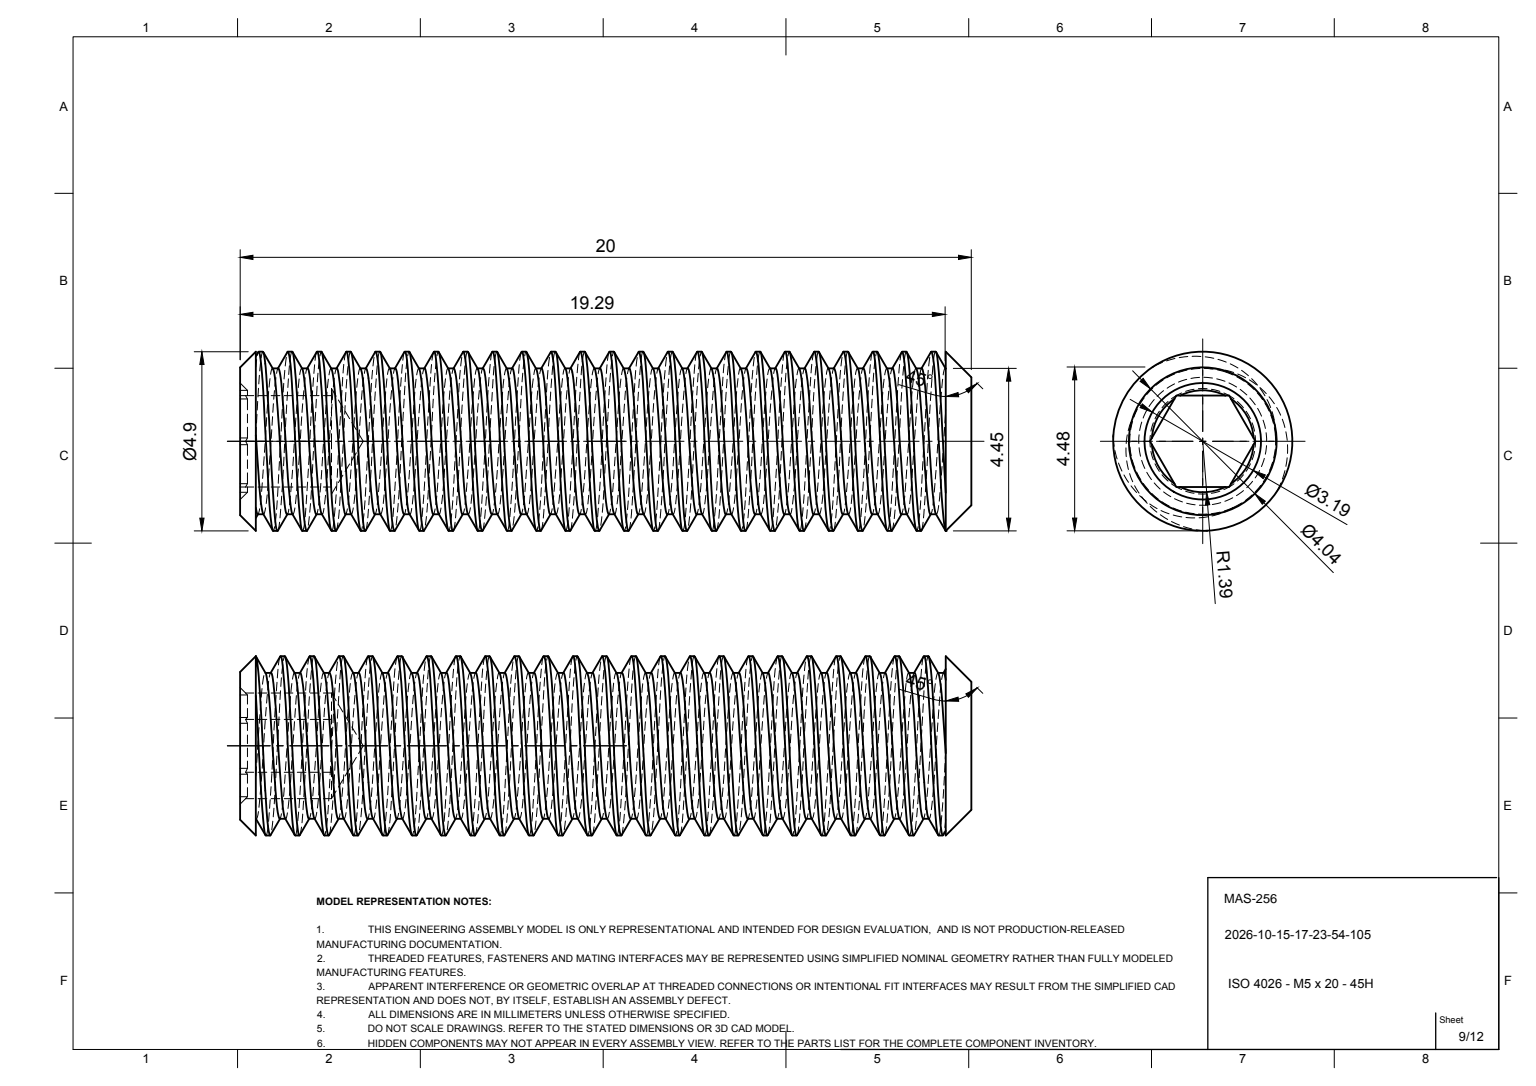
ISO-10303-21;
HEADER;
/* Generated by software containing ST-Developer
 * from STEP Tools, Inc. (www.steptools.com) 
 */

FILE_DESCRIPTION(
/* description */ (''),
/* implementation_level */ '2;1');

FILE_NAME(
/* name */ 'ISO 4026 - M5 x 20 - 45H.step',
/* time_stamp */ '2026-10-14T18:40:07-07:00',
/* author */ (''),
/* organization */ (''),
/* preprocessor_version */ 'ST-DEVELOPER v20.2',
/* originating_system */ 'Autodesk Translation Framework v15.15.0.0',
/* authorisation */ '');

FILE_SCHEMA (('AUTOMOTIVE_DESIGN { 1 0 10303 214 3 1 1 }'));
ENDSEC;

DATA;
#10=MECHANICAL_DESIGN_GEOMETRIC_PRESENTATION_REPRESENTATION('',(#838),#81040);
#344=(
BOUNDED_CURVE()
B_SPLINE_CURVE(2,(#63186,#63187,#63188),.UNSPECIFIED.,.F.,.F.)
B_SPLINE_CURVE_WITH_KNOTS((3,3),(0.,0.0126130588257634),.UNSPECIFIED.)
CURVE()
GEOMETRIC_REPRESENTATION_ITEM()
RATIONAL_B_SPLINE_CURVE((1.,1.00234596681246,1.00329298027559))
REPRESENTATION_ITEM('')
);
#345=(
BOUNDED_CURVE()
B_SPLINE_CURVE(2,(#63192,#63193,#63194),.UNSPECIFIED.,.F.,.F.)
B_SPLINE_CURVE_WITH_KNOTS((3,3),(0.0296897347922137,0.0423027936179765),
 .UNSPECIFIED.)
CURVE()
GEOMETRIC_REPRESENTATION_ITEM()
RATIONAL_B_SPLINE_CURVE((1.00329298027598,1.00234596681273,1.))
REPRESENTATION_ITEM('')
);
#346=(
BOUNDED_CURVE()
B_SPLINE_CURVE(2,(#63196,#63197,#63198),.UNSPECIFIED.,.F.,.F.)
B_SPLINE_CURVE_WITH_KNOTS((3,3),(0.,0.0126130588257622),.UNSPECIFIED.)
CURVE()
GEOMETRIC_REPRESENTATION_ITEM()
RATIONAL_B_SPLINE_CURVE((1.,1.00234596681263,1.00329298027583))
REPRESENTATION_ITEM('')
);
#347=(
BOUNDED_CURVE()
B_SPLINE_CURVE(2,(#63202,#63203,#63204),.UNSPECIFIED.,.F.,.F.)
B_SPLINE_CURVE_WITH_KNOTS((3,3),(0.0296897347922138,0.0423027936179762),
 .UNSPECIFIED.)
CURVE()
GEOMETRIC_REPRESENTATION_ITEM()
RATIONAL_B_SPLINE_CURVE((1.00329298027583,1.00234596681263,1.))
REPRESENTATION_ITEM('')
);
#348=(
BOUNDED_CURVE()
B_SPLINE_CURVE(2,(#63206,#63207,#63208),.UNSPECIFIED.,.F.,.F.)
B_SPLINE_CURVE_WITH_KNOTS((3,3),(0.,0.0126130588257628),.UNSPECIFIED.)
CURVE()
GEOMETRIC_REPRESENTATION_ITEM()
RATIONAL_B_SPLINE_CURVE((1.,1.00234596681273,1.00329298027598))
REPRESENTATION_ITEM('')
);
#349=(
BOUNDED_CURVE()
B_SPLINE_CURVE(2,(#63212,#63213,#63214),.UNSPECIFIED.,.F.,.F.)
B_SPLINE_CURVE_WITH_KNOTS((3,3),(0.0296897347922133,0.0423027936179766),
 .UNSPECIFIED.)
CURVE()
GEOMETRIC_REPRESENTATION_ITEM()
RATIONAL_B_SPLINE_CURVE((1.00329298027559,1.00234596681246,1.))
REPRESENTATION_ITEM('')
);
#350=(
BOUNDED_CURVE()
B_SPLINE_CURVE(2,(#63216,#63217,#63218),.UNSPECIFIED.,.F.,.F.)
B_SPLINE_CURVE_WITH_KNOTS((3,3),(0.,0.0126130588257654),.UNSPECIFIED.)
CURVE()
GEOMETRIC_REPRESENTATION_ITEM()
RATIONAL_B_SPLINE_CURVE((1.,1.00234596681226,1.00329298027532))
REPRESENTATION_ITEM('')
);
#351=(
BOUNDED_CURVE()
B_SPLINE_CURVE(2,(#63222,#63223,#63224),.UNSPECIFIED.,.F.,.F.)
B_SPLINE_CURVE_WITH_KNOTS((3,3),(0.029689734792212,0.0423027936179753),
 .UNSPECIFIED.)
CURVE()
GEOMETRIC_REPRESENTATION_ITEM()
RATIONAL_B_SPLINE_CURVE((1.00329298027571,1.00234596681254,1.))
REPRESENTATION_ITEM('')
);
#352=(
BOUNDED_CURVE()
B_SPLINE_CURVE(2,(#63226,#63227,#63228),.UNSPECIFIED.,.F.,.F.)
B_SPLINE_CURVE_WITH_KNOTS((3,3),(0.,0.0126130588257619),.UNSPECIFIED.)
CURVE()
GEOMETRIC_REPRESENTATION_ITEM()
RATIONAL_B_SPLINE_CURVE((1.,1.00234596681263,1.00329298027583))
REPRESENTATION_ITEM('')
);
#353=(
BOUNDED_CURVE()
B_SPLINE_CURVE(2,(#63232,#63233,#63234),.UNSPECIFIED.,.F.,.F.)
B_SPLINE_CURVE_WITH_KNOTS((3,3),(0.0296897347922146,0.0423027936179762),
 .UNSPECIFIED.)
CURVE()
GEOMETRIC_REPRESENTATION_ITEM()
RATIONAL_B_SPLINE_CURVE((1.00329298027583,1.00234596681263,1.))
REPRESENTATION_ITEM('')
);
#354=(
BOUNDED_CURVE()
B_SPLINE_CURVE(2,(#63236,#63237,#63238),.UNSPECIFIED.,.F.,.F.)
B_SPLINE_CURVE_WITH_KNOTS((3,3),(0.,0.0126130588257574),.UNSPECIFIED.)
CURVE()
GEOMETRIC_REPRESENTATION_ITEM()
RATIONAL_B_SPLINE_CURVE((1.,1.002345966813,1.00329298027635))
REPRESENTATION_ITEM('')
);
#355=(
BOUNDED_CURVE()
B_SPLINE_CURVE(2,(#63241,#63242,#63243),.UNSPECIFIED.,.F.,.F.)
B_SPLINE_CURVE_WITH_KNOTS((3,3),(0.029689734792213,0.0423027936179761),
 .UNSPECIFIED.)
CURVE()
GEOMETRIC_REPRESENTATION_ITEM()
RATIONAL_B_SPLINE_CURVE((1.00329298027557,1.00234596681244,1.))
REPRESENTATION_ITEM('')
);
#366=B_SPLINE_SURFACE_WITH_KNOTS('',3,3,((#61760,#61761,#61762,#61763,#61764,
#61765,#61766,#61767,#61768,#61769,#61770,#61771,#61772,#61773,#61774,#61775,
#61776,#61777,#61778,#61779,#61780,#61781,#61782,#61783,#61784,#61785,#61786,
#61787,#61788,#61789,#61790,#61791,#61792,#61793,#61794,#61795,#61796,#61797,
#61798,#61799,#61800,#61801,#61802,#61803,#61804,#61805,#61806,#61807,#61808,
#61809,#61810,#61811,#61812,#61813,#61814,#61815,#61816,#61817,#61818,#61819,
#61820,#61821,#61822,#61823,#61824,#61825,#61826,#61827,#61828,#61829,#61830,
#61831,#61832,#61833,#61834,#61835,#61836,#61837,#61838,#61839,#61840,#61841,
#61842,#61843,#61844,#61845,#61846,#61847,#61848,#61849,#61850,#61851,#61852,
#61853,#61854,#61855,#61856,#61857,#61858,#61859,#61860,#61861,#61862,#61863,
#61864,#61865,#61866,#61867,#61868,#61869,#61870,#61871,#61872,#61873,#61874,
#61875,#61876,#61877,#61878,#61879,#61880,#61881,#61882,#61883,#61884,#61885,
#61886,#61887,#61888,#61889,#61890,#61891,#61892,#61893,#61894,#61895,#61896,
#61897,#61898,#61899,#61900,#61901,#61902,#61903,#61904,#61905,#61906,#61907,
#61908,#61909,#61910,#61911,#61912,#61913),(#61914,#61915,#61916,#61917,
#61918,#61919,#61920,#61921,#61922,#61923,#61924,#61925,#61926,#61927,#61928,
#61929,#61930,#61931,#61932,#61933,#61934,#61935,#61936,#61937,#61938,#61939,
#61940,#61941,#61942,#61943,#61944,#61945,#61946,#61947,#61948,#61949,#61950,
#61951,#61952,#61953,#61954,#61955,#61956,#61957,#61958,#61959,#61960,#61961,
#61962,#61963,#61964,#61965,#61966,#61967,#61968,#61969,#61970,#61971,#61972,
#61973,#61974,#61975,#61976,#61977,#61978,#61979,#61980,#61981,#61982,#61983,
#61984,#61985,#61986,#61987,#61988,#61989,#61990,#61991,#61992,#61993,#61994,
#61995,#61996,#61997,#61998,#61999,#62000,#62001,#62002,#62003,#62004,#62005,
#62006,#62007,#62008,#62009,#62010,#62011,#62012,#62013,#62014,#62015,#62016,
#62017,#62018,#62019,#62020,#62021,#62022,#62023,#62024,#62025,#62026,#62027,
#62028,#62029,#62030,#62031,#62032,#62033,#62034,#62035,#62036,#62037,#62038,
#62039,#62040,#62041,#62042,#62043,#62044,#62045,#62046,#62047,#62048,#62049,
#62050,#62051,#62052,#62053,#62054,#62055,#62056,#62057,#62058,#62059,#62060,
#62061,#62062,#62063,#62064,#62065,#62066,#62067),(#62068,#62069,#62070,
#62071,#62072,#62073,#62074,#62075,#62076,#62077,#62078,#62079,#62080,#62081,
#62082,#62083,#62084,#62085,#62086,#62087,#62088,#62089,#62090,#62091,#62092,
#62093,#62094,#62095,#62096,#62097,#62098,#62099,#62100,#62101,#62102,#62103,
#62104,#62105,#62106,#62107,#62108,#62109,#62110,#62111,#62112,#62113,#62114,
#62115,#62116,#62117,#62118,#62119,#62120,#62121,#62122,#62123,#62124,#62125,
#62126,#62127,#62128,#62129,#62130,#62131,#62132,#62133,#62134,#62135,#62136,
#62137,#62138,#62139,#62140,#62141,#62142,#62143,#62144,#62145,#62146,#62147,
#62148,#62149,#62150,#62151,#62152,#62153,#62154,#62155,#62156,#62157,#62158,
#62159,#62160,#62161,#62162,#62163,#62164,#62165,#62166,#62167,#62168,#62169,
#62170,#62171,#62172,#62173,#62174,#62175,#62176,#62177,#62178,#62179,#62180,
#62181,#62182,#62183,#62184,#62185,#62186,#62187,#62188,#62189,#62190,#62191,
#62192,#62193,#62194,#62195,#62196,#62197,#62198,#62199,#62200,#62201,#62202,
#62203,#62204,#62205,#62206,#62207,#62208,#62209,#62210,#62211,#62212,#62213,
#62214,#62215,#62216,#62217,#62218,#62219,#62220,#62221),(#62222,#62223,
#62224,#62225,#62226,#62227,#62228,#62229,#62230,#62231,#62232,#62233,#62234,
#62235,#62236,#62237,#62238,#62239,#62240,#62241,#62242,#62243,#62244,#62245,
#62246,#62247,#62248,#62249,#62250,#62251,#62252,#62253,#62254,#62255,#62256,
#62257,#62258,#62259,#62260,#62261,#62262,#62263,#62264,#62265,#62266,#62267,
#62268,#62269,#62270,#62271,#62272,#62273,#62274,#62275,#62276,#62277,#62278,
#62279,#62280,#62281,#62282,#62283,#62284,#62285,#62286,#62287,#62288,#62289,
#62290,#62291,#62292,#62293,#62294,#62295,#62296,#62297,#62298,#62299,#62300,
#62301,#62302,#62303,#62304,#62305,#62306,#62307,#62308,#62309,#62310,#62311,
#62312,#62313,#62314,#62315,#62316,#62317,#62318,#62319,#62320,#62321,#62322,
#62323,#62324,#62325,#62326,#62327,#62328,#62329,#62330,#62331,#62332,#62333,
#62334,#62335,#62336,#62337,#62338,#62339,#62340,#62341,#62342,#62343,#62344,
#62345,#62346,#62347,#62348,#62349,#62350,#62351,#62352,#62353,#62354,#62355,
#62356,#62357,#62358,#62359,#62360,#62361,#62362,#62363,#62364,#62365,#62366,
#62367,#62368,#62369,#62370,#62371,#62372,#62373,#62374,#62375)),
 .UNSPECIFIED.,.F.,.F.,.F.,(4,4),(4,1,1,1,1,1,1,1,1,1,1,1,1,1,1,1,1,1,1,
1,1,1,1,1,1,1,1,1,1,1,1,1,1,1,1,1,1,1,1,1,1,1,1,1,1,1,1,1,1,1,1,1,1,1,1,
1,1,1,1,1,1,1,1,1,1,1,1,1,1,1,1,1,1,1,1,1,1,1,1,1,1,1,1,1,1,1,1,1,1,1,1,
1,1,1,1,1,1,1,1,1,1,1,1,1,1,1,1,1,1,1,1,1,1,1,1,1,1,1,1,1,1,1,1,1,1,1,1,
1,1,1,1,1,1,1,1,1,1,1,1,1,1,1,1,1,1,1,1,1,1,1,1,4),(-0.000410693813861421,
0.0529897430905959),(8.30815772716268,9.30327942982552,10.2984011324884,
11.2935228351512,12.288644537814,13.2837662404769,14.2788879431397,15.2740096458026,
16.2691313484654,17.2642530511282,18.2593747537911,19.2544964564539,20.2496181591168,
21.2447398617796,22.2398615644424,23.2349832671053,24.2301049697681,25.225226672431,
26.2203483750938,27.2154700777567,28.2105917804195,29.2057134830823,30.2008351857452,
31.195956888408,32.1910785910709,33.1862002937337,34.1813219963965,35.1764436990594,
36.1715654017222,37.1666871043851,38.1618088070479,39.1569305097107,40.1520522123736,
41.1471739150364,42.1422956176993,43.1374173203621,44.132539023025,45.1276607256878,
46.1227824283506,47.1179041310135,48.1130258336763,49.1081475363392,50.103269239002,
51.0983909416648,52.0935126443277,53.0886343469905,54.0837560496534,55.0788777523162,
56.073999454979,57.0691211576419,58.0642428603047,59.0593645629676,60.0544862656304,
61.0496079682933,62.0447296709561,63.0398513736189,64.0349730762818,65.0300947789446,
66.0252164816075,67.0203381842703,68.0154598869331,69.010581589596,70.0057032922588,
71.0008249949217,71.9959466975845,72.9910684002473,73.9861901029102,74.981311805573,
75.9764335082359,76.9715552108987,77.9666769135615,78.9617986162244,79.9569203188872,
80.9520420215501,81.9471637242129,82.9422854268758,83.9374071295386,84.9325288322014,
85.9276505348643,86.9227722375271,87.91789394019,88.9130156428528,89.9081373455156,
90.9032590481785,91.8983807508413,92.8935024535042,93.888624156167,94.8837458588298,
95.8788675614927,96.8739892641555,97.8691109668184,98.8642326694812,99.859354372144,
100.854476074807,101.84959777747,102.844719480133,103.839841182795,104.834962885458,
105.830084588121,106.825206290784,107.820327993447,108.81544969611,109.810571398772,
110.805693101435,111.800814804098,112.795936506761,113.791058209424,114.786179912087,
115.781301614749,116.776423317412,117.771545020075,118.766666722738,119.761788425401,
120.756910128064,121.752031830727,122.747153533389,123.742275236052,124.737396938715,
125.732518641378,126.727640344041,127.722762046704,128.717883749366,129.713005452029,
130.708127154692,131.703248857355,132.698370560018,133.693492262681,134.688613965343,
135.683735668006,136.678857370669,137.673979073332,138.669100775995,139.664222478658,
140.659344181321,141.654465883983,142.649587586646,143.644709289309,144.639830991972,
145.634952694635,146.630074397298,147.62519609996,148.620317802623,149.615439505286,
150.610561207949,151.605682910612,152.600804613275,153.595926315937,154.5910480186,
155.586169721263,156.581291423926,157.576413126589,158.571945523066),
 .UNSPECIFIED.);
#367=B_SPLINE_SURFACE_WITH_KNOTS('',3,3,((#62563,#62564,#62565,#62566,#62567,
#62568,#62569,#62570,#62571,#62572,#62573,#62574,#62575,#62576,#62577,#62578,
#62579,#62580,#62581,#62582,#62583,#62584,#62585,#62586,#62587,#62588,#62589,
#62590,#62591,#62592,#62593,#62594,#62595,#62596,#62597,#62598,#62599,#62600,
#62601,#62602,#62603,#62604,#62605,#62606,#62607,#62608,#62609,#62610,#62611,
#62612,#62613,#62614,#62615,#62616,#62617,#62618,#62619,#62620,#62621,#62622,
#62623,#62624,#62625,#62626,#62627,#62628,#62629,#62630,#62631,#62632,#62633,
#62634,#62635,#62636,#62637,#62638,#62639,#62640,#62641,#62642,#62643,#62644,
#62645,#62646,#62647,#62648,#62649,#62650,#62651,#62652,#62653,#62654,#62655,
#62656,#62657,#62658,#62659,#62660,#62661,#62662,#62663,#62664,#62665,#62666,
#62667,#62668,#62669,#62670,#62671,#62672,#62673,#62674,#62675,#62676,#62677,
#62678,#62679,#62680,#62681,#62682,#62683,#62684,#62685,#62686,#62687,#62688,
#62689,#62690,#62691,#62692,#62693,#62694,#62695,#62696,#62697,#62698,#62699,
#62700,#62701,#62702,#62703,#62704,#62705,#62706,#62707,#62708,#62709,#62710,
#62711,#62712,#62713,#62714,#62715,#62716),(#62717,#62718,#62719,#62720,
#62721,#62722,#62723,#62724,#62725,#62726,#62727,#62728,#62729,#62730,#62731,
#62732,#62733,#62734,#62735,#62736,#62737,#62738,#62739,#62740,#62741,#62742,
#62743,#62744,#62745,#62746,#62747,#62748,#62749,#62750,#62751,#62752,#62753,
#62754,#62755,#62756,#62757,#62758,#62759,#62760,#62761,#62762,#62763,#62764,
#62765,#62766,#62767,#62768,#62769,#62770,#62771,#62772,#62773,#62774,#62775,
#62776,#62777,#62778,#62779,#62780,#62781,#62782,#62783,#62784,#62785,#62786,
#62787,#62788,#62789,#62790,#62791,#62792,#62793,#62794,#62795,#62796,#62797,
#62798,#62799,#62800,#62801,#62802,#62803,#62804,#62805,#62806,#62807,#62808,
#62809,#62810,#62811,#62812,#62813,#62814,#62815,#62816,#62817,#62818,#62819,
#62820,#62821,#62822,#62823,#62824,#62825,#62826,#62827,#62828,#62829,#62830,
#62831,#62832,#62833,#62834,#62835,#62836,#62837,#62838,#62839,#62840,#62841,
#62842,#62843,#62844,#62845,#62846,#62847,#62848,#62849,#62850,#62851,#62852,
#62853,#62854,#62855,#62856,#62857,#62858,#62859,#62860,#62861,#62862,#62863,
#62864,#62865,#62866,#62867,#62868,#62869,#62870),(#62871,#62872,#62873,
#62874,#62875,#62876,#62877,#62878,#62879,#62880,#62881,#62882,#62883,#62884,
#62885,#62886,#62887,#62888,#62889,#62890,#62891,#62892,#62893,#62894,#62895,
#62896,#62897,#62898,#62899,#62900,#62901,#62902,#62903,#62904,#62905,#62906,
#62907,#62908,#62909,#62910,#62911,#62912,#62913,#62914,#62915,#62916,#62917,
#62918,#62919,#62920,#62921,#62922,#62923,#62924,#62925,#62926,#62927,#62928,
#62929,#62930,#62931,#62932,#62933,#62934,#62935,#62936,#62937,#62938,#62939,
#62940,#62941,#62942,#62943,#62944,#62945,#62946,#62947,#62948,#62949,#62950,
#62951,#62952,#62953,#62954,#62955,#62956,#62957,#62958,#62959,#62960,#62961,
#62962,#62963,#62964,#62965,#62966,#62967,#62968,#62969,#62970,#62971,#62972,
#62973,#62974,#62975,#62976,#62977,#62978,#62979,#62980,#62981,#62982,#62983,
#62984,#62985,#62986,#62987,#62988,#62989,#62990,#62991,#62992,#62993,#62994,
#62995,#62996,#62997,#62998,#62999,#63000,#63001,#63002,#63003,#63004,#63005,
#63006,#63007,#63008,#63009,#63010,#63011,#63012,#63013,#63014,#63015,#63016,
#63017,#63018,#63019,#63020,#63021,#63022,#63023,#63024),(#63025,#63026,
#63027,#63028,#63029,#63030,#63031,#63032,#63033,#63034,#63035,#63036,#63037,
#63038,#63039,#63040,#63041,#63042,#63043,#63044,#63045,#63046,#63047,#63048,
#63049,#63050,#63051,#63052,#63053,#63054,#63055,#63056,#63057,#63058,#63059,
#63060,#63061,#63062,#63063,#63064,#63065,#63066,#63067,#63068,#63069,#63070,
#63071,#63072,#63073,#63074,#63075,#63076,#63077,#63078,#63079,#63080,#63081,
#63082,#63083,#63084,#63085,#63086,#63087,#63088,#63089,#63090,#63091,#63092,
#63093,#63094,#63095,#63096,#63097,#63098,#63099,#63100,#63101,#63102,#63103,
#63104,#63105,#63106,#63107,#63108,#63109,#63110,#63111,#63112,#63113,#63114,
#63115,#63116,#63117,#63118,#63119,#63120,#63121,#63122,#63123,#63124,#63125,
#63126,#63127,#63128,#63129,#63130,#63131,#63132,#63133,#63134,#63135,#63136,
#63137,#63138,#63139,#63140,#63141,#63142,#63143,#63144,#63145,#63146,#63147,
#63148,#63149,#63150,#63151,#63152,#63153,#63154,#63155,#63156,#63157,#63158,
#63159,#63160,#63161,#63162,#63163,#63164,#63165,#63166,#63167,#63168,#63169,
#63170,#63171,#63172,#63173,#63174,#63175,#63176,#63177,#63178)),
 .UNSPECIFIED.,.F.,.F.,.F.,(4,4),(4,1,1,1,1,1,1,1,1,1,1,1,1,1,1,1,1,1,1,
1,1,1,1,1,1,1,1,1,1,1,1,1,1,1,1,1,1,1,1,1,1,1,1,1,1,1,1,1,1,1,1,1,1,1,1,
1,1,1,1,1,1,1,1,1,1,1,1,1,1,1,1,1,1,1,1,1,1,1,1,1,1,1,1,1,1,1,1,1,1,1,1,
1,1,1,1,1,1,1,1,1,1,1,1,1,1,1,1,1,1,1,1,1,1,1,1,1,1,1,1,1,1,1,1,1,1,1,1,
1,1,1,1,1,1,1,1,1,1,1,1,1,1,1,1,1,1,1,1,1,1,1,1,4),(-0.000364258179702487,
0.0530361410367657),(11.6159825333414,12.6115149000043,13.6066366026672,
14.60175830533,15.5968800079929,16.5920017106557,17.5871234133185,18.5822451159814,
19.5773668186442,20.5724885213071,21.5676102239699,22.5627319266327,23.5578536292956,
24.5529753319584,25.5480970346213,26.5432187372841,27.5383404399469,28.5334621426098,
29.5285838452726,30.5237055479355,31.5188272505983,32.5139489532611,33.509070655924,
34.5041923585868,35.4993140612497,36.4944357639125,37.4895574665754,38.4846791692382,
39.479800871901,40.4749225745639,41.4700442772267,42.4651659798896,43.4602876825524,
44.4554093852152,45.4505310878781,46.4456527905409,47.4407744932038,48.4358961958666,
49.4310178985294,50.4261396011923,51.4212613038551,52.416383006518,53.4115047091808,
54.4066264118436,55.4017481145065,56.3968698171693,57.3919915198322,58.387113222495,
59.3822349251579,60.3773566278207,61.3724783304835,62.3676000331464,63.3627217358092,
64.3578434384721,65.3529651411349,66.3480868437977,67.3432085464606,68.3383302491234,
69.3334519517863,70.3285736544491,71.3236953571119,72.3188170597748,73.3139387624376,
74.3090604651005,75.3041821677633,76.2993038704262,77.294425573089,78.2895472757518,
79.2846689784147,80.2797906810775,81.2749123837404,82.2700340864032,83.265155789066,
84.2602774917289,85.2553991943917,86.2505208970546,87.2456425997174,88.2407643023802,
89.2358860050431,90.2310077077059,91.2261294103688,92.2212511130316,93.2163728156945,
94.2114945183573,95.2066162210201,96.201737923683,97.1968596263458,98.1919813290087,
99.1871030316715,100.182224734334,101.177346436997,102.17246813966,103.167589842323,
104.162711544986,105.157833247649,106.152954950311,107.148076652974,108.143198355637,
109.1383200583,110.133441760963,111.128563463626,112.123685166288,113.118806868951,
114.113928571614,115.109050274277,116.10417197694,117.099293679603,118.094415382265,
119.089537084928,120.084658787591,121.079780490254,122.074902192917,123.07002389558,
124.065145598243,125.060267300905,126.055389003568,127.050510706231,128.045632408894,
129.040754111557,130.03587581422,131.030997516882,132.026119219545,133.021240922208,
134.016362624871,135.011484327534,136.006606030197,137.001727732859,137.996849435522,
138.991971138185,139.987092840848,140.982214543511,141.977336246174,142.972457948837,
143.967579651499,144.962701354162,145.957823056825,146.952944759488,147.948066462151,
148.943188164814,149.938309867476,150.933431570139,151.928553272802,152.923674975465,
153.918796678128,154.913918380791,155.909040083453,156.904161786116,157.899283488779,
158.894405191442,159.889526894105,160.884648596768,161.87977029943),
 .UNSPECIFIED.);
#543=B_SPLINE_CURVE_WITH_KNOTS('',3,(#43212,#43213,#43214,#43215,#43216,
#43217,#43218,#43219,#43220,#43221,#43222,#43223,#43224,#43225,#43226,#43227,
#43228,#43229,#43230,#43231,#43232,#43233,#43234,#43235,#43236,#43237,#43238,
#43239,#43240,#43241,#43242,#43243,#43244,#43245,#43246,#43247,#43248,#43249,
#43250,#43251,#43252,#43253,#43254,#43255,#43256,#43257,#43258,#43259,#43260,
#43261,#43262,#43263,#43264,#43265,#43266,#43267,#43268,#43269,#43270,#43271,
#43272,#43273,#43274,#43275,#43276,#43277,#43278,#43279,#43280,#43281,#43282,
#43283,#43284,#43285,#43286,#43287,#43288,#43289,#43290,#43291,#43292,#43293,
#43294,#43295,#43296,#43297,#43298,#43299,#43300,#43301,#43302,#43303,#43304,
#43305,#43306,#43307,#43308,#43309,#43310,#43311,#43312,#43313,#43314,#43315,
#43316,#43317,#43318,#43319,#43320,#43321,#43322,#43323,#43324,#43325,#43326,
#43327,#43328,#43329,#43330,#43331,#43332,#43333,#43334,#43335,#43336,#43337,
#43338,#43339,#43340,#43341,#43342,#43343,#43344,#43345,#43346,#43347,#43348,
#43349,#43350,#43351,#43352,#43353,#43354,#43355,#43356,#43357,#43358,#43359,
#43360,#43361,#43362,#43363,#43364,#43365,#43366,#43367,#43368,#43369,#43370,
#43371,#43372,#43373,#43374,#43375,#43376,#43377,#43378,#43379,#43380,#43381,
#43382,#43383,#43384,#43385),.UNSPECIFIED.,.F.,.F.,(4,2,2,2,2,2,2,2,2,2,
2,2,2,2,2,2,2,2,2,2,2,2,2,2,2,2,2,2,2,2,2,2,2,2,2,2,2,2,2,2,2,2,2,2,2,2,
2,2,2,2,2,2,2,2,2,2,2,2,2,2,2,2,2,2,2,2,2,2,2,2,2,2,2,2,2,2,2,2,2,2,2,2,
2,2,2,2,4),(-1.02623154465591,-1.02612355094225,-1.0171949105878,-1.00173095718431,
-0.985469014925391,-0.982771946333453,-0.981106865955899,-0.979811649677182,
-0.978304805833221,-0.975593204166809,-0.962004888593598,-0.929009570235146,
-0.890102622931837,-0.885357205821845,-0.882392485048737,-0.88007255803002,
-0.87749442072948,-0.873218763358691,-0.856815386493199,-0.795998925748137,
-0.785774339547155,-0.783194740653446,-0.781700335240677,-0.780528775129861,
-0.778903222255259,-0.775642448166408,-0.771379179015789,-0.761149449011797,
-0.715168121526073,-0.690933730558083,-0.686443744461884,-0.683553504484392,
-0.681237215680206,-0.678604823233647,-0.674096245039031,-0.654637962169762,
-0.609759140741896,-0.587984786080504,-0.584837995230912,-0.583218043592144,
-0.581928744021515,-0.580398002638214,-0.577543750440399,-0.560583467376236,
-0.531668237094072,-0.491978203796283,-0.487259509009561,-0.48431303144165,
-0.482008603588994,-0.479449131679121,-0.475208298310883,-0.459005836096745,
-0.427573337459186,-0.416862164322599,-0.411468759639921,-0.388730249711721,
-0.385591832645818,-0.383978822110257,-0.382688106401478,-0.381143962853957,
-0.378268391996503,-0.361258822960958,-0.332370712217255,-0.292727546811052,
-0.287970926659497,-0.28499512806325,-0.282663948925388,-0.28007054667004,
-0.275762761562799,-0.259131125602471,-0.194877347651408,-0.187936721290845,
-0.185704718486579,-0.184300457443206,-0.182978277960871,-0.181156364600397,
-0.176843676191297,-0.156826183459693,-0.104384960191217,-0.0934748581158038,
-0.0896010514422441,-0.0873381573714681,-0.0849755616014679,-0.0818995433479831,
-0.0753249891341137,-0.0493613703757626,-0.00320473719929889),
 .UNSPECIFIED.);
#544=B_SPLINE_CURVE_WITH_KNOTS('',3,(#43388,#43389,#43390,#43391,#43392,
#43393,#43394,#43395,#43396,#43397,#43398,#43399,#43400,#43401,#43402,#43403,
#43404,#43405,#43406,#43407,#43408,#43409,#43410,#43411,#43412,#43413,#43414,
#43415,#43416,#43417,#43418,#43419,#43420,#43421,#43422,#43423,#43424,#43425,
#43426,#43427,#43428,#43429,#43430,#43431,#43432,#43433,#43434,#43435,#43436,
#43437,#43438,#43439,#43440,#43441,#43442,#43443,#43444,#43445,#43446,#43447,
#43448,#43449,#43450,#43451,#43452,#43453,#43454,#43455,#43456,#43457,#43458,
#43459,#43460,#43461,#43462,#43463,#43464,#43465,#43466,#43467,#43468,#43469,
#43470,#43471,#43472,#43473,#43474,#43475,#43476,#43477,#43478,#43479,#43480,
#43481,#43482,#43483,#43484,#43485,#43486,#43487,#43488,#43489,#43490,#43491,
#43492,#43493,#43494,#43495,#43496,#43497,#43498,#43499,#43500,#43501,#43502,
#43503,#43504,#43505),.UNSPECIFIED.,.F.,.F.,(4,3,3,3,3,3,3,3,3,3,3,3,3,
3,3,3,3,3,3,3,3,3,3,3,3,3,3,3,3,3,3,3,3,3,3,3,3,3,3,4),(11.6163931973415,
11.7237672656018,11.8347357199021,11.9420294578483,12.0493244336209,12.1566495119213,
12.264033585161,12.3715827272617,12.4792279734473,12.5870706422788,12.6115149000043,
12.7155317843677,12.8193765837255,12.9230806912589,13.0267085981463,13.1302971854635,
13.2338832777977,13.3375740056834,13.4413213587812,13.5452523118071,13.6066366026672,
13.7117447872625,13.8166959584208,13.9215236686367,14.0262853677174,14.1310163775997,
14.2357519758657,14.3405953724673,14.4454990552932,14.5505798283899,14.60175830533,
14.7069309232771,14.8119246326924,14.9168178106501,15.0216457587039,15.1264436979783,
15.2312999910099,15.3361865597888,15.4412122486148,15.503392487373),
 .UNSPECIFIED.);
#545=B_SPLINE_CURVE_WITH_KNOTS('',3,(#43510,#43511,#43512,#43513,#43514,
#43515,#43516,#43517,#43518,#43519,#43520,#43521,#43522,#43523,#43524,#43525,
#43526,#43527,#43528,#43529,#43530,#43531,#43532,#43533,#43534,#43535,#43536,
#43537,#43538,#43539,#43540,#43541,#43542,#43543,#43544,#43545,#43546,#43547,
#43548,#43549,#43550,#43551,#43552,#43553,#43554,#43555,#43556,#43557,#43558,
#43559,#43560,#43561,#43562,#43563,#43564,#43565,#43566,#43567,#43568,#43569,
#43570,#43571,#43572,#43573,#43574,#43575,#43576,#43577,#43578,#43579,#43580,
#43581,#43582,#43583,#43584,#43585,#43586,#43587,#43588,#43589,#43590,#43591,
#43592,#43593,#43594,#43595,#43596,#43597,#43598,#43599,#43600,#43601,#43602,
#43603,#43604,#43605,#43606,#43607,#43608,#43609,#43610,#43611,#43612,#43613,
#43614,#43615,#43616,#43617,#43618,#43619,#43620,#43621,#43622,#43623,#43624,
#43625,#43626,#43627,#43628,#43629,#43630,#43631,#43632,#43633,#43634,#43635,
#43636,#43637,#43638,#43639,#43640,#43641,#43642,#43643,#43644,#43645,#43646,
#43647,#43648,#43649,#43650,#43651,#43652,#43653,#43654,#43655,#43656,#43657,
#43658,#43659,#43660,#43661,#43662,#43663,#43664,#43665,#43666,#43667,#43668,
#43669,#43670,#43671,#43672,#43673,#43674,#43675,#43676,#43677,#43678,#43679,
#43680,#43681,#43682,#43683,#43684,#43685,#43686,#43687,#43688,#43689,#43690,
#43691,#43692,#43693,#43694,#43695,#43696,#43697,#43698,#43699,#43700,#43701,
#43702,#43703,#43704,#43705,#43706,#43707,#43708,#43709,#43710,#43711,#43712,
#43713,#43714,#43715,#43716,#43717,#43718,#43719,#43720,#43721,#43722,#43723,
#43724,#43725,#43726,#43727),.UNSPECIFIED.,.F.,.F.,(4,2,2,2,2,2,2,2,2,2,
2,2,2,2,2,2,2,2,2,2,2,2,2,2,2,2,2,2,2,2,2,2,2,2,2,2,2,2,2,2,2,2,2,2,2,2,
2,2,2,2,2,2,2,2,2,2,2,2,2,2,2,2,2,2,2,2,2,2,2,2,2,2,2,2,2,2,2,2,2,2,2,2,
2,2,2,2,2,2,2,2,2,2,2,2,2,2,2,2,2,2,2,2,2,2,2,2,2,2,4),(-2.28248600441818,
-2.2811956203742,-2.27687867721623,-2.27429210537512,-2.27220672013212,
-2.26937453435887,-2.26390906147731,-2.22240610456411,-2.1817125094513,
-2.17715654769303,-2.17543396354253,-2.17420503146357,-2.17287531524768,
-2.17098113067247,-2.16619035367949,-2.15916593209376,-2.13720086913996,
-2.08636498668884,-2.07952178065835,-2.07645687560523,-2.07411645664894,
-2.07161205809893,-2.06766952812952,-2.05478977904954,-2.03300524837185,
-2.00749534956624,-1.98067095547916,-1.97747634366124,-1.97584649129612,
-1.97455315241394,-1.97301858782097,-1.97017919487622,-1.9539413515156,
-1.89828031814689,-1.88325787526814,-1.87893503696039,-1.87634720382067,
-1.87426208439326,-1.87143195211724,-1.86597629628848,-1.82340189586034,
-1.78382863243893,-1.7792291896914,-1.77750098335071,-1.77627059073702,
-1.77494229662179,-1.77305485838914,-1.76830562448201,-1.74354356694527,
-1.70296881418663,-1.68482176820919,-1.6802749108557,-1.67761170307872,
-1.67530475013581,-1.67247298103653,-1.66700863526789,-1.62565360567816,
-1.58480006736649,-1.58025253527128,-1.57853116236556,-1.57730263481814,
-1.5759727918622,-1.57407758744025,-1.56927988593347,-1.56224194230279,
-1.54020668903168,-1.48947398675752,-1.48261819767435,-1.47955102359204,
-1.47721021482659,-1.47470670166459,-1.470768313846,-1.45792728125288,-1.43623945027337,
-1.41793753057054,-1.38622919963296,-1.38140332677764,-1.37944788184294,
-1.37823958839674,-1.37688861791258,-1.37488987940457,-1.36940037275679,
-1.36097330322796,-1.33073525762771,-1.29150189459091,-1.28418747392266,
-1.28124341165959,-1.27907187837465,-1.27671086179762,-1.27347240216341,
-1.26582988204842,-1.25520228059614,-1.2242321460654,-1.18720437551511,
-1.18246923433969,-1.18052893863192,-1.17920364751265,-1.1778234421524,
-1.17568254853977,-1.16908911148502,-1.15824282282221,-1.10372071610207,
-1.08761413813402,-1.08318926839738,-1.08058044249789,-1.07850064437566,
-1.0757066274937,-1.07041846733174,-1.02623154465591),.UNSPECIFIED.);
#546=B_SPLINE_CURVE_WITH_KNOTS('',3,(#43729,#43730,#43731,#43732,#43733,
#43734,#43735),.UNSPECIFIED.,.F.,.F.,(4,3,4),(15.503392487373,15.5968800079929,
15.707963267949),.UNSPECIFIED.);
#547=B_SPLINE_CURVE_WITH_KNOTS('',3,(#43736,#43737,#43738,#43739,#43740,
#43741,#43742,#43743,#43744,#43745,#43746,#43747,#43748,#43749,#43750,#43751,
#43752,#43753,#43754,#43755,#43756,#43757,#43758,#43759,#43760,#43761,#43762,
#43763,#43764,#43765,#43766,#43767,#43768,#43769,#43770,#43771,#43772,#43773,
#43774,#43775,#43776,#43777,#43778,#43779,#43780,#43781,#43782,#43783,#43784,
#43785,#43786,#43787,#43788,#43789,#43790,#43791,#43792,#43793,#43794,#43795,
#43796,#43797,#43798,#43799,#43800,#43801,#43802,#43803,#43804,#43805,#43806,
#43807,#43808,#43809,#43810,#43811,#43812,#43813,#43814,#43815,#43816,#43817,
#43818,#43819,#43820,#43821,#43822,#43823,#43824,#43825,#43826,#43827,#43828,
#43829,#43830,#43831,#43832,#43833,#43834,#43835,#43836,#43837,#43838,#43839,
#43840,#43841,#43842,#43843,#43844,#43845,#43846,#43847,#43848,#43849,#43850,
#43851,#43852,#43853,#43854,#43855,#43856,#43857,#43858,#43859,#43860,#43861,
#43862,#43863,#43864,#43865,#43866,#43867,#43868,#43869,#43870,#43871,#43872,
#43873,#43874,#43875,#43876,#43877,#43878,#43879,#43880,#43881,#43882,#43883,
#43884,#43885,#43886,#43887,#43888,#43889,#43890,#43891,#43892,#43893,#43894,
#43895,#43896,#43897,#43898,#43899,#43900,#43901,#43902,#43903,#43904,#43905,
#43906,#43907,#43908,#43909,#43910,#43911,#43912,#43913,#43914,#43915,#43916,
#43917,#43918,#43919,#43920,#43921,#43922,#43923,#43924,#43925,#43926,#43927,
#43928,#43929,#43930,#43931,#43932,#43933,#43934,#43935,#43936,#43937,#43938,
#43939,#43940,#43941,#43942,#43943,#43944,#43945,#43946,#43947,#43948,#43949),
 .UNSPECIFIED.,.F.,.F.,(4,2,2,2,2,2,2,2,2,2,2,2,2,2,2,2,2,2,2,2,2,2,2,2,
2,2,2,2,2,2,2,2,2,2,2,2,2,2,2,2,2,2,2,2,2,2,2,2,2,2,2,2,2,2,2,2,2,2,2,2,
2,2,2,2,2,2,2,2,2,2,2,2,2,2,2,2,2,2,2,2,2,2,2,2,2,2,2,2,2,2,2,2,2,2,2,2,
2,2,2,2,2,2,2,2,2,2,4),(-2.51348919495808,-2.45995851601186,-2.44925790244611,
-2.44158591510701,-2.43835650598829,-2.43601015635019,-2.4338578317885,
-2.43094871564621,-2.42376843780528,-2.37888300757562,-2.35263301679549,
-2.34484531596076,-2.34133001370335,-2.33859305270455,-2.33707981008272,
-2.33707269722718,-2.33706552307515,-2.33705828660438,-2.33577007911729,
-2.33415682383674,-2.33103861367995,-2.31009322063273,-2.27757904817603,
-2.25647341571697,-2.2438584508448,-2.23994050890193,-2.23743859686416,
-2.23509122518325,-2.2320036340304,-2.22505040650899,-2.17556520315596,
-2.15294426444102,-2.14579343223834,-2.14093587092273,-2.13902757770181,
-2.13769230437777,-2.13646400042466,-2.13474609670009,-2.13023488163978,
-2.08914229634523,-2.04807187876847,-2.04262861400778,-2.03980093767237,
-2.0377159797013,-2.0351262401371,-2.03079518447029,-2.01569288510483,-1.96004720133005,
-1.94913195234409,-1.94250852294172,-1.94036332624446,-1.93898170892837,
-1.93765828295266,-1.93572277165681,-1.93100843533646,-1.8937024317923,
-1.86296822323266,-1.85239159405453,-1.84477896167686,-1.84154836800767,
-1.83919138771524,-1.83702240249185,-1.83408005137926,-1.82676119050772,
-1.78762460911556,-1.7572348490669,-1.74878710216705,-1.7432898879598,-1.74129215945478,
-1.73994297505554,-1.73873568407142,-1.73678361862874,-1.73197564748851,
-1.69766276544465,-1.66518545527833,-1.65397499034014,-1.64601344078746,
-1.64272271925054,-1.64035279401862,-1.63819303988256,-1.63474720272636,
-1.6264172664817,-1.56276533470499,-1.54600974083554,-1.54314824158543,
-1.54160863683973,-1.540315373341,-1.53869096107488,-1.53552191650157,-1.51130281904821,
-1.47920823824311,-1.45300836406659,-1.44645045873991,-1.44340459316045,
-1.44107511265488,-1.4388518615698,-1.43506654701195,-1.42456374894158,
-1.36362634903188,-1.34701421169184,-1.34415923886547,-1.34262140174274,
-1.34132835458456,-1.33970275810793,-1.33652791435823,-1.31186486080438,
-1.29822679571031),.UNSPECIFIED.);
#548=B_SPLINE_CURVE_WITH_KNOTS('',3,(#43954,#43955,#43956,#43957,#43958,
#43959,#43960,#43961,#43962,#43963,#43964,#43965,#43966,#43967,#43968,#43969,
#43970,#43971,#43972,#43973,#43974,#43975,#43976,#43977,#43978,#43979,#43980,
#43981,#43982,#43983,#43984,#43985,#43986,#43987,#43988,#43989,#43990,#43991,
#43992,#43993,#43994,#43995,#43996,#43997,#43998,#43999,#44000,#44001,#44002,
#44003,#44004,#44005,#44006,#44007,#44008,#44009,#44010,#44011,#44012,#44013,
#44014,#44015,#44016,#44017,#44018,#44019,#44020,#44021,#44022,#44023,#44024,
#44025,#44026,#44027,#44028,#44029,#44030,#44031,#44032,#44033,#44034,#44035,
#44036,#44037,#44038,#44039,#44040,#44041,#44042,#44043,#44044,#44045,#44046,
#44047,#44048,#44049,#44050,#44051,#44052,#44053,#44054,#44055,#44056,#44057,
#44058,#44059,#44060,#44061,#44062,#44063,#44064,#44065,#44066,#44067,#44068,
#44069,#44070,#44071,#44072,#44073,#44074,#44075,#44076,#44077,#44078,#44079,
#44080,#44081,#44082,#44083,#44084,#44085,#44086,#44087,#44088,#44089,#44090,
#44091,#44092,#44093,#44094,#44095,#44096,#44097,#44098,#44099,#44100,#44101,
#44102,#44103,#44104,#44105,#44106,#44107,#44108,#44109,#44110,#44111,#44112,
#44113,#44114,#44115,#44116,#44117,#44118,#44119,#44120,#44121,#44122,#44123,
#44124,#44125,#44126,#44127,#44128,#44129,#44130,#44131,#44132,#44133,#44134,
#44135,#44136,#44137,#44138,#44139,#44140,#44141,#44142,#44143,#44144,#44145,
#44146,#44147,#44148,#44149,#44150,#44151,#44152,#44153,#44154,#44155,#44156,
#44157,#44158,#44159,#44160,#44161),.UNSPECIFIED.,.F.,.F.,(4,2,2,2,2,2,
2,2,2,2,2,2,2,2,2,2,2,2,2,2,2,2,2,2,2,2,2,2,2,2,2,2,2,2,2,2,2,2,2,2,2,2,
2,2,2,2,2,2,2,2,2,2,2,2,2,2,2,2,2,2,2,2,2,2,2,2,2,2,2,2,2,2,2,2,2,2,2,2,
2,2,2,2,2,2,2,2,2,2,2,2,2,2,2,2,2,2,2,2,2,2,2,2,2,4),(-3.53887107067202,
-3.50922941979923,-3.48733849991634,-3.47441513608124,-3.470467913123,-3.46796246119239,
-3.46562239711216,-3.46255988650963,-3.4557302926679,-3.40474048486825,
-3.38284495091239,-3.37583391707794,-3.37105038581197,-3.36915729607683,
-3.36782775521713,-3.3665985055681,-3.36487483895307,-3.36031064471525,
-3.31982533440377,-3.27816235897577,-3.27269644904552,-3.26986406919186,
-3.26755671103684,-3.26489313546167,-3.2603458836294,-3.24220191796138,
-3.20157591866347,-3.17681570460497,-3.17206648536367,-3.17017882791212,
-3.16885032819734,-3.16761981723845,-3.1658913646053,-3.16129051200363,
-3.12177121208322,-3.07920057734017,-3.07373035941,-3.0708971336758,-3.06881155608696,
-3.06622548522212,-3.0619111241625,-3.04697946666633,-2.99708607414523,
-2.98220671927603,-2.9767183889018,-2.97275102426313,-2.97099491119951,
-2.96968835147231,-2.96823377014834,-2.9657612443333,-2.95697562944232,
-2.89459661138065,-2.88367988327608,-2.87587851006771,-2.87261431699605,
-2.87024941465539,-2.86808457032404,-2.86516515011988,-2.85799153066069,
-2.81315219504935,-2.78712172843256,-2.77936190439719,-2.77419973397115,
-2.77224900268981,-2.77090836458305,-2.76969179651282,-2.76801607549204,
-2.76376836909518,-2.719655069334,-2.68136267313181,-2.67579019806618,-2.67293625034027,
-2.67064898845357,-2.66800983413166,-2.6635681375633,-2.64681610415624,
-2.59300891475173,-2.58220210556648,-2.57562530060871,-2.57348515905856,
-2.57210425470312,-2.57077848069766,-2.56883592423162,-2.56408679120747,
-2.52775288602899,-2.49631919577921,-2.48560181711695,-2.4779096554613,
-2.47466341619169,-2.47230152682221,-2.4701325213564,-2.46719697413253,
-2.45990329011298,-2.41824165612287,-2.38095092334477,-2.37622882016353,
-2.37429070004303,-2.37296574929545,-2.37158352194142,-2.36943753105829,
-2.36281254517813,-2.351896197006,-2.29615580431147,-2.28248600441818),
 .UNSPECIFIED.);
#549=B_SPLINE_CURVE_WITH_KNOTS('',3,(#44162,#44163,#44164,#44165,#44166,
#44167,#44168,#44169,#44170,#44171,#44172,#44173,#44174,#44175,#44176,#44177,
#44178,#44179,#44180,#44181,#44182,#44183,#44184,#44185,#44186,#44187,#44188,
#44189,#44190,#44191,#44192,#44193,#44194,#44195,#44196,#44197,#44198,#44199,
#44200,#44201,#44202,#44203,#44204,#44205,#44206,#44207,#44208,#44209,#44210,
#44211,#44212,#44213,#44214,#44215,#44216,#44217,#44218,#44219,#44220,#44221,
#44222,#44223,#44224,#44225,#44226,#44227,#44228,#44229,#44230,#44231,#44232,
#44233,#44234,#44235,#44236,#44237,#44238,#44239,#44240,#44241,#44242,#44243,
#44244,#44245,#44246,#44247,#44248,#44249,#44250,#44251,#44252,#44253,#44254,
#44255,#44256,#44257,#44258,#44259,#44260,#44261,#44262,#44263,#44264,#44265,
#44266,#44267,#44268,#44269,#44270,#44271,#44272,#44273,#44274,#44275,#44276,
#44277,#44278,#44279,#44280,#44281,#44282,#44283,#44284,#44285,#44286,#44287,
#44288,#44289,#44290,#44291,#44292,#44293,#44294,#44295,#44296,#44297,#44298,
#44299,#44300,#44301,#44302,#44303,#44304,#44305,#44306,#44307,#44308,#44309,
#44310,#44311,#44312,#44313,#44314,#44315,#44316,#44317,#44318,#44319,#44320,
#44321,#44322,#44323,#44324,#44325,#44326,#44327,#44328,#44329,#44330,#44331,
#44332,#44333,#44334,#44335,#44336,#44337,#44338,#44339,#44340,#44341,#44342,
#44343,#44344,#44345,#44346,#44347,#44348,#44349,#44350,#44351,#44352,#44353,
#44354,#44355,#44356,#44357,#44358,#44359,#44360,#44361,#44362,#44363,#44364,
#44365,#44366,#44367,#44368,#44369,#44370,#44371,#44372,#44373,#44374,#44375,
#44376,#44377,#44378,#44379,#44380,#44381),.UNSPECIFIED.,.F.,.F.,(4,2,2,
2,2,2,2,2,2,2,2,2,2,2,2,2,2,2,2,2,2,2,2,2,2,2,2,2,2,2,2,2,2,2,2,2,2,2,2,
2,2,2,2,2,2,2,2,2,2,2,2,2,2,2,2,2,2,2,2,2,2,2,2,2,2,2,2,2,2,2,2,2,2,2,2,
2,2,2,2,2,2,2,2,2,2,2,2,2,2,2,2,2,2,2,2,2,2,2,2,2,2,2,2,2,2,2,2,2,2,4),
(-1.29822679571031,-1.27895328969278,-1.25748672292451,-1.24864679765181,
-1.24511425309564,-1.24293884239871,-1.24058220098635,-1.23736524512498,
-1.22984615447287,-1.2194403163622,-1.16517567209637,-1.15788701334334,
-1.14761048742258,-1.14502837285733,-1.14353448051516,-1.1423664724244,
-1.14074924654084,-1.13751266436597,-1.13328644493537,-1.12317473779889,
-1.0786034610789,-1.05258498715359,-1.04802980704026,-1.04512275966436,
-1.04280920358247,-1.04019728265348,-1.03576682629165,-1.0173495029958,
-0.995874651050368,-0.95342497157346,-0.947648200200771,-0.94554254440962,
-0.944305538288356,-0.942981332078365,-0.941118073008606,-0.936522665539095,
-0.913386836116961,-0.888507509418362,-0.853989835326333,-0.849240647417688,
-0.846275000556268,-0.843955225127735,-0.841378163669728,-0.837106446233343,
-0.820747916845267,-0.760566052442591,-0.749677041194939,-0.747043947049844,
-0.74553806763779,-0.74425367182106,-0.742590563867531,-0.739123204089172,
-0.70954213204649,-0.657042481989379,-0.650393441978837,-0.64736294342257,
-0.645027347281515,-0.642507002341059,-0.638494072369844,-0.624950277399896,
-0.577450201276283,-0.551551734857781,-0.548362023650472,-0.546732844587719,
-0.545439098388867,-0.543902956566073,-0.541057689924605,-0.524698486331764,
-0.467528651101692,-0.45382606962641,-0.449641770181674,-0.447083822184037,
-0.444759448228052,-0.441757309449051,-0.435435615512219,-0.41104635857681,
-0.370013757478364,-0.36653701133575,-0.351960870592596,-0.349342541283221,
-0.347700151387892,-0.346405670633289,-0.344880089868795,-0.342083786621802,
-0.326831189945612,-0.280945091773491,-0.256309066476146,-0.251806534446449,
-0.248915399231092,-0.246603147222507,-0.243980528682811,-0.239708530630539,
-0.223567978482093,-0.191787527481715,-0.155877454641331,-0.151109484257704,
-0.149163463807437,-0.147836747515223,-0.146456246517117,-0.144319167732365,
-0.138696197858469,-0.11440300777536,-0.0894439206500073,-0.0577409661094255,
-0.0530218085822374,-0.0500650464892128,-0.0477461167947669,-0.0451637001010432,
-0.0424932371688889,-0.0416143629966081),.UNSPECIFIED.);
#550=B_SPLINE_CURVE_WITH_KNOTS('',3,(#44386,#44387,#44388,#44389,#44390,
#44391,#44392,#44393,#44394,#44395,#44396,#44397,#44398,#44399,#44400,#44401,
#44402,#44403,#44404,#44405,#44406,#44407,#44408,#44409,#44410,#44411,#44412,
#44413,#44414,#44415,#44416,#44417,#44418,#44419,#44420,#44421,#44422,#44423,
#44424,#44425,#44426,#44427,#44428,#44429,#44430,#44431,#44432,#44433,#44434,
#44435,#44436,#44437,#44438,#44439,#44440,#44441,#44442,#44443,#44444,#44445,
#44446,#44447,#44448,#44449,#44450,#44451,#44452,#44453,#44454,#44455,#44456,
#44457,#44458,#44459,#44460,#44461,#44462,#44463,#44464,#44465,#44466,#44467,
#44468,#44469,#44470,#44471,#44472,#44473,#44474,#44475,#44476,#44477,#44478,
#44479,#44480,#44481,#44482,#44483,#44484,#44485,#44486,#44487,#44488,#44489,
#44490,#44491,#44492,#44493,#44494,#44495,#44496,#44497,#44498,#44499,#44500,
#44501,#44502,#44503,#44504,#44505,#44506,#44507,#44508,#44509,#44510,#44511,
#44512,#44513,#44514,#44515,#44516,#44517,#44518,#44519,#44520,#44521,#44522,
#44523,#44524,#44525,#44526,#44527,#44528,#44529,#44530,#44531,#44532,#44533,
#44534,#44535,#44536,#44537,#44538,#44539,#44540,#44541,#44542,#44543,#44544,
#44545,#44546,#44547,#44548,#44549,#44550,#44551,#44552,#44553,#44554,#44555,
#44556,#44557,#44558,#44559,#44560,#44561,#44562,#44563,#44564,#44565,#44566,
#44567,#44568,#44569,#44570,#44571,#44572,#44573,#44574,#44575,#44576,#44577,
#44578,#44579,#44580,#44581,#44582,#44583,#44584,#44585,#44586,#44587,#44588,
#44589,#44590,#44591,#44592,#44593,#44594,#44595,#44596,#44597,#44598,#44599,
#44600,#44601,#44602,#44603,#44604,#44605,#44606,#44607,#44608,#44609,#44610,
#44611,#44612,#44613),.UNSPECIFIED.,.F.,.F.,(4,2,2,2,2,2,2,2,2,2,2,2,2,
2,2,2,2,2,2,2,2,2,2,2,2,2,2,2,2,2,2,2,2,2,2,2,2,2,2,2,2,2,2,2,2,2,2,2,2,
2,2,2,2,2,2,2,2,2,2,2,2,2,2,2,2,2,2,2,2,2,2,2,2,2,2,2,2,2,2,2,2,2,2,2,2,
2,2,2,2,2,2,2,2,2,2,2,2,2,2,2,2,2,2,2,2,2,2,2,2,2,2,2,2,4),(-4.79482997017295,
-4.77764623982758,-4.76922698254938,-4.76374262386725,-4.76174563263966,
-4.76039581283252,-4.7591881320624,-4.75723372644256,-4.75241090604438,
-4.72110610674379,-4.69427235077831,-4.67790801877642,-4.67084377371781,
-4.66534344969845,-4.66251519899233,-4.66029444284504,-4.65770135159296,
-4.65335261600249,-4.63807321811889,-4.59409640502174,-4.56937372866805,
-4.56462882140078,-4.56274222830511,-4.56141425632179,-4.56018405801937,
-4.5584558033292,-4.5538535997449,-4.51440833386472,-4.47142065959173,-4.46617668390806,
-4.46339089781846,-4.46131078331815,-4.45869309379428,-4.45423220543829,
-4.43786809123279,-4.38366584296189,-4.37283694175938,-4.36625098757193,
-4.36411006014671,-4.36272920012707,-4.36140395163977,-4.35946289693512,
-4.35472108591198,-4.318207846487,-4.28691406775286,-4.27622501850695,-4.26854888940172,
-4.26530580909572,-4.262944914523,-4.26077591839745,-4.25783900633327,-4.25056161927958,
-4.20863871521683,-4.19581447241706,-4.1714906864455,-4.16678286524389,
-4.16490205653054,-4.16357507980018,-4.16234333255227,-4.16060952994487,
-4.15596723145889,-4.11714354836527,-4.07376345262449,-4.06841021923842,
-4.06560155388367,-4.06351906919686,-4.06091752448886,-4.05653085092519,
-4.04084227114978,-3.98588408005581,-3.97501007467649,-3.9684043906448,
-3.96626096522958,-3.96487947694789,-3.9635544656636,-3.96161505461155,
-3.95688373404647,-3.9198347620443,-3.88892102005205,-3.87830615709546,
-3.87067079777651,-3.86743438585452,-3.86507451263597,-3.86290378945798,
-3.85996046878927,-3.8526461892945,-3.81327521715505,-3.78308608347465,
-3.77466625112952,-3.76918128045648,-3.76718391610852,-3.76583379955797,
-3.76462581931788,-3.76267086652365,-3.75784638340767,-3.72605209796989,
-3.69169657447381,-3.67417021710501,-3.66980669939626,-3.66721000705005,
-3.66489490984255,-3.66196566879379,-3.65733558871987,-3.6289447070153,
-3.57735130450709,-3.57280642681377,-3.56938034182256,-3.56772567830787,
-3.56643068883029,-3.56491515314762,-3.56223822761924,-3.55074954275652,
-3.5395432496804,-3.53887107067202),.UNSPECIFIED.);
#551=B_SPLINE_CURVE_WITH_KNOTS('',3,(#44615,#44616,#44617,#44618,#44619,
#44620),.UNSPECIFIED.,.F.,.F.,(4,2,4),(-0.0416143629966081,-0.0385168137734201,
-0.000582969486234699),.UNSPECIFIED.);
#552=B_SPLINE_CURVE_WITH_KNOTS('',3,(#44621,#44622,#44623,#44624,#44625,
#44626,#44627,#44628,#44629,#44630,#44631,#44632,#44633,#44634,#44635,#44636,
#44637,#44638,#44639,#44640,#44641,#44642,#44643,#44644,#44645,#44646,#44647,
#44648,#44649,#44650,#44651,#44652,#44653,#44654,#44655,#44656,#44657,#44658,
#44659,#44660,#44661,#44662,#44663,#44664,#44665,#44666,#44667,#44668,#44669,
#44670,#44671,#44672,#44673,#44674,#44675,#44676,#44677,#44678,#44679,#44680,
#44681,#44682,#44683,#44684,#44685,#44686,#44687,#44688,#44689,#44690,#44691,
#44692,#44693,#44694,#44695,#44696,#44697,#44698,#44699,#44700,#44701,#44702,
#44703,#44704,#44705,#44706,#44707,#44708,#44709,#44710,#44711,#44712,#44713,
#44714,#44715,#44716,#44717,#44718,#44719,#44720,#44721,#44722,#44723,#44724,
#44725,#44726,#44727,#44728,#44729,#44730,#44731,#44732,#44733,#44734,#44735,
#44736,#44737,#44738,#44739,#44740,#44741,#44742,#44743,#44744,#44745,#44746,
#44747,#44748,#44749,#44750,#44751,#44752,#44753,#44754,#44755,#44756,#44757,
#44758,#44759,#44760,#44761,#44762,#44763,#44764,#44765,#44766,#44767,#44768,
#44769,#44770,#44771,#44772,#44773,#44774,#44775,#44776,#44777,#44778,#44779,
#44780,#44781,#44782,#44783,#44784,#44785,#44786,#44787,#44788,#44789,#44790,
#44791,#44792,#44793,#44794,#44795,#44796,#44797,#44798,#44799,#44800,#44801),
 .UNSPECIFIED.,.F.,.F.,(4,3,3,3,3,3,3,3,3,3,3,3,3,3,3,3,3,3,3,3,3,3,3,3,
3,3,3,3,3,3,3,3,3,3,3,3,3,3,3,3,3,3,3,3,3,3,3,3,3,3,3,3,3,3,3,3,3,3,3,3,
4),(28.274333882559,28.4078755781023,28.5334621426098,28.6384554085175,
28.7432919913857,28.8480062043826,28.9526551590355,29.0572743614538,29.1618992742995,
29.2666344758122,29.3714312307972,29.4764081877237,29.5285838452726,29.6335770945177,
29.7384136605605,29.8431278565749,29.9477767941578,30.0523959794451,30.1570208751251,
30.2617560595375,30.3665527974347,30.4715297374735,30.5237055479355,30.6286987928139,
30.7335353543564,30.838249545694,30.9428984784934,31.0475176588977,31.1521425496021,
31.256877728932,31.3616744616784,31.4666513965143,31.5188272505983,31.6238205022426,
31.7286570706674,31.8333712690265,31.9380202089294,32.0426393965084,32.147264294448,
32.2519994810554,32.3567962211141,32.461773163239,32.5139489532611,32.6189422022832,
32.7237787680559,32.8284929637316,32.9331419009333,33.0377610857974,33.1423859810126,
33.2471211649,33.3519179022371,33.4568948416669,33.509070655924,33.6145354527492,
33.7193523119969,33.8240640404197,33.9287062339165,34.0347269330688,34.1393751681461,
34.2460820993359,34.3527890305257),.UNSPECIFIED.);
#553=B_SPLINE_CURVE_WITH_KNOTS('',3,(#44807,#44808,#44809,#44810,#44811,
#44812,#44813,#44814,#44815,#44816,#44817,#44818,#44819,#44820,#44821,#44822,
#44823,#44824,#44825,#44826,#44827,#44828,#44829,#44830,#44831,#44832,#44833,
#44834,#44835,#44836,#44837,#44838,#44839,#44840,#44841,#44842,#44843,#44844,
#44845,#44846,#44847,#44848,#44849,#44850,#44851,#44852,#44853,#44854,#44855,
#44856,#44857,#44858,#44859,#44860,#44861,#44862,#44863,#44864,#44865,#44866,
#44867,#44868,#44869,#44870,#44871,#44872,#44873,#44874,#44875,#44876,#44877,
#44878,#44879,#44880,#44881,#44882,#44883,#44884,#44885,#44886,#44887,#44888,
#44889,#44890,#44891,#44892,#44893,#44894,#44895,#44896,#44897,#44898,#44899,
#44900,#44901,#44902,#44903,#44904,#44905,#44906,#44907,#44908,#44909,#44910,
#44911,#44912,#44913,#44914,#44915,#44916,#44917,#44918,#44919,#44920,#44921,
#44922,#44923,#44924,#44925,#44926,#44927,#44928,#44929,#44930,#44931,#44932,
#44933,#44934,#44935,#44936,#44937,#44938,#44939,#44940,#44941,#44942,#44943,
#44944,#44945,#44946,#44947,#44948,#44949,#44950,#44951,#44952,#44953,#44954,
#44955,#44956,#44957,#44958,#44959,#44960,#44961,#44962,#44963,#44964,#44965,
#44966,#44967,#44968,#44969,#44970,#44971,#44972,#44973,#44974,#44975,#44976,
#44977,#44978,#44979,#44980,#44981,#44982,#44983,#44984,#44985,#44986,#44987,
#44988,#44989,#44990,#44991,#44992,#44993,#44994,#44995,#44996,#44997,#44998,
#44999,#45000,#45001,#45002,#45003,#45004,#45005,#45006,#45007,#45008,#45009,
#45010,#45011,#45012,#45013,#45014,#45015,#45016,#45017,#45018,#45019,#45020,
#45021,#45022,#45023,#45024,#45025,#45026,#45027,#45028,#45029,#45030,#45031,
#45032,#45033,#45034,#45035,#45036,#45037,#45038,#45039,#45040,#45041,#45042,
#45043,#45044,#45045,#45046,#45047,#45048,#45049,#45050,#45051,#45052,#45053,
#45054,#45055,#45056,#45057,#45058,#45059,#45060,#45061,#45062),
 .UNSPECIFIED.,.F.,.F.,(4,2,2,2,2,2,2,2,2,2,2,2,2,2,2,2,2,2,2,2,2,2,2,2,
2,2,2,2,2,2,2,2,2,2,2,2,2,2,2,2,2,2,2,2,2,2,2,2,2,2,2,2,2,2,2,2,2,2,2,2,
2,2,2,2,2,2,2,2,2,2,2,2,2,2,2,2,2,2,2,2,2,2,2,2,2,2,2,2,2,2,2,2,2,2,2,2,
2,2,2,2,2,2,2,2,2,2,2,2,2,2,2,2,2,2,2,2,2,2,2,2,2,2,2,2,2,2,2,4),(-1.21647185737743,
-1.21574655815076,-1.21140130549938,-1.19412114657841,-1.16062994279692,
-1.12762346677669,-1.12280095659216,-1.12084607037418,-1.11963790956277,
-1.11828737085617,-1.11628900652554,-1.11079885561553,-1.10236991516711,
-1.07212174717415,-1.0328502328975,-1.02553392661769,-1.02258987310533,
-1.02041863281981,-1.01805821985302,-1.01482112132328,-1.00718443816655,
-0.996566735416115,-0.965644232856276,-0.928543458792508,-0.923811121510414,
-0.92187123342243,-0.920545882514452,-0.919164018685551,-0.91701998760303,
-0.910412110785537,-0.8995355742952,-0.844509223842372,-0.828891860005707,
-0.824511168412601,-0.821910458068376,-0.819827131788921,-0.817015353896145,
-0.81164951182727,-0.767426867210257,-0.761872755202397,-0.747367535836241,
-0.739496965535903,-0.726512349777988,-0.723978604624732,-0.722362145974492,
-0.721069457705053,-0.719523812841109,-0.716632311116422,-0.699084973079515,
-0.670756543271938,-0.631506502268718,-0.626768082625019,-0.623805964803542,
-0.621486979092822,-0.618908767952702,-0.614630387967659,-0.598184357742755,
-0.536935064731781,-0.527071046981134,-0.524524638498465,-0.523038839300196,
-0.521869498478946,-0.520240452832437,-0.516945085351468,-0.512620914457062,
-0.502167929542529,-0.453496104684904,-0.433510236196657,-0.427593378772528,
-0.424669907447243,-0.422354800141479,-0.419753289145133,-0.415370062620266,
-0.397595933830812,-0.360476731321582,-0.345496125494898,-0.328842668633675,
-0.326127853350555,-0.324456598900775,-0.323159978644721,-0.321655589971298,
-0.318956768971214,-0.305610888592713,-0.273764237793886,-0.233455786535155,
-0.228729439617405,-0.225770751020104,-0.223451904777254,-0.223416428661751,
-0.223365488623818,-0.223318920660677,-0.22327634690799,-0.223237421829452,
-0.223201829683931,-0.223169282092572,-0.223139515701249,-0.223112290223071,
-0.223087386375076,-0.223064604014682,-0.223043760455055,-0.223024689007459,
-0.223007237569998,-0.222980072421483,-0.222953431311812,-0.222927301882303,
-0.222901672115073,-0.220168080228804,-0.215097309546578,-0.208729735302207,
-0.194653055997958,-0.135256349340276,-0.128422165925436,-0.126172185808727,
-0.124766764027862,-0.123440046395093,-0.121563596451935,-0.116887027265773,
-0.0929104680205791,-0.0540443370026769,-0.0386634350423491,-0.0307681848463778,
-0.0277285071760984,-0.0255325108033753,-0.0233171458246013,-0.0210389377766114,
-0.0180653078849011,-0.0113560425394448,-0.000720790627167),
 .UNSPECIFIED.);
#554=B_SPLINE_CURVE_WITH_KNOTS('',3,(#45063,#45064,#45065,#45066),
 .UNSPECIFIED.,.F.,.F.,(4,4),(-4.83557347754785,-4.79482997017295),
 .UNSPECIFIED.);
#555=B_SPLINE_CURVE_WITH_KNOTS('',3,(#45068,#45069,#45070,#45071,#45072,
#45073,#45074,#45075,#45076,#45077),.UNSPECIFIED.,.F.,.F.,(4,3,3,4),(34.3527890305257,
34.45776855454,34.5041923585868,34.5575191894877),.UNSPECIFIED.);
#556=B_SPLINE_CURVE_WITH_KNOTS('',3,(#45078,#45079,#45080,#45081,#45082,
#45083,#45084,#45085,#45086,#45087,#45088,#45089,#45090,#45091,#45092,#45093,
#45094,#45095,#45096,#45097,#45098,#45099,#45100,#45101,#45102,#45103,#45104,
#45105,#45106,#45107,#45108,#45109,#45110,#45111,#45112,#45113,#45114,#45115,
#45116,#45117,#45118,#45119,#45120,#45121,#45122,#45123,#45124,#45125,#45126,
#45127,#45128,#45129,#45130,#45131,#45132,#45133,#45134,#45135,#45136,#45137,
#45138,#45139,#45140,#45141,#45142,#45143,#45144,#45145,#45146,#45147,#45148,
#45149,#45150,#45151,#45152,#45153,#45154,#45155,#45156,#45157,#45158,#45159,
#45160,#45161,#45162,#45163,#45164,#45165,#45166,#45167,#45168,#45169,#45170,
#45171,#45172,#45173,#45174,#45175,#45176,#45177,#45178,#45179,#45180,#45181,
#45182,#45183,#45184,#45185,#45186,#45187,#45188,#45189,#45190,#45191,#45192,
#45193,#45194,#45195,#45196,#45197,#45198,#45199,#45200,#45201,#45202,#45203,
#45204,#45205,#45206,#45207,#45208,#45209,#45210,#45211,#45212,#45213,#45214,
#45215,#45216,#45217,#45218,#45219,#45220,#45221,#45222,#45223,#45224,#45225,
#45226,#45227,#45228,#45229,#45230,#45231,#45232,#45233,#45234,#45235,#45236,
#45237,#45238,#45239,#45240,#45241,#45242,#45243,#45244,#45245,#45246,#45247,
#45248,#45249,#45250,#45251,#45252,#45253,#45254,#45255,#45256,#45257,#45258,
#45259,#45260,#45261,#45262,#45263,#45264,#45265,#45266,#45267,#45268,#45269,
#45270,#45271,#45272,#45273,#45274,#45275,#45276,#45277,#45278,#45279,#45280,
#45281,#45282,#45283,#45284,#45285,#45286,#45287,#45288,#45289,#45290,#45291,
#45292,#45293,#45294,#45295,#45296,#45297,#45298,#45299,#45300,#45301,#45302,
#45303),.UNSPECIFIED.,.F.,.F.,(4,2,2,2,2,2,2,2,2,2,2,2,2,2,2,2,2,2,2,2,
2,2,2,2,2,2,2,2,2,2,2,2,2,2,2,2,2,2,2,2,2,2,2,2,2,2,2,2,2,2,2,2,2,2,2,2,
2,2,2,2,2,2,2,2,2,2,2,2,2,2,2,2,2,2,2,2,2,2,2,2,2,2,2,2,2,2,2,2,2,2,2,2,
2,2,2,2,2,2,2,2,2,2,2,2,2,2,2,2,2,2,2,2,4),(-2.51415926376174,-2.45595526132352,
-2.44112870201634,-2.43452733147181,-2.42926422031906,-2.42647356109047,
-2.42418954217027,-2.42149939363548,-2.41683691594838,-2.39707458547378,
-2.35094125696788,-2.33730636174485,-2.33212687745788,-2.32948552374808,
-2.32782396871898,-2.326294915424,-2.32628755800407,-2.32628014471568,-2.32627267422959,
-2.32626514551919,-2.32625755771562,-2.32624990970272,-2.32624220000473,
-2.32623442757019,-2.32622659123447,-2.32621868979411,-2.32496383987108,
-2.32334421218533,-2.32019835187765,-2.28767943860881,-2.26308488322178,
-2.23749095992347,-2.23101021476857,-2.22797818918882,-2.22565002438273,
-2.22310713799184,-2.21899074630113,-2.20589127340483,-2.14801148543067,
-2.13159679594088,-2.12874919284554,-2.12721258566695,-2.12591890451106,
-2.12429039737408,-2.12110376386547,-2.09598235628415,-2.05862531199044,
-2.04337535354933,-2.03335250231701,-2.02975417991429,-2.02732287246096,
-2.02496766086127,-2.02215054080926,-2.01513674188087,-1.9658654929862,
-1.95999471481222,-1.93541361300809,-1.9306801491706,-1.92879455543864,
-1.9274660726498,-1.92623442727144,-1.92450281351788,-1.91988148136306,
-1.88068929779506,-1.83778802082334,-1.83231421054579,-1.82947960385203,
-1.82717135622286,-1.82450778460227,-1.81996305645371,-1.80186986694142,
-1.76119638828816,-1.73639913349757,-1.73164560845845,-1.72975686854339,
-1.7284278215718,-1.72719697685618,-1.7254682890548,-1.72086863832788,-1.68127207798351,
-1.63862324798777,-1.63322505035667,-1.63040604947331,-1.62832139991219,
-1.62572423664867,-1.62136204267509,-1.60595289813047,-1.55651091477708,
-1.53664836875506,-1.53238776034315,-1.53057996895369,-1.52926513719045,
-1.52783349288848,-1.5254657537729,-1.51765735873293,-1.45415996457956,
-1.44318799478322,-1.43535578666817,-1.43208580874529,-1.42971924490477,
-1.42755461856165,-1.42463811815043,-1.41748492338795,-1.37215876014298,
-1.34645902812729,-1.33875441889072,-1.33361926215697,-1.33167212977002,
-1.33033187909921,-1.32911403718709,-1.32743443630268,-1.32316557584655,
-1.29810802178685),.UNSPECIFIED.);
#557=B_SPLINE_CURVE_WITH_KNOTS('',3,(#45308,#45309,#45310,#45311,#45312,
#45313,#45314,#45315,#45316,#45317,#45318,#45319,#45320,#45321,#45322,#45323,
#45324,#45325,#45326,#45327,#45328,#45329,#45330,#45331,#45332,#45333,#45334,
#45335,#45336,#45337,#45338,#45339,#45340,#45341,#45342,#45343,#45344,#45345,
#45346,#45347,#45348,#45349,#45350,#45351,#45352,#45353,#45354,#45355,#45356,
#45357,#45358,#45359,#45360,#45361,#45362,#45363,#45364,#45365,#45366,#45367,
#45368,#45369,#45370,#45371,#45372,#45373,#45374,#45375,#45376,#45377,#45378,
#45379,#45380,#45381,#45382,#45383,#45384,#45385,#45386,#45387,#45388,#45389,
#45390,#45391,#45392,#45393,#45394,#45395,#45396,#45397,#45398,#45399,#45400,
#45401,#45402,#45403,#45404,#45405,#45406,#45407,#45408,#45409,#45410,#45411,
#45412,#45413,#45414,#45415,#45416,#45417,#45418,#45419,#45420,#45421,#45422,
#45423,#45424,#45425,#45426,#45427,#45428,#45429,#45430,#45431,#45432,#45433,
#45434,#45435,#45436,#45437,#45438,#45439,#45440,#45441,#45442,#45443,#45444,
#45445,#45446,#45447,#45448,#45449,#45450,#45451,#45452,#45453,#45454,#45455,
#45456,#45457,#45458,#45459,#45460,#45461,#45462,#45463,#45464,#45465,#45466,
#45467,#45468,#45469,#45470,#45471,#45472,#45473,#45474,#45475,#45476,#45477,
#45478,#45479,#45480,#45481,#45482,#45483,#45484,#45485,#45486,#45487,#45488,
#45489,#45490,#45491,#45492,#45493,#45494,#45495,#45496,#45497,#45498,#45499,
#45500,#45501,#45502,#45503,#45504,#45505,#45506,#45507,#45508,#45509,#45510,
#45511,#45512,#45513,#45514,#45515,#45516,#45517,#45518,#45519),
 .UNSPECIFIED.,.F.,.F.,(4,2,2,2,2,2,2,2,2,2,2,2,2,2,2,2,2,2,2,2,2,2,2,2,
2,2,2,2,2,2,2,2,2,2,2,2,2,2,2,2,2,2,2,2,2,2,2,2,2,2,2,2,2,2,2,2,2,2,2,2,
2,2,2,2,2,2,2,2,2,2,2,2,2,2,2,2,2,2,2,2,2,2,2,2,2,2,2,2,2,2,2,2,2,2,2,2,
2,2,2,2,2,2,2,2,2,4),(-2.47295895309433,-2.44885936015139,-2.42419073849797,
-2.41783273887889,-2.41482448410038,-2.41250015570533,-2.40994705421754,
-2.40578159271537,-2.39223916332579,-2.33091091400115,-2.32240612463165,
-2.31688006810118,-2.31535570403553,-2.31412526478104,-2.31285727071393,
-2.31129528108774,-2.30833276977913,-2.29138578503038,-2.25408028794101,
-2.23337007549272,-2.22092288113042,-2.21702746204059,-2.21453321692116,
-2.21218836561025,-2.20909736242905,-2.20210785950399,-2.1526253717665,
-2.12977042082761,-2.12257655604796,-2.11769920213401,-2.11579142600398,
-2.11445905282926,-2.11323313253996,-2.11152211860302,-2.1070531863777,
-2.06511431395827,-2.02468895833362,-2.01927338729105,-2.0164512905228,
-2.01436682142138,-2.01177305459244,-2.00742417792338,-1.99215762227006,
-1.93671938522095,-1.92049283900378,-1.91765352130429,-1.91611884903683,
-1.91482528343907,-1.91319500426234,-1.9099992639834,-1.8818553179476,-1.86947680546592,
-1.8258164753382,-1.82031104387951,-1.81747029700834,-1.81516209315476,
-1.81250417492365,-1.80798271493916,-1.79014346356711,-1.74932881024771,
-1.72440976591321,-1.71964544664394,-1.71775522863683,-1.71642609751042,
-1.71519594002091,-1.71346925608493,-1.70888312775535,-1.66896429166959,
-1.62681496629872,-1.62131035018889,-1.61846980829889,-1.61616166478901,
-1.61350369818846,-1.60898186989493,-1.59113674761483,-1.54330699008263,
-1.52934334943206,-1.52408093000085,-1.52024034953513,-1.51850703450817,
-1.51720342664469,-1.51573663905622,-1.51320952468757,-1.50387412678734,
-1.44208537499504,-1.42559853136642,-1.42131675556956,-1.41873774531891,
-1.41641883129294,-1.41345789590429,-1.40872353746256,-1.36923943640455,
-1.34043543714986,-1.32350222914285,-1.32063419059999,-1.31909349594471,
-1.31780047657174,-1.3161779760227,-1.31301816763087,-1.28949542319404,
-1.25744063422231,-1.22824698623945,-1.22359274400703,-1.22065587844616,
-1.21833957189857,-1.21647185737743),.UNSPECIFIED.);
#558=B_SPLINE_CURVE_WITH_KNOTS('',3,(#45520,#45521,#45522,#45523,#45524,
#45525,#45526,#45527,#45528,#45529,#45530,#45531,#45532,#45533,#45534,#45535,
#45536,#45537,#45538,#45539,#45540,#45541,#45542,#45543,#45544,#45545,#45546,
#45547,#45548,#45549,#45550,#45551,#45552,#45553,#45554,#45555,#45556,#45557,
#45558,#45559,#45560,#45561,#45562,#45563,#45564,#45565,#45566,#45567,#45568,
#45569,#45570,#45571,#45572,#45573,#45574,#45575,#45576,#45577,#45578,#45579,
#45580,#45581,#45582,#45583,#45584,#45585,#45586,#45587,#45588,#45589,#45590,
#45591,#45592,#45593,#45594,#45595,#45596,#45597,#45598,#45599,#45600,#45601,
#45602,#45603,#45604,#45605,#45606,#45607,#45608,#45609,#45610,#45611,#45612,
#45613,#45614,#45615,#45616,#45617,#45618,#45619,#45620,#45621,#45622,#45623,
#45624,#45625,#45626,#45627,#45628,#45629,#45630,#45631,#45632,#45633,#45634,
#45635,#45636,#45637,#45638,#45639,#45640,#45641,#45642,#45643,#45644,#45645,
#45646,#45647,#45648,#45649,#45650,#45651,#45652,#45653,#45654,#45655,#45656,
#45657,#45658,#45659,#45660,#45661,#45662,#45663,#45664,#45665,#45666,#45667,
#45668,#45669,#45670,#45671,#45672,#45673,#45674,#45675,#45676,#45677,#45678,
#45679,#45680,#45681,#45682,#45683,#45684,#45685,#45686,#45687,#45688,#45689,
#45690,#45691,#45692,#45693,#45694,#45695,#45696,#45697,#45698,#45699,#45700,
#45701,#45702,#45703,#45704,#45705,#45706,#45707,#45708,#45709,#45710,#45711,
#45712,#45713,#45714,#45715,#45716,#45717,#45718,#45719,#45720,#45721,#45722,
#45723,#45724,#45725,#45726,#45727,#45728,#45729,#45730,#45731,#45732,#45733),
 .UNSPECIFIED.,.F.,.F.,(4,2,2,2,2,2,2,2,2,2,2,2,2,2,2,2,2,2,2,2,2,2,2,2,
2,2,2,2,2,2,2,2,2,2,2,2,2,2,2,2,2,2,2,2,2,2,2,2,2,2,2,2,2,2,2,2,2,2,2,2,
2,2,2,2,2,2,2,2,2,2,2,2,2,2,2,2,2,2,2,2,2,2,2,2,2,2,2,2,2,2,2,2,2,2,2,2,
2,2,2,2,2,2,2,2,2,2,4),(-1.29810802178685,-1.27921968545388,-1.25740555526706,
-1.23913038927513,-1.23457302838182,-1.23190672518364,-1.22959893476656,
-1.22676847374173,-1.2213140342513,-1.17962531716193,-1.13908164133103,
-1.13451676629869,-1.13279266191125,-1.13156307978308,-1.13023314682969,
-1.12833945162829,-1.12355409597805,-1.11654090740784,-1.09463840588977,
-1.0436781063232,-1.03684524936847,-1.03378163402275,-1.03144086216804,
-1.02893478620726,-1.02498686655944,-1.01206414164423,-0.990174758022966,
-0.960432153605713,-0.954391929902206,-0.937617396760882,-0.934897699586889,
-0.933224903647788,-0.931928030582676,-0.930424431422591,-0.92772965350664,
-0.914459243445751,-0.882965176492135,-0.845615597736493,-0.838306231331341,
-0.835368303227181,-0.833198359625308,-0.830836242992282,-0.827591150025706,
-0.819908708757381,-0.809208565701869,-0.777869762669467,-0.741335846481875,
-0.736590370490525,-0.734648110946369,-0.733322144659396,-0.731940632363951,
-0.729798874527761,-0.723211649543973,-0.712383419186299,-0.658201778397501,
-0.641810645576294,-0.637345838904488,-0.634726400837247,-0.632645200840464,
-0.629858340402704,-0.624613627725498,-0.581988792211057,-0.542068460938666,
-0.537480744494982,-0.53575373735109,-0.534523436709312,-0.533194238350855,
-0.531304075073505,-0.526540631472104,-0.501635579523521,-0.46088752252969,
-0.443006830540535,-0.438482072609989,-0.435823246267246,-0.433514881573657,
-0.430674738472802,-0.425173053104665,-0.382423295479736,-0.343084514515821,
-0.338470607530021,-0.336740056333561,-0.335508758284075,-0.334180185378971,
-0.332293707319613,-0.327554064687245,-0.302907111397752,-0.259189159116442,
-0.243603092652693,-0.239224539240506,-0.236623827500584,-0.234539791031282,
-0.231782183630919,-0.226613675264722,-0.220084264009965,-0.205490397402259,
-0.171518442852611,-0.141918102513248,-0.138721093394758,-0.137090410452765,
-0.135796653401168,-0.134261898089649,-0.131422819245342,-0.115206972302946,
-0.0787110639488752,-0.0628294140565956,-0.0449915074260607,-0.0415745928430485),
 .UNSPECIFIED.);
#559=B_SPLINE_CURVE_WITH_KNOTS('',3,(#45739,#45740,#45741,#45742,#45743,
#45744,#45745,#45746,#45747,#45748,#45749,#45750,#45751,#45752,#45753,#45754,
#45755,#45756,#45757,#45758,#45759,#45760,#45761,#45762,#45763,#45764,#45765,
#45766,#45767,#45768,#45769,#45770,#45771,#45772,#45773,#45774,#45775,#45776,
#45777,#45778,#45779,#45780,#45781,#45782,#45783,#45784,#45785,#45786,#45787,
#45788,#45789,#45790,#45791,#45792,#45793,#45794,#45795,#45796,#45797,#45798,
#45799,#45800,#45801,#45802,#45803,#45804,#45805,#45806,#45807,#45808,#45809,
#45810,#45811,#45812,#45813,#45814,#45815,#45816,#45817,#45818,#45819,#45820,
#45821,#45822,#45823,#45824,#45825,#45826,#45827,#45828,#45829,#45830,#45831,
#45832,#45833,#45834,#45835,#45836,#45837,#45838,#45839,#45840,#45841,#45842,
#45843,#45844,#45845,#45846,#45847,#45848,#45849,#45850,#45851,#45852,#45853,
#45854,#45855,#45856,#45857,#45858,#45859,#45860,#45861,#45862,#45863,#45864,
#45865,#45866,#45867,#45868,#45869,#45870,#45871,#45872,#45873,#45874,#45875,
#45876,#45877,#45878,#45879,#45880,#45881,#45882,#45883,#45884,#45885,#45886,
#45887,#45888,#45889,#45890,#45891,#45892,#45893,#45894,#45895,#45896,#45897,
#45898,#45899,#45900,#45901,#45902,#45903,#45904,#45905,#45906,#45907,#45908,
#45909,#45910,#45911,#45912,#45913,#45914,#45915,#45916,#45917,#45918,#45919,
#45920,#45921,#45922,#45923,#45924,#45925,#45926,#45927,#45928,#45929,#45930,
#45931,#45932,#45933,#45934,#45935,#45936,#45937,#45938,#45939,#45940,#45941,
#45942,#45943,#45944,#45945,#45946,#45947,#45948,#45949,#45950),
 .UNSPECIFIED.,.F.,.F.,(4,2,2,2,2,2,2,2,2,2,2,2,2,2,2,2,2,2,2,2,2,2,2,2,
2,2,2,2,2,2,2,2,2,2,2,2,2,2,2,2,2,2,2,2,2,2,2,2,2,2,2,2,2,2,2,2,2,2,2,2,
2,2,2,2,2,2,2,2,2,2,2,2,2,2,2,2,2,2,2,2,2,2,2,2,2,2,2,2,2,2,2,2,2,2,2,2,
2,2,2,2,2,2,2,2,2,4),(-1.21635119563388,-1.21207693671559,-1.19844759531399,
-1.19587794698547,-1.19425035099548,-1.19295682588383,-1.19141972505711,
-1.18856944154117,-1.17208333925388,-1.11309186406727,-1.10098107335217,
-1.09698257431772,-1.0944656612982,-1.09212938763119,-1.0890399361622,-1.08224769086417,
-1.05418399880212,-1.01644351206329,-0.999686296433748,-0.996967468468187,
-0.995295017567689,-0.993998289871211,-0.992494718966433,-0.989799651530586,
-0.976520655133499,-0.944984061690785,-0.907692231951055,-0.90038466347107,
-0.897447591220026,-0.895278003603272,-0.892916007321181,-0.889670593564283,
-0.881985074577244,-0.871279020686648,-0.839907549747837,-0.803427769017373,
-0.7986811834416,-0.796738853724702,-0.795412967688485,-0.794031665585379,
-0.791890453571497,-0.785306640849499,-0.774485835176934,-0.720415292109332,
-0.703926583731855,-0.699453709753687,-0.696832666042673,-0.694751896931358,
-0.691967797231712,-0.686735487484548,-0.64551684598223,-0.604077088579714,
-0.599565585103356,-0.597848675202553,-0.596621137953344,-0.595289942912662,
-0.593388713075026,-0.588553985358996,-0.581444358726452,-0.559036431683413,
-0.508893290218511,-0.502661604160232,-0.499274297743984,-0.49690976655445,
-0.494491691723901,-0.49095549117952,-0.481377810867618,-0.46703959914776,
-0.409751164883505,-0.40156629560217,-0.399156747565236,-0.397715926037381,
-0.396404654981518,-0.394618485250298,-0.390482406086816,-0.371756048263399,
-0.324110396351523,-0.306076910972717,-0.301537001155339,-0.298874719136166,
-0.296566659625016,-0.29373110166172,-0.288251708739175,-0.244198789376967,
-0.206226513255702,-0.201550418454958,-0.199651325819143,-0.198332751277305,
-0.19712369071345,-0.195239451184165,-0.190233719447223,-0.182788182716142,
-0.158564860469068,-0.111171174588618,-0.10399933478888,-0.101157208042907,
-0.0987957852667561,-0.0963731207737606,-0.0928157729289583,-0.0830895012703083,
-0.0684493069859314,-0.0395665089118686,-0.00519260416459741,-0.00195456514998335,
-0.000894772399990085,-0.000582812181395608),.UNSPECIFIED.);
#560=B_SPLINE_CURVE_WITH_KNOTS('',3,(#45951,#45952,#45953,#45954,#45955,
#45956,#45957,#45958,#45959,#45960,#45961,#45962,#45963,#45964,#45965,#45966),
 .UNSPECIFIED.,.F.,.F.,(4,2,2,2,2,2,2,4),(-2.51378930048981,-2.51347511735793,
-2.51242511769801,-2.51119511618193,-2.509198543763,-2.50386821565292,-2.49916942911693,
-2.47295895309433),.UNSPECIFIED.);
#561=B_SPLINE_CURVE_WITH_KNOTS('',3,(#45968,#45969,#45970,#45971,#45972,
#45973,#45974,#45975,#45976,#45977,#45978,#45979,#45980,#45981,#45982,#45983),
 .UNSPECIFIED.,.F.,.F.,(4,2,2,2,2,2,2,4),(-0.0415745928430485,-0.0404697249184593,
-0.0378114675414129,-0.0355028788490026,-0.033286401809328,-0.0305091547635283,
-0.0262748328075838,-0.000581010966936684),.UNSPECIFIED.);
#562=B_SPLINE_CURVE_WITH_KNOTS('',3,(#45984,#45985,#45986,#45987,#45988,
#45989,#45990,#45991,#45992,#45993,#45994,#45995,#45996,#45997,#45998,#45999,
#46000,#46001,#46002,#46003,#46004,#46005,#46006,#46007,#46008,#46009,#46010,
#46011,#46012,#46013,#46014,#46015,#46016,#46017,#46018,#46019,#46020,#46021,
#46022,#46023,#46024,#46025,#46026,#46027,#46028,#46029,#46030,#46031,#46032,
#46033,#46034,#46035,#46036,#46037,#46038,#46039,#46040,#46041,#46042,#46043,
#46044,#46045,#46046,#46047,#46048,#46049,#46050,#46051,#46052,#46053,#46054,
#46055,#46056,#46057,#46058,#46059,#46060,#46061,#46062,#46063,#46064,#46065,
#46066,#46067,#46068,#46069,#46070,#46071,#46072,#46073,#46074,#46075,#46076,
#46077,#46078,#46079,#46080,#46081,#46082,#46083,#46084,#46085,#46086,#46087,
#46088,#46089,#46090,#46091,#46092,#46093,#46094,#46095,#46096,#46097,#46098,
#46099,#46100,#46101,#46102,#46103,#46104,#46105,#46106,#46107,#46108,#46109,
#46110,#46111,#46112,#46113,#46114,#46115,#46116,#46117,#46118,#46119,#46120,
#46121,#46122,#46123,#46124,#46125,#46126,#46127,#46128,#46129,#46130,#46131,
#46132,#46133,#46134,#46135,#46136,#46137,#46138,#46139,#46140,#46141,#46142,
#46143,#46144,#46145,#46146,#46147,#46148,#46149,#46150,#46151,#46152,#46153,
#46154,#46155,#46156,#46157,#46158,#46159,#46160,#46161,#46162,#46163,#46164,
#46165,#46166,#46167,#46168,#46169,#46170,#46171,#46172,#46173,#46174,#46175,
#46176,#46177,#46178,#46179,#46180,#46181,#46182,#46183,#46184,#46185,#46186,
#46187),.UNSPECIFIED.,.F.,.F.,(4,2,2,2,2,2,2,2,2,2,2,2,2,2,2,2,2,2,2,2,
2,2,2,2,2,2,2,2,2,2,2,2,2,2,2,2,2,2,2,2,2,2,2,2,2,2,2,2,2,2,2,2,2,2,2,2,
2,2,2,2,2,2,2,2,2,2,2,2,2,2,2,2,2,2,2,2,2,2,2,2,2,2,2,2,2,2,2,2,2,2,2,2,
2,2,2,2,2,2,2,2,2,4),(-2.51486360124677,-2.48403448716676,-2.45940953353798,
-2.45467126794229,-2.45278458334456,-2.4514556130955,-2.45022374120684,
-2.4484921160338,-2.44387308597346,-2.40461054723988,-2.38051108660902,
-2.36710296080089,-2.35803643117646,-2.35469104542183,-2.35252903686565,
-2.35018327990953,-2.34709395636076,-2.3401208102182,-2.28982035667201,
-2.26751988023639,-2.26042907836603,-2.2556037056259,-2.25370326378715,
-2.25237165648517,-2.25114296638613,-2.24942341637417,-2.24489669596251,
-2.2036451249633,-2.16257882785529,-2.15714412037568,-2.15431696599936,
-2.15223078681754,-2.14963748721678,-2.14529560393497,-2.13011299363908,
-2.07453448222296,-2.05828890689929,-2.0554473756231,-2.05391162340847,
-2.05261721713411,-2.05098596671736,-2.04778858253313,-2.01879006596697,
-1.98665963626305,-1.97056016401614,-1.96357182846481,-1.95806431332904,
-1.95522196527578,-1.95291220141417,-1.95025219941751,-1.94572649715321,
-1.92785973427864,-1.88702599408337,-1.86209738422806,-1.85733049396155,
-1.85543908995706,-1.85410906846883,-1.85287804180157,-1.85115007668674,
-1.84656006016643,-1.80663506731546,-1.76432930337709,-1.75888592787529,
-1.75605678149165,-1.75374785620934,-1.75107777205386,-1.74650788670798,
-1.72808338397844,-1.68070786973389,-1.66684723767386,-1.66160951953553,
-1.65778232774098,-1.6560507619294,-1.65474664477987,-1.65327726100032,
-1.65074119392919,-1.64132371175794,-1.57957476062324,-1.56308307315322,
-1.55879889922861,-1.5562182430151,-1.55389772104179,-1.55093455602256,
-1.5461962745907,-1.50671247433801,-1.47794789754119,-1.46092342575762,
-1.45805028099995,-1.45650786442857,-1.45521400168965,-1.45359120108154,
-1.45043300679088,-1.42726983135739,-1.38359092894409,-1.36437053185251,
-1.35988241854872,-1.35725698896054,-1.35494388063394,-1.3520538140911,
-1.34755704445447,-1.32311316954842,-1.29859447736914),.UNSPECIFIED.);
#563=B_SPLINE_CURVE_WITH_KNOTS('',3,(#46192,#46193,#46194,#46195,#46196,
#46197,#46198,#46199,#46200,#46201,#46202,#46203,#46204,#46205,#46206,#46207,
#46208,#46209,#46210,#46211,#46212,#46213,#46214,#46215,#46216,#46217,#46218,
#46219,#46220,#46221,#46222,#46223,#46224,#46225,#46226,#46227,#46228,#46229,
#46230,#46231,#46232,#46233,#46234,#46235,#46236,#46237,#46238,#46239,#46240,
#46241,#46242,#46243,#46244,#46245,#46246,#46247,#46248,#46249,#46250,#46251,
#46252,#46253,#46254,#46255,#46256,#46257,#46258,#46259,#46260,#46261,#46262,
#46263,#46264,#46265,#46266,#46267,#46268,#46269,#46270,#46271,#46272,#46273,
#46274,#46275,#46276,#46277,#46278,#46279,#46280,#46281,#46282,#46283,#46284,
#46285,#46286,#46287,#46288,#46289,#46290,#46291,#46292,#46293,#46294,#46295,
#46296,#46297,#46298,#46299,#46300,#46301,#46302,#46303,#46304,#46305,#46306,
#46307,#46308,#46309,#46310,#46311,#46312,#46313,#46314,#46315,#46316,#46317,
#46318,#46319,#46320,#46321,#46322,#46323,#46324,#46325,#46326,#46327,#46328,
#46329,#46330,#46331,#46332,#46333,#46334,#46335,#46336,#46337,#46338,#46339,
#46340,#46341,#46342,#46343,#46344,#46345,#46346,#46347,#46348,#46349,#46350,
#46351,#46352,#46353,#46354,#46355,#46356,#46357,#46358,#46359,#46360,#46361,
#46362,#46363,#46364,#46365,#46366,#46367,#46368,#46369,#46370,#46371,#46372,
#46373,#46374,#46375,#46376,#46377,#46378,#46379,#46380,#46381,#46382,#46383,
#46384,#46385,#46386,#46387,#46388,#46389,#46390,#46391,#46392,#46393,#46394,
#46395,#46396,#46397,#46398,#46399,#46400,#46401),.UNSPECIFIED.,.F.,.F.,
(4,2,2,2,2,2,2,2,2,2,2,2,2,2,2,2,2,2,2,2,2,2,2,2,2,2,2,2,2,2,2,2,2,2,2,
2,2,2,2,2,2,2,2,2,2,2,2,2,2,2,2,2,2,2,2,2,2,2,2,2,2,2,2,2,2,2,2,2,2,2,2,
2,2,2,2,2,2,2,2,2,2,2,2,2,2,2,2,2,2,2,2,2,2,2,2,2,2,2,2,2,2,2,2,2,4),(-2.47309949534992,
-2.47127547339437,-2.45596006103672,-2.40491628643083,-2.39650863763585,
-2.39102905683977,-2.38903204129656,-2.387681681759,-2.38647312092219,-2.38451655599,
-2.37968473310878,-2.34873412281988,-2.32256922059027,-2.30553640783741,
-2.29827512753788,-2.29264198515644,-2.28979067358952,-2.28752610877192,
-2.28493184131325,-2.28058202631575,-2.26531082848368,-2.20986465472809,
-2.19363535655162,-2.19079553552778,-2.18926058893448,-2.18796679075073,
-2.18633621672529,-2.18313989340236,-2.15500002971538,-2.14261097198826,
-2.09858912234754,-2.09329500086617,-2.09049757612045,-2.08841510342249,
-2.08580273203755,-2.0813713009813,-2.06523230300893,-2.01636580159925,
-1.99675119591292,-1.99251736917353,-1.99071416212996,-1.98940007293583,
-1.98796647751316,-1.98558996315499,-1.97770421885991,-1.91429458288821,
-1.9033265672142,-1.89549651655011,-1.89222689205334,-1.88986038948655,
-1.88769568549551,-1.88477887864323,-1.87762391498049,-1.83233270826694,
-1.79710198034846,-1.79323600267408,-1.7914979399305,-1.79019359028901,
-1.78872909218208,-1.78621279111138,-1.77699129438329,-1.71507102457687,
-1.69857269557366,-1.69428966290926,-1.69171020055042,-1.68939107364854,
-1.68643013346672,-1.68169630883242,-1.64216279367231,-1.61325631853494,
-1.59645466063384,-1.59359163290892,-1.59205190488581,-1.59075867741116,
-1.58913462970404,-1.58596806924658,-1.56197965001694,-1.52371842417782,
-1.50831703627055,-1.50153991034737,-1.49616569710578,-1.49335192528585,
-1.49126810996243,-1.48866807496836,-1.48429162041681,-1.46872416729493,
-1.41360197174489,-1.3973997909313,-1.39456123801109,-1.39302661330261,
-1.39173286921736,-1.39010208809483,-1.38690454782772,-1.35708558526728,
-1.31884710612772,-1.30080077525413,-1.29639700584974,-1.29379077646065,
-1.29147608003524,-1.28855932084928,-1.28397261106968,-1.25702096238711,
-1.2318851758174,-1.21887035561419,-1.21635119563388),.UNSPECIFIED.);
#564=B_SPLINE_CURVE_WITH_KNOTS('',3,(#46402,#46403,#46404,#46405,#46406,
#46407,#46408,#46409,#46410,#46411,#46412,#46413,#46414,#46415,#46416,#46417,
#46418,#46419,#46420,#46421,#46422,#46423,#46424,#46425,#46426,#46427,#46428,
#46429,#46430,#46431,#46432,#46433,#46434,#46435,#46436,#46437,#46438,#46439,
#46440,#46441,#46442,#46443,#46444,#46445,#46446,#46447,#46448,#46449,#46450,
#46451,#46452,#46453,#46454,#46455,#46456,#46457,#46458,#46459,#46460,#46461,
#46462,#46463,#46464,#46465,#46466,#46467,#46468,#46469,#46470,#46471,#46472,
#46473,#46474,#46475,#46476,#46477,#46478,#46479,#46480,#46481,#46482,#46483,
#46484,#46485,#46486,#46487,#46488,#46489,#46490,#46491,#46492,#46493,#46494,
#46495,#46496,#46497,#46498,#46499,#46500,#46501,#46502,#46503,#46504,#46505,
#46506,#46507,#46508,#46509,#46510,#46511,#46512,#46513,#46514,#46515,#46516,
#46517,#46518,#46519,#46520,#46521,#46522,#46523,#46524,#46525,#46526,#46527,
#46528,#46529,#46530,#46531,#46532,#46533,#46534,#46535,#46536,#46537,#46538,
#46539,#46540,#46541,#46542,#46543,#46544,#46545,#46546,#46547,#46548,#46549,
#46550,#46551,#46552,#46553,#46554,#46555,#46556,#46557,#46558,#46559,#46560,
#46561,#46562,#46563,#46564,#46565,#46566,#46567,#46568,#46569,#46570,#46571,
#46572,#46573,#46574,#46575,#46576,#46577,#46578,#46579,#46580,#46581,#46582,
#46583,#46584,#46585,#46586,#46587,#46588,#46589,#46590,#46591,#46592,#46593,
#46594,#46595,#46596,#46597,#46598,#46599,#46600,#46601,#46602,#46603,#46604,
#46605,#46606,#46607,#46608,#46609,#46610,#46611,#46612,#46613,#46614,#46615,
#46616,#46617,#46618,#46619,#46620,#46621,#46622,#46623,#46624,#46625,#46626,
#46627,#46628,#46629,#46630,#46631),.UNSPECIFIED.,.F.,.F.,(4,2,2,2,2,2,
2,2,2,2,2,2,2,2,2,2,2,2,2,2,2,2,2,2,2,2,2,2,2,2,2,2,2,2,2,2,2,2,2,2,2,2,
2,2,2,2,2,2,2,2,2,2,2,2,2,2,2,2,2,2,2,2,2,2,2,2,2,2,2,2,2,2,2,2,2,2,2,2,
2,2,2,2,2,2,2,2,2,2,2,2,2,2,2,2,2,2,2,2,2,2,2,2,2,2,2,2,2,2,2,2,2,2,2,2,
4),(-1.29859447736914,-1.28129283734518,-1.26820788588034,-1.2631684333074,
-1.25945426865517,-1.25774374785694,-1.25644235569197,-1.25496132484305,
-1.25237185122733,-1.24082785893824,-1.21516384004797,-1.16979233478358,
-1.162639221935,-1.15972194754688,-1.15755644932196,-1.15518864174769,-1.15191642406315,
-1.1440763531082,-1.13309031562372,-1.06942196452236,-1.06170599567376,
-1.0593480342408,-1.05791807363478,-1.05660155986945,-1.05478690255315,
-1.05048942982765,-1.03029546681689,-0.978697638071059,-0.965382691780355,
-0.961240019357399,-0.958690243456607,-0.95636193703801,-0.953338548582027,
-0.946910346128419,-0.921731856699086,-0.888847539858425,-0.864065687375207,
-0.860886464234897,-0.859259032453427,-0.857964765139316,-0.856425750023858,
-0.853569203110952,-0.836963675480725,-0.776223441941107,-0.765537558119888,
-0.761724595605466,-0.759494709965725,-0.757165137336825,-0.754130468325904,
-0.747640946311518,-0.721989899614708,-0.68730331149973,-0.681821045869953,
-0.677837000456514,-0.664290686584514,-0.661724609722285,-0.660097688471191,
-0.658803613579935,-0.657264574536392,-0.654407318071632,-0.637777125920965,
-0.576594586152884,-0.566277214713519,-0.562516695795688,-0.5602971750145,
-0.557963746862912,-0.554899642784734,-0.548250413348906,-0.52134826547736,
-0.490388923078804,-0.465763674943844,-0.462587198713617,-0.460960615809743,
-0.459666727180571,-0.458127811600798,-0.455270526206553,-0.438632178116423,
-0.377279559925415,-0.3671078915294,-0.36336875654538,-0.361153567188859,
-0.358818646675264,-0.355742441571501,-0.349026011748525,-0.321584123080141,
-0.295621854099429,-0.266687527647133,-0.263490946993484,-0.261860210784585,
-0.260566267907173,-0.259031122765637,-0.256190880536305,-0.239955303435136,
-0.184399156138189,-0.169244673385418,-0.16490679653023,-0.162314912300009,
-0.160229323722529,-0.160187496920376,-0.160147215561924,-0.160108385173283,
-0.160070918697468,-0.157225475235737,-0.15169789706795,-0.144559425541735,
-0.127947301775496,-0.106655130377444,-0.0699756605761903,-0.0652331800173265,
-0.0632912907347226,-0.0619652915547201,-0.0605834626182379,-0.0584407227816428,
-0.051846602696853,-0.0412924016477382),.UNSPECIFIED.);
#565=B_SPLINE_CURVE_WITH_KNOTS('',3,(#46637,#46638,#46639,#46640,#46641,
#46642,#46643,#46644,#46645,#46646,#46647,#46648,#46649,#46650,#46651,#46652,
#46653,#46654,#46655,#46656,#46657,#46658,#46659,#46660,#46661,#46662,#46663,
#46664,#46665,#46666,#46667,#46668,#46669,#46670,#46671,#46672,#46673,#46674,
#46675,#46676,#46677,#46678,#46679,#46680,#46681,#46682,#46683,#46684,#46685,
#46686,#46687,#46688,#46689,#46690,#46691,#46692,#46693,#46694,#46695,#46696,
#46697,#46698,#46699,#46700,#46701,#46702,#46703,#46704,#46705,#46706,#46707,
#46708,#46709,#46710,#46711,#46712,#46713,#46714,#46715,#46716,#46717,#46718,
#46719,#46720,#46721,#46722,#46723,#46724,#46725,#46726,#46727,#46728,#46729,
#46730,#46731,#46732,#46733,#46734,#46735,#46736,#46737,#46738,#46739,#46740,
#46741,#46742,#46743,#46744,#46745,#46746,#46747,#46748,#46749,#46750,#46751,
#46752,#46753,#46754,#46755,#46756,#46757,#46758,#46759,#46760,#46761,#46762,
#46763,#46764,#46765,#46766,#46767,#46768,#46769,#46770,#46771,#46772,#46773,
#46774,#46775,#46776,#46777,#46778,#46779,#46780,#46781,#46782,#46783,#46784,
#46785,#46786,#46787,#46788,#46789,#46790,#46791,#46792,#46793,#46794,#46795,
#46796,#46797,#46798,#46799,#46800,#46801,#46802,#46803,#46804,#46805,#46806,
#46807,#46808,#46809,#46810,#46811,#46812,#46813,#46814,#46815,#46816,#46817,
#46818,#46819,#46820,#46821,#46822,#46823,#46824,#46825,#46826,#46827,#46828,
#46829,#46830,#46831,#46832,#46833,#46834,#46835,#46836,#46837,#46838,#46839,
#46840,#46841,#46842,#46843,#46844,#46845,#46846,#46847,#46848,#46849,#46850),
 .UNSPECIFIED.,.F.,.F.,(4,2,2,2,2,2,2,2,2,2,2,2,2,2,2,2,2,2,2,2,2,2,2,2,
2,2,2,2,2,2,2,2,2,2,2,2,2,2,2,2,2,2,2,2,2,2,2,2,2,2,2,2,2,2,2,2,2,2,2,2,
2,2,2,2,2,2,2,2,2,2,2,2,2,2,2,2,2,2,2,2,2,2,2,2,2,2,2,2,2,2,2,2,2,2,2,2,
2,2,2,2,2,2,2,2,2,2,4),(-1.21647209020946,-1.20589754521165,-1.17728609578228,
-1.17264689952674,-1.1697137667687,-1.16739678821615,-1.16479923697488,
-1.16043729128841,-1.14296139717832,-1.10880317286871,-1.09664657958352,
-1.09359574351831,-1.08782688556157,-1.07362109533104,-1.07102075317838,
-1.06938357257115,-1.06808910253175,-1.06655872237724,-1.06374126600813,
-1.04803646139591,-0.998223915396606,-0.977575769909869,-0.972853143571639,
-0.970148711929969,-0.967864416501892,-0.965087923199884,-0.959895474988632,
-0.921988001161925,-0.881110384082842,-0.873542277167189,-0.871202010586539,
-0.869776299564524,-0.868458714016256,-0.866635502902323,-0.862285213711711,
-0.841584302635778,-0.781913120280027,-0.774961987239186,-0.771876960211157,
-0.769532311194114,-0.767034120193988,-0.763123862939929,-0.750552668497476,
-0.729540240789816,-0.692915539454742,-0.689092808822501,-0.675376451790558,
-0.672801756170647,-0.671172440856944,-0.669878557342289,-0.668342221213909,
-0.665496475777756,-0.649130957240392,-0.591892213373294,-0.578244083325774,
-0.574065535528693,-0.571508697372987,-0.569183762550786,-0.566178680668933,
-0.559842405967283,-0.53534628654806,-0.493815537298598,-0.489903610915842,
-0.476285836237096,-0.473716544678314,-0.472088936057674,-0.47079523786801,
-0.469257738613073,-0.466406210156904,-0.449897471486241,-0.390592061796495,
-0.378739380276266,-0.374772798373961,-0.372262637225479,-0.369923422814105,
-0.366816339259474,-0.359928228156171,-0.331080622654647,-0.296216517854237,
-0.292222645233031,-0.277342208287288,-0.274709165460133,-0.273062352041594,
-0.271767585211212,-0.270245401868124,-0.267464838261181,-0.252545203241682,
-0.209212567071252,-0.181880435471606,-0.177266988788374,-0.174342167002432,
-0.172026731425725,-0.169527458724321,-0.165387238678503,-0.160407971473687,
-0.150490071467178,-0.122941966355962,-0.0808072168409335,-0.076350980466186,
-0.074641486042469,-0.0734157974432842,-0.0720826928009046,-0.0701722454890665,
-0.0652792612178099,-0.0580560680089516,-0.0350476812884346,-0.000583285542807006),
 .UNSPECIFIED.);
#566=B_SPLINE_CURVE_WITH_KNOTS('',3,(#46851,#46852,#46853,#46854,#46855,
#46856,#46857,#46858,#46859,#46860,#46861,#46862,#46863,#46864,#46865,#46866,
#46867,#46868),.UNSPECIFIED.,.F.,.F.,(4,2,2,2,2,2,2,2,4),(-2.51402391418862,
-2.50161511808339,-2.49426729550675,-2.49130566087207,-2.48903181552238,
-2.48681378261952,-2.48461343489582,-2.48094913905227,-2.47309949534992),
 .UNSPECIFIED.);
#567=B_SPLINE_CURVE_WITH_KNOTS('',3,(#46870,#46871,#46872,#46873),
 .UNSPECIFIED.,.F.,.F.,(4,4),(-0.0412924016477382,-0.00058319047411503),
 .UNSPECIFIED.);
#568=B_SPLINE_CURVE_WITH_KNOTS('',3,(#46874,#46875,#46876,#46877,#46878,
#46879,#46880,#46881,#46882,#46883,#46884,#46885,#46886,#46887,#46888,#46889,
#46890,#46891,#46892,#46893,#46894,#46895,#46896,#46897,#46898,#46899,#46900,
#46901,#46902,#46903,#46904,#46905,#46906,#46907,#46908,#46909,#46910,#46911,
#46912,#46913,#46914,#46915,#46916,#46917,#46918,#46919,#46920,#46921,#46922,
#46923,#46924,#46925,#46926,#46927,#46928,#46929,#46930,#46931,#46932,#46933,
#46934,#46935,#46936,#46937,#46938,#46939,#46940,#46941,#46942,#46943,#46944,
#46945,#46946,#46947,#46948,#46949,#46950,#46951,#46952,#46953,#46954,#46955,
#46956,#46957,#46958,#46959,#46960,#46961,#46962,#46963,#46964,#46965,#46966,
#46967,#46968,#46969,#46970,#46971,#46972,#46973,#46974,#46975,#46976,#46977,
#46978,#46979,#46980,#46981,#46982,#46983,#46984,#46985,#46986,#46987,#46988,
#46989,#46990,#46991,#46992,#46993,#46994,#46995,#46996,#46997,#46998,#46999,
#47000,#47001,#47002,#47003,#47004,#47005,#47006,#47007,#47008,#47009,#47010,
#47011,#47012,#47013,#47014,#47015,#47016,#47017,#47018,#47019,#47020,#47021,
#47022,#47023,#47024,#47025,#47026,#47027,#47028,#47029,#47030,#47031,#47032,
#47033,#47034,#47035,#47036,#47037,#47038,#47039,#47040,#47041,#47042,#47043,
#47044,#47045,#47046,#47047,#47048,#47049,#47050,#47051,#47052,#47053,#47054,
#47055,#47056,#47057,#47058,#47059,#47060,#47061,#47062,#47063,#47064,#47065,
#47066,#47067,#47068,#47069,#47070,#47071,#47072,#47073,#47074,#47075,#47076,
#47077,#47078,#47079,#47080,#47081,#47082,#47083,#47084,#47085,#47086,#47087,
#47088,#47089,#47090,#47091,#47092,#47093,#47094,#47095,#47096,#47097,#47098,
#47099,#47100,#47101,#47102,#47103,#47104,#47105,#47106,#47107,#47108,#47109,
#47110,#47111,#47112,#47113),.UNSPECIFIED.,.F.,.F.,(4,2,2,2,2,2,2,2,2,2,
2,2,2,2,2,2,2,2,2,2,2,2,2,2,2,2,2,2,2,2,2,2,2,2,2,2,2,2,2,2,2,2,2,2,2,2,
2,2,2,2,2,2,2,2,2,2,2,2,2,2,2,2,2,2,2,2,2,2,2,2,2,2,2,2,2,2,2,2,2,2,2,2,
2,2,2,2,2,2,2,2,2,2,2,2,2,2,2,2,2,2,2,2,2,2,2,2,2,2,2,2,2,2,2,2,2,2,2,2,
2,4),(-2.51466580210535,-2.48688043602376,-2.48277505446942,-2.48005091685726,
-2.47784835815228,-2.47556362045631,-2.47286451274943,-2.46816601787414,
-2.44788520736209,-2.43123540376619,-2.39822109209008,-2.38199005697294,
-2.37914957060266,-2.3776142267035,-2.37632007114578,-2.37468901830606,
-2.37149167276508,-2.34203292298677,-2.30698665792291,-2.29296590346264,
-2.28661466642606,-2.28156095138116,-2.27882637395884,-2.27880121072071,
-2.27877556151567,-2.27874941389501,-2.27872275507702,-2.27869557186183,
-2.27867790142337,-2.27865859030209,-2.27863748217226,-2.27861440508373,
-2.27858916990709,-2.27856156847561,-2.27853137153467,-2.27849832659295,
-2.2784621552807,-2.27842255072964,-2.27837917458935,-2.27833165364839,
-2.2782795759228,-2.2782362568903,-2.27816849121875,-2.27806256515577,-2.27572531069299,
-2.2726878408054,-2.26600358860942,-2.21372177780222,-2.18363399095287,
-2.18034140120792,-2.1787124315905,-2.17754261698338,-2.17605547546703,
-2.17350518619371,-2.1636065206156,-2.10238719054798,-2.08593977255182,
-2.08165972058762,-2.07908023978216,-2.07675994361423,-2.07379591987535,
-2.06905393715311,-2.02967739097466,-2.00112346715458,-1.98382227877162,
-1.98093875177067,-1.97939428168329,-1.97810076280821,-1.97648099236103,
-1.97333620040045,-1.95168560699098,-1.89917127732409,-1.88620410615282,
-1.88225086801538,-1.87974324891727,-1.87740230765782,-1.87434030136554,
-1.86751886251849,-1.81639903645351,-1.78569005745561,-1.78219212378759,
-1.78052287570537,-1.77923766987557,-1.7777354265077,-1.77511904348417,
-1.76444159799782,-1.70405503714433,-1.68767854334814,-1.68340466630013,
-1.68082672169296,-1.67850641648367,-1.67554045928842,-1.67079147746974,
-1.6366133362829,-1.59931894013552,-1.58532429091377,-1.58258963623933,
-1.58107717856096,-1.57978108284506,-1.57812019096764,-1.57544095440127,
-1.5596530589867,-1.52414295979256,-1.49330714115335,-1.48618344248167,
-1.48303394117644,-1.48068764341093,-1.47819318793872,-1.47430020272724,
-1.46302056253795,-1.41965460667862,-1.38992742748971,-1.38474642238979,
-1.38279217985026,-1.38145025889512,-1.38023340354888,-1.37855843139856,
-1.37431868058543,-1.33008093193916,-1.29825834795597),.UNSPECIFIED.);
#569=B_SPLINE_CURVE_WITH_KNOTS('',3,(#47118,#47119,#47120,#47121,#47122,
#47123,#47124,#47125,#47126,#47127,#47128,#47129,#47130,#47131,#47132,#47133,
#47134,#47135,#47136,#47137,#47138,#47139,#47140,#47141,#47142,#47143,#47144,
#47145,#47146,#47147,#47148,#47149,#47150,#47151,#47152,#47153,#47154,#47155,
#47156,#47157,#47158,#47159,#47160,#47161,#47162,#47163,#47164,#47165,#47166,
#47167,#47168,#47169,#47170,#47171,#47172,#47173,#47174,#47175,#47176,#47177,
#47178,#47179,#47180,#47181,#47182,#47183,#47184,#47185,#47186,#47187,#47188,
#47189,#47190,#47191,#47192,#47193,#47194,#47195,#47196,#47197,#47198,#47199,
#47200,#47201,#47202,#47203,#47204,#47205,#47206,#47207,#47208,#47209,#47210,
#47211,#47212,#47213,#47214,#47215,#47216,#47217,#47218,#47219,#47220,#47221,
#47222,#47223,#47224,#47225,#47226,#47227,#47228,#47229,#47230,#47231,#47232,
#47233,#47234,#47235,#47236,#47237,#47238,#47239,#47240,#47241,#47242,#47243,
#47244,#47245,#47246,#47247,#47248,#47249,#47250,#47251,#47252,#47253,#47254,
#47255,#47256,#47257,#47258,#47259,#47260,#47261,#47262,#47263,#47264,#47265,
#47266,#47267,#47268,#47269,#47270,#47271,#47272,#47273,#47274,#47275,#47276,
#47277,#47278,#47279,#47280,#47281,#47282,#47283,#47284,#47285,#47286,#47287,
#47288,#47289,#47290,#47291,#47292,#47293,#47294,#47295,#47296,#47297,#47298,
#47299,#47300,#47301,#47302,#47303,#47304,#47305,#47306,#47307,#47308,#47309,
#47310,#47311,#47312,#47313,#47314,#47315,#47316,#47317,#47318,#47319,#47320,
#47321,#47322,#47323,#47324,#47325,#47326,#47327,#47328,#47329,#47330,#47331,
#47332,#47333,#47334,#47335,#47336,#47337,#47338,#47339,#47340,#47341),
 .UNSPECIFIED.,.F.,.F.,(4,2,2,2,2,2,2,2,2,2,2,2,2,2,2,2,2,2,2,2,2,2,2,2,
2,2,2,2,2,2,2,2,2,2,2,2,2,2,2,2,2,2,2,2,2,2,2,2,2,2,2,2,2,2,2,2,2,2,2,2,
2,2,2,2,2,2,2,2,2,2,2,2,2,2,2,2,2,2,2,2,2,2,2,2,2,2,2,2,2,2,2,2,2,2,2,2,
2,2,2,2,2,2,2,2,2,2,2,2,2,2,2,4),(-2.4734065574123,-2.47297094298435,-2.46819529786363,
-2.46570077595541,-2.46356993923343,-2.46219069903809,-2.46086279749131,
-2.45891133447964,-2.45411149328566,-2.41957982033227,-2.39731631674372,
-2.37192125438772,-2.36680120692414,-2.36450853056401,-2.36216850816659,
-2.35965931269944,-2.35569815671919,-2.34389108645553,-2.30261089368116,
-2.27161104047677,-2.2663939033618,-2.26439611016055,-2.26304535843778,
-2.26183654803884,-2.2598797668444,-2.2550483480496,-2.2224529611183,-2.1886717061223,
-2.17720764647332,-2.16910831427439,-2.16579433853441,-2.16341932628676,
-2.16126284188574,-2.15783926750935,-2.15147425401397,-2.10279534521424,
-2.07054523797849,-2.06670121460668,-2.06496693257838,-2.06366284590181,
-2.062195794547,-2.05966883269793,-2.05034059131633,-1.98852054316546,-1.97202744021389,
-1.96774419256317,-1.96516432295667,-1.96284465350098,-1.95988277733525,
-1.95514696292316,-1.91564611785823,-1.88704685311041,-1.86991096625504,
-1.86703424787001,-1.86549140296358,-1.86419805741198,-1.86257700882889,
-1.86002925029812,-1.84679845275327,-1.83938011510562,-1.82656853589027,
-1.80145622565971,-1.77658074803303,-1.77019356539879,-1.76717876093513,
-1.76485248085871,-1.76230034545287,-1.75814350271749,-1.74469187152918,
-1.68719789561958,-1.6708084491133,-1.6679614382322,-1.66642475992443,-1.66513078620306,
-1.66350161623062,-1.66031282125465,-1.63454604213219,-1.60799301556141,
-1.58618626350811,-1.57329380082639,-1.56934835693358,-1.56684230940579,
-1.56450048853119,-1.56143394646554,-1.55458797190715,-1.50367731083793,
-1.48170022316211,-1.47467177393256,-1.46987857180819,-1.46798328022903,
-1.46665274259573,-1.46542301038193,-1.4636992611816,-1.45913961508351,
-1.41890134726393,-1.41680857109891,-1.37718360549119,-1.37156448972294,
-1.3686998114636,-1.3663889940198,-1.36374653607847,-1.35929561310345,-1.3423972858068,
-1.29381662297137,-1.27470587676728,-1.27052657001854,-1.2687324676093,
-1.26741955150624,-1.26616162001951,-1.26395179797613,-1.25742858636991,
-1.21647209020946),.UNSPECIFIED.);
#570=B_SPLINE_CURVE_WITH_KNOTS('',3,(#47342,#47343,#47344,#47345,#47346,
#47347,#47348,#47349,#47350,#47351,#47352,#47353,#47354,#47355,#47356,#47357,
#47358,#47359,#47360,#47361,#47362,#47363,#47364,#47365,#47366,#47367,#47368,
#47369,#47370,#47371,#47372,#47373,#47374,#47375,#47376,#47377,#47378,#47379,
#47380,#47381,#47382,#47383,#47384,#47385,#47386,#47387,#47388,#47389,#47390,
#47391,#47392,#47393,#47394,#47395,#47396,#47397,#47398,#47399,#47400,#47401,
#47402,#47403,#47404,#47405,#47406,#47407,#47408,#47409,#47410,#47411,#47412,
#47413,#47414,#47415,#47416,#47417,#47418,#47419,#47420,#47421,#47422,#47423,
#47424,#47425,#47426,#47427,#47428,#47429,#47430,#47431,#47432,#47433,#47434,
#47435,#47436,#47437,#47438,#47439,#47440,#47441,#47442,#47443,#47444,#47445,
#47446,#47447,#47448,#47449,#47450,#47451,#47452,#47453,#47454,#47455,#47456,
#47457,#47458,#47459,#47460,#47461,#47462,#47463,#47464,#47465,#47466,#47467,
#47468,#47469,#47470,#47471,#47472,#47473,#47474,#47475,#47476,#47477,#47478,
#47479,#47480,#47481,#47482,#47483,#47484,#47485,#47486,#47487,#47488,#47489,
#47490,#47491,#47492,#47493,#47494,#47495,#47496,#47497,#47498,#47499,#47500,
#47501,#47502,#47503,#47504,#47505,#47506,#47507,#47508,#47509,#47510,#47511,
#47512,#47513,#47514,#47515,#47516,#47517,#47518,#47519,#47520,#47521,#47522,
#47523,#47524,#47525,#47526,#47527,#47528,#47529,#47530,#47531,#47532,#47533,
#47534,#47535,#47536,#47537,#47538,#47539,#47540,#47541,#47542,#47543,#47544,
#47545,#47546,#47547,#47548,#47549,#47550,#47551,#47552,#47553,#47554,#47555,
#47556,#47557,#47558,#47559,#47560,#47561,#47562,#47563,#47564,#47565,#47566,
#47567,#47568,#47569,#47570,#47571,#47572,#47573,#47574,#47575,#47576,#47577,
#47578,#47579),.UNSPECIFIED.,.F.,.F.,(4,2,2,2,2,2,2,2,2,2,2,2,2,2,2,2,2,
2,2,2,2,2,2,2,2,2,2,2,2,2,2,2,2,2,2,2,2,2,2,2,2,2,2,2,2,2,2,2,2,2,2,2,2,
2,2,2,2,2,2,2,2,2,2,2,2,2,2,2,2,2,2,2,2,2,2,2,2,2,2,2,2,2,2,2,2,2,2,2,2,
2,2,2,2,2,2,2,2,2,2,2,2,2,2,2,2,2,2,2,2,2,2,2,2,2,2,2,2,2,4),(-1.29825834795597,
-1.29123229092342,-1.28602653061877,-1.28324731967477,-1.28116624603691,
-1.27853959641259,-1.27404412637148,-1.25730238843777,-1.22458933826295,
-1.19048854204325,-1.18567886039837,-1.18372563591847,-1.18251742264463,
-1.18116576825898,-1.17916390624951,-1.17365253509172,-1.16518073419774,
-1.1046732911913,-1.09040568752403,-1.08615969824611,-1.08358801057558,
-1.08126657320199,-1.0782897747918,-1.07210141763832,-1.04869905839798,
-1.02244590874265,-0.991437463326771,-0.986604499062264,-0.98464753312995,
-0.98343874508643,-0.982088148423329,-0.980090820162957,-0.974610538158568,
-0.966202942906196,-0.936106345915818,-0.896617770542071,-0.889303357891865,
-0.886359127148623,-0.884187423377715,-0.881826185490253,-0.878587373419486,
-0.870943890916088,-0.860314813266051,-0.829341363081878,-0.792290315776044,
-0.787553784610154,-0.785612862203943,-0.784287032959841,-0.782904896261069,
-0.780760835209874,-0.774155979058116,-0.763287687444722,-0.708443228461425,
-0.692639211776866,-0.68823984302026,-0.685634550525839,-0.683551169459506,
-0.680744019251714,-0.675402913302647,-0.632480468576317,-0.593034951823787,
-0.588426491595111,-0.586696601157218,-0.585465433331811,-0.584136622106021,
-0.582249183658804,-0.577503904549001,-0.552798002155749,-0.512281684402921,
-0.493995753103682,-0.489437230267483,-0.486770463735911,-0.484462403020355,
-0.481631776240677,-0.476177541548953,-0.469272896926145,-0.453448973639084,
-0.416407945837161,-0.391843153536159,-0.388662103396604,-0.387034752223112,
-0.385741088598687,-0.384203429399182,-0.381351076316759,-0.364821427219705,
-0.305192063682197,-0.293613971076619,-0.289682514395162,-0.287180055190972,
-0.284837889688967,-0.281711620366249,-0.274716410776126,-0.244971085234562,
-0.213389191432959,-0.192666474932515,-0.189556669796834,-0.187944726748438,
-0.18669092098631,-0.186683178564903,-0.186675500392306,-0.186667885331728,
-0.186660332243027,-0.186652840091513,-0.186645407650691,-0.186638033859088,
-0.186630717608753,-0.185102328142878,-0.183441804139831,-0.180803067062052,
-0.175631169124425,-0.162027308915024,-0.11606608232098,-0.0961395206307786,
-0.0914679593369492,-0.088775632090244,-0.0864915565936915,-0.0837030370058112,
-0.0784507275611289,-0.041493788302871),.UNSPECIFIED.);
#571=B_SPLINE_CURVE_WITH_KNOTS('',3,(#47585,#47586,#47587,#47588,#47589,
#47590,#47591,#47592,#47593,#47594,#47595,#47596,#47597,#47598,#47599,#47600,
#47601,#47602,#47603,#47604,#47605,#47606,#47607,#47608,#47609,#47610,#47611,
#47612,#47613,#47614,#47615,#47616,#47617,#47618,#47619,#47620,#47621,#47622,
#47623,#47624,#47625,#47626,#47627,#47628,#47629,#47630,#47631,#47632,#47633,
#47634,#47635,#47636,#47637,#47638,#47639,#47640,#47641,#47642,#47643,#47644,
#47645,#47646,#47647,#47648,#47649,#47650,#47651,#47652,#47653,#47654,#47655,
#47656,#47657,#47658,#47659,#47660,#47661,#47662,#47663,#47664,#47665,#47666,
#47667,#47668,#47669,#47670,#47671,#47672,#47673,#47674,#47675,#47676,#47677,
#47678,#47679,#47680,#47681,#47682,#47683,#47684,#47685,#47686,#47687,#47688,
#47689,#47690,#47691,#47692,#47693,#47694,#47695,#47696,#47697,#47698,#47699,
#47700,#47701,#47702,#47703,#47704,#47705,#47706,#47707,#47708,#47709,#47710,
#47711,#47712,#47713,#47714,#47715,#47716,#47717,#47718,#47719,#47720,#47721,
#47722,#47723,#47724,#47725,#47726,#47727,#47728,#47729,#47730,#47731,#47732,
#47733,#47734,#47735,#47736,#47737,#47738,#47739,#47740,#47741,#47742,#47743,
#47744,#47745,#47746,#47747,#47748,#47749,#47750,#47751,#47752,#47753,#47754,
#47755,#47756,#47757,#47758,#47759,#47760,#47761,#47762,#47763,#47764,#47765,
#47766,#47767,#47768),.UNSPECIFIED.,.F.,.F.,(4,3,3,3,3,3,3,3,3,3,3,3,3,
3,3,3,3,3,3,3,3,3,3,3,3,3,3,3,3,3,3,3,3,3,3,3,3,3,3,3,3,3,3,3,3,3,3,3,3,
3,3,3,3,3,3,3,3,3,3,3,3,4),(72.2566310325653,72.3602553809559,72.4638199284958,
72.5673616020167,72.6732883015743,72.7769587590038,72.8840135796256,72.9910684002473,
73.0960616494774,73.200898215455,73.3056124113295,73.4102613487264,73.5148805337815,
73.6195054291833,73.7242406132493,73.8290373507608,73.9340142903564,73.9861901029102,
74.0911833521404,74.1960199181177,74.3007341139922,74.4053830513891,74.5100022364442,
74.6146271318463,74.7193623159124,74.8241590534239,74.9291359930195,74.981311805573,
75.0863050548031,75.1911416207804,75.2958558166549,75.4005047540517,75.5051239391068,
75.6097488345088,75.7144840185748,75.8192807560863,75.9242576956819,75.9764335082359,
76.0814267574661,76.1862633234431,76.2909775193177,76.3956264567146,76.5002456417698,
76.6048705371713,76.7096057212374,76.8144024587489,76.9193793983445,76.9715552108987,
77.0765484601287,77.1813850261059,77.2860992219805,77.3907481593772,77.4953673444324,
77.5999922398345,77.7047274239005,77.8095241614122,77.9145011010078,77.9666769135615,
78.0739238974765,78.1810066065371,78.2879201148065,78.336051653945),
 .UNSPECIFIED.);
#572=B_SPLINE_CURVE_WITH_KNOTS('',3,(#47769,#47770,#47771,#47772),
 .UNSPECIFIED.,.F.,.F.,(4,4),(-2.51409019964695,-2.4734065574123),
 .UNSPECIFIED.);
#573=B_SPLINE_CURVE_WITH_KNOTS('',3,(#47774,#47775,#47776,#47777,#47778,
#47779),.UNSPECIFIED.,.F.,.F.,(4,2,4),(-0.041493788302871,-0.0346416690046193,
-0.000583262449505623),.UNSPECIFIED.);
#574=B_SPLINE_CURVE_WITH_KNOTS('',3,(#47780,#47781,#47782,#47783,#47784,
#47785,#47786,#47787,#47788,#47789,#47790,#47791,#47792,#47793,#47794,#47795,
#47796,#47797,#47798,#47799,#47800,#47801,#47802,#47803,#47804,#47805,#47806,
#47807,#47808,#47809,#47810,#47811,#47812,#47813,#47814,#47815,#47816,#47817,
#47818,#47819,#47820,#47821,#47822,#47823,#47824,#47825,#47826,#47827,#47828,
#47829,#47830,#47831,#47832,#47833,#47834,#47835,#47836,#47837,#47838,#47839,
#47840,#47841,#47842,#47843,#47844,#47845,#47846,#47847,#47848,#47849,#47850,
#47851,#47852,#47853,#47854,#47855,#47856,#47857,#47858,#47859,#47860,#47861,
#47862,#47863,#47864,#47865,#47866,#47867,#47868,#47869,#47870,#47871,#47872,
#47873,#47874,#47875,#47876,#47877,#47878,#47879,#47880,#47881,#47882,#47883,
#47884,#47885,#47886,#47887,#47888,#47889,#47890,#47891,#47892,#47893,#47894,
#47895,#47896,#47897,#47898,#47899,#47900,#47901,#47902,#47903,#47904,#47905,
#47906,#47907,#47908,#47909,#47910,#47911,#47912,#47913,#47914,#47915,#47916,
#47917,#47918,#47919,#47920,#47921,#47922,#47923,#47924,#47925,#47926,#47927,
#47928,#47929,#47930,#47931,#47932,#47933,#47934,#47935,#47936,#47937,#47938,
#47939,#47940,#47941,#47942,#47943,#47944,#47945,#47946,#47947,#47948,#47949,
#47950,#47951,#47952,#47953,#47954,#47955,#47956,#47957,#47958,#47959,#47960,
#47961,#47962,#47963,#47964,#47965,#47966,#47967,#47968,#47969,#47970,#47971,
#47972,#47973,#47974,#47975,#47976,#47977,#47978,#47979,#47980,#47981,#47982,
#47983,#47984,#47985,#47986,#47987,#47988,#47989,#47990,#47991,#47992,#47993,
#47994,#47995,#47996,#47997,#47998,#47999,#48000,#48001,#48002,#48003),
 .UNSPECIFIED.,.F.,.F.,(4,2,2,2,2,2,2,2,2,2,2,2,2,2,2,2,2,2,2,2,2,2,2,2,
2,2,2,2,2,2,2,2,2,2,2,2,2,2,2,2,2,2,2,2,2,2,2,2,2,2,2,2,2,2,2,2,2,2,2,2,
2,2,2,2,2,2,2,2,2,2,2,2,2,2,2,2,2,2,2,2,2,2,2,2,2,2,2,2,2,2,2,2,2,2,2,2,
2,2,2,2,2,2,2,2,2,2,2,2,2,2,2,4),(-2.51380311614403,-2.5057188902465,-2.50390337305145,
-2.50257646804571,-2.50135832362811,-2.50014405372957,-2.49847678018933,
-2.49513428537836,-2.48528681981277,-2.44176071704383,-2.41372553721965,
-2.40693781727606,-2.4038499815795,-2.40151474568926,-2.39930555125731,
-2.39559180528697,-2.38558201918726,-2.32022389081281,-2.31145165745222,
-2.30762322644957,-2.30548677708257,-2.30362737465592,-2.30231906796012,
-2.30109681102103,-2.2993992272215,-2.29502015054223,-2.25255271667082,
-2.2122212141153,-2.20699962375403,-2.20421810288363,-2.20213792126715,
-2.19951586008346,-2.19503687021547,-2.17846988738744,-2.12446576606885,
-2.10836160348672,-2.10552785894564,-2.10399453337647,-2.1027011064052,
-2.10106973833147,-2.09786813605386,-2.06988250608802,-2.03673414804337,
-2.02068900706426,-2.01371865924593,-2.00822332833925,-2.00538488588434,
-2.00307712132473,-2.00041811730562,-1.99589094348477,-1.9779692450429,
-1.93720972933782,-1.91233601420066,-1.90757622789669,-1.90568688219965,
-1.90435804943943,-1.90312791592093,-1.90140092337691,-1.89681126371826,
-1.85701485778536,-1.81449304220479,-1.80915018370927,-1.80634320712155,
-1.80426040555171,-1.80165643180366,-1.79726072499105,-1.78148587064127,
-1.72660185231637,-1.71573004400992,-1.70912479807251,-1.70698105967961,
-1.70559925545828,-1.70427384355068,-1.70233369566118,-1.69759982566183,
-1.66056625049074,-1.62962657454605,-1.61900536744556,-1.61136602308453,
-1.60812841143886,-1.60576784127861,-1.60359660075783,-1.60065276770379,
-1.59333819324359,-1.5538687041214,-1.52373991786759,-1.51532798084632,
-1.50984642709876,-1.50784921361958,-1.50649887481976,-1.50529044989673,
-1.50333432227674,-1.49850466511426,-1.46609143223948,-1.43219103696873,
-1.42070617305763,-1.41259625959539,-1.40928120813914,-1.40690654525286,
-1.4047511351797,-1.4013308910304,-1.39497634440314,-1.34617882612164,-1.3228721828953,
-1.31559392671055,-1.31067345759629,-1.30875891696104,-1.30742515108399,
-1.30620059109701,-1.30449499662752,-1.3000647200745,-1.29834900329513),
 .UNSPECIFIED.);
#575=B_SPLINE_CURVE_WITH_KNOTS('',3,(#48009,#48010,#48011,#48012,#48013,
#48014,#48015,#48016,#48017,#48018,#48019,#48020,#48021,#48022,#48023,#48024,
#48025,#48026,#48027,#48028,#48029,#48030,#48031,#48032,#48033,#48034,#48035,
#48036,#48037,#48038,#48039,#48040,#48041,#48042,#48043,#48044,#48045,#48046,
#48047,#48048,#48049,#48050,#48051,#48052,#48053,#48054,#48055,#48056,#48057,
#48058,#48059,#48060,#48061,#48062,#48063,#48064,#48065,#48066,#48067,#48068,
#48069,#48070,#48071,#48072,#48073,#48074,#48075,#48076,#48077,#48078,#48079,
#48080,#48081,#48082,#48083,#48084,#48085,#48086,#48087,#48088,#48089,#48090,
#48091,#48092,#48093,#48094,#48095,#48096,#48097,#48098,#48099,#48100,#48101,
#48102,#48103,#48104,#48105,#48106,#48107,#48108,#48109,#48110,#48111,#48112,
#48113,#48114,#48115,#48116,#48117,#48118,#48119,#48120,#48121,#48122,#48123,
#48124,#48125,#48126,#48127,#48128,#48129,#48130,#48131,#48132,#48133,#48134,
#48135,#48136,#48137,#48138,#48139,#48140,#48141,#48142,#48143,#48144,#48145,
#48146,#48147,#48148,#48149,#48150,#48151,#48152,#48153,#48154,#48155,#48156,
#48157,#48158,#48159,#48160,#48161,#48162,#48163,#48164,#48165,#48166,#48167,
#48168,#48169,#48170,#48171,#48172,#48173,#48174,#48175,#48176,#48177,#48178,
#48179,#48180,#48181,#48182,#48183,#48184,#48185,#48186,#48187,#48188,#48189,
#48190,#48191,#48192,#48193,#48194,#48195,#48196,#48197,#48198,#48199,#48200,
#48201,#48202,#48203,#48204,#48205,#48206,#48207,#48208,#48209,#48210,#48211,
#48212,#48213,#48214,#48215,#48216,#48217,#48218,#48219,#48220,#48221,#48222,
#48223,#48224,#48225,#48226,#48227,#48228,#48229,#48230,#48231,#48232,#48233,
#48234,#48235,#48236,#48237,#48238,#48239,#48240,#48241,#48242,#48243,#48244,
#48245,#48246),.UNSPECIFIED.,.F.,.F.,(4,2,2,2,2,2,2,2,2,2,2,2,2,2,2,2,2,
2,2,2,2,2,2,2,2,2,2,2,2,2,2,2,2,2,2,2,2,2,2,2,2,2,2,2,2,2,2,2,2,2,2,2,2,
2,2,2,2,2,2,2,2,2,2,2,2,2,2,2,2,2,2,2,2,2,2,2,2,2,2,2,2,2,2,2,2,2,2,2,2,
2,2,2,2,2,2,2,2,2,2,2,2,2,2,2,2,2,2,2,2,2,2,2,2,2,2,2,2,2,4),(-1.21658137004514,
-1.1891249839804,-1.1843917540007,-1.18143090687014,-1.17911169725611,-1.17653198226384,
-1.17224815723712,-1.15574253158255,-1.09376935906015,-1.08456372110044,
-1.08204876568971,-1.08058446891245,-1.07927988123128,-1.07754095822139,
-1.07367086323986,-1.06835697899584,-1.0541898966876,-1.00572967857163,
-0.988715278580078,-0.984255077292539,-0.981610878746839,-0.979300866989459,
-0.976440201664556,-0.970838824113962,-0.931739979786828,-0.888544954491291,
-0.884191888413404,-0.882497926606543,-0.881276221370208,-0.879939249599092,
-0.878009546020247,-0.872991747009221,-0.865522653847871,-0.841170505219558,
-0.793952846619021,-0.786766266065938,-0.783921548247851,-0.781559209727695,
-0.77913686767823,-0.775582341858262,-0.765878726818815,-0.751285666006921,
-0.721090668731977,-0.690178943060794,-0.685342668611477,-0.683385110578194,
-0.682176185169055,-0.680825658063772,-0.678828821404486,-0.673352317519568,
-0.66495265862472,-0.634910248621997,-0.59535003929974,-0.588036431321171,
-0.585092277732971,-0.582920543405897,-0.580559187884376,-0.577320061322963,
-0.569675110979303,-0.559043485783338,-0.52805790291404,-0.491021286121869,
-0.486284099893265,-0.484343028524726,-0.483017137351736,-0.481634975426314,
-0.479490943649205,-0.472886718508895,-0.462020032633777,-0.407207753238175,
-0.391371892227016,-0.386969374816044,-0.384363333825422,-0.382279973594379,
-0.379473655660843,-0.374136846508977,-0.330609740525097,-0.291816863380292,
-0.287164954229007,-0.285429083749242,-0.28419628866504,-0.282868640438062,
-0.280987634957947,-0.276283151283912,-0.252013880783432,-0.222217868926318,
-0.193681998635353,-0.189039120965494,-0.186105130120254,-0.183845936529115,
-0.183750679937684,-0.183675581972278,-0.183615743063987,-0.183567664959165,
-0.183528781625933,-0.183497169253304,-0.183444700826453,-0.183394391883649,
-0.183346079567604,-0.183299616694927,-0.183254869807652,-0.183211717708318,
-0.183170049975852,-0.183129765793954,-0.183090772939764,-0.183052986826154,
-0.180212188641947,-0.177123262222999,-0.172136563485539,-0.162198427827386,
-0.115791646890992,-0.090547535821272,-0.0873640374779424,-0.0857360691090431,
-0.0844422519689053,-0.0829048087542316,-0.0800539024920105,-0.0635645684128408,
-0.000583171670547464),.UNSPECIFIED.);
#576=B_SPLINE_CURVE_WITH_KNOTS('',3,(#48247,#48248,#48249,#48250,#48251,
#48252,#48253),.UNSPECIFIED.,.F.,.F.,(4,3,4),(78.336051653945,78.4428050925864,
78.5398163397449),.UNSPECIFIED.);
#577=B_SPLINE_CURVE_WITH_KNOTS('',3,(#48254,#48255,#48256,#48257,#48258,
#48259,#48260,#48261,#48262,#48263,#48264,#48265,#48266,#48267,#48268,#48269,
#48270,#48271,#48272,#48273,#48274,#48275,#48276,#48277,#48278,#48279,#48280,
#48281,#48282,#48283,#48284,#48285,#48286,#48287,#48288,#48289,#48290,#48291,
#48292,#48293,#48294,#48295,#48296,#48297,#48298,#48299,#48300,#48301,#48302,
#48303,#48304,#48305,#48306,#48307,#48308,#48309,#48310,#48311,#48312,#48313,
#48314,#48315,#48316,#48317,#48318,#48319,#48320,#48321,#48322,#48323,#48324,
#48325,#48326,#48327,#48328,#48329,#48330,#48331,#48332,#48333,#48334,#48335,
#48336,#48337,#48338,#48339,#48340,#48341,#48342,#48343,#48344,#48345,#48346,
#48347,#48348,#48349,#48350,#48351,#48352,#48353,#48354,#48355,#48356,#48357,
#48358,#48359,#48360,#48361,#48362,#48363,#48364,#48365,#48366,#48367,#48368,
#48369,#48370,#48371,#48372,#48373,#48374,#48375,#48376,#48377,#48378,#48379,
#48380,#48381,#48382,#48383,#48384,#48385,#48386,#48387,#48388,#48389,#48390,
#48391,#48392,#48393,#48394,#48395,#48396,#48397,#48398,#48399,#48400,#48401,
#48402,#48403,#48404,#48405,#48406,#48407,#48408,#48409,#48410,#48411,#48412,
#48413,#48414,#48415,#48416,#48417,#48418,#48419,#48420,#48421,#48422,#48423,
#48424,#48425,#48426,#48427,#48428,#48429,#48430,#48431,#48432,#48433,#48434,
#48435,#48436,#48437,#48438,#48439,#48440,#48441,#48442,#48443,#48444,#48445,
#48446,#48447,#48448,#48449,#48450,#48451,#48452,#48453,#48454,#48455,#48456,
#48457,#48458,#48459,#48460,#48461,#48462,#48463,#48464,#48465,#48466,#48467),
 .UNSPECIFIED.,.F.,.F.,(4,2,2,2,2,2,2,2,2,2,2,2,2,2,2,2,2,2,2,2,2,2,2,2,
2,2,2,2,2,2,2,2,2,2,2,2,2,2,2,2,2,2,2,2,2,2,2,2,2,2,2,2,2,2,2,2,2,2,2,2,
2,2,2,2,2,2,2,2,2,2,2,2,2,2,2,2,2,2,2,2,2,2,2,2,2,2,2,2,2,2,2,2,2,2,2,2,
2,2,2,2,2,2,2,2,2,2,4),(-1.29834900329513,-1.25769021628927,-1.21735607324619,
-1.21263190090603,-1.20967386889312,-1.20735510138914,-1.20477406029058,
-1.20048375289467,-1.18389667504742,-1.12081858482312,-1.11261720688062,
-1.11020573147173,-1.10876440566488,-1.10745315500985,-1.10566768037584,
-1.1015361016775,-1.08285159066525,-1.03535184568982,-1.01714043042331,
-1.01258739326859,-1.00992196706622,-1.0078447531676,-1.00511361576107,
-1.00013392309523,-0.970900720720121,-0.935194953403005,-0.927291043545992,
-0.914321163787172,-0.911787692663085,-0.910171056051705,-0.908877980806288,
-0.90733158191397,-0.904437888767709,-0.886850461634557,-0.858538343808799,
-0.819287970420795,-0.814548009231563,-0.811584950934823,-0.809265243273779,
-0.806686244241806,-0.802406591509152,-0.78595612430463,-0.7246961065986,
-0.71482123216225,-0.712273339026079,-0.710786918663496,-0.709617240942895,
-0.70798792288454,-0.704692698584166,-0.700369134651098,-0.689919742061426,
-0.641322050429228,-0.632048711086285,-0.618247549860236,-0.614051893361414,
-0.611491123602568,-0.609166864531534,-0.606168650993029,-0.599869433120256,
-0.575652327407577,-0.535264902496132,-0.531253714115416,-0.516369866010922,
-0.513736250728469,-0.512089083090206,-0.510794040321335,-0.509271535630656,
-0.506490392836548,-0.49156785183812,-0.448228001386511,-0.42086121195442,
-0.416260735079831,-0.413339515701385,-0.411024012225265,-0.408419758047953,
-0.404026337512082,-0.386128308483794,-0.348514712031086,-0.3401378681956,
-0.335459963329045,-0.331895901021324,-0.317310579935759,-0.314691496716336,
-0.313048744779638,-0.311754048660356,-0.310228294326044,-0.307431898677704,
-0.292184788732463,-0.246355848138599,-0.221671323967535,-0.217152841288632,
-0.214256590269068,-0.21216828598887,-0.209677527262702,-0.20707537119769,
-0.203265316565563,-0.196486150564352,-0.181078706396089,-0.142737591051673,
-0.118770649616248,-0.115603323007869,-0.113978849986806,-0.112685266448303,
-0.111145086787342,-0.108281161234025,-0.0914698421241412,-0.0414797095138316),
 .UNSPECIFIED.);
#578=B_SPLINE_CURVE_WITH_KNOTS('',3,(#48472,#48473,#48474,#48475,#48476,
#48477,#48478,#48479,#48480,#48481,#48482,#48483,#48484,#48485,#48486,#48487,
#48488,#48489,#48490,#48491,#48492,#48493,#48494,#48495,#48496,#48497,#48498,
#48499,#48500,#48501,#48502,#48503,#48504,#48505,#48506,#48507,#48508,#48509,
#48510,#48511,#48512,#48513,#48514,#48515,#48516,#48517,#48518,#48519,#48520,
#48521,#48522,#48523,#48524,#48525,#48526,#48527,#48528,#48529,#48530,#48531,
#48532,#48533,#48534,#48535,#48536,#48537,#48538,#48539,#48540,#48541,#48542,
#48543,#48544,#48545,#48546,#48547,#48548,#48549,#48550,#48551,#48552,#48553,
#48554,#48555,#48556,#48557,#48558,#48559,#48560,#48561,#48562,#48563,#48564,
#48565,#48566,#48567,#48568,#48569,#48570,#48571,#48572,#48573,#48574,#48575,
#48576,#48577,#48578,#48579,#48580,#48581,#48582,#48583,#48584,#48585,#48586,
#48587,#48588,#48589,#48590,#48591,#48592,#48593,#48594,#48595,#48596,#48597,
#48598,#48599,#48600,#48601,#48602,#48603,#48604,#48605,#48606,#48607,#48608,
#48609,#48610,#48611,#48612,#48613,#48614,#48615,#48616,#48617,#48618,#48619,
#48620,#48621,#48622,#48623,#48624,#48625,#48626,#48627,#48628,#48629,#48630,
#48631,#48632,#48633,#48634,#48635,#48636,#48637,#48638,#48639,#48640,#48641,
#48642,#48643,#48644,#48645,#48646,#48647,#48648,#48649,#48650,#48651,#48652,
#48653,#48654,#48655,#48656,#48657,#48658,#48659,#48660,#48661,#48662,#48663,
#48664,#48665,#48666,#48667,#48668,#48669,#48670,#48671,#48672,#48673,#48674,
#48675,#48676,#48677,#48678,#48679,#48680,#48681,#48682,#48683),
 .UNSPECIFIED.,.F.,.F.,(4,2,2,2,2,2,2,2,2,2,2,2,2,2,2,2,2,2,2,2,2,2,2,2,
2,2,2,2,2,2,2,2,2,2,2,2,2,2,2,2,2,2,2,2,2,2,2,2,2,2,2,2,2,2,2,2,2,2,2,2,
2,2,2,2,2,2,2,2,2,2,2,2,2,2,2,2,2,2,2,2,2,2,2,2,2,2,2,2,2,2,2,2,2,2,2,2,
2,2,2,2,2,2,2,2,2,4),(-2.47330352940323,-2.47280614242241,-2.4711756610841,
-2.46797964661157,-2.43960318315561,-2.42172026383921,-2.40591459269085,
-2.38677460043587,-2.37943395651363,-2.37618822907268,-2.37382579792882,
-2.37165566101622,-2.36871761703384,-2.36140609639352,-2.32049284656353,
-2.29148639305627,-2.27915696341582,-2.27658115067425,-2.27532535894301,
-2.2741550328263,-2.27267372870349,-2.27014746237708,-2.26050939864939,
-2.19903388004811,-2.18256954668905,-2.17828905454494,-2.17571000992547,
-2.17339055189566,-2.17042821398372,-2.16569017671535,-2.126337966641,-2.09782835895185,
-2.08048501145368,-2.07760059542768,-2.07605623995757,-2.07476316327683,
-2.07314438168212,-2.07000276304802,-2.04844520065214,-1.99588895420398,
-1.98290086511098,-1.97894623463244,-1.9764388474031,-1.97409889657658,
-1.97103929983643,-1.96422796104393,-1.91305571414945,-1.88238468702453,
-1.87890681664904,-1.87724177884773,-1.87595733776832,-1.87445308451574,
-1.87182665421821,-1.8610179778599,-1.80653839398111,-1.78511786598161,
-1.78049289825892,-1.77783848381455,-1.77552993218143,-1.77268441683706,
-1.76833045158494,-1.74687689351158,-1.69787064445871,-1.68225286051899,
-1.67943989844966,-1.67791078637913,-1.67661667464073,-1.67497904740741,
-1.67237633995476,-1.65811016173779,-1.65252892927466,-1.6128500606956,
-1.58884361882339,-1.58257311247748,-1.57958078748119,-1.57725770531214,
-1.57469480614609,-1.57048780261165,-1.55657746088346,-1.50562015581286,
-1.49060640987102,-1.48508494857162,-1.48109885171595,-1.47933909390867,
-1.47803171681945,-1.47657829054539,-1.47411213578008,-1.46539313685228,
-1.40292039766669,-1.38637984987438,-1.38209329515882,-1.37951302275186,
-1.37719399952684,-1.3742343382562,-1.36950488169606,-1.32953036843299,
-1.29738107416082,-1.28397005257281,-1.28126745941335,-1.27976221539201,
-1.27846564292004,-1.27679548575481,-1.27408449122815,-1.25752712896311,
-1.22864179188508,-1.21658137004514),.UNSPECIFIED.);
#579=B_SPLINE_CURVE_WITH_KNOTS('',3,(#48685,#48686,#48687,#48688,#48689,
#48690,#48691,#48692,#48693,#48694,#48695,#48696,#48697,#48698,#48699,#48700,
#48701,#48702),.UNSPECIFIED.,.F.,.F.,(4,2,2,2,2,2,2,2,4),(-0.0414797095138316,
-0.0326304630026233,-0.0206541176175663,-0.0166774261868832,-0.0141649808844975,
-0.0119423353386409,-0.00967246363527554,-0.00562235294686388,-0.000582410650389689),
 .UNSPECIFIED.);
#580=B_SPLINE_CURVE_WITH_KNOTS('',3,(#48703,#48704,#48705,#48706,#48707,
#48708,#48709,#48710,#48711,#48712,#48713,#48714,#48715,#48716,#48717,#48718,
#48719,#48720,#48721,#48722,#48723,#48724,#48725,#48726,#48727,#48728,#48729,
#48730,#48731,#48732,#48733,#48734,#48735,#48736,#48737,#48738,#48739,#48740,
#48741,#48742,#48743,#48744,#48745,#48746,#48747,#48748,#48749,#48750,#48751,
#48752,#48753,#48754,#48755,#48756,#48757,#48758,#48759,#48760,#48761,#48762,
#48763,#48764,#48765,#48766,#48767,#48768,#48769,#48770,#48771,#48772,#48773,
#48774,#48775,#48776,#48777,#48778,#48779,#48780,#48781,#48782,#48783,#48784,
#48785,#48786,#48787,#48788,#48789,#48790,#48791,#48792,#48793,#48794,#48795,
#48796,#48797,#48798,#48799,#48800,#48801,#48802,#48803,#48804,#48805,#48806,
#48807,#48808,#48809,#48810,#48811,#48812,#48813,#48814,#48815,#48816,#48817,
#48818,#48819,#48820,#48821,#48822,#48823,#48824,#48825,#48826,#48827,#48828,
#48829,#48830,#48831,#48832,#48833,#48834,#48835,#48836,#48837,#48838,#48839,
#48840,#48841,#48842,#48843,#48844,#48845,#48846,#48847,#48848,#48849,#48850,
#48851,#48852,#48853,#48854,#48855,#48856,#48857,#48858,#48859,#48860,#48861,
#48862,#48863,#48864,#48865,#48866,#48867,#48868,#48869,#48870,#48871,#48872,
#48873,#48874,#48875,#48876,#48877,#48878,#48879,#48880,#48881,#48882,#48883,
#48884,#48885,#48886,#48887,#48888,#48889,#48890,#48891,#48892,#48893,#48894,
#48895,#48896,#48897,#48898,#48899,#48900,#48901,#48902,#48903,#48904,#48905,
#48906),.UNSPECIFIED.,.F.,.F.,(4,2,2,2,2,2,2,2,2,2,2,2,2,2,2,2,2,2,2,2,
2,2,2,2,2,2,2,2,2,2,2,2,2,2,2,2,2,2,2,2,2,2,2,2,2,2,2,2,2,2,2,2,2,2,2,2,
2,2,2,2,2,2,2,2,2,2,2,2,2,2,2,2,2,2,2,2,2,2,2,2,2,2,2,2,2,2,2,2,2,2,2,2,
2,2,2,2,2,2,2,2,2,4),(-2.51371035365293,-2.4579504817706,-2.43416740516342,
-2.43004801671431,-2.42826483372786,-2.42695409888032,-2.42569340243194,
-2.42346779248273,-2.41682035801184,-2.35198938452692,-2.34096226702292,
-2.33559623235447,-2.33235203769843,-2.32953209064636,-2.32727584407651,
-2.32477982545212,-2.32087622259088,-2.3095078309908,-2.24961716772916,
-2.23306859439498,-2.2302157801933,-2.22867820112247,-2.22738479512049,
-2.22575801653735,-2.22257881244245,-2.19266679039188,-2.16151537431149,
-2.14539267592957,-2.13839880197559,-2.13288853662587,-2.13004669736339,
-2.12773829558897,-2.12508091436886,-2.12056222319378,-2.10276249916337,
-2.06192160984306,-2.03698100262777,-2.03221454124705,-2.03032391678356,
-2.02899465054679,-2.0277644886657,-2.02603796230798,-2.02145355324458,
-1.98147467137878,-1.93910692738182,-1.93376530375697,-1.93095824545593,
-1.92865178809561,-1.92596695496633,-1.92132805618564,-1.90187319043129,
-1.85083571142052,-1.83500549762557,-1.83218303215559,-1.83065185447081,
-1.82935786235572,-1.82772276086709,-1.82512848123981,-1.81102895595153,
-1.80513103306592,-1.78987777237792,-1.76117246414887,-1.74649221279437,
-1.73674525407137,-1.7331849049545,-1.73076151742669,-1.72840040203304,
-1.72555985795933,-1.71839878120607,-1.67081827678341,-1.64668913940135,
-1.6392602371041,-1.63426322589407,-1.6323367728804,-1.63100052242948,-1.62977826650148,
-1.62774906672787,-1.62247715032362,-1.55594593902264,-1.54485413063994,
-1.53695669802163,-1.53367609684562,-1.53130770775992,-1.5291454278617,
-1.52623813228733,-1.51913780518289,-1.47286199762123,-1.43759508102176,
-1.43434305891225,-1.43272266618112,-1.43155422303622,-1.43006225098546,
-1.42748922832941,-1.41732204744941,-1.35642138730097,-1.34000533668762,
-1.33572919419386,-1.3331513145379,-1.33083197846093,-1.32786851809341,
-1.32312609003501,-1.29776408237656),.UNSPECIFIED.);
#581=B_SPLINE_CURVE_WITH_KNOTS('',3,(#48912,#48913,#48914,#48915,#48916,
#48917,#48918,#48919,#48920,#48921,#48922,#48923,#48924,#48925,#48926,#48927,
#48928,#48929,#48930,#48931,#48932,#48933,#48934,#48935,#48936,#48937,#48938,
#48939,#48940,#48941,#48942,#48943,#48944,#48945,#48946,#48947,#48948,#48949,
#48950,#48951,#48952,#48953,#48954,#48955,#48956,#48957,#48958,#48959,#48960,
#48961,#48962,#48963,#48964,#48965,#48966,#48967,#48968,#48969,#48970,#48971,
#48972,#48973,#48974,#48975,#48976,#48977,#48978,#48979,#48980,#48981,#48982,
#48983,#48984,#48985,#48986,#48987,#48988,#48989,#48990,#48991,#48992,#48993,
#48994,#48995,#48996,#48997,#48998,#48999,#49000,#49001,#49002,#49003,#49004,
#49005,#49006,#49007,#49008,#49009,#49010,#49011,#49012,#49013,#49014,#49015,
#49016,#49017,#49018,#49019,#49020,#49021,#49022,#49023,#49024,#49025,#49026,
#49027,#49028,#49029,#49030,#49031,#49032,#49033,#49034,#49035,#49036,#49037,
#49038,#49039,#49040,#49041,#49042,#49043,#49044,#49045,#49046,#49047,#49048,
#49049,#49050,#49051,#49052,#49053,#49054,#49055,#49056,#49057,#49058,#49059,
#49060,#49061,#49062,#49063,#49064,#49065,#49066,#49067,#49068,#49069,#49070,
#49071,#49072,#49073,#49074,#49075,#49076,#49077,#49078,#49079,#49080,#49081,
#49082,#49083,#49084,#49085,#49086,#49087,#49088,#49089,#49090,#49091,#49092,
#49093,#49094,#49095,#49096,#49097,#49098,#49099,#49100,#49101,#49102,#49103,
#49104,#49105,#49106,#49107,#49108,#49109,#49110,#49111,#49112,#49113),
 .UNSPECIFIED.,.F.,.F.,(4,2,2,2,2,2,2,2,2,2,2,2,2,2,2,2,2,2,2,2,2,2,2,2,
2,2,2,2,2,2,2,2,2,2,2,2,2,2,2,2,2,2,2,2,2,2,2,2,2,2,2,2,2,2,2,2,2,2,2,2,
2,2,2,2,2,2,2,2,2,2,2,2,2,2,2,2,2,2,2,2,2,2,2,2,2,2,2,2,2,2,2,2,2,2,2,2,
2,2,2,2,4),(-1.21683047486584,-1.20679256159222,-1.16543709119454,-1.15844305223591,
-1.15617277744239,-1.15476283884563,-1.15343845239932,-1.15157488200906,
-1.14697850405559,-1.12383611992667,-1.09895533047361,-1.06443264535201,
-1.05968271506895,-1.0567166080109,-1.05439647483337,-1.05181901809905,
-1.04754664991083,-1.03118564928897,-0.970992344237733,-0.960105421157891,
-0.957472203332062,-0.955966145548304,-0.954681525503829,-0.953018031781168,
-0.949549535957342,-0.919942748590857,-0.867462827865426,-0.860809245694334,
-0.857777619158547,-0.855441539367763,-0.85292105326658,-0.84890872049112,
-0.835375022146676,-0.787857423192222,-0.761950954079996,-0.758760696070722,
-0.757131243673212,-0.75583729204823,-0.754300923174751,-0.751455243089941,
-0.735093884907736,-0.677919693028221,-0.664211245605211,-0.660025908777287,
-0.65746749366856,-0.655142804267596,-0.652140412272213,-0.645818768518974,
-0.621433276428417,-0.580427602991764,-0.576908853820052,-0.562329284511881,
-0.559710511922897,-0.558067866435139,-0.556773194997694,-0.555247400364807,
-0.552450753535979,-0.537197571217976,-0.491318514544147,-0.466663890333215,
-0.462160077727896,-0.459268318599959,-0.456955695209536,-0.454332792450086,
-0.44985392187971,-0.430755985057016,-0.387693860348781,-0.363777477763212,
-0.360610822319399,-0.358986486659055,-0.357692902078161,-0.356152590255361,
-0.3532880729308,-0.336462345462607,-0.273037661111589,-0.264549335977496,
-0.26107690882888,-0.25891193296584,-0.256545443178191,-0.253276419378178,
-0.245714404202163,-0.235092338387338,-0.204152554346614,-0.177308349506666,
-0.164066311524436,-0.161518036181473,-0.159896923336077,-0.158603699368851,
-0.157061198063145,-0.154514459216343,-0.141476710761522,-0.110310002664115,
-0.0724072341375291,-0.0650899867698462,-0.0621454468154719,-0.0599738095846168,
-0.0576129282440144,-0.0543751205765847,-0.0507846473231634,-0.0394419541871347,
-0.000582966585860259),.UNSPECIFIED.);
#582=B_SPLINE_CURVE_WITH_KNOTS('',3,(#49114,#49115,#49116,#49117,#49118,
#49119,#49120,#49121,#49122,#49123,#49124,#49125),.UNSPECIFIED.,.F.,.F.,
(4,2,2,2,2,4),(-2.5139747976882,-2.47986063878101,-2.47727398228966,-2.47563484175021,
-2.47409990132521,-2.47330352940323),.UNSPECIFIED.);
#583=B_SPLINE_CURVE_WITH_KNOTS('',3,(#49126,#49127,#49128,#49129,#49130,
#49131,#49132,#49133,#49134,#49135,#49136,#49137,#49138,#49139,#49140,#49141,
#49142,#49143,#49144,#49145,#49146,#49147,#49148,#49149,#49150,#49151,#49152,
#49153,#49154,#49155,#49156,#49157,#49158,#49159,#49160,#49161,#49162,#49163,
#49164,#49165,#49166,#49167,#49168,#49169,#49170,#49171,#49172,#49173,#49174,
#49175,#49176,#49177,#49178,#49179,#49180,#49181,#49182,#49183,#49184,#49185,
#49186,#49187,#49188,#49189,#49190,#49191,#49192,#49193,#49194,#49195,#49196,
#49197,#49198,#49199,#49200,#49201,#49202,#49203,#49204,#49205,#49206,#49207,
#49208,#49209,#49210,#49211,#49212,#49213,#49214,#49215,#49216,#49217,#49218,
#49219,#49220,#49221,#49222,#49223,#49224,#49225,#49226,#49227,#49228,#49229,
#49230,#49231,#49232,#49233,#49234,#49235,#49236,#49237,#49238,#49239,#49240,
#49241,#49242,#49243,#49244,#49245,#49246,#49247,#49248,#49249,#49250,#49251,
#49252,#49253,#49254,#49255,#49256,#49257,#49258,#49259,#49260,#49261,#49262,
#49263,#49264,#49265,#49266,#49267,#49268,#49269,#49270,#49271,#49272,#49273,
#49274,#49275,#49276,#49277,#49278,#49279,#49280,#49281,#49282,#49283,#49284,
#49285,#49286,#49287,#49288,#49289,#49290,#49291,#49292,#49293,#49294,#49295,
#49296,#49297,#49298,#49299,#49300,#49301,#49302,#49303,#49304,#49305,#49306,
#49307,#49308,#49309,#49310,#49311,#49312,#49313,#49314,#49315,#49316,#49317,
#49318,#49319,#49320,#49321,#49322,#49323,#49324,#49325,#49326,#49327,#49328,
#49329,#49330,#49331,#49332,#49333,#49334,#49335,#49336,#49337,#49338,#49339,
#49340,#49341,#49342,#49343,#49344,#49345),.UNSPECIFIED.,.F.,.F.,(4,2,2,
2,2,2,2,2,2,2,2,2,2,2,2,2,2,2,2,2,2,2,2,2,2,2,2,2,2,2,2,2,2,2,2,2,2,2,2,
2,2,2,2,2,2,2,2,2,2,2,2,2,2,2,2,2,2,2,2,2,2,2,2,2,2,2,2,2,2,2,2,2,2,2,2,
2,2,2,2,2,2,2,2,2,2,2,2,2,2,2,2,2,2,2,2,2,2,2,2,2,2,2,2,2,2,2,2,2,2,4),
(-1.29776408237656,-1.28432009226333,-1.25680382844245,-1.2528784758829,
-1.23800659097861,-1.23537428957193,-1.23372784705557,-1.23243331005041,
-1.23091132484804,-1.22813094060947,-1.21320760685108,-1.1698366198042,
-1.14253210028953,-1.13793505328303,-1.13501546220267,-1.13270090182622,
-1.13009734162604,-1.12570420162332,-1.10779405108135,-1.07011660389385,
-1.06348480410166,-1.03951434998688,-1.03634797718423,-1.03472404202459,
-1.03343091275736,-1.03189130473323,-1.02902852341146,-1.01222648624909,
-0.983346385135795,-0.943834982664761,-0.93910228251295,-0.93614177289407,
-0.933822831428776,-0.931243418614563,-0.926960104619756,-0.9104565711911,
-0.848492997300875,-0.839286150291822,-0.836771264950108,-0.835307088991741,
-0.834002664845639,-0.832264035653893,-0.828394895937816,-0.823082526364711,
-0.808920694111929,-0.76047429163564,-0.743450207156665,-0.738989535784814,
-0.73634541689553,-0.734035695925081,-0.731175676896869,-0.725576499116564,
-0.68652992082639,-0.643280646736572,-0.638934287405839,-0.637241530728495,
-0.636020230429521,-0.634683168190679,-0.632752438849346,-0.627726975238482,
-0.620242377925727,-0.595801390165363,-0.548722755129127,-0.541621265703519,
-0.538742473485475,-0.536586957222302,-0.534211696795687,-0.530894923104883,
-0.522776324393855,-0.51127450535185,-0.477290137704637,-0.44492794974094,
-0.440100232826018,-0.438144219647476,-0.436935662348577,-0.435584973786195,
-0.43358689960873,-0.428100753148054,-0.419680792069218,-0.389499198547466,
-0.350124516892673,-0.342808609693789,-0.339864240633898,-0.337692598974088,
-0.33533158697108,-0.332093371917713,-0.324452658339215,-0.313828379069186,
-0.282877708697353,-0.245786866345511,-0.24106096326923,-0.239121886924017,
-0.237796481891147,-0.236413959221531,-0.234381199865635,-0.228326969423526,
-0.185284654858206,-0.17930286323177,-0.147675970453935,-0.1429582134248,
-0.140001846486526,-0.137682927946228,-0.13510021508179,-0.130803582133839,
-0.114308930124998,-0.0928284065903526,-0.0721380315305199,-0.0444747427209316,
-0.041277742169082,-0.0412313986595946),.UNSPECIFIED.);
#584=B_SPLINE_CURVE_WITH_KNOTS('',3,(#49350,#49351,#49352,#49353,#49354,
#49355,#49356,#49357,#49358,#49359,#49360,#49361,#49362,#49363,#49364,#49365,
#49366,#49367,#49368,#49369,#49370,#49371,#49372,#49373,#49374,#49375,#49376,
#49377,#49378,#49379,#49380,#49381,#49382,#49383,#49384,#49385,#49386,#49387,
#49388,#49389,#49390,#49391,#49392,#49393,#49394,#49395,#49396,#49397,#49398,
#49399,#49400,#49401,#49402,#49403,#49404,#49405,#49406,#49407,#49408,#49409,
#49410,#49411,#49412,#49413,#49414,#49415,#49416,#49417,#49418,#49419,#49420,
#49421,#49422,#49423,#49424,#49425,#49426,#49427,#49428,#49429,#49430,#49431,
#49432,#49433,#49434,#49435,#49436,#49437,#49438,#49439,#49440,#49441,#49442,
#49443,#49444,#49445,#49446,#49447,#49448,#49449,#49450,#49451,#49452,#49453,
#49454,#49455,#49456,#49457,#49458,#49459,#49460,#49461,#49462,#49463,#49464,
#49465,#49466,#49467,#49468,#49469,#49470,#49471,#49472,#49473,#49474,#49475,
#49476,#49477,#49478,#49479,#49480,#49481,#49482,#49483,#49484,#49485,#49486,
#49487,#49488,#49489,#49490,#49491,#49492,#49493,#49494,#49495,#49496,#49497,
#49498,#49499,#49500,#49501,#49502,#49503,#49504,#49505,#49506,#49507,#49508,
#49509,#49510,#49511,#49512,#49513,#49514,#49515,#49516,#49517,#49518,#49519,
#49520,#49521,#49522,#49523,#49524,#49525,#49526,#49527,#49528,#49529,#49530,
#49531,#49532,#49533,#49534,#49535,#49536,#49537,#49538,#49539,#49540,#49541,
#49542,#49543,#49544,#49545,#49546,#49547,#49548,#49549,#49550,#49551,#49552,
#49553,#49554,#49555,#49556,#49557,#49558,#49559,#49560,#49561,#49562,#49563,
#49564,#49565,#49566,#49567,#49568,#49569,#49570,#49571),.UNSPECIFIED.,
 .F.,.F.,(4,2,2,2,2,2,2,2,2,2,2,2,2,2,2,2,2,2,2,2,2,2,2,2,2,2,2,2,2,2,2,
2,2,2,2,2,2,2,2,2,2,2,2,2,2,2,2,2,2,2,2,2,2,2,2,2,2,2,2,2,2,2,2,2,2,2,2,
2,2,2,2,2,2,2,2,2,2,2,2,2,2,2,2,2,2,2,2,2,2,2,2,2,2,2,2,2,2,2,2,2,2,2,2,
2,2,2,2,2,2,2,4),(-2.47379053097235,-2.47277706034237,-2.45616941361428,
-2.45187626101787,-2.44929391236621,-2.44697422438702,-2.44401536844734,
-2.4392905461352,-2.4002035463753,-2.37895316559793,-2.36207130719172,-2.35611108284694,
-2.35194700764502,-2.35014091991578,-2.34881997424031,-2.34740211450615,
-2.34509699755382,-2.3378229275557,-2.28755552908443,-2.2681124474593,-2.26017314504604,
-2.25408168955763,-2.25112344436621,-2.24880395067457,-2.24622152430073,
-2.24192755427174,-2.22722079040336,-2.2202433820079,-2.21471035435831,
-2.17644297809176,-2.15703383368175,-2.15282214965174,-2.15102263979531,
-2.14970904056391,-2.14827362748805,-2.14588934700611,-2.13793590743231,
-2.07459555771243,-2.05799040386735,-2.05369808027617,-2.05111626267205,
-2.04879707225391,-2.04583887922292,-2.0411151726313,-2.00202601282964,
-1.96913687927961,-1.95556962679675,-1.9528580948639,-1.95135075592513,
-1.95005420588683,-1.94838644972539,-1.94568396764216,-1.92934438661946,
-1.9139883508809,-1.8891589058606,-1.86281369368209,-1.85623546600458,-1.85318489192438,
-1.85085378274345,-1.84863046111866,-1.84484870177201,-1.83437924532905,
-1.77954755202239,-1.75904552485829,-1.75471657034165,-1.75289705397616,
-1.75158018145489,-1.75015316904785,-1.74780669110749,-1.74018419259941,
-1.67646746340632,-1.66548488211813,-1.65764669069571,-1.65437552253935,
-1.65200856163981,-1.64984389111909,-1.64692781252371,-1.63977807666126,
-1.59436499454103,-1.56872167767359,-1.56102640836016,-1.5558957727273,
-1.55394919225547,-1.55260895397547,-1.55139083685934,-1.54971048141597,
-1.54543769895588,-1.5015197045881,-1.46303829476585,-1.45745757749046,
-1.45460117703445,-1.45229155263442,-1.44964444198346,-1.44517129780746,
-1.42796859692916,-1.37961831176807,-1.36063108595812,-1.35646600106596,
-1.35467466373518,-1.35336247171798,-1.35192371217131,-1.34952392215997,
-1.34142946178886,-1.28348471803442,-1.26228869855122,-1.25767659876421,
-1.25502481699826,-1.25271576582657,-1.24986605401527,-1.24431776853978,
-1.21683047486584),.UNSPECIFIED.);
#585=B_SPLINE_CURVE_WITH_KNOTS('',3,(#49573,#49574,#49575,#49576,#49577,
#49578,#49579,#49580,#49581,#49582,#49583,#49584,#49585,#49586),
 .UNSPECIFIED.,.F.,.F.,(4,2,2,2,2,2,4),(-0.0412313986595946,-0.0396470820645504,
-0.038353352883166,-0.036818642137068,-0.0351798751504305,-0.0325941196013304,
-0.000582505019790992),.UNSPECIFIED.);
#586=B_SPLINE_CURVE_WITH_KNOTS('',3,(#49587,#49588,#49589,#49590,#49591,
#49592,#49593,#49594,#49595,#49596,#49597,#49598,#49599,#49600,#49601,#49602,
#49603,#49604,#49605,#49606,#49607,#49608,#49609,#49610,#49611,#49612,#49613,
#49614,#49615,#49616,#49617,#49618,#49619,#49620,#49621,#49622,#49623,#49624,
#49625,#49626,#49627,#49628,#49629,#49630,#49631,#49632,#49633,#49634,#49635,
#49636,#49637,#49638,#49639,#49640,#49641,#49642,#49643,#49644,#49645,#49646,
#49647,#49648,#49649,#49650,#49651,#49652,#49653,#49654,#49655,#49656,#49657,
#49658,#49659,#49660,#49661,#49662,#49663,#49664,#49665,#49666,#49667,#49668,
#49669,#49670,#49671,#49672,#49673,#49674,#49675,#49676,#49677,#49678,#49679,
#49680,#49681,#49682,#49683,#49684,#49685,#49686,#49687,#49688,#49689,#49690,
#49691,#49692,#49693,#49694,#49695,#49696,#49697,#49698,#49699,#49700,#49701,
#49702,#49703,#49704,#49705,#49706,#49707,#49708,#49709,#49710,#49711,#49712,
#49713,#49714,#49715,#49716,#49717,#49718,#49719,#49720,#49721,#49722,#49723,
#49724,#49725,#49726,#49727,#49728,#49729,#49730,#49731,#49732,#49733,#49734,
#49735,#49736,#49737,#49738,#49739,#49740,#49741,#49742,#49743,#49744,#49745,
#49746,#49747,#49748,#49749,#49750,#49751,#49752,#49753,#49754,#49755,#49756,
#49757,#49758,#49759,#49760,#49761,#49762,#49763,#49764,#49765,#49766,#49767,
#49768,#49769,#49770,#49771,#49772,#49773,#49774,#49775,#49776,#49777,#49778,
#49779,#49780,#49781,#49782,#49783,#49784,#49785,#49786,#49787,#49788,#49789,
#49790,#49791,#49792,#49793,#49794),.UNSPECIFIED.,.F.,.F.,(4,2,2,2,2,2,
2,2,2,2,2,2,2,2,2,2,2,2,2,2,2,2,2,2,2,2,2,2,2,2,2,2,2,2,2,2,2,2,2,2,2,2,
2,2,2,2,2,2,2,2,2,2,2,2,2,2,2,2,2,2,2,2,2,2,2,2,2,2,2,2,2,2,2,2,2,2,2,2,
2,2,2,2,2,2,2,2,2,2,2,2,2,2,2,2,2,2,2,2,2,2,2,2,2,4),(-2.51364950707999,
-2.46516245737415,-2.46005517763998,-2.45576754002935,-2.45318755664763,
-2.45086938983275,-2.44791164329971,-2.44318691055976,-2.40403108147615,
-2.3817763523131,-2.36570047798798,-2.3570881685732,-2.35478757315713,-2.35355825771939,
-2.35226531411621,-2.35063936543889,-2.34746250935437,-2.32261004107419,
-2.28039792543269,-2.26151107224442,-2.25702874626616,-2.25440603863628,
-2.25209492729012,-2.24920682686437,-2.2447120938145,-2.22024105461167,
-2.17419215983501,-2.15892103831632,-2.15612462883171,-2.1545993970621,
-2.15330546089989,-2.15166408790375,-2.14904800061621,-2.13450001635116,
-2.13105269901126,-2.11744862642065,-2.08021139904624,-2.06241048495044,
-2.05802609220555,-2.05542474162584,-2.05311030301585,-2.05018838508111,
-2.04558273145918,-2.01799466936758,-1.97486230763878,-1.95997130895771,
-1.95719271316586,-1.95567125582441,-1.95437688474557,-1.95273030180939,
-1.95009713149807,-1.93532539569104,-1.93156099143708,-1.89096967889108,
-1.86670067938995,-1.86039573032512,-1.85739736873002,-1.85507410795253,
-1.85251555981715,-1.84832611334552,-1.83456904106027,-1.77745464575305,
-1.7610988176287,-1.75825422161019,-1.75671849278625,-1.75542510772869,
-1.7537964120863,-1.7506077621314,-1.72470375950036,-1.68334369378189,-1.66459879954058,
-1.66014551148911,-1.65752876310615,-1.65521619427778,-1.65231738443914,
-1.64778871577487,-1.62247466217351,-1.58530993182366,-1.56447655225384,
-1.56011372478146,-1.55828894767348,-1.55697160527419,-1.5555475979752,
-1.55321297052502,-1.54568659129769,-1.48188938944291,-1.4709066146748,
-1.46306907324937,-1.45979882400841,-1.45743275793673,-1.45526906370794,
-1.45235453859142,-1.44520981142519,-1.39977491042776,-1.37417104185583,
-1.36648389757969,-1.36135784304428,-1.35941243019359,-1.35807281538934,
-1.35685512431365,-1.35517517251909,-1.35090243194385,-1.30701829225585,
-1.298038620556),.UNSPECIFIED.);
#587=B_SPLINE_CURVE_WITH_KNOTS('',3,(#49800,#49801,#49802,#49803,#49804,
#49805,#49806,#49807,#49808,#49809,#49810,#49811,#49812,#49813,#49814,#49815,
#49816,#49817,#49818,#49819,#49820,#49821,#49822,#49823,#49824,#49825,#49826,
#49827,#49828,#49829,#49830,#49831,#49832,#49833,#49834,#49835,#49836,#49837,
#49838,#49839,#49840,#49841,#49842,#49843,#49844,#49845,#49846,#49847,#49848,
#49849,#49850,#49851,#49852,#49853,#49854,#49855,#49856,#49857,#49858,#49859,
#49860,#49861,#49862,#49863,#49864,#49865,#49866,#49867,#49868,#49869,#49870,
#49871,#49872,#49873,#49874,#49875,#49876,#49877,#49878,#49879,#49880,#49881,
#49882,#49883,#49884,#49885,#49886,#49887,#49888,#49889,#49890,#49891,#49892,
#49893,#49894,#49895,#49896,#49897,#49898,#49899,#49900,#49901,#49902,#49903,
#49904,#49905,#49906,#49907,#49908,#49909,#49910,#49911,#49912,#49913,#49914,
#49915,#49916,#49917,#49918,#49919,#49920,#49921,#49922,#49923,#49924,#49925,
#49926,#49927,#49928,#49929,#49930,#49931,#49932,#49933,#49934,#49935,#49936,
#49937,#49938,#49939,#49940,#49941,#49942,#49943,#49944,#49945,#49946,#49947,
#49948,#49949,#49950,#49951,#49952,#49953,#49954,#49955,#49956,#49957,#49958,
#49959,#49960,#49961,#49962,#49963,#49964,#49965,#49966,#49967,#49968,#49969,
#49970,#49971,#49972,#49973,#49974,#49975,#49976,#49977,#49978,#49979,#49980,
#49981,#49982,#49983,#49984,#49985,#49986,#49987,#49988,#49989,#49990,#49991,
#49992,#49993,#49994,#49995,#49996,#49997,#49998,#49999,#50000,#50001,#50002,
#50003,#50004,#50005,#50006,#50007,#50008,#50009,#50010,#50011,#50012,#50013,
#50014,#50015,#50016,#50017,#50018,#50019,#50020,#50021,#50022,#50023,#50024,
#50025,#50026,#50027,#50028,#50029,#50030,#50031,#50032,#50033,#50034,#50035,
#50036,#50037,#50038,#50039,#50040,#50041,#50042,#50043,#50044,#50045,#50046,
#50047,#50048,#50049,#50050,#50051,#50052,#50053,#50054,#50055,#50056,#50057,
#50058,#50059,#50060,#50061,#50062,#50063,#50064,#50065,#50066,#50067),
 .UNSPECIFIED.,.F.,.F.,(4,2,2,2,2,2,2,2,2,2,2,2,2,2,2,2,2,2,2,2,2,2,2,2,
2,2,2,2,2,2,2,2,2,2,2,2,2,2,2,2,2,2,2,2,2,2,2,2,2,2,2,2,2,2,2,2,2,2,2,2,
2,2,2,2,2,2,2,2,2,2,2,2,2,2,2,2,2,2,2,2,2,2,2,2,2,2,2,2,2,2,2,2,2,2,2,2,
2,2,2,2,2,2,2,2,2,2,2,2,2,2,2,2,2,2,2,2,2,2,2,2,2,2,2,2,2,2,2,2,2,2,2,2,
2,4),(-1.21618442679459,-1.20602901916137,-1.17728167417851,-1.13783240099854,
-1.13309869507937,-1.13013798205412,-1.12781914414893,-1.1252401172321,
-1.12095808040505,-1.10446782140823,-1.04266508258569,-1.03331449682863,
-1.03078585013742,-1.02931869540624,-1.02801511219157,-1.02628232619738,
-1.02244482358703,-1.01718836886191,-1.00324957104713,-0.955506687798199,
-0.937586429586425,-0.933058921434141,-0.930399566244293,-0.928091403480923,
-0.925252352269582,-0.919755475683438,-0.91278238757453,-0.896728103080514,
-0.863506038814794,-0.835538756173074,-0.83234234548286,-0.8307119055099,
-0.829418308326185,-0.827883703775578,-0.825044802242606,-0.808826962190664,
-0.753450396021484,-0.738150714936052,-0.733798986162438,-0.731204503752045,
-0.729120016153655,-0.726298614565452,-0.720886880598065,-0.714049446300602,
-0.698447023878693,-0.660039824643096,-0.636474652985608,-0.633313804152959,
-0.631691031287016,-0.63039793471395,-0.62885730689311,-0.625989828171946,
-0.609071221681158,-0.58027714965765,-0.540804177800965,-0.536070537089696,
-0.533109711905419,-0.530790691707117,-0.528211364776918,-0.523928601172082,
-0.507432541859197,-0.445568323423664,-0.436268722056494,-0.433744828592099,
-0.432278644704489,-0.430974683344121,-0.429239716823355,-0.425390775152348,
-0.395529266777317,-0.344092827437908,-0.337314901950657,-0.334261190319299,
-0.331922060740202,-0.329411963983509,-0.325445430559417,-0.312347012519461,
-0.264606013869831,-0.238419037081571,-0.235227146902527,-0.233597557176833,
-0.232303864908656,-0.232298630006489,-0.232293472873671,-0.23228839252191,
-0.232283387303515,-0.232278456074548,-0.232273597844024,-0.232268811324586,
-0.232264095336892,-0.23225944866851,-0.232254870064762,-0.232250358445751,
-0.232245912749121,-0.232241531906298,-0.232237214942207,-0.232232960853369,
-0.232228654517377,-0.232224361742382,-0.232220082421133,-0.232215816227752,
-0.232211563214092,-0.232207323363667,-0.232203096720666,-0.232198882956517,
-0.232194682048601,-0.232190494181375,-0.232186319252025,-0.232182156831804,
-0.232178007069417,-0.232173869813819,-0.23216974514067,-0.232165632685057,
-0.230598809036455,-0.227597573119974,-0.223698117333866,-0.185933129451229,
-0.146059040181378,-0.138739071096871,-0.135799644110363,-0.133629232272127,
-0.131267223567011,-0.128023401909181,-0.12034931857652,-0.0993266993999184,
-0.0816547681768319,-0.0627343545680858,-0.0393728063109915,-0.0362144430830506,
-0.0345920434080208,-0.0332987611035165,-0.0320681220626925,-0.0305437290303957,
-0.0282358676238496,-0.00058235440496028),.UNSPECIFIED.);
#588=B_SPLINE_CURVE_WITH_KNOTS('',3,(#50068,#50069,#50070,#50071),
 .UNSPECIFIED.,.F.,.F.,(4,4),(-2.51480909694823,-2.47379053097235),
 .UNSPECIFIED.);
#589=B_SPLINE_CURVE_WITH_KNOTS('',3,(#50072,#50073,#50074,#50075,#50076,
#50077,#50078,#50079,#50080,#50081,#50082,#50083,#50084,#50085,#50086,#50087,
#50088,#50089,#50090,#50091,#50092,#50093,#50094,#50095,#50096,#50097,#50098,
#50099,#50100,#50101,#50102,#50103,#50104,#50105,#50106,#50107,#50108,#50109,
#50110,#50111,#50112,#50113,#50114,#50115,#50116,#50117,#50118,#50119,#50120,
#50121,#50122,#50123,#50124,#50125,#50126,#50127,#50128,#50129,#50130,#50131,
#50132,#50133,#50134,#50135,#50136,#50137,#50138,#50139,#50140,#50141,#50142,
#50143,#50144,#50145,#50146,#50147,#50148,#50149,#50150,#50151,#50152,#50153,
#50154,#50155,#50156,#50157,#50158,#50159,#50160,#50161,#50162,#50163,#50164,
#50165,#50166,#50167,#50168,#50169,#50170,#50171,#50172,#50173,#50174,#50175,
#50176,#50177,#50178,#50179,#50180,#50181,#50182,#50183,#50184,#50185,#50186,
#50187,#50188,#50189,#50190,#50191,#50192,#50193,#50194,#50195,#50196,#50197,
#50198,#50199,#50200,#50201,#50202,#50203,#50204,#50205,#50206,#50207,#50208,
#50209,#50210,#50211,#50212,#50213,#50214,#50215,#50216,#50217,#50218,#50219,
#50220,#50221,#50222,#50223,#50224,#50225,#50226,#50227,#50228,#50229,#50230,
#50231,#50232,#50233,#50234,#50235,#50236,#50237,#50238,#50239,#50240,#50241,
#50242,#50243,#50244,#50245,#50246,#50247,#50248,#50249,#50250,#50251,#50252,
#50253,#50254,#50255,#50256,#50257,#50258,#50259,#50260,#50261,#50262,#50263,
#50264,#50265,#50266,#50267,#50268,#50269,#50270,#50271,#50272,#50273,#50274,
#50275,#50276,#50277,#50278,#50279,#50280,#50281,#50282,#50283,#50284,#50285,
#50286,#50287,#50288,#50289,#50290,#50291,#50292,#50293,#50294,#50295,#50296,
#50297),.UNSPECIFIED.,.F.,.F.,(4,2,2,2,2,2,2,2,2,2,2,2,2,2,2,2,2,2,2,2,
2,2,2,2,2,2,2,2,2,2,2,2,2,2,2,2,2,2,2,2,2,2,2,2,2,2,2,2,2,2,2,2,2,2,2,2,
2,2,2,2,2,2,2,2,2,2,2,2,2,2,2,2,2,2,2,2,2,2,2,2,2,2,2,2,2,2,2,2,2,2,2,2,
2,2,2,2,2,2,2,2,2,2,2,2,2,2,2,2,2,2,2,2,4),(-1.298038620556,-1.28518477492575,
-1.26659110951169,-1.26214889648848,-1.25953479674532,-1.25722221376322,
-1.25432025570229,-1.2485099737604,-1.24103059169013,-1.22323486762303,
-1.18182496135094,-1.17836580391313,-1.16422782172899,-1.16163208277177,
-1.15999681531125,-1.15870319260542,-1.15717303208584,-1.15435395906807,
-1.13858350023123,-1.08807524478368,-1.06815460073119,-1.06348447848502,
-1.06079298808077,-1.05850962691057,-1.05572198480439,-1.05047134461615,
-1.00668118447764,-1.00437172518463,-0.968198674133801,-0.963441883720382,
-0.961498094337659,-0.960172118688768,-0.958791618565002,-0.956653204195387,
-0.950090216242167,-0.939316412722717,-0.88598819475271,-0.868801014420672,
-0.864330576459267,-0.861684811153804,-0.859376203650546,-0.856520858579278,
-0.850941559411361,-0.812451150535233,-0.768542688842383,-0.764269501946701,
-0.762589470364484,-0.761371760340662,-0.760032159631958,-0.758086834263315,
-0.752961332050261,-0.745276149825901,-0.719682632012063,-0.674275634441559,
-0.667131684008038,-0.664217292874704,-0.66205362633767,-0.659687520292765,
-0.656417099670902,-0.648578626422449,-0.63759289911443,-0.573788637756297,
-0.566240713939279,-0.563903430862806,-0.562478766745775,-0.561161553900476,
-0.559338013177925,-0.554983019012877,-0.53422835773226,-0.509010619116768,
-0.472134220389905,-0.467372634548957,-0.464403311419755,-0.462083160494708,
-0.459508245663754,-0.455246081259015,-0.439001343358237,-0.407501199655168,
-0.371216127374185,-0.366452132230693,-0.364506867544745,-0.363180376456594,
-0.361799824160692,-0.359662169040866,-0.353108098743345,-0.342355806521128,
-0.289398155463731,-0.271840828526119,-0.267340865108757,-0.264687930608783,
-0.262379378787629,-0.259532212314096,-0.253995100933304,-0.246957478626795,
-0.23068548910416,-0.180067527739042,-0.168886447477057,-0.166232598349115,
-0.164722109847122,-0.163426175483797,-0.162162938960683,-0.159612812438825,
-0.146885778986395,-0.117779555395451,-0.0774601860868628,-0.0742590008540955,
-0.0694234780118543,-0.0664319935225179,-0.0641090963614894,-0.0615459281247616,
-0.0573373953712801,-0.0523476908568135,-0.0416325986123643),
 .UNSPECIFIED.);
#590=B_SPLINE_CURVE_WITH_KNOTS('',3,(#50302,#50303,#50304,#50305,#50306,
#50307,#50308,#50309,#50310,#50311,#50312,#50313,#50314,#50315,#50316,#50317,
#50318,#50319,#50320,#50321,#50322,#50323,#50324,#50325,#50326,#50327,#50328,
#50329,#50330,#50331,#50332,#50333,#50334,#50335,#50336,#50337,#50338,#50339,
#50340,#50341,#50342,#50343,#50344,#50345,#50346,#50347,#50348,#50349,#50350,
#50351,#50352,#50353,#50354,#50355,#50356,#50357,#50358,#50359,#50360,#50361,
#50362,#50363,#50364,#50365,#50366,#50367,#50368,#50369,#50370,#50371,#50372,
#50373,#50374,#50375,#50376,#50377,#50378,#50379,#50380,#50381,#50382,#50383,
#50384,#50385,#50386,#50387,#50388,#50389,#50390,#50391,#50392,#50393,#50394,
#50395,#50396,#50397,#50398,#50399,#50400,#50401,#50402,#50403,#50404,#50405,
#50406,#50407,#50408,#50409,#50410,#50411,#50412,#50413,#50414,#50415,#50416,
#50417,#50418,#50419,#50420,#50421,#50422,#50423,#50424,#50425,#50426,#50427,
#50428,#50429,#50430,#50431,#50432,#50433,#50434,#50435,#50436,#50437,#50438,
#50439,#50440,#50441,#50442,#50443,#50444,#50445,#50446,#50447,#50448,#50449,
#50450,#50451,#50452,#50453,#50454,#50455,#50456,#50457,#50458,#50459,#50460,
#50461,#50462,#50463,#50464,#50465,#50466,#50467,#50468,#50469,#50470,#50471,
#50472,#50473,#50474,#50475,#50476,#50477,#50478,#50479,#50480,#50481,#50482,
#50483,#50484,#50485,#50486,#50487,#50488,#50489,#50490,#50491,#50492,#50493,
#50494,#50495,#50496,#50497,#50498,#50499,#50500,#50501,#50502,#50503,#50504,
#50505,#50506,#50507,#50508,#50509,#50510,#50511,#50512,#50513,#50514,#50515,
#50516,#50517,#50518,#50519,#50520,#50521,#50522,#50523,#50524,#50525,#50526,
#50527,#50528,#50529,#50530,#50531,#50532,#50533),.UNSPECIFIED.,.F.,.F.,
(4,2,2,2,2,2,2,2,2,2,2,2,2,2,2,2,2,2,2,2,2,2,2,2,2,2,2,2,2,2,2,2,2,2,2,
2,2,2,2,2,2,2,2,2,2,2,2,2,2,2,2,2,2,2,2,2,2,2,2,2,2,2,2,2,2,2,2,2,2,2,2,
2,2,2,2,2,2,2,2,2,2,2,2,2,2,2,2,2,2,2,2,2,2,2,2,2,2,2,2,2,2,2,2,2,2,2,2,
2,2,2,2,2,2,2,2,4),(-2.47226785878759,-2.44315262999097,-2.4265493773509,
-2.42369517961594,-2.4221576717896,-2.42086481042697,-2.41923932921738,
-2.41606445023606,-2.39136211892146,-2.34495212060522,-2.32954671256529,
-2.32646922213363,-2.32372673233149,-2.32368173597199,-2.32363591157625,
-2.32358917750693,-2.32354144531909,-2.32349261869542,-2.32138662359374,
-2.31878608606322,-2.31458483610215,-2.29992789744491,-2.24972977461377,
-2.23484724352276,-2.22935852650405,-2.22539113236106,-2.22363522959312,
-2.22232891709944,-2.22087470883029,-2.21840303053684,-2.20962256755983,
-2.14725270028537,-2.13072560853464,-2.12644158137443,-2.12386266129053,
-2.12154474615733,-2.11858635123024,-2.11385861866163,-2.07437290301597,
-2.0455643345363,-2.0286571824889,-2.02579096297739,-2.02425098809859,-2.02295842092606,
-2.02133629634428,-2.01817666430633,-1.99459470257733,-1.95619068143742,
-1.94064592648934,-1.93382638990624,-1.92842599729637,-1.92560760865676,
-1.9235241398696,-1.92092938379755,-1.91657348357221,-1.9012135598243,-1.84589992968617,
-1.82968748645245,-1.8268494962571,-1.82531542242399,-1.82402229010215,
-1.82239246683785,-1.81919735475115,-1.78964838535882,-1.75122451981294,
-1.73313848852572,-1.72873323226305,-1.72612743795481,-1.72381393800529,
-1.72089977282247,-1.71631928020207,-1.68950850830298,-1.6456623496029,
-1.63067487493781,-1.62789183078225,-1.62636949052947,-1.62507531930725,
-1.62343020791712,-1.62080168706969,-1.60599736991801,-1.6016956259522,
-1.58936041687335,-1.5573174904848,-1.54240876289479,-1.53578261411349,
-1.53050406740892,-1.52771061083931,-1.52562929209383,-1.52301601410596,
-1.51857725781707,-1.50234770938831,-1.44796322564263,-1.43712141379915,
-1.43052934755061,-1.42838731951397,-1.42700597246057,-1.42568044721729,
-1.42373928147752,-1.41899866957122,-1.38237238157978,-1.35114408966658,
-1.33498087006502,-1.33072601837987,-1.32815295531946,-1.32583283076147,
-1.32286126356138,-1.31809138604049,-1.28162623786546,-1.25685729748551,
-1.23348909408972,-1.23033134675811,-1.22870931924426,-1.22741636345724,
-1.22587536583413,-1.2230057744408,-1.21618442679459),.UNSPECIFIED.);
#591=B_SPLINE_CURVE_WITH_KNOTS('',3,(#50535,#50536,#50537,#50538),
 .UNSPECIFIED.,.F.,.F.,(4,4),(-0.0416325986123643,-0.00058313060358834),
 .UNSPECIFIED.);
#592=B_SPLINE_CURVE_WITH_KNOTS('',3,(#50539,#50540,#50541,#50542,#50543,
#50544,#50545,#50546,#50547,#50548,#50549,#50550,#50551,#50552,#50553,#50554,
#50555,#50556,#50557,#50558,#50559,#50560,#50561,#50562,#50563,#50564,#50565,
#50566,#50567,#50568,#50569,#50570,#50571,#50572,#50573,#50574,#50575,#50576,
#50577,#50578,#50579,#50580,#50581,#50582,#50583,#50584,#50585,#50586,#50587,
#50588,#50589,#50590,#50591,#50592,#50593,#50594,#50595,#50596,#50597,#50598,
#50599,#50600,#50601,#50602,#50603,#50604,#50605,#50606,#50607,#50608,#50609,
#50610,#50611,#50612,#50613,#50614,#50615,#50616,#50617,#50618,#50619,#50620,
#50621,#50622,#50623,#50624,#50625,#50626,#50627,#50628,#50629,#50630,#50631,
#50632,#50633,#50634,#50635,#50636,#50637,#50638,#50639,#50640,#50641,#50642,
#50643,#50644,#50645,#50646,#50647,#50648,#50649,#50650,#50651,#50652,#50653,
#50654,#50655,#50656,#50657,#50658,#50659,#50660,#50661,#50662,#50663,#50664,
#50665,#50666,#50667,#50668,#50669,#50670,#50671,#50672,#50673,#50674,#50675,
#50676,#50677,#50678,#50679,#50680,#50681,#50682,#50683,#50684,#50685,#50686,
#50687,#50688,#50689,#50690,#50691,#50692,#50693,#50694,#50695,#50696,#50697,
#50698,#50699,#50700,#50701,#50702,#50703,#50704,#50705,#50706,#50707,#50708,
#50709,#50710,#50711,#50712,#50713,#50714,#50715,#50716,#50717,#50718,#50719,
#50720,#50721,#50722,#50723,#50724,#50725,#50726,#50727,#50728,#50729,#50730,
#50731,#50732,#50733,#50734,#50735,#50736,#50737,#50738,#50739,#50740,#50741,
#50742,#50743,#50744,#50745,#50746,#50747,#50748,#50749,#50750,#50751,#50752,
#50753,#50754,#50755,#50756,#50757,#50758,#50759,#50760,#50761,#50762,#50763,
#50764,#50765,#50766,#50767,#50768,#50769,#50770,#50771,#50772,#50773,#50774,
#50775,#50776,#50777,#50778,#50779,#50780,#50781,#50782,#50783,#50784,#50785,
#50786,#50787,#50788,#50789,#50790,#50791,#50792,#50793,#50794,#50795,#50796,
#50797,#50798,#50799,#50800),.UNSPECIFIED.,.F.,.F.,(4,2,2,2,2,2,2,2,2,2,
2,2,2,2,2,2,2,2,2,2,2,2,2,2,2,2,2,2,2,2,2,2,2,2,2,2,2,2,2,2,2,2,2,2,2,2,
2,2,2,2,2,2,2,2,2,2,2,2,2,2,2,2,2,2,2,2,2,2,2,2,2,2,2,2,2,2,2,2,2,2,2,2,
2,2,2,2,2,2,2,2,2,2,2,2,2,2,2,2,2,2,2,2,2,2,2,2,2,2,2,2,2,2,2,2,2,2,2,2,
2,2,2,2,2,2,2,2,2,2,2,2,4),(-2.51400264948435,-2.48421836071445,-2.48192163669727,
-2.48040181517654,-2.47917229137992,-2.47787865972753,-2.47625012840667,
-2.47306319379138,-2.44741318866998,-2.42529602530809,-2.40088110763266,
-2.38642684357947,-2.38230233158867,-2.37975744191638,-2.37742943659178,
-2.37445087829526,-2.36955085144401,-2.36646446508994,-2.32614418677038,
-2.28874616452835,-2.28486187851215,-2.28187238973397,-2.28030678901279,
-2.28030267401512,-2.2802985464738,-2.28029440633816,-2.28029025383883,
-2.28028608858994,-2.28028191080908,-2.28027771999208,-2.28027351615463,
-2.28026929938522,-2.28026506959409,-2.28026082671353,-2.28025657058589,
-2.28025230108468,-2.28024801814176,-2.28024372186064,-2.2802394120175,
-2.28023513939178,-2.28023080342924,-2.28022640299119,-2.28022193709567,
-2.2802174049142,-2.28021280536375,-2.28020813695118,-2.28020339868081,
-2.28019858944706,-2.28019370816035,-2.28018875346816,-2.2801837239967,
-2.27889021515564,-2.2772669983009,-2.27410549855148,-2.24256840317327,
-2.22909775646131,-2.19000465811213,-2.18440338265633,-2.18154262245319,
-2.17923245949173,-2.17658800594296,-2.17212717701184,-2.15510854333331,
-2.10627900681833,-2.09233449351235,-2.08707633689177,-2.08323790214284,
-2.08150466404738,-2.08020073617748,-2.07873317016305,-2.0762037903952,
-2.06684996307841,-2.00505911035982,-1.98856852355242,-1.98428554311218,
-1.98170576625952,-1.97938613691062,-1.97642425226807,-1.9716883033089,
-1.93219771653853,-1.90339715313762,-1.88644220837923,-1.88357263561294,
-1.88203132944743,-1.88073792230771,-1.87911509336461,-1.87595510449785,
-1.85285401555903,-1.82068547130729,-1.79355103555675,-1.78687294651153,
-1.78380395321282,-1.78147025418424,-1.77894362239403,-1.77490255597318,
-1.7624480762994,-1.70991782953796,-1.68961524574869,-1.68530747157291,
-1.68349158038617,-1.68217534868089,-1.68074693338009,-1.67839399384082,
-1.67071536034148,-1.61287886515058,-1.59112116830058,-1.58647611847225,
-1.58381703823214,-1.58150843128679,-1.57866796227263,-1.57433128493264,
-1.55313559585049,-1.50385364861007,-1.4933504819802,-1.48901191318128,
-1.48570798427628,-1.48407701440211,-1.48290724750031,-1.48142219231935,
-1.47887988230922,-1.46906552985234,-1.40777556394142,-1.39132554786916,
-1.38704608146942,-1.3844671771677,-1.38214754171373,-1.37918455818483,
-1.37444463789547,-1.33513412792569,-1.30671152878061,-1.2981223786512),
 .UNSPECIFIED.);
#593=B_SPLINE_CURVE_WITH_KNOTS('',3,(#50806,#50807,#50808,#50809,#50810,
#50811,#50812,#50813,#50814,#50815,#50816,#50817,#50818,#50819,#50820,#50821,
#50822,#50823,#50824,#50825,#50826,#50827,#50828,#50829,#50830,#50831,#50832,
#50833,#50834,#50835,#50836,#50837,#50838,#50839,#50840,#50841,#50842,#50843,
#50844,#50845,#50846,#50847,#50848,#50849,#50850,#50851,#50852,#50853,#50854,
#50855,#50856,#50857,#50858,#50859,#50860,#50861,#50862,#50863,#50864,#50865,
#50866,#50867,#50868,#50869,#50870,#50871,#50872,#50873,#50874,#50875,#50876,
#50877,#50878,#50879,#50880,#50881,#50882,#50883,#50884,#50885,#50886,#50887,
#50888,#50889,#50890,#50891,#50892,#50893,#50894,#50895,#50896,#50897,#50898,
#50899,#50900,#50901,#50902,#50903,#50904,#50905,#50906,#50907,#50908,#50909,
#50910,#50911,#50912,#50913,#50914,#50915,#50916,#50917,#50918,#50919,#50920,
#50921,#50922,#50923,#50924,#50925,#50926,#50927,#50928,#50929,#50930,#50931,
#50932,#50933,#50934,#50935,#50936,#50937,#50938,#50939,#50940,#50941,#50942,
#50943,#50944,#50945,#50946,#50947,#50948,#50949,#50950,#50951,#50952,#50953,
#50954,#50955,#50956,#50957,#50958,#50959,#50960,#50961,#50962,#50963,#50964,
#50965,#50966,#50967,#50968,#50969,#50970,#50971,#50972,#50973,#50974,#50975,
#50976,#50977,#50978,#50979,#50980,#50981,#50982,#50983,#50984,#50985,#50986,
#50987,#50988,#50989,#50990,#50991,#50992,#50993,#50994,#50995,#50996,#50997,
#50998,#50999,#51000,#51001,#51002,#51003,#51004,#51005,#51006,#51007,#51008,
#51009,#51010,#51011,#51012,#51013,#51014,#51015,#51016,#51017,#51018,#51019,
#51020,#51021,#51022,#51023,#51024,#51025),.UNSPECIFIED.,.F.,.F.,(4,2,2,
2,2,2,2,2,2,2,2,2,2,2,2,2,2,2,2,2,2,2,2,2,2,2,2,2,2,2,2,2,2,2,2,2,2,2,2,
2,2,2,2,2,2,2,2,2,2,2,2,2,2,2,2,2,2,2,2,2,2,2,2,2,2,2,2,2,2,2,2,2,2,2,2,
2,2,2,2,2,2,2,2,2,2,2,2,2,2,2,2,2,2,2,2,2,2,2,2,2,2,2,2,2,2,2,2,2,2,4),
(-1.21660469756962,-1.21560513177792,-1.20832163108235,-1.20538563640586,
-1.2032160417423,-1.20085326046503,-1.19760535281686,-1.18990717030479,
-1.17917873754424,-1.147696759036,-1.11135820733462,-1.10660537746665,-1.1046617879558,
-1.1033354744309,-1.10195415414047,-1.09981365600362,-1.0932378797993,-1.0824363957164,
-1.02870806498096,-1.01187539626733,-1.00737826174651,-1.00475158765139,
-1.00246182527359,-0.999587416253969,-0.993917377552048,-0.95259563762134,
-0.912034853681237,-0.907470599208752,-0.905746551472394,-0.904516967928173,
-0.903186986538914,-0.901293145058762,-0.896507014298174,-0.889492369840031,
-0.867582639851953,-0.816632155793302,-0.80979793441561,-0.806734035387213,
-0.804393177932454,-0.801887137747357,-0.797939543990976,-0.785020376258243,
-0.763140183789312,-0.733722921882351,-0.727883598997912,-0.724268933398251,
-0.710320822671981,-0.707734310524198,-0.706101580902123,-0.704807746316235,
-0.703274720763992,-0.700443584799953,-0.684411747932148,-0.631217593331959,
-0.61388102336528,-0.609397841651758,-0.606748631557248,-0.60443953544755,
-0.601586828982065,-0.596023203713855,-0.55804042668657,-0.515496433565771,
-0.509809636449915,-0.507718001094443,-0.50648372969871,-0.505157492075355,
-0.503283384681019,-0.498621099075318,-0.474793280554394,-0.453883256124921,
-0.416142165685547,-0.411406773649788,-0.408445143824071,-0.406125672957546,
-0.403546029663099,-0.399263175365165,-0.382772470098717,-0.32100364952033,
-0.31160406007368,-0.30907029991932,-0.307601774890138,-0.306298078656024,
-0.304566633046494,-0.30073794472848,-0.295497469601035,-0.281624077645052,
-0.234094897535137,-0.215890789942289,-0.211336251199948,-0.208670270878735,
-0.206407968288284,-0.203850973880011,-0.200965344285523,-0.196470140986856,
-0.170933518498077,-0.13529488257053,-0.113675948221446,-0.110532110167491,
-0.108912655120551,-0.107619292972448,-0.106074890376176,-0.103191184303473,
-0.0858759175043473,-0.0250529057732762,-0.0150319442351391,-0.0113202422794324,
-0.00911053038409564,-0.0068859470510532,-0.00461814312859361,-0.000582527892639659),
 .UNSPECIFIED.);
#594=B_SPLINE_CURVE_WITH_KNOTS('',3,(#51026,#51027,#51028,#51029,#51030,
#51031,#51032,#51033),.UNSPECIFIED.,.F.,.F.,(4,2,2,4),(-2.51302961979646,
-2.50312569535042,-2.47230189720855,-2.47226785878759),.UNSPECIFIED.);
#595=B_SPLINE_CURVE_WITH_KNOTS('',3,(#51034,#51035,#51036,#51037,#51038,
#51039,#51040,#51041,#51042,#51043,#51044,#51045,#51046,#51047,#51048,#51049,
#51050,#51051,#51052,#51053,#51054,#51055,#51056,#51057,#51058,#51059,#51060,
#51061,#51062,#51063,#51064,#51065,#51066,#51067,#51068,#51069,#51070,#51071,
#51072,#51073,#51074,#51075,#51076,#51077,#51078,#51079,#51080,#51081,#51082,
#51083,#51084,#51085,#51086,#51087,#51088,#51089,#51090,#51091,#51092,#51093,
#51094,#51095,#51096,#51097,#51098,#51099,#51100,#51101,#51102,#51103,#51104,
#51105,#51106,#51107,#51108,#51109,#51110,#51111,#51112,#51113,#51114,#51115,
#51116,#51117,#51118,#51119,#51120,#51121,#51122,#51123,#51124,#51125,#51126,
#51127,#51128,#51129,#51130,#51131,#51132,#51133,#51134,#51135,#51136,#51137,
#51138,#51139,#51140,#51141,#51142,#51143,#51144,#51145,#51146,#51147,#51148,
#51149,#51150,#51151,#51152,#51153,#51154,#51155,#51156,#51157,#51158,#51159,
#51160,#51161,#51162,#51163,#51164,#51165,#51166,#51167,#51168,#51169,#51170,
#51171,#51172,#51173,#51174,#51175,#51176,#51177,#51178,#51179,#51180,#51181,
#51182,#51183,#51184,#51185,#51186,#51187,#51188,#51189,#51190,#51191,#51192,
#51193,#51194,#51195,#51196,#51197,#51198,#51199,#51200,#51201,#51202,#51203,
#51204,#51205,#51206,#51207,#51208,#51209,#51210,#51211,#51212,#51213,#51214,
#51215,#51216,#51217,#51218,#51219,#51220,#51221,#51222,#51223,#51224,#51225,
#51226,#51227,#51228,#51229,#51230,#51231,#51232,#51233,#51234,#51235,#51236,
#51237,#51238,#51239,#51240,#51241,#51242,#51243,#51244,#51245,#51246,#51247,
#51248,#51249,#51250,#51251,#51252,#51253,#51254,#51255,#51256,#51257,#51258,
#51259,#51260,#51261,#51262,#51263,#51264,#51265,#51266,#51267,#51268,#51269,
#51270,#51271,#51272,#51273,#51274,#51275,#51276,#51277,#51278,#51279),
 .UNSPECIFIED.,.F.,.F.,(4,2,2,2,2,2,2,2,2,2,2,2,2,2,2,2,2,2,2,2,2,2,2,2,
2,2,2,2,2,2,2,2,2,2,2,2,2,2,2,2,2,2,2,2,2,2,2,2,2,2,2,2,2,2,2,2,2,2,2,2,
2,2,2,2,2,2,2,2,2,2,2,2,2,2,2,2,2,2,2,2,2,2,2,2,2,2,2,2,2,2,2,2,2,2,2,2,
2,2,2,2,2,2,2,2,2,2,2,2,2,2,2,2,2,2,2,2,2,2,2,2,2,2,4),(-1.2981223786512,
-1.2892459881527,-1.2863568195862,-1.28481140686892,-1.28351831515963,-1.28190060790969,
-1.27876421797423,-1.2574525993154,-1.20862501435937,-1.19257426809608,
-1.18815147564813,-1.185541125541,-1.18345857202648,-1.18065884250332,-1.17535303922238,
-1.13132657066651,-1.11873435243647,-1.09078747636709,-1.08759075686629,
-1.08596016618755,-1.08466645304877,-1.08313171527733,-1.08029257868359,
-1.06407373543308,-1.00869780993439,-0.993391491732283,-0.989038921728858,
-0.986444107872633,-0.98435944952,-0.981537942179059,-0.976126435237369,
-0.969289520945197,-0.95368945582181,-0.915268874499263,-0.891705299202744,
-0.888544219078316,-0.886921312012993,-0.885628100256878,-0.884087325497926,
-0.881219547656855,-0.864298360366526,-0.835502470743149,-0.796026287637618,
-0.791292213826143,-0.788331120784207,-0.786011892691552,-0.783432336506779,
-0.779149196934187,-0.762651752870428,-0.700783273382089,-0.691481607473425,
-0.688957369455633,-0.687491028149465,-0.68618695650777,-0.684451883529049,
-0.680602864638799,-0.651467332720191,-0.599132316921038,-0.592462231962627,
-0.589427857296861,-0.587091611470286,-0.584572872022557,-0.580567474829767,
-0.567097949324753,-0.519537403066136,-0.493609003853499,-0.490418963370928,
-0.488789688590706,-0.487495913237913,-0.485959795333883,-0.483114689260777,
-0.466759911375288,-0.409651956494921,-0.395893709953167,-0.391703266766024,
-0.389143953734435,-0.386819895074774,-0.38382035859433,-0.37751241408995,
-0.353226022170356,-0.312599495962939,-0.308832167592656,-0.2940459943494,
-0.291411380084304,-0.289764071049895,-0.288469238850304,-0.28694735713961,
-0.284168303378318,-0.269281203640925,-0.226186761564817,-0.198573150191097,
-0.193962823065936,-0.191038905908958,-0.188778399240402,-0.188684497229446,
-0.188608927082289,-0.188547336342364,-0.188496637954795,-0.188454572900009,
-0.188419445739269,-0.188389957202828,-0.188337538842759,-0.188286914050502,
-0.188237938368303,-0.188190481228795,-0.18814442419915,-0.188099659591416,
-0.188056089114478,-0.188013622782854,-0.187972178006164,-0.185170242457677,
-0.182083928901597,-0.177103198736196,-0.16718128626347,-0.120765531311188,
-0.0955142687044764,-0.0923311215095132,-0.0907033688591454,-0.0894097423535389,
-0.0878725484329314,-0.0850221642633632,-0.0685376748017855,-0.0413768992123694),
 .UNSPECIFIED.);
#596=B_SPLINE_CURVE_WITH_KNOTS('',3,(#51284,#51285,#51286,#51287,#51288,
#51289,#51290,#51291,#51292,#51293,#51294,#51295,#51296,#51297,#51298,#51299,
#51300,#51301,#51302,#51303,#51304,#51305,#51306,#51307,#51308,#51309,#51310,
#51311,#51312,#51313,#51314,#51315,#51316,#51317,#51318,#51319,#51320,#51321,
#51322,#51323,#51324,#51325,#51326,#51327,#51328,#51329,#51330,#51331,#51332,
#51333,#51334,#51335,#51336,#51337,#51338,#51339,#51340,#51341,#51342,#51343,
#51344,#51345,#51346,#51347,#51348,#51349,#51350,#51351,#51352,#51353,#51354,
#51355,#51356,#51357,#51358,#51359,#51360,#51361,#51362,#51363,#51364,#51365,
#51366,#51367,#51368,#51369,#51370,#51371,#51372,#51373,#51374,#51375,#51376,
#51377,#51378,#51379,#51380,#51381,#51382,#51383,#51384,#51385,#51386,#51387,
#51388,#51389,#51390,#51391,#51392,#51393,#51394,#51395,#51396,#51397,#51398,
#51399,#51400,#51401,#51402,#51403,#51404,#51405,#51406,#51407,#51408,#51409,
#51410,#51411,#51412,#51413,#51414,#51415,#51416,#51417,#51418,#51419,#51420,
#51421,#51422,#51423,#51424,#51425,#51426,#51427,#51428,#51429,#51430,#51431,
#51432,#51433,#51434,#51435,#51436,#51437,#51438,#51439,#51440,#51441,#51442,
#51443,#51444,#51445,#51446,#51447,#51448,#51449,#51450,#51451,#51452,#51453,
#51454,#51455,#51456,#51457,#51458,#51459,#51460,#51461,#51462,#51463,#51464,
#51465,#51466,#51467,#51468,#51469,#51470,#51471,#51472,#51473,#51474,#51475,
#51476,#51477,#51478,#51479,#51480,#51481,#51482,#51483,#51484,#51485,#51486,
#51487),.UNSPECIFIED.,.F.,.F.,(4,2,2,2,2,2,2,2,2,2,2,2,2,2,2,2,2,2,2,2,
2,2,2,2,2,2,2,2,2,2,2,2,2,2,2,2,2,2,2,2,2,2,2,2,2,2,2,2,2,2,2,2,2,2,2,2,
2,2,2,2,2,2,2,2,2,2,2,2,2,2,2,2,2,2,2,2,2,2,2,2,2,2,2,2,2,2,2,2,2,2,2,2,
2,2,2,2,2,2,2,2,2,4),(-2.47330243401613,-2.42245091809077,-2.40486508519416,
-2.40049612610248,-2.39789774407745,-2.39558210310781,-2.39265347595769,
-2.38802695167722,-2.35979244577488,-2.30812033644537,-2.30351601419034,
-2.30108490173506,-2.29902432207317,-2.29767158938404,-2.29634483716351,
-2.2943986594292,-2.28962973924138,-2.25379289806888,-2.22199101529607,
-2.2056553257859,-2.20138531570239,-2.19880849348897,-2.19648842755216,
-2.19352170992676,-2.18876934135159,-2.15384875722703,-2.12912419348526,
-2.1061643608833,-2.10158618358893,-2.09972563089072,-2.09840185315068,
-2.09699096812524,-2.09471618273464,-2.087685359805,-2.02912550058502,-2.0147172656301,
-2.00510401090219,-2.00156268898467,-1.99914346871885,-1.99677963687774,
-1.99392760018832,-1.98698233139921,-1.9379740026273,-1.90603539007453,
-1.90219087256393,-1.90045679003201,-1.89915303213149,-1.89768654845573,
-1.89516100085917,-1.88584271509496,-1.82403207922562,-1.80754299005997,
-1.80326089516825,-1.80068173939704,-1.79836272417135,-1.79540170044825,
-1.7906672836817,-1.75117477108976,-1.72235506387672,-1.70544042188533,
-1.70257301873896,-1.70103241645799,-1.69973932772334,-1.6981165549582,
-1.69495567882391,-1.67136645436436,-1.6329670902671,-1.61740218266273,
-1.61057570165538,-1.6051704929249,-1.60235042224918,-1.6002660540789,-1.59767062009864,
-1.59331464426795,-1.57796748675147,-1.52261106371159,-1.50639040547052,
-1.50355119815981,-1.50201648948937,-1.5007228358218,-1.49909237293609,
-1.49589605837859,-1.46861168488881,-1.43317733018402,-1.41809223435838,
-1.41141130619422,-1.4060977246328,-1.40329640277701,-1.40121371354766,
-1.39860456922296,-1.39418717582083,-1.37819303451522,-1.32352925888638,
-1.31266838404468,-1.30606740809001,-1.30392384900638,-1.30254185730772,
-1.30121600648613,-1.29927481619259,-1.29453640384491,-1.25762792083579,
-1.21660469756962),.UNSPECIFIED.);
#597=B_SPLINE_CURVE_WITH_KNOTS('',3,(#51489,#51490,#51491,#51492,#51493,
#51494),.UNSPECIFIED.,.F.,.F.,(4,2,4),(-0.0413768992123694,-0.0396266779595947,
-0.000583049282567826),.UNSPECIFIED.);
#598=B_SPLINE_CURVE_WITH_KNOTS('',3,(#51495,#51496,#51497,#51498,#51499,
#51500,#51501,#51502,#51503,#51504,#51505,#51506,#51507,#51508,#51509,#51510,
#51511,#51512,#51513,#51514,#51515,#51516,#51517,#51518,#51519,#51520,#51521,
#51522,#51523,#51524,#51525,#51526,#51527,#51528,#51529,#51530,#51531,#51532,
#51533,#51534,#51535,#51536,#51537,#51538,#51539,#51540,#51541,#51542,#51543,
#51544,#51545,#51546,#51547,#51548,#51549,#51550,#51551,#51552,#51553,#51554,
#51555,#51556,#51557,#51558,#51559,#51560,#51561,#51562,#51563,#51564,#51565,
#51566,#51567,#51568,#51569,#51570,#51571,#51572,#51573,#51574,#51575,#51576,
#51577,#51578,#51579,#51580,#51581,#51582,#51583,#51584,#51585,#51586,#51587,
#51588,#51589,#51590,#51591,#51592,#51593,#51594,#51595,#51596,#51597,#51598,
#51599,#51600,#51601,#51602,#51603,#51604,#51605,#51606,#51607,#51608,#51609,
#51610,#51611,#51612,#51613,#51614,#51615,#51616,#51617,#51618,#51619,#51620,
#51621,#51622,#51623,#51624,#51625,#51626,#51627,#51628,#51629,#51630,#51631,
#51632,#51633,#51634,#51635,#51636,#51637,#51638,#51639,#51640,#51641,#51642,
#51643,#51644,#51645,#51646,#51647,#51648,#51649,#51650,#51651,#51652,#51653,
#51654,#51655,#51656,#51657,#51658,#51659,#51660,#51661,#51662,#51663,#51664,
#51665,#51666,#51667,#51668,#51669,#51670,#51671,#51672,#51673,#51674,#51675,
#51676,#51677,#51678,#51679,#51680,#51681,#51682,#51683,#51684,#51685,#51686,
#51687,#51688,#51689,#51690,#51691,#51692,#51693,#51694,#51695,#51696,#51697,
#51698,#51699,#51700,#51701,#51702,#51703,#51704,#51705,#51706,#51707,#51708,
#51709,#51710,#51711,#51712),.UNSPECIFIED.,.F.,.F.,(4,2,2,2,2,2,2,2,2,2,
2,2,2,2,2,2,2,2,2,2,2,2,2,2,2,2,2,2,2,2,2,2,2,2,2,2,2,2,2,2,2,2,2,2,2,2,
2,2,2,2,2,2,2,2,2,2,2,2,2,2,2,2,2,2,2,2,2,2,2,2,2,2,2,2,2,2,2,2,2,2,2,2,
2,2,2,2,2,2,2,2,2,2,2,2,2,2,2,2,2,2,2,2,2,2,2,2,2,2,4),(-2.51327713688667,
-2.51013830636087,-2.50709747201508,-2.50484278771018,-2.50260877932776,
-2.50038437760381,-2.4965899563431,-2.48597608443706,-2.42540070554653,
-2.40862072766969,-2.40575971115735,-2.4042208962479,-2.402928336082,-2.40130500076025,
-2.39813946372172,-2.37411751586636,-2.33645917876175,-2.32073492763113,
-2.31386141821673,-2.31001529286203,-2.30739913737221,-2.30489807320466,
-2.30264335814387,-2.29968183354299,-2.29494350057941,-2.25551157182444,
-2.22729377002798,-2.20980399058925,-2.20691533209874,-2.20537062231407,
-2.20407837016926,-2.20246202895205,-2.19992771589964,-2.18692044017818,
-2.18500081396825,-2.18054274361608,-2.14353957294601,-2.11422385720625,
-2.10924421555971,-2.10651419163426,-2.10443830128812,-2.10177523738696,
-2.09722784245689,-2.07906677141334,-2.02674393302767,-2.01603252412601,
-2.00949767248197,-2.00736291749321,-2.00598339693557,-2.00465716641096,
-2.00271116465616,-1.99793973470904,-1.96229386775239,-1.91598641569552,
-1.91058744700268,-1.90776931635448,-1.90568583743934,-1.90309081052351,
-1.89873383491006,-1.88336259831357,-1.82805960200115,-1.81184777304384,
-1.80900976361067,-1.80747566618814,-1.80618250612422,-1.8045526380147,
-1.80135740896999,-1.7738513440458,-1.76684167449921,-1.7326897473506,-1.71522098034031,
-1.71086186562058,-1.70826614185077,-1.7059508796863,-1.70302003710355,
-1.69838465557649,-1.66981556500371,-1.61828518355143,-1.61162197191828,
-1.60947146357422,-1.60808829828351,-1.60676413741854,-1.60482975605356,
-1.60012961498056,-1.56251287398724,-1.51785616806351,-1.51257839467297,
-1.50978503745772,-1.50770366179424,-1.50509014099243,-1.50065055068393,
-1.48441328876514,-1.43003445574989,-1.41919269728428,-1.41260058492475,
-1.41045850217162,-1.40907710985822,-1.40775153269376,-1.40581027789016,
-1.40106938347263,-1.36444695536187,-1.33321373418801,-1.32253511182631,
-1.31486418271768,-1.31162137447143,-1.30925998138158,-1.30709004375631,
-1.3041511197482,-1.2979599651136),.UNSPECIFIED.);
#599=B_SPLINE_CURVE_WITH_KNOTS('',3,(#51718,#51719,#51720,#51721,#51722,
#51723,#51724,#51725,#51726,#51727,#51728,#51729,#51730,#51731,#51732,#51733,
#51734,#51735,#51736,#51737,#51738,#51739,#51740,#51741,#51742,#51743,#51744,
#51745,#51746,#51747,#51748,#51749,#51750,#51751,#51752,#51753,#51754,#51755,
#51756,#51757,#51758,#51759,#51760,#51761,#51762,#51763,#51764,#51765,#51766,
#51767,#51768,#51769,#51770,#51771,#51772,#51773,#51774,#51775,#51776,#51777,
#51778,#51779,#51780,#51781,#51782,#51783,#51784,#51785,#51786,#51787,#51788,
#51789,#51790,#51791,#51792,#51793,#51794,#51795,#51796,#51797,#51798,#51799,
#51800,#51801,#51802,#51803,#51804,#51805,#51806,#51807,#51808,#51809,#51810,
#51811,#51812,#51813,#51814,#51815,#51816,#51817,#51818,#51819,#51820,#51821,
#51822,#51823,#51824,#51825,#51826,#51827,#51828,#51829,#51830,#51831,#51832,
#51833,#51834,#51835,#51836,#51837,#51838,#51839,#51840,#51841,#51842,#51843,
#51844,#51845,#51846,#51847,#51848,#51849,#51850,#51851,#51852,#51853,#51854,
#51855,#51856,#51857,#51858,#51859,#51860,#51861,#51862,#51863,#51864,#51865,
#51866,#51867,#51868,#51869,#51870,#51871,#51872,#51873,#51874,#51875,#51876,
#51877,#51878,#51879,#51880,#51881,#51882,#51883,#51884,#51885,#51886,#51887,
#51888,#51889,#51890,#51891,#51892,#51893,#51894,#51895,#51896,#51897,#51898,
#51899,#51900,#51901,#51902,#51903,#51904,#51905,#51906,#51907,#51908,#51909,
#51910,#51911,#51912,#51913,#51914,#51915,#51916,#51917,#51918,#51919,#51920,
#51921),.UNSPECIFIED.,.F.,.F.,(4,2,2,2,2,2,2,2,2,2,2,2,2,2,2,2,2,2,2,2,
2,2,2,2,2,2,2,2,2,2,2,2,2,2,2,2,2,2,2,2,2,2,2,2,2,2,2,2,2,2,2,2,2,2,2,2,
2,2,2,2,2,2,2,2,2,2,2,2,2,2,2,2,2,2,2,2,2,2,2,2,2,2,2,2,2,2,2,2,2,2,2,2,
2,2,2,2,2,2,2,2,2,4),(-1.21650036072889,-1.20367186994537,-1.18282116663411,
-1.17970077907486,-1.17808664867918,-1.17679388214389,-1.17524582955073,
-1.17234360293463,-1.15451466079211,-1.12652620541326,-1.08722012356821,
-1.08248265487359,-1.0795206005624,-1.07720133689639,-1.07462247951083,
-1.0703422350816,-1.05387867748003,-0.99243291407614,-0.982742471554037,
-0.980211444729834,-0.978729065316574,-0.977558951089079,-0.97592432504103,
-0.972601684253843,-0.9682320273792,-0.957619681100799,-0.906781926283804,
-0.887158309976383,-0.882507253059537,-0.879819477496966,-0.877512917767558,
-0.874708755984211,-0.86938195344554,-0.862679662250612,-0.847523928323767,
-0.811106078629044,-0.784862251302172,-0.781669943467085,-0.780040265626657,
-0.778746569580856,-0.777211017242905,-0.774368191834507,-0.758063423902879,
-0.701603942797503,-0.687274339295151,-0.683022133879214,-0.680449360193734,
-0.678128657692247,-0.675155185270078,-0.668982492772153,-0.66090702588705,
-0.640955800900654,-0.613221779684546,-0.585848361861189,-0.582651647437803,
-0.581021134736983,-0.579727523258687,-0.578192952960173,-0.575354248457255,
-0.55914148528599,-0.503828590668287,-0.488469185439362,-0.484112206372492,
-0.481516555517238,-0.479432229843889,-0.476612490472009,-0.471208886787708,
-0.426874476351277,-0.389086557088364,-0.384388177306999,-0.382453870014954,
-0.381129550381289,-0.37974600356618,-0.377594538691698,-0.370925306233708,
-0.319405261909269,-0.290851926464014,-0.286216345164176,-0.283285068668805,
-0.280969286795655,-0.278372794614662,-0.274011947866813,-0.256530708865576,
-0.222340001321887,-0.190273831804208,-0.185441780683738,-0.183485268354989,
-0.182276786076821,-0.180953642407111,-0.179088867087865,-0.17689189933228,
-0.172907165168017,-0.163617848116005,-0.126922269847658,-0.0921073323921683,
-0.0873569083596852,-0.0843910316936627,-0.082071410488705,-0.0794948632014784,
-0.0752248005201745,-0.0588829643078642,-0.000583356136067976),
 .UNSPECIFIED.);
#600=B_SPLINE_CURVE_WITH_KNOTS('',3,(#51922,#51923,#51924,#51925,#51926,
#51927,#51928,#51929,#51930,#51931,#51932,#51933,#51934,#51935,#51936,#51937,
#51938,#51939,#51940,#51941,#51942,#51943),.UNSPECIFIED.,.F.,.F.,(4,2,2,
2,2,2,2,2,2,2,4),(-2.51402463792542,-2.50549522727735,-2.50071004123171,
-2.49896216044422,-2.49765999716403,-2.49642378936312,-2.49500799844318,
-2.49271099182215,-2.48550006123663,-2.47542634793241,-2.47330243401613),
 .UNSPECIFIED.);
#601=B_SPLINE_CURVE_WITH_KNOTS('',3,(#51944,#51945,#51946,#51947,#51948,
#51949,#51950,#51951,#51952,#51953,#51954,#51955,#51956,#51957,#51958,#51959,
#51960,#51961,#51962,#51963,#51964,#51965,#51966,#51967,#51968,#51969,#51970,
#51971,#51972,#51973,#51974,#51975,#51976,#51977,#51978,#51979,#51980,#51981,
#51982,#51983,#51984,#51985,#51986,#51987,#51988,#51989,#51990,#51991,#51992,
#51993,#51994,#51995,#51996,#51997,#51998,#51999,#52000,#52001,#52002,#52003,
#52004,#52005,#52006,#52007,#52008,#52009,#52010,#52011,#52012,#52013,#52014,
#52015,#52016,#52017,#52018,#52019,#52020,#52021,#52022,#52023,#52024,#52025,
#52026,#52027,#52028,#52029,#52030,#52031,#52032,#52033,#52034,#52035,#52036,
#52037,#52038,#52039,#52040,#52041,#52042,#52043,#52044,#52045,#52046,#52047,
#52048,#52049,#52050,#52051,#52052,#52053,#52054,#52055,#52056,#52057,#52058,
#52059,#52060,#52061,#52062,#52063,#52064,#52065,#52066,#52067,#52068,#52069,
#52070,#52071,#52072,#52073,#52074,#52075,#52076,#52077,#52078,#52079,#52080,
#52081,#52082,#52083,#52084,#52085,#52086,#52087,#52088,#52089,#52090,#52091,
#52092,#52093,#52094,#52095,#52096,#52097,#52098,#52099,#52100,#52101,#52102,
#52103,#52104,#52105,#52106,#52107,#52108,#52109,#52110,#52111,#52112,#52113,
#52114,#52115,#52116,#52117,#52118,#52119,#52120,#52121,#52122,#52123,#52124,
#52125,#52126,#52127,#52128,#52129,#52130,#52131,#52132,#52133,#52134,#52135,
#52136,#52137,#52138,#52139,#52140,#52141,#52142,#52143,#52144,#52145,#52146,
#52147,#52148,#52149,#52150,#52151,#52152,#52153,#52154,#52155,#52156,#52157),
 .UNSPECIFIED.,.F.,.F.,(4,2,2,2,2,2,2,2,2,2,2,2,2,2,2,2,2,2,2,2,2,2,2,2,
2,2,2,2,2,2,2,2,2,2,2,2,2,2,2,2,2,2,2,2,2,2,2,2,2,2,2,2,2,2,2,2,2,2,2,2,
2,2,2,2,2,2,2,2,2,2,2,2,2,2,2,2,2,2,2,2,2,2,2,2,2,2,2,2,2,2,2,2,2,2,2,2,
2,2,2,2,2,2,2,2,2,2,4),(-1.2979599651136,-1.29683172309349,-1.25693384069821,
-1.21777271999702,-1.21314919010135,-1.2114175514501,-1.21018610818971,
-1.20885807811842,-1.20697351826947,-1.20224462656028,-1.177707910862,-1.17094480686257,
-1.1227154856321,-1.11561286154691,-1.11278199147127,-1.11042371348871,
-1.10799791325747,-1.10442405447166,-1.09457601726633,-1.07968485494448,
-1.04817950923121,-1.03165926508212,-1.01618198226899,-1.01351288545697,
-1.01185539675462,-1.01056005896471,-1.00904627471541,-1.00630375452611,
-0.992140708472749,-0.956198918232946,-0.920941082911946,-0.91618815099358,
-0.913221600078467,-0.910902000352238,-0.90832604029203,-0.904058269750652,
-0.887742257023649,-0.85599919378957,-0.820052965067163,-0.815287322838515,
-0.813341917151239,-0.812015507705065,-0.810635215782818,-0.808498267819918,
-0.801948746498178,-0.79120639885158,-0.738391663700838,-0.720705173585745,
-0.716195765677733,-0.713540850855021,-0.711232766319075,-0.70838898213429,
-0.702867467485636,-0.659823902089313,-0.620866468667174,-0.616229215977293,
-0.614495756431457,-0.613263866081292,-0.611936295925047,-0.610053932615929,
-0.605338507600838,-0.580944205932299,-0.569982853823161,-0.526199998315964,
-0.518981285203984,-0.516053857762003,-0.513886780194649,-0.511523038667,
-0.508267051420153,-0.500517252130685,-0.489694002144564,-0.429173972315372,
-0.418618658252525,-0.416012841042599,-0.414513325419673,-0.41322821998872,
-0.411556214653473,-0.408042297653843,-0.376664048771488,-0.326446396702602,
-0.320220844124137,-0.316835043363872,-0.314470653002961,-0.312051961087735,
-0.308513451095731,-0.298920708482545,-0.284552365815458,-0.255289392249783,
-0.223082005537083,-0.218254892260719,-0.216299106064572,-0.215090683644324,
-0.213767393184338,-0.211838465352321,-0.209600408345692,-0.205508614267596,
-0.195858245778487,-0.175151099567017,-0.127853858338076,-0.120675676913724,
-0.117832690836522,-0.115471183934514,-0.113049075906374,-0.109493741974358,
-0.0997805979002047,-0.0851668180726992,-0.0414579409595978),
 .UNSPECIFIED.);
#602=B_SPLINE_CURVE_WITH_KNOTS('',3,(#52162,#52163,#52164,#52165,#52166,
#52167,#52168,#52169,#52170,#52171,#52172,#52173,#52174,#52175,#52176,#52177,
#52178,#52179,#52180,#52181,#52182,#52183,#52184,#52185,#52186,#52187,#52188,
#52189,#52190,#52191,#52192,#52193,#52194,#52195,#52196,#52197,#52198,#52199,
#52200,#52201,#52202,#52203,#52204,#52205,#52206,#52207,#52208,#52209,#52210,
#52211,#52212,#52213,#52214,#52215,#52216,#52217,#52218,#52219,#52220,#52221,
#52222,#52223,#52224,#52225,#52226,#52227,#52228,#52229,#52230,#52231,#52232,
#52233,#52234,#52235,#52236,#52237,#52238,#52239,#52240,#52241,#52242,#52243,
#52244,#52245,#52246,#52247,#52248,#52249,#52250,#52251,#52252,#52253,#52254,
#52255,#52256,#52257,#52258,#52259,#52260,#52261,#52262,#52263,#52264,#52265,
#52266,#52267,#52268,#52269,#52270,#52271,#52272,#52273,#52274,#52275,#52276,
#52277,#52278,#52279,#52280,#52281,#52282,#52283,#52284,#52285,#52286,#52287,
#52288,#52289,#52290,#52291,#52292,#52293,#52294,#52295,#52296,#52297,#52298,
#52299,#52300,#52301,#52302,#52303,#52304,#52305,#52306,#52307,#52308,#52309,
#52310,#52311,#52312,#52313,#52314,#52315,#52316,#52317,#52318,#52319,#52320,
#52321,#52322,#52323,#52324,#52325,#52326,#52327,#52328,#52329,#52330,#52331,
#52332,#52333,#52334,#52335,#52336,#52337,#52338,#52339,#52340,#52341,#52342,
#52343,#52344,#52345,#52346,#52347,#52348,#52349,#52350,#52351,#52352,#52353,
#52354,#52355,#52356,#52357,#52358,#52359,#52360,#52361,#52362,#52363,#52364,
#52365,#52366,#52367,#52368,#52369,#52370,#52371,#52372,#52373,#52374,#52375,
#52376,#52377),.UNSPECIFIED.,.F.,.F.,(4,2,2,2,2,2,2,2,2,2,2,2,2,2,2,2,2,
2,2,2,2,2,2,2,2,2,2,2,2,2,2,2,2,2,2,2,2,2,2,2,2,2,2,2,2,2,2,2,2,2,2,2,2,
2,2,2,2,2,2,2,2,2,2,2,2,2,2,2,2,2,2,2,2,2,2,2,2,2,2,2,2,2,2,2,2,2,2,2,2,
2,2,2,2,2,2,2,2,2,2,2,2,2,2,2,2,2,2,4),(-2.47274746625746,-2.471414553606,
-2.4691009156549,-2.46618274476928,-2.46158840004806,-2.43433135557283,
-2.41229008486747,-2.39217407961196,-2.37612000131115,-2.37327759320698,
-2.37174271505682,-2.37044985026478,-2.36882156090834,-2.36563297270697,
-2.33958927769404,-2.29182976432504,-2.28311859426973,-2.27661796832897,
-2.27359455315258,-2.27125990403053,-2.26874299723464,-2.26474075416736,
-2.2525895908786,-2.19365390955991,-2.17717296614671,-2.17432382067116,
-2.17278740135833,-2.17149448489933,-2.16986770744262,-2.16668670669114,
-2.14146194487422,-2.09509765707905,-2.08518190363019,-2.07793721140512,
-2.07476787307734,-2.07241965899032,-2.06993507353194,-2.06608200034155,
-2.05508728776842,-1.99476793322313,-1.97819590965774,-1.97534272824399,
-1.97380532529832,-1.9725122893131,-1.97088625647507,-1.96770932991216,
-1.93763787784834,-1.93316837088126,-1.89900600571225,-1.88153374191713,
-1.87717415023586,-1.87457820814676,-1.87226279214933,-1.8693318102059,
-1.86469631835272,-1.83613233668754,-1.7845960136792,-1.77792831817086,
-1.77577718045054,-1.77439381391977,-1.77306963358639,-1.77113548983019,
-1.76643725668463,-1.72861795153154,-1.68417771525276,-1.67888623353082,
-1.67608990196283,-1.67400811585188,-1.67139643961998,-1.66696578001415,
-1.65082510687123,-1.59633679487874,-1.58548801942921,-1.57889273009809,
-1.57675016942139,-1.57536860824337,-1.57404298812628,-1.57210185424649,
-1.56736217354812,-1.53064984976071,-1.49947755820319,-1.48881054279297,
-1.48114588825112,-1.47790399433372,-1.47554263746853,-1.47337229590405,
-1.47043215790565,-1.4631124173592,-1.42369519390846,-1.39351920021738,
-1.38510018450829,-1.37961519610419,-1.37761747722383,-1.3762670178633,
-1.37505865278752,-1.3731029323962,-1.36827583132125,-1.33550052528379,
-1.31531667455507,-1.2883766060435,-1.28172364296457,-1.27865966399012,
-1.27632708699658,-1.27379905200053,-1.26975002003021,-1.25722474018032,
-1.23573035801547,-1.21650036072889),.UNSPECIFIED.);
#603=B_SPLINE_CURVE_WITH_KNOTS('',3,(#52379,#52380,#52381,#52382,#52383,
#52384,#52385,#52386,#52387,#52388,#52389,#52390,#52391,#52392,#52393,#52394,
#52395,#52396,#52397,#52398,#52399,#52400),.UNSPECIFIED.,.F.,.F.,(4,2,2,
2,2,2,2,2,2,2,4),(-0.0414579409595978,-0.035082825383997,-0.0251484303517282,
-0.0195179196149325,-0.0174347627193792,-0.0162021523227704,-0.0149718856855802,
-0.0136622933178273,-0.011894101725279,-0.00763339607549248,-0.000737909110566063),
 .UNSPECIFIED.);
#604=B_SPLINE_CURVE_WITH_KNOTS('',3,(#52401,#52402,#52403,#52404,#52405,
#52406,#52407,#52408,#52409,#52410,#52411,#52412,#52413,#52414,#52415,#52416,
#52417,#52418,#52419,#52420,#52421,#52422,#52423,#52424,#52425,#52426,#52427,
#52428,#52429,#52430,#52431,#52432,#52433,#52434,#52435,#52436,#52437,#52438,
#52439,#52440,#52441,#52442,#52443,#52444,#52445,#52446,#52447,#52448,#52449,
#52450,#52451,#52452,#52453,#52454,#52455,#52456,#52457,#52458,#52459,#52460,
#52461,#52462,#52463,#52464,#52465,#52466,#52467,#52468,#52469,#52470,#52471,
#52472,#52473,#52474,#52475,#52476,#52477,#52478,#52479,#52480,#52481,#52482,
#52483,#52484,#52485,#52486,#52487,#52488,#52489,#52490,#52491,#52492,#52493,
#52494,#52495,#52496,#52497,#52498,#52499,#52500,#52501,#52502,#52503,#52504,
#52505,#52506,#52507,#52508,#52509,#52510,#52511,#52512,#52513,#52514,#52515,
#52516,#52517,#52518,#52519,#52520,#52521,#52522,#52523,#52524,#52525,#52526,
#52527,#52528,#52529,#52530,#52531,#52532,#52533,#52534,#52535,#52536,#52537,
#52538,#52539,#52540,#52541,#52542,#52543,#52544,#52545,#52546,#52547,#52548,
#52549,#52550,#52551,#52552,#52553,#52554,#52555,#52556,#52557,#52558,#52559,
#52560,#52561,#52562,#52563,#52564,#52565,#52566,#52567,#52568,#52569,#52570,
#52571,#52572,#52573,#52574,#52575,#52576,#52577,#52578,#52579,#52580,#52581,
#52582,#52583,#52584,#52585,#52586,#52587,#52588,#52589,#52590,#52591,#52592,
#52593,#52594,#52595,#52596,#52597,#52598,#52599,#52600,#52601,#52602,#52603,
#52604,#52605,#52606),.UNSPECIFIED.,.F.,.F.,(4,2,2,2,2,2,2,2,2,2,2,2,2,
2,2,2,2,2,2,2,2,2,2,2,2,2,2,2,2,2,2,2,2,2,2,2,2,2,2,2,2,2,2,2,2,2,2,2,2,
2,2,2,2,2,2,2,2,2,2,2,2,2,2,2,2,2,2,2,2,2,2,2,2,2,2,2,2,2,2,2,2,2,2,2,2,
2,2,2,2,2,2,2,2,2,2,2,2,2,2,2,2,2,4),(-4.94417392363714,-4.91309937476047,
-4.86968439704114,-4.86421139772586,-4.86137802808041,-4.85907119219392,
-4.85640970024793,-4.85186962012977,-4.83381261522179,-4.79315018454536,
-4.77433350418817,-4.76794881584999,-4.76488705623448,-4.76305437616443,
-4.76140466693561,-4.76014136217213,-4.7586591429474,-4.75612644877624,
-4.74640621522903,-4.68506455852927,-4.66861826655063,-4.66434111431908,
-4.66176384290726,-4.65944582765207,-4.65648512272851,-4.65174927183508,
-4.61252305738833,-4.58424604816674,-4.56661882160062,-4.56372513596879,
-4.56217940540007,-4.56088727226615,-4.55927230071572,-4.55614562071163,
-4.53444460522209,-4.50393169553112,-4.48204132577849,-4.46911966755911,
-4.46517352707056,-4.46266888840275,-4.46032967164745,-4.45726839648233,
-4.45044209682022,-4.39946217048655,-4.37757928544131,-4.3705716713677,
-4.36579031290003,-4.36389796509929,-4.3625689053494,-4.36134006837862,
-4.35961693724228,-4.35505381427277,-4.31459501537612,-4.2728386550215,
-4.26743289722181,-4.26461349687611,-4.26253001990676,-4.25993620408022,
-4.25558416503592,-4.24026614476112,-4.18491133340216,-4.1686961834239,
-4.16585819813638,-4.16432417700165,-4.16303111903489,-4.16140142748592,
-4.15820668555396,-4.13035592368184,-4.09706635616234,-4.08103120601792,
-4.07406433375861,-4.06857143507874,-4.06573388044859,-4.06342665600911,
-4.06076807240829,-4.05624112352644,-4.03831269015808,-3.99057379301517,
-3.97663377193337,-3.97137788468322,-3.96754129516396,-3.96580906450669,
-3.96450596841191,-3.96303942038778,-3.96051197589568,-3.95116727443693,
-3.88941325803181,-3.87293312617115,-3.86865290733104,-3.86607480205627,
-3.86375668091635,-3.86079672924062,-3.85606388556261,-3.81659782472707,
-3.78781351117836,-3.7708729000657,-3.7680053230561,-3.76646504626298,-3.76517247769287,
-3.76355066910472,-3.76039257516026,-3.73692200761545,-3.72889146245253),
 .UNSPECIFIED.);
#605=B_SPLINE_CURVE_WITH_KNOTS('',3,(#52612,#52613,#52614,#52615,#52616,
#52617,#52618,#52619,#52620,#52621,#52622,#52623,#52624,#52625,#52626,#52627,
#52628,#52629,#52630,#52631,#52632,#52633,#52634,#52635,#52636,#52637,#52638,
#52639,#52640,#52641,#52642,#52643,#52644,#52645,#52646,#52647,#52648,#52649,
#52650,#52651,#52652,#52653,#52654,#52655,#52656,#52657,#52658,#52659,#52660,
#52661,#52662,#52663,#52664,#52665,#52666,#52667,#52668,#52669,#52670,#52671,
#52672,#52673,#52674,#52675,#52676,#52677,#52678,#52679,#52680,#52681,#52682,
#52683,#52684,#52685,#52686,#52687,#52688,#52689,#52690,#52691,#52692,#52693,
#52694,#52695,#52696,#52697,#52698,#52699,#52700,#52701,#52702,#52703,#52704,
#52705,#52706,#52707,#52708,#52709,#52710,#52711,#52712,#52713,#52714,#52715,
#52716,#52717,#52718,#52719,#52720,#52721,#52722,#52723,#52724,#52725,#52726,
#52727,#52728,#52729,#52730,#52731,#52732,#52733,#52734,#52735,#52736,#52737,
#52738,#52739,#52740,#52741,#52742,#52743,#52744,#52745,#52746,#52747,#52748,
#52749,#52750,#52751,#52752,#52753,#52754,#52755,#52756,#52757,#52758,#52759,
#52760,#52761,#52762,#52763,#52764,#52765,#52766,#52767,#52768,#52769,#52770,
#52771,#52772,#52773,#52774,#52775,#52776,#52777,#52778,#52779,#52780,#52781,
#52782,#52783,#52784,#52785,#52786,#52787,#52788,#52789,#52790,#52791,#52792,
#52793,#52794,#52795,#52796,#52797,#52798,#52799,#52800,#52801,#52802,#52803,
#52804,#52805,#52806,#52807,#52808,#52809,#52810,#52811,#52812,#52813,#52814,
#52815,#52816,#52817,#52818,#52819,#52820,#52821,#52822,#52823),
 .UNSPECIFIED.,.F.,.F.,(4,2,2,2,2,2,2,2,2,2,2,2,2,2,2,2,2,2,2,2,2,2,2,2,
2,2,2,2,2,2,2,2,2,2,2,2,2,2,2,2,2,2,2,2,2,2,2,2,2,2,2,2,2,2,2,2,2,2,2,2,
2,2,2,2,2,2,2,2,2,2,2,2,2,2,2,2,2,2,2,2,2,2,2,2,2,2,2,2,2,2,2,2,2,2,2,2,
2,2,2,2,2,2,2,2,2,4),(-1.21629508419202,-1.19678839020098,-1.16104491785065,
-1.15628570130955,-1.15331657066828,-1.15099577848306,-1.14841933863923,
-1.14415274393049,-1.12786642522531,-1.09623267748193,-1.06010503978159,
-1.05534344462364,-1.05339816777709,-1.0520713401155,-1.05069017862987,
-1.04855099304072,-1.04198762072658,-1.03121523453434,-0.977972166463608,
-0.96066908255111,-0.956187881121162,-0.953538795504893,-0.951229165488729,
-0.948374972133484,-0.942805766748834,-0.904684326654697,-0.861756292261737,
-0.856453418023476,-0.854419258705664,-0.85319596308645,-0.851860389793916,
-0.849937951754468,-0.844968078723773,-0.837593936543774,-0.813768795062902,
-0.765769968466468,-0.758644059750312,-0.755808917826503,-0.75344900265554,
-0.751023487926242,-0.747453738513993,-0.73764084906406,-0.722823887910961,
-0.691827481436309,-0.674143142336256,-0.659114303260826,-0.656473920147491,
-0.654824785869057,-0.653529694837953,-0.652008874976559,-0.649235250193616,
-0.634465333703563,-0.592212401814593,-0.563669993955392,-0.559033585760423,
-0.556101591969151,-0.553785121086686,-0.551187727972645,-0.546825058547546,
-0.52933203433922,-0.495107882335919,-0.463078324795227,-0.458234173098523,
-0.456275288138125,-0.455066111876199,-0.45371586914444,-0.451720418063046,
-0.446253730874893,-0.437874421452672,-0.40796825578915,-0.368245711051937,
-0.360927040955379,-0.357982029059069,-0.355810079437357,-0.353448892914874,
-0.350210729175154,-0.342571513127716,-0.331950278381618,-0.301017417565392,
-0.263904490107245,-0.25917058714467,-0.257230063246971,-0.255904279963507,
-0.254521966778183,-0.252377242892097,-0.246048019081636,-0.235678356871826,
-0.188090172556569,-0.165225680098754,-0.160793078874204,-0.157923110737925,
-0.155612349271606,-0.153439380975918,-0.149679596395542,-0.137398977606132,
-0.11699930020956,-0.0983284252223009,-0.0772706239788904,-0.0620776668811129,
-0.0594294807345166,-0.0577780454785035,-0.0564828586952099,-0.054963922106604,
-0.0521987249030516,-0.0487365117228446,-0.00058344341590058),
 .UNSPECIFIED.);
#606=B_SPLINE_CURVE_WITH_KNOTS('',3,(#52824,#52825,#52826,#52827,#52828,
#52829,#52830,#52831,#52832,#52833),.UNSPECIFIED.,.F.,.F.,(4,2,2,2,4),(-2.51371913210301,
-2.47983225959379,-2.47613607850828,-2.4735811998181,-2.47274746625746),
 .UNSPECIFIED.);
#607=B_SPLINE_CURVE_WITH_KNOTS('',3,(#52834,#52835,#52836,#52837,#52838,
#52839,#52840,#52841,#52842,#52843,#52844,#52845,#52846,#52847,#52848,#52849,
#52850,#52851,#52852,#52853,#52854,#52855,#52856,#52857,#52858,#52859,#52860,
#52861,#52862,#52863,#52864,#52865,#52866,#52867,#52868,#52869,#52870,#52871,
#52872,#52873,#52874,#52875,#52876,#52877,#52878,#52879,#52880,#52881,#52882,
#52883,#52884,#52885,#52886,#52887,#52888,#52889,#52890,#52891,#52892,#52893,
#52894,#52895,#52896,#52897,#52898,#52899,#52900,#52901,#52902,#52903,#52904,
#52905,#52906,#52907,#52908,#52909,#52910,#52911,#52912,#52913,#52914,#52915,
#52916,#52917,#52918,#52919,#52920,#52921,#52922,#52923,#52924,#52925,#52926,
#52927,#52928,#52929,#52930,#52931,#52932,#52933,#52934,#52935,#52936,#52937,
#52938,#52939,#52940,#52941,#52942,#52943,#52944,#52945,#52946,#52947,#52948,
#52949,#52950,#52951,#52952,#52953,#52954,#52955,#52956,#52957,#52958,#52959,
#52960,#52961,#52962,#52963,#52964,#52965,#52966,#52967,#52968,#52969,#52970,
#52971,#52972,#52973,#52974,#52975,#52976,#52977,#52978,#52979,#52980,#52981,
#52982,#52983,#52984,#52985,#52986,#52987,#52988,#52989,#52990,#52991,#52992,
#52993,#52994,#52995,#52996,#52997,#52998,#52999,#53000,#53001,#53002,#53003,
#53004,#53005,#53006,#53007,#53008,#53009,#53010,#53011,#53012,#53013,#53014,
#53015,#53016,#53017,#53018,#53019,#53020,#53021,#53022,#53023,#53024,#53025,
#53026,#53027,#53028,#53029,#53030,#53031,#53032,#53033,#53034,#53035,#53036,
#53037,#53038,#53039,#53040,#53041,#53042,#53043,#53044,#53045,#53046,#53047,
#53048,#53049),.UNSPECIFIED.,.F.,.F.,(4,2,2,2,2,2,2,2,2,2,2,2,2,2,2,2,2,
2,2,2,2,2,2,2,2,2,2,2,2,2,2,2,2,2,2,2,2,2,2,2,2,2,2,2,2,2,2,2,2,2,2,2,2,
2,2,2,2,2,2,2,2,2,2,2,2,2,2,2,2,2,2,2,2,2,2,2,2,2,2,2,2,2,2,2,2,2,2,2,2,
2,2,2,2,2,2,2,2,2,2,2,2,2,2,2,2,2,2,4),(-3.72889146245253,-3.70814737956327,
-3.67850138071064,-3.6715193570599,-3.66839644412708,-3.66605578815816,
-3.66355399236289,-3.6596215820007,-3.648026213805,-3.59456838646231,-3.57418488333566,
-3.56986991519399,-3.56805350092186,-3.56673783224545,-3.56548844789078,
-3.56331816032759,-3.55707816967706,-3.51509719579875,-3.47674241207794,
-3.47154701262265,-3.46877116179606,-3.46648852465219,-3.46378738866586,
-3.45907390511088,-3.43852733930262,-3.38863019253642,-3.37808559430011,
-3.37373601979671,-3.37042592299356,-3.36879427702333,-3.36762499636274,
-3.36614188270185,-3.36360576439069,-3.35384974949012,-3.29253812922952,
-3.27609291442109,-3.27181551147186,-3.26923799499472,-3.26691969959496,
-3.26395855442644,-3.25922183203965,-3.21998596548248,-3.19219438895693,
-3.17411045379676,-3.17119990338276,-3.16965049307307,-3.16835837464804,
-3.16674728923823,-3.16423037400043,-3.15154337062974,-3.14325158106825,
-3.1288173075177,-3.09480300866722,-3.07737428864688,-3.07301858821809,
-3.07042380086867,-3.06810869042,-3.06517711349699,-3.0605387265637,-3.03185332947279,
-2.98974000692742,-2.97499389114168,-2.97222264186156,-2.97070291720249,
-2.96940861376678,-2.96776031224662,-2.96512097607141,-2.95008743550299,
-2.93245114892786,-2.90150021336824,-2.88669189827361,-2.88009682737053,
-2.87483807038743,-2.8720488845178,-2.86976565030023,-2.86707593473933,
-2.86241297354053,-2.84259391659081,-2.79195382484259,-2.7813557142552,
-2.77487012829037,-2.77274118511584,-2.77136280098706,-2.7700354057418,
-2.76808419274215,-2.76328250359025,-2.72885535548839,-2.69644499336853,
-2.68524758058578,-2.67729326456345,-2.67400386593341,-2.67163432594743,
-2.66947454417706,-2.66602785580541,-2.6595723626451,-2.6121355126774,-2.57810149475438,
-2.57474320419319,-2.57310186053851,-2.57180781952792,-2.57028230126718,
-2.56756159203472,-2.55545353712949,-2.51816897716757,-2.48693956435907,
-2.4785150864885,-2.47515044650355,-2.47285424115159),.UNSPECIFIED.);
#608=B_SPLINE_CURVE_WITH_KNOTS('',3,(#53054,#53055,#53056,#53057,#53058,
#53059,#53060,#53061,#53062,#53063,#53064,#53065,#53066,#53067,#53068,#53069,
#53070,#53071,#53072,#53073,#53074,#53075,#53076,#53077,#53078,#53079,#53080,
#53081,#53082,#53083,#53084,#53085,#53086,#53087,#53088,#53089,#53090,#53091,
#53092,#53093,#53094,#53095,#53096,#53097,#53098,#53099,#53100,#53101,#53102,
#53103,#53104,#53105,#53106,#53107,#53108,#53109,#53110,#53111,#53112,#53113,
#53114,#53115,#53116,#53117,#53118,#53119,#53120,#53121,#53122,#53123,#53124,
#53125,#53126,#53127,#53128,#53129,#53130,#53131,#53132,#53133,#53134,#53135,
#53136,#53137,#53138,#53139,#53140,#53141,#53142,#53143,#53144,#53145,#53146,
#53147,#53148,#53149,#53150,#53151,#53152,#53153,#53154,#53155,#53156,#53157,
#53158,#53159,#53160,#53161,#53162,#53163,#53164,#53165,#53166,#53167,#53168,
#53169,#53170,#53171,#53172,#53173,#53174,#53175,#53176,#53177,#53178,#53179,
#53180,#53181,#53182,#53183,#53184,#53185,#53186,#53187,#53188,#53189,#53190,
#53191,#53192,#53193,#53194,#53195,#53196,#53197,#53198,#53199,#53200,#53201,
#53202,#53203,#53204,#53205,#53206,#53207,#53208,#53209,#53210,#53211,#53212,
#53213,#53214,#53215,#53216,#53217,#53218,#53219,#53220,#53221,#53222,#53223,
#53224,#53225,#53226,#53227,#53228,#53229,#53230,#53231,#53232,#53233,#53234,
#53235,#53236,#53237,#53238,#53239,#53240,#53241,#53242,#53243,#53244,#53245,
#53246,#53247,#53248,#53249,#53250,#53251,#53252,#53253,#53254,#53255,#53256,
#53257,#53258,#53259,#53260,#53261,#53262,#53263,#53264,#53265,#53266,#53267,
#53268,#53269,#53270,#53271,#53272,#53273,#53274,#53275,#53276,#53277,#53278,
#53279,#53280,#53281,#53282,#53283,#53284,#53285,#53286,#53287,#53288,#53289,
#53290,#53291,#53292,#53293,#53294,#53295,#53296,#53297,#53298,#53299,#53300,
#53301,#53302,#53303,#53304,#53305),.UNSPECIFIED.,.F.,.F.,(4,2,2,2,2,2,
2,2,2,2,2,2,2,2,2,2,2,2,2,2,2,2,2,2,2,2,2,2,2,2,2,2,2,2,2,2,2,2,2,2,2,2,
2,2,2,2,2,2,2,2,2,2,2,2,2,2,2,2,2,2,2,2,2,2,2,2,2,2,2,2,2,2,2,2,2,2,2,2,
2,2,2,2,2,2,2,2,2,2,2,2,2,2,2,2,2,2,2,2,2,2,2,2,2,2,2,2,2,2,2,2,2,2,2,2,
2,2,2,2,2,2,2,2,2,2,2,4),(-2.47288460460841,-2.46217668520358,-2.45385741648579,
-2.44842797008862,-2.44644735082339,-2.44510673058267,-2.44389844342252,
-2.44194264161838,-2.43711557726936,-2.40584105658942,-2.37909361016463,
-2.36259189401898,-2.35548163686839,-2.34995499696683,-2.34711409768511,
-2.34707612557772,-2.34703676848092,-2.34699593631053,-2.34695353125495,
-2.34690944682533,-2.34686356696828,-2.34681576497736,-2.34676590221363,
-2.34671382678595,-2.34668493887874,-2.34664924377911,-2.34660498019936,
-2.34654984827375,-2.34648080002835,-2.34639372332381,-2.34407313383829,
-2.34113701045427,-2.33649584305399,-2.30851326433016,-2.25667588832234,
-2.25002761095081,-2.24787382212599,-2.24648639122181,-2.24515909700479,
-2.24321700903982,-2.23847996446942,-2.20156569123459,-2.17057301912225,
-2.15994183953601,-2.15229669829309,-2.14905718721466,-2.14669541064296,
-2.14452318098929,-2.14157818494998,-2.13426162132827,-2.09452750657146,
-2.06455304929185,-2.05616275930657,-2.05069146109291,-2.04869575205888,
-2.04734580481157,-2.0461379936048,-2.04418213507868,-2.03934922351807,
-2.00848058426198,-1.98246078709795,-1.95879954636734,-1.95257820089051,
-1.94959690266899,-1.94727697053376,-1.94471207503551,-1.94048923367701,
-1.92641218740427,-1.86960509081213,-1.8532692903952,-1.85042685223263,
-1.84889223881666,-1.84759901138635,-1.84596987209372,-1.84278053276337,
-1.81689711895634,-1.76942955283411,-1.75587601875855,-1.75186136709879,
-1.74934014183666,-1.74700385540109,-1.74397262251822,-1.73732256888089,
-1.68484089034511,-1.68174005283103,-1.65710191660181,-1.65236252691992,
-1.65047546692496,-1.64914630902854,-1.64791466889562,-1.6461833084425,
-1.64156475153857,-1.60233722297374,-1.55952867962303,-1.55402525946383,
-1.55118463893462,-1.54887608804044,-1.54621727100728,-1.54169307227898,
-1.52382460898796,-1.47113653147148,-1.46039630121876,-1.45384771448924,
-1.45171051214816,-1.45032992927386,-1.4490031886144,-1.44705716119622,
-1.44228925704491,-1.40640458344367,-1.37462873679908,-1.3638434844486,
-1.35611341149774,-1.35286025042937,-1.35049659613107,-1.34832823557855,
-1.34483722250932,-1.33623989256087,-1.28593147523885,-1.25709695277123,
-1.25365003001172,-1.25199090293672,-1.25069502957743,-1.24918144133462,
-1.2464416207899,-1.23234706953041,-1.21629508419202),.UNSPECIFIED.);
#609=B_SPLINE_CURVE_WITH_KNOTS('',3,(#53306,#53307,#53308,#53309,#53310,
#53311,#53312,#53313,#53314,#53315,#53316,#53317,#53318,#53319,#53320,#53321,
#53322,#53323,#53324,#53325,#53326,#53327,#53328,#53329,#53330,#53331,#53332,
#53333,#53334,#53335,#53336,#53337,#53338,#53339,#53340,#53341,#53342,#53343,
#53344,#53345,#53346,#53347,#53348,#53349,#53350,#53351,#53352,#53353,#53354,
#53355,#53356,#53357,#53358,#53359,#53360,#53361,#53362,#53363,#53364,#53365,
#53366,#53367,#53368,#53369,#53370,#53371,#53372,#53373,#53374,#53375,#53376,
#53377,#53378,#53379,#53380,#53381,#53382,#53383,#53384,#53385,#53386,#53387,
#53388,#53389,#53390,#53391,#53392,#53393,#53394,#53395,#53396,#53397,#53398,
#53399,#53400,#53401,#53402,#53403,#53404,#53405,#53406,#53407,#53408,#53409,
#53410,#53411,#53412,#53413,#53414,#53415,#53416,#53417,#53418,#53419,#53420,
#53421,#53422,#53423,#53424,#53425,#53426,#53427,#53428,#53429,#53430,#53431,
#53432,#53433,#53434,#53435,#53436,#53437,#53438,#53439,#53440,#53441,#53442,
#53443,#53444,#53445,#53446,#53447,#53448,#53449,#53450,#53451,#53452,#53453,
#53454,#53455,#53456,#53457,#53458,#53459,#53460,#53461,#53462,#53463,#53464,
#53465,#53466,#53467,#53468,#53469,#53470,#53471,#53472,#53473,#53474,#53475,
#53476,#53477,#53478,#53479,#53480,#53481,#53482,#53483,#53484,#53485,#53486,
#53487,#53488,#53489,#53490,#53491,#53492,#53493,#53494,#53495,#53496,#53497,
#53498,#53499,#53500,#53501,#53502,#53503,#53504,#53505,#53506,#53507,#53508,
#53509,#53510,#53511,#53512,#53513,#53514,#53515),.UNSPECIFIED.,.F.,.F.,
(4,2,2,2,2,2,2,2,2,2,2,2,2,2,2,2,2,2,2,2,2,2,2,2,2,2,2,2,2,2,2,2,2,2,2,
2,2,2,2,2,2,2,2,2,2,2,2,2,2,2,2,2,2,2,2,2,2,2,2,2,2,2,2,2,2,2,2,2,2,2,2,
2,2,2,2,2,2,2,2,2,2,2,2,2,2,2,2,2,2,2,2,2,2,2,2,2,2,2,2,2,2,2,2,2,4),(-2.47285424115159,
-2.47276667947185,-2.47033894217288,-2.46675482693037,-2.45683029588147,
-2.44178044602466,-2.40684632584979,-2.37898262027467,-2.37578675672441,
-2.37415662269162,-2.37286329111761,-2.37132903311689,-2.36849081884094,
-2.35227832689895,-2.29693818648215,-2.28161785796799,-2.27726499472531,
-2.27467061613181,-2.2725866502792,-2.26976653019207,-2.2643592274727,-2.25752846390797,
-2.24194665569387,-2.20350418876136,-2.17995793241073,-2.17679795186298,
-2.17517556984587,-2.17388275549834,-2.17234243148313,-2.1694754358018,
-2.15255718248808,-2.12377036895969,-2.08430526037572,-2.07957252906431,
-2.07661229050696,-2.07429374131368,-2.07171495030411,-2.06743310510509,
-2.05094095163634,-1.98909488659044,-1.97979259054865,-1.97726874465643,
-1.97580274176805,-1.9744989898905,-1.97276440617903,-1.96891683109184,
-1.94091340271781,-1.89126325847109,-1.88208288643013,-1.87849833832595,
-1.87631303482458,-1.87396273849936,-1.87078471944681,-1.86349400104512,
-1.85349661124895,-1.80717375464674,-1.78198557872692,-1.7788037541961,
-1.77717648193925,-1.77588320504334,-1.7743464246059,-1.77149650921252,
-1.75500620911808,-1.69592313324971,-1.68389686184406,-1.67990947750519,
-1.67739542005782,-1.67505895586755,-1.67196503480076,-1.66514559041506,
-1.63685336161741,-1.59902673518337,-1.58261252315578,-1.5799077788609,
-1.57823975519537,-1.57694370123558,-1.57543773093574,-1.57273073884975,
-1.5592303819701,-1.52665110341384,-1.48726192284892,-1.48252798105792,
-1.47956720277366,-1.47724836684289,-1.47466939688573,-1.47038758219181,
-1.45389970584968,-1.39211166860824,-1.3827544126248,-1.38022496419106,
-1.37875753431934,-1.37745344989107,-1.37571989915154,-1.37188101517732,
-1.36662266732064,-1.35267808394763,-1.30495527656979,-1.28706433057526,
-1.28253825140109,-1.27987872429951,-1.27756978354487,-1.27472896091304,
-1.26922600650835,-1.22641655877088,-1.21637204632693),.UNSPECIFIED.);
#610=B_SPLINE_CURVE_WITH_KNOTS('',3,(#53519,#53520,#53521,#53522,#53523,
#53524),.UNSPECIFIED.,.F.,.F.,(4,1,1,4),(-4.09157007060747,-3.98048681065136,
-2.98536510798852,-2.06680503374274),.UNSPECIFIED.);
#611=B_SPLINE_CURVE_WITH_KNOTS('',3,(#53528,#53529,#53530,#53531,#53532),
 .UNSPECIFIED.,.F.,.F.,(4,1,4),(0.,0.995121702662836,1.11662023360664),
 .UNSPECIFIED.);
#612=B_SPLINE_CURVE_WITH_KNOTS('',3,(#53534,#53535,#53536,#53537,#53538,
#53539,#53540,#53541,#53542,#53543,#53544,#53545,#53546,#53547,#53548,#53549,
#53550,#53551,#53552,#53553,#53554,#53555,#53556,#53557,#53558,#53559,#53560,
#53561,#53562,#53563,#53564,#53565,#53566,#53567,#53568,#53569,#53570,#53571,
#53572,#53573,#53574,#53575,#53576,#53577,#53578,#53579,#53580,#53581,#53582,
#53583,#53584,#53585,#53586,#53587,#53588,#53589,#53590,#53591,#53592,#53593,
#53594,#53595,#53596,#53597,#53598,#53599,#53600,#53601,#53602,#53603,#53604,
#53605,#53606,#53607,#53608,#53609,#53610,#53611,#53612,#53613,#53614,#53615,
#53616,#53617,#53618,#53619,#53620,#53621,#53622,#53623,#53624,#53625,#53626,
#53627,#53628,#53629,#53630,#53631,#53632,#53633,#53634,#53635,#53636,#53637,
#53638,#53639,#53640,#53641,#53642,#53643,#53644,#53645,#53646,#53647,#53648,
#53649,#53650,#53651,#53652,#53653,#53654,#53655,#53656,#53657,#53658,#53659,
#53660,#53661,#53662,#53663,#53664,#53665,#53666,#53667,#53668,#53669,#53670,
#53671,#53672,#53673,#53674,#53675,#53676,#53677,#53678,#53679,#53680,#53681,
#53682,#53683,#53684,#53685,#53686,#53687,#53688,#53689,#53690,#53691,#53692,
#53693,#53694,#53695,#53696,#53697,#53698,#53699,#53700,#53701,#53702,#53703,
#53704,#53705,#53706,#53707,#53708,#53709,#53710,#53711,#53712,#53713,#53714,
#53715,#53716,#53717,#53718,#53719,#53720,#53721,#53722,#53723),
 .UNSPECIFIED.,.F.,.F.,(4,3,3,3,3,3,3,3,3,3,3,3,3,3,3,3,3,3,3,3,3,3,3,3,
3,3,3,3,3,3,3,3,3,3,3,3,3,3,3,3,3,3,3,3,3,3,3,3,3,3,3,3,3,3,3,3,3,3,3,3,
3,3,3,4),(1.11662023360664,1.21406248760952,1.31136251306232,1.40858355403428,
1.50575826510081,1.60291922999088,1.70016613702826,1.79745265447162,1.8949147603219,
1.99024340532568,2.0900809264776,2.18977589743065,2.28935514905995,2.38887084056714,
2.4883532496785,2.58783261362238,2.68740727963367,2.78702701630181,2.88682420965512,
2.98536510798852,3.08525785857347,3.18501169700715,3.28465506891586,3.3842380426777,
3.48379080751166,3.58334351505092,3.68299577388001,3.78269553538725,3.88257601633546,
3.98048681065136,4.08009956575734,4.17956843680165,4.27907344636572,4.37836158923314,
4.47761636387469,4.57686832789242,4.67655337424787,4.77594858235294,4.87577854783357,
4.9756085133142,5.07535894551674,5.17496719232404,5.27446071472182,5.37389132531015,
5.47328942836856,5.57268538835164,5.67219659525799,5.77173596693952,5.87145546527129,
5.97073021597704,6.07047695669942,6.17008183754323,6.26957250648138,6.36900057641264,
6.46839645591088,6.56779051402169,6.66730586517624,6.76684415007728,6.86656306647563,
6.96585191863989,7.0743403241005,7.18223019824974,7.29101786936603,7.39980554048232),
 .UNSPECIFIED.);
#613=B_SPLINE_CURVE_WITH_KNOTS('',3,(#53725,#53726,#53727,#53728,#53729,
#53730,#53731,#53732,#53733,#53734,#53735,#53736,#53737,#53738,#53739,#53740,
#53741,#53742,#53743,#53744,#53745,#53746,#53747,#53748,#53749,#53750,#53751,
#53752,#53753,#53754,#53755,#53756,#53757,#53758,#53759,#53760,#53761,#53762,
#53763,#53764,#53765,#53766,#53767,#53768,#53769,#53770,#53771,#53772,#53773,
#53774,#53775,#53776,#53777,#53778,#53779,#53780,#53781,#53782,#53783,#53784,
#53785,#53786,#53787,#53788,#53789,#53790,#53791,#53792,#53793,#53794,#53795,
#53796,#53797,#53798,#53799,#53800,#53801,#53802,#53803,#53804,#53805,#53806,
#53807,#53808,#53809,#53810,#53811,#53812,#53813,#53814,#53815,#53816,#53817,
#53818,#53819,#53820,#53821,#53822,#53823,#53824,#53825,#53826,#53827,#53828,
#53829,#53830,#53831,#53832,#53833,#53834,#53835,#53836,#53837,#53838,#53839,
#53840,#53841,#53842,#53843,#53844,#53845,#53846,#53847,#53848,#53849,#53850,
#53851,#53852,#53853,#53854,#53855,#53856,#53857,#53858,#53859,#53860,#53861,
#53862,#53863,#53864,#53865,#53866,#53867,#53868,#53869,#53870,#53871,#53872,
#53873,#53874,#53875,#53876,#53877,#53878,#53879,#53880,#53881,#53882,#53883,
#53884,#53885,#53886,#53887,#53888,#53889,#53890,#53891,#53892,#53893,#53894,
#53895,#53896,#53897,#53898,#53899,#53900,#53901,#53902,#53903,#53904,#53905,
#53906,#53907,#53908,#53909,#53910,#53911,#53912,#53913,#53914,#53915,#53916,
#53917),.UNSPECIFIED.,.F.,.F.,(4,3,3,3,3,3,3,3,3,3,3,3,3,3,3,3,3,3,3,3,
3,3,3,3,3,3,3,3,3,3,3,3,3,3,3,3,3,3,3,3,3,3,3,3,3,3,3,3,3,3,3,3,3,3,3,3,
3,3,3,3,3,3,3,3,4),(7.39980554078624,7.50151138056856,7.60328677665983,
7.7052395287897,7.80729009445515,7.90955145809102,7.96097362130273,8.06070626983946,
8.16029669361446,8.25977242032754,8.35918526010481,8.45856564232094,8.5579439565598,
8.65748179841125,8.75700390142675,8.85670650664603,8.95609532396558,9.05582580586708,
9.15541407968061,9.25488944804909,9.3543001957416,9.4536785121954,9.55305479000452,
9.6525953491605,9.75211550952065,9.85181624478125,9.95121702662841,10.0509435670901,
10.1505278213335,10.2500041848282,10.3494107525505,10.4487848377975,10.548156838838,
10.6477023114513,10.7472181266395,10.8469145096764,10.9463387292913,11.0460680233656,
11.145655070275,11.2451307404849,11.3445401750104,11.4439171485967,11.5432920555783,
11.6428341496723,11.7423528843177,11.842052171866,11.9414604319541,12.0411892223499,
12.1407757642195,12.2402515605191,12.3396604905676,12.4390369610488,12.5384113670061,
12.6379540589088,12.7374723028274,12.8371711097881,12.936582134617,13.035137737167,
13.1335648679788,13.2318955025576,13.3301614969694,13.4284230365986,13.5266798090921,
13.6250124709493,13.6829908479658),.UNSPECIFIED.);
#614=B_SPLINE_CURVE_WITH_KNOTS('',3,(#53919,#53920,#53921,#53922,#53923,
#53924,#53925,#53926,#53927,#53928,#53929,#53930,#53931,#53932,#53933,#53934,
#53935,#53936,#53937,#53938,#53939,#53940,#53941,#53942,#53943,#53944,#53945,
#53946,#53947,#53948,#53949,#53950,#53951,#53952,#53953,#53954,#53955,#53956,
#53957,#53958,#53959,#53960,#53961,#53962,#53963,#53964,#53965,#53966,#53967,
#53968,#53969,#53970,#53971,#53972,#53973,#53974,#53975,#53976,#53977,#53978,
#53979,#53980,#53981,#53982,#53983,#53984,#53985,#53986,#53987,#53988,#53989,
#53990,#53991,#53992,#53993,#53994,#53995,#53996,#53997,#53998,#53999,#54000,
#54001,#54002,#54003,#54004,#54005,#54006,#54007,#54008,#54009,#54010,#54011,
#54012,#54013,#54014,#54015,#54016,#54017,#54018,#54019,#54020,#54021,#54022,
#54023,#54024,#54025,#54026,#54027,#54028,#54029,#54030,#54031,#54032,#54033,
#54034,#54035,#54036,#54037,#54038,#54039,#54040,#54041,#54042,#54043,#54044,
#54045,#54046,#54047,#54048,#54049,#54050,#54051,#54052,#54053,#54054,#54055,
#54056,#54057,#54058,#54059,#54060,#54061,#54062,#54063,#54064,#54065,#54066,
#54067,#54068,#54069,#54070,#54071,#54072,#54073,#54074,#54075,#54076,#54077,
#54078,#54079,#54080,#54081,#54082,#54083,#54084,#54085,#54086,#54087,#54088,
#54089,#54090,#54091,#54092,#54093,#54094,#54095,#54096,#54097,#54098,#54099,
#54100,#54101,#54102,#54103,#54104,#54105,#54106,#54107,#54108),
 .UNSPECIFIED.,.F.,.F.,(4,3,3,3,3,3,3,3,3,3,3,3,3,3,3,3,3,3,3,3,3,3,3,3,
3,3,3,3,3,3,3,3,3,3,3,3,3,3,3,3,3,3,3,3,3,3,3,3,3,3,3,3,3,3,3,3,3,3,3,3,
3,3,3,4),(13.6829908483353,13.8119049794007,13.9317038372798,14.031432564536,
14.1310190394365,14.2304948519997,14.3299037062129,14.4292800976703,14.5286544215113,
14.6281972011191,14.7277153561338,14.8274140707772,14.9268255399426,15.0265541732415,
15.1261405535332,15.2256163896673,15.3250251484058,15.4244014442795,15.5237756725604,
15.6233185650717,15.7228366255694,15.8225352470782,15.9219472426055,16.0216758307429,
16.1212621647812,16.2207380123421,16.320146722509,16.4195229690432,16.5188971472824,
16.6184400967789,16.717958106017,16.8176566759335,16.9170689452683,17.0167975829567,
17.1163839673222,17.2158598023983,17.3152685644057,17.4146448632355,17.5140190941541,
17.6135619825984,17.713080044921,17.8127786677469,17.9121906479311,18.011919269849,
18.111505638297,18.2109814773342,18.3103902231869,18.4097665058091,18.5091407204898,
18.6086836280159,18.7082016741926,18.8079002810564,18.907312350594,19.0070409683728,
19.1066273325613,19.2061031726482,19.3055119139792,19.4048881919906,19.5042624019773,
19.6038053147972,19.7033233561234,19.8030219580802,19.9024340532568,19.9661761551454),
 .UNSPECIFIED.);
#615=B_SPLINE_CURVE_WITH_KNOTS('',3,(#54110,#54111,#54112,#54113,#54114,
#54115,#54116,#54117,#54118,#54119,#54120,#54121,#54122,#54123,#54124,#54125,
#54126,#54127,#54128,#54129,#54130,#54131,#54132,#54133,#54134,#54135,#54136,
#54137,#54138,#54139,#54140,#54141,#54142,#54143,#54144,#54145,#54146,#54147,
#54148,#54149,#54150,#54151,#54152,#54153,#54154,#54155,#54156,#54157,#54158,
#54159,#54160,#54161,#54162,#54163,#54164,#54165,#54166,#54167,#54168,#54169,
#54170,#54171,#54172,#54173,#54174,#54175,#54176,#54177,#54178,#54179,#54180,
#54181,#54182,#54183,#54184,#54185,#54186,#54187,#54188,#54189,#54190,#54191,
#54192,#54193,#54194,#54195,#54196,#54197,#54198,#54199,#54200,#54201,#54202,
#54203,#54204,#54205,#54206,#54207,#54208,#54209,#54210,#54211,#54212,#54213,
#54214,#54215,#54216,#54217,#54218,#54219,#54220,#54221,#54222,#54223,#54224,
#54225,#54226,#54227,#54228,#54229,#54230,#54231,#54232,#54233,#54234,#54235,
#54236,#54237,#54238,#54239,#54240,#54241,#54242,#54243,#54244,#54245,#54246,
#54247,#54248,#54249,#54250,#54251,#54252,#54253,#54254,#54255,#54256,#54257,
#54258,#54259,#54260,#54261,#54262,#54263,#54264,#54265,#54266,#54267,#54268,
#54269,#54270,#54271,#54272,#54273,#54274,#54275,#54276,#54277,#54278,#54279,
#54280,#54281,#54282,#54283,#54284,#54285,#54286,#54287,#54288,#54289,#54290,
#54291,#54292,#54293,#54294,#54295,#54296,#54297,#54298,#54299,#54300,#54301,
#54302),.UNSPECIFIED.,.F.,.F.,(4,3,3,3,3,3,3,3,3,3,3,3,3,3,3,3,3,3,3,3,
3,3,3,3,3,3,3,3,3,3,3,3,3,3,3,3,3,3,3,3,3,3,3,3,3,3,3,3,3,3,3,3,3,3,3,3,
3,3,3,3,3,3,3,3,4),(19.9661761555181,20.0649597355301,20.1636079450829,
20.2621527857533,20.3606432135408,20.4591107687241,20.5575869594835,20.656164904063,
20.7548007419313,20.8535976761377,20.8975557559197,20.9972843776227,21.0968707458138,
21.1963465849099,21.2957553304038,21.3951316126294,21.4945058268761,21.5940487348027,
21.6935667804576,21.7932653867505,21.8926774585825,21.9924060799964,22.0919924478857,
22.1914682870557,22.29087703222,22.3902533141063,22.4896275280042,22.5891704363145,
22.6886884816009,22.7883870875165,22.8877991612453,22.9875277834658,23.0871141521756,
23.1865899911422,23.2859987371549,23.3853750198979,23.48474923466,23.5842921419721,
23.6838101881323,23.7835087949203,23.8829208639082,23.982649485756,24.0822358540888,
24.1817116931491,24.2811204387762,24.3804967211317,24.4798709355044,24.5794138432711,
24.6789318890418,24.7786304954433,24.878042566571,24.9777711884159,25.0773575567441,
25.1768333958053,25.2762421414259,25.3756184237736,25.4749926381377,25.5745355459117,
25.6740535916712,25.7737521980603,25.8731642692339,25.9856807881721,26.0977868859121,
26.2091942719789,26.2493614621018),.UNSPECIFIED.);
#616=B_SPLINE_CURVE_WITH_KNOTS('',3,(#54304,#54305,#54306,#54307,#54308,
#54309,#54310,#54311,#54312,#54313,#54314,#54315,#54316,#54317,#54318,#54319,
#54320,#54321,#54322,#54323,#54324,#54325,#54326,#54327,#54328,#54329,#54330,
#54331,#54332,#54333,#54334,#54335,#54336,#54337,#54338,#54339,#54340,#54341,
#54342,#54343,#54344,#54345,#54346,#54347,#54348,#54349,#54350,#54351,#54352,
#54353,#54354,#54355,#54356,#54357,#54358,#54359,#54360,#54361,#54362,#54363,
#54364,#54365,#54366,#54367,#54368,#54369,#54370,#54371,#54372,#54373,#54374,
#54375,#54376,#54377,#54378,#54379,#54380,#54381,#54382,#54383,#54384,#54385,
#54386,#54387,#54388,#54389,#54390,#54391,#54392,#54393,#54394,#54395,#54396,
#54397,#54398,#54399,#54400,#54401,#54402,#54403,#54404,#54405,#54406,#54407,
#54408,#54409,#54410,#54411,#54412,#54413,#54414,#54415,#54416,#54417,#54418,
#54419,#54420,#54421,#54422,#54423,#54424,#54425,#54426,#54427,#54428,#54429,
#54430,#54431,#54432,#54433,#54434,#54435,#54436,#54437,#54438,#54439,#54440,
#54441,#54442,#54443,#54444,#54445,#54446,#54447,#54448,#54449,#54450,#54451,
#54452,#54453,#54454,#54455,#54456,#54457,#54458,#54459,#54460,#54461,#54462,
#54463,#54464,#54465,#54466,#54467,#54468,#54469,#54470,#54471,#54472,#54473,
#54474,#54475,#54476,#54477,#54478,#54479,#54480,#54481,#54482,#54483,#54484,
#54485,#54486,#54487,#54488,#54489,#54490,#54491,#54492,#54493,#54494,#54495,
#54496),.UNSPECIFIED.,.F.,.F.,(4,3,3,3,3,3,3,3,3,3,3,3,3,3,3,3,3,3,3,3,
3,3,3,3,3,3,3,3,3,3,3,3,3,3,3,3,3,3,3,3,3,3,3,3,3,3,3,3,3,3,3,3,3,3,3,3,
3,3,3,3,3,3,3,3,4),(26.249361462325,26.3495432146859,26.4497399602872,26.5543764631896,
26.6547586687675,26.7552256738968,26.8558647706909,26.8682859718967,26.9680145937861,
27.0676009621604,27.1670768012103,27.2664855468789,27.3658618292753,27.4652360436889,
27.5647789514065,27.6642969972169,27.7639956036571,27.8634076745596,27.9631362964534,
28.0627226648318,28.1621985038807,28.2616072495533,28.3609835319537,28.4603577463712,
28.559900654084,28.659418699898,28.7591173063415,28.8585293772224,28.9582579991278,
29.0578443675181,29.157320206564,29.2567289522489,29.3561052346618,29.4554794490917,
29.5550223567901,29.6545404026167,29.754239009073,29.8536510798852,29.9533797017831,
30.0529660701657,30.1524419092135,30.2518506548906,30.3512269372956,30.4506011517176,
30.5501440594253,30.6496621052439,30.7493607116922,30.8487727825481,30.9485014044471,
31.048087772831,31.1475636118785,31.2469723575565,31.3463486399627,31.4457228543857,
31.545265762092,31.6447838079117,31.7444824143612,31.8438944852109,31.9431350382334,
32.0422407490315,32.1412428341483,32.2401841982582,32.3390858292702,32.4380241896836,
32.5325467695046),.UNSPECIFIED.);
#617=B_SPLINE_CURVE_WITH_KNOTS('',3,(#54498,#54499,#54500,#54501,#54502,
#54503,#54504,#54505,#54506,#54507,#54508,#54509,#54510,#54511,#54512,#54513,
#54514,#54515,#54516,#54517,#54518,#54519,#54520,#54521,#54522,#54523,#54524,
#54525,#54526,#54527,#54528,#54529,#54530,#54531,#54532,#54533,#54534,#54535,
#54536,#54537,#54538,#54539,#54540,#54541,#54542,#54543,#54544,#54545,#54546,
#54547,#54548,#54549,#54550,#54551,#54552,#54553,#54554,#54555,#54556,#54557,
#54558,#54559,#54560,#54561,#54562,#54563,#54564,#54565,#54566,#54567,#54568,
#54569,#54570,#54571,#54572,#54573,#54574,#54575,#54576,#54577,#54578,#54579,
#54580,#54581,#54582,#54583,#54584,#54585,#54586,#54587,#54588,#54589,#54590,
#54591,#54592,#54593,#54594,#54595,#54596,#54597,#54598,#54599,#54600,#54601,
#54602,#54603,#54604,#54605,#54606,#54607,#54608,#54609,#54610,#54611,#54612,
#54613,#54614,#54615,#54616,#54617,#54618,#54619,#54620,#54621,#54622,#54623,
#54624,#54625,#54626,#54627,#54628,#54629,#54630,#54631,#54632,#54633,#54634,
#54635,#54636,#54637,#54638,#54639,#54640,#54641,#54642,#54643,#54644,#54645,
#54646,#54647,#54648,#54649,#54650,#54651,#54652,#54653,#54654,#54655,#54656,
#54657,#54658,#54659,#54660,#54661,#54662,#54663,#54664,#54665,#54666,#54667,
#54668,#54669,#54670,#54671,#54672,#54673,#54674,#54675,#54676,#54677,#54678,
#54679,#54680,#54681,#54682,#54683,#54684,#54685,#54686,#54687,#54688,#54689,
#54690),.UNSPECIFIED.,.F.,.F.,(4,3,3,3,3,3,3,3,3,3,3,3,3,3,3,3,3,3,3,3,
3,3,3,3,3,3,3,3,3,3,3,3,3,3,3,3,3,3,3,3,3,3,3,3,3,3,3,3,3,3,3,3,3,3,3,3,
3,3,3,3,3,3,3,3,4),(32.5325467698621,32.6510766728329,32.7711063593354,
32.8390161878737,32.9387448097729,33.038331178157,33.1378070172045,33.237215762883,
33.3365920452893,33.4359662597127,33.5355091674187,33.6350272132388,33.7347258196885,
33.8341378905366,33.9338665124361,34.0334528808205,34.1329287198679,34.2323374655466,
34.3317137479533,34.4310879623771,34.5306308700827,34.6301489159031,34.7298475223531,
34.8292595931994,34.9289882150991,35.0285745834837,35.128050422531,35.2274591682099,
35.3268354506168,35.4262096650407,35.5257525727461,35.6252706185667,35.7249692250169,
35.8243812958623,35.9241099177618,36.0236962861461,36.1231721251935,36.2225808708722,
36.3219571532788,36.4213313677026,36.5208742754082,36.6203923212285,36.7200909276785,
36.8195029985251,36.9192316204247,37.0188179888092,37.1182938278566,37.2177025735354,
37.3170788559422,37.4164530703661,37.5159959780715,37.615514023892,37.7152126303422,
37.814624701188,37.9143533230875,38.013939691472,38.1134155305193,38.2128242761981,
38.3122005586049,38.4115747730288,38.5111176807343,38.6106357265547,38.7103343330047,
38.8097464038508,38.8157320766842),.UNSPECIFIED.);
#618=B_SPLINE_CURVE_WITH_KNOTS('',3,(#54692,#54693,#54694,#54695,#54696,
#54697,#54698,#54699,#54700,#54701,#54702,#54703,#54704,#54705,#54706,#54707,
#54708,#54709,#54710,#54711,#54712,#54713,#54714,#54715,#54716,#54717,#54718,
#54719,#54720,#54721,#54722,#54723,#54724,#54725,#54726,#54727,#54728,#54729,
#54730,#54731,#54732,#54733,#54734,#54735,#54736,#54737,#54738,#54739,#54740,
#54741,#54742,#54743,#54744,#54745,#54746,#54747,#54748,#54749,#54750,#54751,
#54752,#54753,#54754,#54755,#54756,#54757,#54758,#54759,#54760,#54761,#54762,
#54763,#54764,#54765,#54766,#54767,#54768,#54769,#54770,#54771,#54772,#54773,
#54774,#54775,#54776,#54777,#54778,#54779,#54780,#54781,#54782,#54783,#54784,
#54785,#54786,#54787,#54788,#54789,#54790,#54791,#54792,#54793,#54794,#54795,
#54796,#54797,#54798,#54799,#54800,#54801,#54802,#54803,#54804,#54805,#54806,
#54807,#54808,#54809,#54810,#54811,#54812,#54813,#54814,#54815,#54816,#54817,
#54818,#54819,#54820,#54821,#54822,#54823,#54824,#54825,#54826,#54827,#54828,
#54829,#54830,#54831,#54832,#54833,#54834,#54835,#54836,#54837,#54838,#54839,
#54840,#54841,#54842,#54843,#54844,#54845,#54846,#54847,#54848,#54849,#54850,
#54851,#54852,#54853,#54854,#54855,#54856,#54857,#54858,#54859,#54860,#54861,
#54862,#54863,#54864,#54865,#54866,#54867,#54868,#54869,#54870,#54871,#54872,
#54873,#54874,#54875,#54876,#54877,#54878,#54879,#54880,#54881),
 .UNSPECIFIED.,.F.,.F.,(4,3,3,3,3,3,3,3,3,3,3,3,3,3,3,3,3,3,3,3,3,3,3,3,
3,3,3,3,3,3,3,3,3,3,3,3,3,3,3,3,3,3,3,3,3,3,3,3,3,3,3,3,3,3,3,3,3,3,3,3,
3,3,3,4),(38.8157320770262,38.9153542708244,39.0148343426844,39.1142001341494,
39.2135034514798,39.3127748761239,39.4120449501345,39.5114128104276,39.610827763068,
39.7104214250461,39.8048681065136,39.9045967284132,40.0041830967977,40.103658935845,
40.2030676815239,40.3024439639307,40.4018181783547,40.5013610860602,40.6008791318807,
40.7005777383308,40.7999898091765,40.8997184310759,40.9993047994602,41.0987806385076,
41.1981893841863,41.2975656665931,41.396939881017,41.4964827887225,41.5960008345429,
41.6956994409929,41.7951115118393,41.8948401337389,41.9944265021234,42.0939023411707,
42.1933110868495,42.2926873692563,42.3920615836801,42.4916044913856,42.5911225372061,
42.6908211436562,42.7902332145022,42.8899618364017,42.9895482047862,43.0890240438336,
43.1884327895123,43.2878090719191,43.3871832863429,43.4867261940484,43.586244239869,
43.6859428463191,43.785354917165,43.8850835390646,43.9846699074492,44.0841457464966,
44.1835544921752,44.282930774582,44.3823049890059,44.4818478967114,44.5813659425318,
44.6810645489819,44.7804766198279,44.899085633739,45.0164064706586,45.0989173834712),
 .UNSPECIFIED.);
#619=B_SPLINE_CURVE_WITH_KNOTS('',3,(#54883,#54884,#54885,#54886,#54887,
#54888,#54889,#54890,#54891,#54892,#54893,#54894,#54895,#54896,#54897,#54898,
#54899,#54900,#54901,#54902,#54903,#54904,#54905,#54906,#54907,#54908,#54909,
#54910,#54911,#54912,#54913,#54914,#54915,#54916,#54917,#54918,#54919,#54920,
#54921,#54922,#54923,#54924,#54925,#54926,#54927,#54928,#54929,#54930,#54931,
#54932,#54933,#54934,#54935,#54936,#54937,#54938,#54939,#54940,#54941,#54942,
#54943,#54944,#54945,#54946,#54947,#54948,#54949,#54950,#54951,#54952,#54953,
#54954,#54955,#54956,#54957,#54958,#54959,#54960,#54961,#54962,#54963,#54964,
#54965,#54966,#54967,#54968,#54969,#54970,#54971,#54972,#54973,#54974,#54975,
#54976,#54977,#54978,#54979,#54980,#54981,#54982,#54983,#54984,#54985,#54986,
#54987,#54988,#54989,#54990,#54991,#54992,#54993,#54994,#54995,#54996,#54997,
#54998,#54999,#55000,#55001,#55002,#55003,#55004,#55005,#55006,#55007,#55008,
#55009,#55010,#55011,#55012,#55013,#55014,#55015,#55016,#55017,#55018,#55019,
#55020,#55021,#55022,#55023,#55024,#55025,#55026,#55027,#55028,#55029,#55030,
#55031,#55032,#55033,#55034,#55035,#55036,#55037,#55038,#55039,#55040,#55041,
#55042,#55043,#55044,#55045,#55046,#55047,#55048,#55049,#55050,#55051,#55052,
#55053,#55054,#55055,#55056,#55057,#55058,#55059,#55060,#55061,#55062,#55063,
#55064,#55065,#55066,#55067,#55068,#55069,#55070,#55071,#55072,#55073,#55074,
#55075),.UNSPECIFIED.,.F.,.F.,(4,3,3,3,3,3,3,3,3,3,3,3,3,3,3,3,3,3,3,3,
3,3,3,3,3,3,3,3,3,3,3,3,3,3,3,3,3,3,3,3,3,3,3,3,3,3,3,3,3,3,3,3,3,3,3,3,
3,3,3,3,3,3,3,3,4),(45.0989173838638,45.1980218083953,45.2971017503985,
45.3961879153463,45.4953804966537,45.5946271163157,45.6940543865298,45.7755983224907,
45.8753269443902,45.9749133127746,46.0743891518219,46.1737978975007,46.2731741799074,
46.3725483943313,46.4720913020368,46.5716093478572,46.6713079543073,46.7707200251535,
46.870448647053,46.9700350154376,47.0695108544849,47.1689196001637,47.2682958825704,
47.3676700969942,47.4672130046997,47.5667310505201,47.6664296569702,47.7658417278164,
47.865570349716,47.9651567181005,48.0646325571478,48.1640413028266,48.2634175852335,
48.3627917996575,48.4623347073629,48.5618527531833,48.6615513596333,48.7609634304792,
48.8606920523788,48.9602784207636,49.0597542598109,49.1591630054897,49.2585392878962,
49.35791350232,49.4574564100255,49.5569744558458,49.6566730622959,49.7560851331421,
49.8558137550418,49.955400123426,50.0548759624733,50.1542847081522,50.2536609905587,
50.3530352049826,50.4525781126882,50.5520961585087,50.6517947649588,50.7512068358049,
50.8515389897043,50.9517252562119,51.0517952162203,51.1517736522124,51.2516994680995,
51.3516134530358,51.3821026910434),.UNSPECIFIED.);
#620=B_SPLINE_CURVE_WITH_KNOTS('',3,(#55077,#55078,#55079,#55080,#55081,
#55082,#55083,#55084,#55085,#55086,#55087,#55088,#55089,#55090,#55091,#55092,
#55093,#55094,#55095,#55096,#55097,#55098,#55099,#55100,#55101,#55102,#55103,
#55104,#55105,#55106,#55107,#55108,#55109,#55110,#55111,#55112,#55113,#55114,
#55115,#55116,#55117,#55118,#55119,#55120,#55121,#55122,#55123,#55124,#55125,
#55126,#55127,#55128,#55129,#55130,#55131,#55132,#55133,#55134,#55135,#55136,
#55137,#55138,#55139,#55140,#55141,#55142,#55143,#55144,#55145,#55146,#55147,
#55148,#55149,#55150,#55151,#55152,#55153,#55154,#55155,#55156,#55157,#55158,
#55159,#55160,#55161,#55162,#55163,#55164,#55165,#55166,#55167,#55168,#55169,
#55170,#55171,#55172,#55173,#55174,#55175,#55176,#55177,#55178,#55179,#55180,
#55181,#55182,#55183,#55184,#55185,#55186,#55187,#55188,#55189,#55190,#55191,
#55192,#55193,#55194,#55195,#55196,#55197,#55198,#55199,#55200,#55201,#55202,
#55203,#55204,#55205,#55206,#55207,#55208,#55209,#55210,#55211,#55212,#55213,
#55214,#55215,#55216,#55217,#55218,#55219,#55220,#55221,#55222,#55223,#55224,
#55225,#55226,#55227,#55228,#55229,#55230,#55231,#55232,#55233,#55234,#55235,
#55236,#55237,#55238,#55239,#55240,#55241,#55242,#55243,#55244,#55245,#55246,
#55247,#55248,#55249,#55250,#55251,#55252,#55253,#55254,#55255,#55256,#55257,
#55258,#55259,#55260,#55261,#55262,#55263,#55264,#55265,#55266,#55267,#55268,
#55269),.UNSPECIFIED.,.F.,.F.,(4,3,3,3,3,3,3,3,3,3,3,3,3,3,3,3,3,3,3,3,
3,3,3,3,3,3,3,3,3,3,3,3,3,3,3,3,3,3,3,3,3,3,3,3,3,3,3,3,3,3,3,3,3,3,3,3,
3,3,3,3,3,3,3,3,4),(51.38210269127,51.494631253354,51.6077050198739,51.721416463853,
51.7463285384677,51.8460571603673,51.9456435287518,52.0451193677992,52.1445281134779,
52.2439043958847,52.3432786103086,52.4428215180141,52.5423395638346,52.6420381702847,
52.7414502411306,52.8411788630301,52.9407652314146,53.0402410704619,53.1396498161407,
53.2390260985474,53.3384003129713,53.4379432206768,53.5374612664973,53.6371598729474,
53.7365719437934,53.836300565693,53.9358869340774,54.0353627731248,54.1347715188035,
54.2341478012102,54.3335220156341,54.4330649233396,54.5325829691601,54.6322815756102,
54.7316936464563,54.8314222683558,54.9310086367403,55.0304844757877,55.1298932214664,
55.2292695038732,55.328643718297,55.4281866260025,55.527704671823,55.6274032782731,
55.7268153491191,55.8265439710186,55.9261303394031,56.0256061784504,56.1250149241292,
56.2243912065359,56.3237654209597,56.4233083286653,56.5228263744857,56.6225249809357,
56.7219370517819,56.8208847371964,56.9196908790247,57.0183844674433,57.1170176925836,
57.2156219572361,57.3142286261182,57.4129302438207,57.5116840268029,57.6105975209941,
57.6652879978908),.UNSPECIFIED.);
#621=B_SPLINE_CURVE_WITH_KNOTS('',3,(#55271,#55272,#55273,#55274,#55275,
#55276,#55277,#55278,#55279,#55280,#55281,#55282,#55283,#55284,#55285,#55286,
#55287,#55288,#55289,#55290,#55291,#55292,#55293,#55294,#55295,#55296,#55297,
#55298,#55299,#55300,#55301,#55302,#55303,#55304,#55305,#55306,#55307,#55308,
#55309,#55310,#55311,#55312,#55313,#55314,#55315,#55316,#55317,#55318,#55319,
#55320,#55321,#55322,#55323,#55324,#55325,#55326,#55327,#55328,#55329,#55330,
#55331,#55332,#55333,#55334,#55335,#55336,#55337,#55338,#55339,#55340,#55341,
#55342,#55343,#55344,#55345,#55346,#55347,#55348,#55349,#55350,#55351,#55352,
#55353,#55354,#55355,#55356,#55357,#55358,#55359,#55360,#55361,#55362,#55363,
#55364,#55365,#55366,#55367,#55368,#55369,#55370,#55371,#55372,#55373,#55374,
#55375,#55376,#55377,#55378,#55379,#55380,#55381,#55382,#55383,#55384,#55385,
#55386,#55387,#55388,#55389,#55390,#55391,#55392,#55393,#55394,#55395,#55396,
#55397,#55398,#55399,#55400,#55401,#55402,#55403,#55404,#55405,#55406,#55407,
#55408,#55409,#55410,#55411,#55412,#55413,#55414,#55415,#55416,#55417,#55418,
#55419,#55420,#55421,#55422,#55423,#55424,#55425,#55426,#55427,#55428,#55429,
#55430,#55431,#55432,#55433,#55434,#55435,#55436,#55437,#55438,#55439,#55440,
#55441,#55442,#55443,#55444,#55445,#55446,#55447,#55448,#55449,#55450,#55451,
#55452,#55453,#55454,#55455,#55456,#55457,#55458,#55459,#55460),
 .UNSPECIFIED.,.F.,.F.,(4,3,3,3,3,3,3,3,3,3,3,3,3,3,3,3,3,3,3,3,3,3,3,3,
3,3,3,3,3,3,3,3,3,3,3,3,3,3,3,3,3,3,3,3,3,3,3,3,3,3,3,3,3,3,3,3,3,3,3,3,
3,3,3,4),(57.665287998223,57.7170587544448,57.8167873763444,57.916373744729,
58.0158495837763,58.1152583294552,58.2146346118619,58.3140088262859,58.4135517339914,
58.5130697798119,58.612768386262,58.7121804571076,58.8119090790072,58.9114954473916,
59.0109712864389,59.1103800321177,59.2097563145245,59.3091305289483,59.4086734366539,
59.5081914824743,59.6078900889244,59.7073021597705,59.80703078167,59.9066171500545,
60.0060929891018,60.1055017347806,60.2048780171873,60.3042522316111,60.4037951393166,
60.503313185137,60.6030117915871,60.7024238624333,60.8021524843328,60.9017388527173,
61.0012146917646,61.1006234374434,61.1999997198501,61.2993739342739,61.3989168419794,
61.4984348877999,61.5981334942499,61.6975455650961,61.7972741869957,61.8968605553802,
61.9963363944276,62.0957451401064,62.1951214225132,62.2944956369371,62.3940385446426,
62.4935565904631,62.5932551969132,62.692667267759,62.7923958896585,62.8919822580429,
62.9914580970903,63.090866842769,63.1902431251756,63.2896173395995,63.389160247305,
63.4886782931254,63.5883768995755,63.6877889704218,63.8181311377544,63.9484733050871),
 .UNSPECIFIED.);
#622=B_SPLINE_CURVE_WITH_KNOTS('',3,(#55462,#55463,#55464,#55465,#55466,
#55467,#55468,#55469,#55470,#55471,#55472,#55473,#55474,#55475,#55476,#55477,
#55478,#55479,#55480,#55481,#55482,#55483,#55484,#55485,#55486,#55487,#55488,
#55489,#55490,#55491,#55492,#55493,#55494,#55495,#55496,#55497,#55498,#55499,
#55500,#55501,#55502,#55503,#55504,#55505,#55506,#55507,#55508,#55509,#55510,
#55511,#55512,#55513,#55514,#55515,#55516,#55517,#55518,#55519,#55520,#55521,
#55522,#55523,#55524,#55525,#55526,#55527,#55528,#55529,#55530,#55531,#55532,
#55533,#55534,#55535,#55536,#55537,#55538,#55539,#55540,#55541,#55542,#55543,
#55544,#55545,#55546,#55547,#55548,#55549,#55550,#55551,#55552,#55553,#55554,
#55555,#55556,#55557,#55558,#55559,#55560,#55561,#55562,#55563,#55564,#55565,
#55566,#55567,#55568,#55569,#55570,#55571,#55572,#55573,#55574,#55575,#55576,
#55577,#55578,#55579,#55580,#55581,#55582,#55583,#55584,#55585,#55586,#55587,
#55588,#55589,#55590,#55591,#55592,#55593,#55594,#55595,#55596,#55597,#55598,
#55599,#55600,#55601,#55602,#55603,#55604,#55605,#55606,#55607,#55608,#55609,
#55610,#55611,#55612,#55613,#55614,#55615,#55616,#55617,#55618,#55619,#55620,
#55621,#55622,#55623,#55624,#55625,#55626,#55627,#55628,#55629,#55630,#55631,
#55632,#55633,#55634,#55635,#55636,#55637,#55638,#55639,#55640,#55641,#55642,
#55643,#55644,#55645,#55646,#55647,#55648,#55649,#55650,#55651,#55652,#55653,
#55654),.UNSPECIFIED.,.F.,.F.,(4,3,3,3,3,3,3,3,3,3,3,3,3,3,3,3,3,3,3,3,
3,3,3,3,3,3,3,3,3,3,3,3,3,3,3,3,3,3,3,3,3,3,3,3,3,3,3,3,3,3,3,3,3,3,3,3,
3,3,3,3,3,3,3,3,4),(63.9484733054025,64.0469016666163,64.1452752386828,
64.2436256686098,64.3419845708388,64.440445668635,64.5389646754106,64.6376460323145,
64.6829106730847,64.7826392949843,64.8822256633687,64.9817015024161,65.0811102480948,
65.1804865305015,65.2798607449253,65.3794036526308,65.4789216984512,65.5786203049012,
65.6780323757475,65.777760997647,65.8773473660316,65.9768232050789,66.0762319507576,
66.1756082331642,66.274982447588,66.3745253552936,66.4740434011141,66.5737420075641,
66.6731540784104,66.77288270031,66.8724690686947,66.9719449077421,67.0713536534208,
67.1707299358277,67.2701041502517,67.3696470579571,67.4691651037777,67.5688637102279,
67.6682757810732,67.7680044029727,67.8675907713569,67.9670666104043,68.0664753560831,
68.1658516384898,68.2652258529134,68.3647687606191,68.4642868064395,68.5639854128896,
68.663397483736,68.7631261056355,68.8627124740203,68.9621883130676,69.0615970587463,
69.1609733411528,69.2603475555769,69.3598904632824,69.4594085091028,69.5591071155529,
69.6585191863989,69.760413026184,69.8621421786056,69.963700362568,70.0651579293423,
70.1665318849402,70.2316586125821),.UNSPECIFIED.);
#623=B_SPLINE_CURVE_WITH_KNOTS('',3,(#55656,#55657,#55658,#55659,#55660,
#55661,#55662,#55663,#55664,#55665,#55666,#55667,#55668,#55669,#55670,#55671,
#55672,#55673,#55674,#55675,#55676,#55677,#55678,#55679,#55680,#55681,#55682,
#55683,#55684,#55685,#55686,#55687,#55688,#55689,#55690,#55691,#55692,#55693,
#55694,#55695,#55696,#55697,#55698,#55699,#55700,#55701,#55702,#55703,#55704,
#55705,#55706,#55707,#55708,#55709,#55710,#55711,#55712,#55713,#55714,#55715,
#55716,#55717,#55718,#55719,#55720,#55721,#55722,#55723,#55724,#55725,#55726,
#55727,#55728,#55729,#55730,#55731,#55732,#55733,#55734,#55735,#55736,#55737,
#55738,#55739,#55740,#55741,#55742,#55743,#55744,#55745,#55746,#55747,#55748,
#55749,#55750,#55751,#55752,#55753,#55754,#55755,#55756,#55757,#55758,#55759,
#55760,#55761,#55762,#55763,#55764,#55765,#55766,#55767,#55768,#55769,#55770,
#55771,#55772,#55773,#55774,#55775,#55776,#55777,#55778,#55779,#55780,#55781,
#55782,#55783,#55784,#55785,#55786,#55787,#55788,#55789,#55790,#55791,#55792,
#55793,#55794,#55795,#55796,#55797,#55798,#55799,#55800,#55801,#55802,#55803,
#55804,#55805,#55806,#55807,#55808,#55809,#55810,#55811,#55812,#55813,#55814,
#55815,#55816,#55817,#55818,#55819,#55820,#55821,#55822,#55823,#55824,#55825,
#55826,#55827,#55828,#55829,#55830,#55831,#55832,#55833,#55834,#55835,#55836,
#55837,#55838,#55839,#55840,#55841,#55842,#55843,#55844,#55845),
 .UNSPECIFIED.,.F.,.F.,(4,3,3,3,3,3,3,3,3,3,3,3,3,3,3,3,3,3,3,3,3,3,3,3,
3,3,3,3,3,3,3,3,3,3,3,3,3,3,3,3,3,3,3,3,3,3,3,3,3,3,3,3,3,3,3,3,3,3,3,3,
3,3,3,4),(70.2316586129268,70.3398756418851,70.4483885887339,70.5573687920858,
70.6536408890617,70.7533695109613,70.8529558793459,70.9524317183932,71.051840464072,
71.1512167464788,71.2505909609028,71.3501338686082,71.4496519144287,71.5493505208788,
71.6487625917246,71.7484912136241,71.8480775820085,71.9475534210559,72.0469621667347,
72.1463384491414,72.2457126635652,72.3452555712707,72.4447736170912,72.5444722235412,
72.6438842943874,72.7436129162869,72.8431992846713,72.9426751237187,73.0420838693974,
73.1414601518041,73.2408343662279,73.3403772739335,73.4398953197539,73.5395939262039,
73.6390059970502,73.7387346189498,73.8383209873343,73.9377968263817,74.0372055720605,
74.1365818544673,74.2359560688912,74.3354989765967,74.4350170224171,74.5347156288673,
74.6341276997131,74.7338563216126,74.833442689997,74.9329185290444,75.0323272747231,
75.1317035571298,75.2310777715536,75.3306206792592,75.4301387250796,75.5298373315296,
75.6292494023759,75.7276742477903,75.8260704567589,75.9242418456712,76.0223541015018,
76.1204391481535,76.2190403409999,76.3172158795948,76.4160298995669,76.5148439195389),
 .UNSPECIFIED.);
#624=B_SPLINE_CURVE_WITH_KNOTS('',3,(#55847,#55848,#55849,#55850,#55851,
#55852,#55853,#55854,#55855,#55856,#55857,#55858,#55859,#55860,#55861,#55862,
#55863,#55864,#55865,#55866,#55867,#55868,#55869,#55870,#55871,#55872,#55873,
#55874,#55875,#55876,#55877,#55878,#55879,#55880,#55881,#55882,#55883,#55884,
#55885,#55886,#55887,#55888,#55889,#55890,#55891,#55892,#55893,#55894,#55895,
#55896,#55897,#55898,#55899,#55900,#55901,#55902,#55903,#55904,#55905,#55906,
#55907,#55908,#55909,#55910,#55911,#55912,#55913,#55914,#55915,#55916,#55917,
#55918,#55919,#55920,#55921,#55922,#55923,#55924,#55925,#55926,#55927,#55928,
#55929,#55930,#55931,#55932,#55933,#55934,#55935,#55936,#55937,#55938,#55939,
#55940,#55941,#55942,#55943,#55944,#55945,#55946,#55947,#55948,#55949,#55950,
#55951,#55952,#55953,#55954,#55955,#55956,#55957,#55958,#55959,#55960,#55961,
#55962,#55963,#55964,#55965,#55966,#55967,#55968,#55969,#55970,#55971,#55972,
#55973,#55974,#55975,#55976,#55977,#55978,#55979,#55980,#55981,#55982,#55983,
#55984,#55985,#55986,#55987,#55988,#55989,#55990,#55991,#55992,#55993,#55994,
#55995,#55996,#55997,#55998,#55999,#56000,#56001,#56002,#56003,#56004,#56005,
#56006,#56007,#56008,#56009,#56010,#56011,#56012,#56013,#56014,#56015,#56016,
#56017,#56018,#56019,#56020,#56021,#56022,#56023,#56024,#56025,#56026,#56027,
#56028,#56029,#56030,#56031,#56032,#56033,#56034,#56035,#56036),
 .UNSPECIFIED.,.F.,.F.,(4,3,3,3,3,3,3,3,3,3,3,3,3,3,3,3,3,3,3,3,3,3,3,3,
3,3,3,3,3,3,3,3,3,3,3,3,3,3,3,3,3,3,3,3,3,3,3,3,3,3,3,3,3,3,3,3,3,3,3,3,
3,3,3,4),(76.5148439197617,76.6243711050387,76.7240997269381,76.8236860953223,
76.9231619343697,77.0225706800483,77.1219469624549,77.2213211768786,77.3208640845843,
77.4203821304046,77.5200807368545,77.6194928077016,77.7192214296011,77.8188077979855,
77.9182836370329,78.0176923827116,78.1170686651182,78.216442879542,78.3159857872476,
78.415503833068,78.5152024395181,78.6146145103644,78.714343132264,78.8139295006486,
78.913405339696,79.0128140853748,79.1121903677816,79.2115645822056,79.311107489911,
79.4106255357315,79.5103241421817,79.6097362130273,79.7094648349268,79.8090512033113,
79.9085270423586,80.0079357880374,80.1073120704441,80.2066862848679,80.3062291925735,
80.4057472383939,80.5054458448439,80.6048579156901,80.7045865375896,80.8041729059741,
80.9036487450215,81.0030574907002,81.1024337731069,81.2018079875307,81.3013508952363,
81.4008689410567,81.5005675475068,81.599979618353,81.6997082402526,81.7992946086371,
81.8987704476845,81.9981791933633,82.0975554757701,82.1969296901939,82.2964725978994,
82.3959906437198,82.49568925017,82.5951013210158,82.7361481116942,82.7980292269413),
 .UNSPECIFIED.);
#625=B_SPLINE_CURVE_WITH_KNOTS('',3,(#56038,#56039,#56040,#56041,#56042,
#56043,#56044,#56045,#56046,#56047,#56048,#56049,#56050,#56051,#56052,#56053,
#56054,#56055,#56056,#56057,#56058,#56059,#56060,#56061,#56062,#56063,#56064,
#56065,#56066,#56067,#56068,#56069,#56070,#56071,#56072,#56073,#56074,#56075,
#56076,#56077,#56078,#56079,#56080,#56081,#56082,#56083,#56084,#56085,#56086,
#56087,#56088,#56089,#56090,#56091,#56092,#56093,#56094,#56095,#56096,#56097,
#56098,#56099,#56100,#56101,#56102,#56103,#56104,#56105,#56106,#56107,#56108,
#56109,#56110,#56111,#56112,#56113,#56114,#56115,#56116,#56117,#56118,#56119,
#56120,#56121,#56122,#56123,#56124,#56125,#56126,#56127,#56128,#56129,#56130,
#56131,#56132,#56133,#56134,#56135,#56136,#56137,#56138,#56139,#56140,#56141,
#56142,#56143,#56144,#56145,#56146,#56147,#56148,#56149,#56150,#56151,#56152,
#56153,#56154,#56155,#56156,#56157,#56158,#56159,#56160,#56161,#56162,#56163,
#56164,#56165,#56166,#56167,#56168,#56169,#56170,#56171,#56172,#56173,#56174,
#56175,#56176,#56177,#56178,#56179,#56180,#56181,#56182,#56183,#56184,#56185,
#56186,#56187,#56188,#56189,#56190,#56191,#56192,#56193,#56194,#56195,#56196,
#56197,#56198,#56199,#56200,#56201,#56202,#56203,#56204,#56205,#56206,#56207,
#56208,#56209,#56210,#56211,#56212,#56213,#56214,#56215,#56216,#56217,#56218,
#56219,#56220,#56221,#56222,#56223,#56224,#56225,#56226,#56227),
 .UNSPECIFIED.,.F.,.F.,(4,3,3,3,3,3,3,3,3,3,3,3,3,3,3,3,3,3,3,3,3,3,3,3,
3,3,3,3,3,3,3,3,3,3,3,3,3,3,3,3,3,3,3,3,3,3,3,3,3,3,3,3,3,3,3,3,3,3,3,3,
3,3,3,4),(82.7980292272367,82.8970534517919,82.9950894977502,83.0930789271652,
83.1910537466629,83.2908460659168,83.3889446960583,83.4895838598685,83.5902230236787,
83.6899516455782,83.7895380139627,83.88901385301,83.9884225986888,84.0877988810955,
84.1871730955195,84.286716003225,84.3862340490455,84.4859326554956,84.5853447263415,
84.6850733482411,84.7846597166256,84.8841355556729,84.9835443013518,85.0829205837586,
85.1822947981825,85.2818377058879,85.3813557517083,85.4810543581584,85.5804664290043,
85.6801950509038,85.7797814192885,85.8792572583358,85.9786660040146,86.0780422864214,
86.1774165008454,86.2769594085509,86.3764774543713,86.4761760608214,86.5755881316672,
86.6753167535667,86.7749031219511,86.8743789609985,86.9737877066772,87.0731639890841,
87.1725382035081,87.2720811112135,87.3715991570341,87.4712977634842,87.57070983433,
87.6704384562295,87.7700248246142,87.8695006636615,87.9689094093401,88.0682856917468,
88.1676599061707,88.2672028138763,88.3667208596967,88.4664194661467,88.5658315369929,
88.6698572087964,88.7736129224715,88.877209535948,88.9806129425655,89.0812145341209),
 .UNSPECIFIED.);
#626=B_SPLINE_CURVE_WITH_KNOTS('',3,(#56229,#56230,#56231,#56232,#56233,
#56234,#56235,#56236,#56237,#56238,#56239,#56240,#56241,#56242,#56243,#56244,
#56245,#56246,#56247,#56248,#56249,#56250,#56251,#56252,#56253,#56254,#56255,
#56256,#56257,#56258,#56259,#56260,#56261,#56262,#56263,#56264,#56265,#56266,
#56267,#56268,#56269,#56270,#56271,#56272,#56273,#56274,#56275,#56276,#56277,
#56278,#56279,#56280,#56281,#56282,#56283,#56284,#56285,#56286,#56287,#56288,
#56289,#56290,#56291,#56292,#56293,#56294,#56295,#56296,#56297,#56298,#56299,
#56300,#56301,#56302,#56303,#56304,#56305,#56306,#56307,#56308,#56309,#56310,
#56311,#56312,#56313,#56314,#56315,#56316,#56317,#56318,#56319,#56320,#56321,
#56322,#56323,#56324,#56325,#56326,#56327,#56328,#56329,#56330,#56331,#56332,
#56333,#56334,#56335,#56336,#56337,#56338,#56339,#56340,#56341,#56342,#56343,
#56344,#56345,#56346,#56347,#56348,#56349,#56350,#56351,#56352,#56353,#56354,
#56355,#56356,#56357,#56358,#56359,#56360,#56361,#56362,#56363,#56364,#56365,
#56366,#56367,#56368,#56369,#56370,#56371,#56372,#56373,#56374,#56375,#56376,
#56377,#56378,#56379,#56380,#56381,#56382,#56383,#56384,#56385,#56386,#56387,
#56388,#56389,#56390,#56391,#56392,#56393,#56394,#56395,#56396,#56397,#56398,
#56399,#56400,#56401,#56402,#56403,#56404,#56405,#56406,#56407,#56408,#56409,
#56410,#56411,#56412,#56413,#56414,#56415,#56416,#56417,#56418,#56419,#56420,
#56421),.UNSPECIFIED.,.F.,.F.,(4,3,3,3,3,3,3,3,3,3,3,3,3,3,3,3,3,3,3,3,
3,3,3,3,3,3,3,3,3,3,3,3,3,3,3,3,3,3,3,3,3,3,3,3,3,3,3,3,3,3,3,3,3,3,3,3,
3,3,3,3,3,3,3,3,4),(89.0812145344922,89.1860740166197,89.2912565031786,
89.3966087067022,89.5022553233101,89.5609532396557,89.6606818615553,89.7602682299397,
89.8597440689871,89.9591528146659,90.0585290970726,90.1579033114963,90.2574462192019,
90.3569642650223,90.4566628714724,90.5560749423185,90.655803564218,90.7553899326024,
90.8548657716498,90.9542745173286,91.0536507997353,91.1530250141591,91.2525679218647,
91.352085967685,91.4517845741351,91.5511966449814,91.6509252668809,91.7505116352654,
91.8499874743128,91.9493962199916,92.0487725023983,92.1481467168222,92.2476896245277,
92.3472076703481,92.4469062767982,92.5463183476442,92.6460469695437,92.7456333379281,
92.8451091769755,92.9445179226543,93.043894205061,93.1432684194848,93.2428113271904,
93.3423293730108,93.4420279794608,93.541440050307,93.6411686722065,93.7407550405911,
93.8402308796384,93.9396396253172,94.039015907724,94.1383901221479,94.2379330298534,
94.3374510756738,94.4371496821239,94.5365617529699,94.6348132263263,94.7329006641366,
94.8308961695538,94.9288319032292,95.0267399465123,95.1246969666554,95.2226815253506,
95.3207833079917,95.3643998409918),.UNSPECIFIED.);
#627=B_SPLINE_CURVE_WITH_KNOTS('',3,(#56423,#56424,#56425,#56426,#56427,
#56428,#56429,#56430,#56431,#56432,#56433,#56434,#56435,#56436,#56437,#56438,
#56439,#56440,#56441,#56442,#56443,#56444,#56445,#56446,#56447,#56448,#56449,
#56450,#56451,#56452,#56453,#56454,#56455,#56456,#56457,#56458,#56459,#56460,
#56461,#56462,#56463,#56464,#56465,#56466,#56467,#56468,#56469,#56470,#56471,
#56472,#56473,#56474,#56475,#56476,#56477,#56478,#56479,#56480,#56481,#56482,
#56483,#56484,#56485,#56486,#56487,#56488,#56489,#56490,#56491,#56492,#56493,
#56494,#56495,#56496,#56497,#56498,#56499,#56500,#56501,#56502,#56503,#56504,
#56505,#56506,#56507,#56508,#56509,#56510,#56511,#56512,#56513,#56514,#56515,
#56516,#56517,#56518,#56519,#56520,#56521,#56522,#56523,#56524,#56525,#56526,
#56527,#56528,#56529,#56530,#56531,#56532,#56533,#56534,#56535,#56536,#56537,
#56538,#56539,#56540,#56541,#56542,#56543,#56544,#56545,#56546,#56547,#56548,
#56549,#56550,#56551,#56552,#56553,#56554,#56555,#56556,#56557,#56558,#56559,
#56560,#56561,#56562,#56563,#56564,#56565,#56566,#56567,#56568,#56569,#56570,
#56571,#56572,#56573,#56574,#56575,#56576,#56577,#56578,#56579,#56580,#56581,
#56582,#56583,#56584,#56585,#56586,#56587,#56588,#56589,#56590,#56591,#56592,
#56593,#56594,#56595,#56596,#56597,#56598,#56599,#56600,#56601,#56602,#56603,
#56604,#56605,#56606,#56607,#56608,#56609,#56610,#56611,#56612),
 .UNSPECIFIED.,.F.,.F.,(4,3,3,3,3,3,3,3,3,3,3,3,3,3,3,3,3,3,3,3,3,3,3,3,
3,3,3,3,3,3,3,3,3,3,3,3,3,3,3,3,3,3,3,3,3,3,3,3,3,3,3,3,3,3,3,3,3,3,3,3,
3,3,3,4),(95.3643998413005,95.5209226988385,95.5316834556327,95.6314120775325,
95.730998445917,95.8304742849643,95.9298830306433,96.0292593130502,96.1286335274742,
96.2281764351796,96.3276944810002,96.4273930874506,96.5268051582956,96.626533780195,
96.7261201485794,96.8255959876268,96.9250047333054,97.024381015712,97.1237552301357,
97.2232981378414,97.3228161836617,97.4225147901116,97.5219268609584,97.6216554828579,
97.7212418512424,97.8207176902898,97.9201264359686,98.0195027183753,98.1188769327992,
98.2184198405047,98.3179378863252,98.4176364927753,98.5170485636213,98.6167771855208,
98.7163635539053,98.8158393929527,98.9152481386314,99.0146244210382,99.113998635462,
99.2135415431676,99.313059588988,99.4127581954381,99.5121702662841,99.6118988881836,
99.711485256568,99.8109610956154,99.9103698412941,100.009746123701,100.109120338125,
100.20866324583,100.308181291651,100.407879898101,100.507291968947,100.607020590847,
100.706606959231,100.806082798279,100.905491543958,101.004867826364,101.104242040788,
101.203784948494,101.303302994314,101.403001600765,101.50241367161,101.64758514848),
 .UNSPECIFIED.);
#628=B_SPLINE_CURVE_WITH_KNOTS('',3,(#56614,#56615,#56616,#56617,#56618,
#56619,#56620,#56621,#56622,#56623,#56624,#56625,#56626,#56627,#56628,#56629,
#56630,#56631,#56632,#56633,#56634,#56635,#56636,#56637,#56638,#56639,#56640,
#56641,#56642,#56643,#56644,#56645,#56646,#56647,#56648,#56649,#56650,#56651,
#56652,#56653,#56654,#56655,#56656,#56657,#56658,#56659,#56660,#56661,#56662,
#56663,#56664,#56665,#56666,#56667,#56668,#56669,#56670,#56671,#56672,#56673,
#56674,#56675,#56676,#56677,#56678,#56679,#56680,#56681,#56682,#56683,#56684,
#56685,#56686,#56687,#56688,#56689,#56690,#56691,#56692,#56693,#56694,#56695,
#56696,#56697,#56698,#56699,#56700,#56701,#56702,#56703,#56704,#56705,#56706,
#56707,#56708,#56709,#56710,#56711,#56712,#56713,#56714,#56715,#56716,#56717,
#56718,#56719,#56720,#56721,#56722,#56723,#56724,#56725,#56726,#56727,#56728,
#56729,#56730,#56731,#56732,#56733,#56734,#56735,#56736,#56737,#56738,#56739,
#56740,#56741,#56742,#56743,#56744,#56745,#56746,#56747,#56748,#56749,#56750,
#56751,#56752,#56753,#56754,#56755,#56756,#56757,#56758,#56759,#56760,#56761,
#56762,#56763,#56764,#56765,#56766,#56767,#56768,#56769,#56770,#56771,#56772,
#56773,#56774,#56775,#56776,#56777,#56778,#56779,#56780,#56781,#56782,#56783,
#56784,#56785,#56786,#56787,#56788,#56789,#56790,#56791,#56792,#56793,#56794,
#56795,#56796,#56797,#56798,#56799,#56800,#56801,#56802,#56803,#56804,#56805,
#56806),.UNSPECIFIED.,.F.,.F.,(4,3,3,3,3,3,3,3,3,3,3,3,3,3,3,3,3,3,3,3,
3,3,3,3,3,3,3,3,3,3,3,3,3,3,3,3,3,3,3,3,3,3,3,3,3,3,3,3,3,3,3,3,3,3,3,3,
3,3,3,3,3,3,3,3,4),(101.647585148862,101.745752943682,101.843798677613,
101.941778175553,102.039723508507,102.137666700871,102.235703069986,102.333788608231,
102.432039269302,102.497535374273,102.597263996172,102.696850364556,102.796326203604,
102.895734949282,102.995111231688,103.094485446112,103.194028353818,103.293546399638,
103.393245006088,103.492657076935,103.592385698834,103.691972067219,103.791447906266,
103.890856651945,103.990232934352,104.089607148775,104.189150056481,104.288668102301,
104.388366708751,104.487778779598,104.587507401498,104.687093769882,104.78656960893,
104.885978354609,104.985354637016,105.08472885144,105.184271759145,105.283789804966,
105.383488411416,105.482900482261,105.58262910416,105.682215472545,105.781691311592,
105.881100057271,105.980476339678,106.079850554102,106.179393461807,106.278911507628,
106.378610114078,106.478022184924,106.577750806823,106.677337175208,106.776813014255,
106.876221759934,106.975598042341,107.074972256764,107.17451516447,107.274033210291,
107.373731816741,107.473143887587,107.580031519542,107.686559866531,107.792861004934,
107.898852412545,107.930770455256),.UNSPECIFIED.);
#629=B_SPLINE_CURVE_WITH_KNOTS('',3,(#56808,#56809,#56810,#56811,#56812,
#56813,#56814,#56815,#56816,#56817,#56818,#56819,#56820,#56821,#56822,#56823,
#56824,#56825,#56826,#56827,#56828,#56829,#56830,#56831,#56832,#56833,#56834,
#56835,#56836,#56837,#56838,#56839,#56840,#56841,#56842,#56843,#56844,#56845,
#56846,#56847,#56848,#56849,#56850,#56851,#56852,#56853,#56854,#56855,#56856,
#56857,#56858,#56859,#56860,#56861,#56862,#56863,#56864,#56865,#56866,#56867,
#56868,#56869,#56870,#56871,#56872,#56873,#56874,#56875,#56876,#56877,#56878,
#56879,#56880,#56881,#56882,#56883,#56884,#56885,#56886,#56887,#56888,#56889,
#56890,#56891,#56892,#56893,#56894,#56895,#56896,#56897,#56898,#56899,#56900,
#56901,#56902,#56903,#56904,#56905,#56906,#56907,#56908,#56909,#56910,#56911,
#56912,#56913,#56914,#56915,#56916,#56917,#56918,#56919,#56920,#56921,#56922,
#56923,#56924,#56925,#56926,#56927,#56928,#56929,#56930,#56931,#56932,#56933,
#56934,#56935,#56936,#56937,#56938,#56939,#56940,#56941,#56942,#56943,#56944,
#56945,#56946,#56947,#56948,#56949,#56950,#56951,#56952,#56953,#56954,#56955,
#56956,#56957,#56958,#56959,#56960,#56961,#56962,#56963,#56964,#56965,#56966,
#56967,#56968,#56969,#56970,#56971,#56972,#56973,#56974,#56975,#56976,#56977,
#56978,#56979,#56980,#56981,#56982,#56983,#56984,#56985,#56986,#56987,#56988,
#56989,#56990,#56991,#56992,#56993,#56994,#56995,#56996,#56997,#56998,#56999,
#57000),.UNSPECIFIED.,.F.,.F.,(4,3,3,3,3,3,3,3,3,3,3,3,3,3,3,3,3,3,3,3,
3,3,3,3,3,3,3,3,3,3,3,3,3,3,3,3,3,3,3,3,3,3,3,3,3,3,3,3,3,3,3,3,3,3,3,3,
3,3,3,3,3,3,3,3,4),(107.93077045566,108.033274088848,108.135876649722,108.238684310835,
108.341609860134,108.444749596055,108.46826559025,108.56799421215,108.667580580534,
108.767056419582,108.866465165261,108.965841447667,109.065215662091,109.164758569797,
109.264276615617,109.363975222067,109.463387292913,109.563115914812,109.662702283196,
109.762178122244,109.861586867922,109.960963150329,110.060337364752,110.159880272458,
110.259398318278,110.359096924728,110.458508995575,110.558237617474,110.657823985859,
110.757299824906,110.856708570585,110.956084852992,111.055459067415,111.155001975121,
111.254520020941,111.354218627391,111.453630698238,111.553359320138,111.652945688522,
111.75242152757,111.851830273249,111.951206555656,112.05058077008,112.150123677785,
112.249641723605,112.349340330056,112.448752400901,112.5484810228,112.648067391185,
112.747543230233,112.846951975911,112.946328258318,113.045702472742,113.145245380447,
113.244763426268,113.344462032718,113.443874103564,113.542257329618,113.640513780549,
113.738675593745,113.836774785775,113.934878007869,114.032978129635,114.131171661169,
114.213955762534),.UNSPECIFIED.);
#630=B_SPLINE_CURVE_WITH_KNOTS('',3,(#57002,#57003,#57004,#57005,#57006,
#57007,#57008,#57009,#57010,#57011,#57012,#57013,#57014,#57015,#57016,#57017,
#57018,#57019,#57020,#57021,#57022,#57023,#57024,#57025,#57026,#57027,#57028,
#57029,#57030,#57031,#57032,#57033,#57034,#57035,#57036,#57037,#57038,#57039,
#57040,#57041,#57042,#57043,#57044,#57045,#57046,#57047,#57048,#57049,#57050,
#57051,#57052,#57053,#57054,#57055,#57056,#57057,#57058,#57059,#57060,#57061,
#57062,#57063,#57064,#57065,#57066,#57067,#57068,#57069,#57070,#57071,#57072,
#57073,#57074,#57075,#57076,#57077,#57078,#57079,#57080,#57081,#57082,#57083,
#57084,#57085,#57086,#57087,#57088,#57089,#57090,#57091,#57092,#57093,#57094,
#57095,#57096,#57097,#57098,#57099,#57100,#57101,#57102,#57103,#57104,#57105,
#57106,#57107,#57108,#57109,#57110,#57111,#57112,#57113,#57114,#57115,#57116,
#57117,#57118,#57119,#57120,#57121,#57122,#57123,#57124,#57125,#57126,#57127,
#57128,#57129,#57130,#57131,#57132,#57133,#57134,#57135,#57136,#57137,#57138,
#57139,#57140,#57141,#57142,#57143,#57144,#57145,#57146,#57147,#57148,#57149,
#57150,#57151,#57152,#57153,#57154,#57155,#57156,#57157,#57158,#57159,#57160,
#57161,#57162,#57163,#57164,#57165,#57166,#57167,#57168,#57169,#57170,#57171,
#57172,#57173,#57174,#57175,#57176,#57177,#57178,#57179,#57180,#57181,#57182,
#57183,#57184,#57185,#57186,#57187,#57188,#57189,#57190,#57191),
 .UNSPECIFIED.,.F.,.F.,(4,3,3,3,3,3,3,3,3,3,3,3,3,3,3,3,3,3,3,3,3,3,3,3,
3,3,3,3,3,3,3,3,3,3,3,3,3,3,3,3,3,3,3,3,3,3,3,3,3,3,3,3,3,3,3,3,3,3,3,3,
3,3,3,4),(114.213955762839,114.348406921202,114.438995806227,114.538724428126,
114.63831079651,114.737786635558,114.837195381236,114.936571663642,115.035945878065,
115.135488785772,115.235006831591,115.334705438041,115.43411750889,115.533846130789,
115.633432499173,115.732908338221,115.832317083899,115.931693366306,116.031067580729,
116.130610488435,116.230128534255,116.329827140705,116.429239211552,116.528967833451,
116.628554201836,116.728030040883,116.827438786562,116.926815068968,117.026189283392,
117.125732191097,117.225250236918,117.324948843368,117.424360914215,117.524089536115,
117.623675904501,117.723151743548,117.822560489228,117.921936771635,118.02131098606,
118.120853893765,118.220371939586,118.320070546037,118.419482616878,118.519211238777,
118.618797607161,118.718273446208,118.817682191886,118.917058474292,119.016432688716,
119.115975596422,119.215493642242,119.315192248691,119.414604319541,119.514332941439,
119.613919309822,119.713395148869,119.812803894546,119.912180176951,120.011554391374,
120.111097299081,120.2106153449,120.310313951348,120.409726022204,120.497141070019),
 .UNSPECIFIED.);
#631=B_SPLINE_CURVE_WITH_KNOTS('',3,(#57193,#57194,#57195,#57196,#57197,
#57198,#57199,#57200,#57201,#57202,#57203,#57204,#57205,#57206,#57207,#57208,
#57209,#57210,#57211,#57212,#57213,#57214,#57215,#57216,#57217,#57218,#57219,
#57220,#57221,#57222,#57223,#57224,#57225,#57226,#57227,#57228,#57229,#57230,
#57231,#57232,#57233,#57234,#57235,#57236,#57237,#57238,#57239,#57240,#57241,
#57242,#57243,#57244,#57245,#57246,#57247,#57248,#57249,#57250,#57251,#57252,
#57253,#57254,#57255,#57256,#57257,#57258,#57259,#57260,#57261,#57262,#57263,
#57264,#57265,#57266,#57267,#57268,#57269,#57270,#57271,#57272,#57273,#57274,
#57275,#57276,#57277,#57278,#57279,#57280,#57281,#57282,#57283,#57284,#57285,
#57286,#57287,#57288,#57289,#57290,#57291,#57292,#57293,#57294,#57295,#57296,
#57297,#57298,#57299,#57300,#57301,#57302,#57303,#57304,#57305,#57306,#57307,
#57308,#57309,#57310,#57311,#57312,#57313,#57314,#57315,#57316,#57317,#57318,
#57319,#57320,#57321,#57322,#57323,#57324,#57325,#57326,#57327,#57328,#57329,
#57330,#57331,#57332,#57333,#57334,#57335,#57336,#57337,#57338,#57339,#57340,
#57341,#57342,#57343,#57344,#57345,#57346,#57347,#57348,#57349,#57350,#57351,
#57352,#57353,#57354,#57355,#57356,#57357,#57358,#57359,#57360,#57361,#57362,
#57363,#57364,#57365,#57366,#57367,#57368,#57369,#57370,#57371,#57372,#57373,
#57374,#57375,#57376,#57377,#57378,#57379,#57380,#57381,#57382,#57383,#57384,
#57385),.UNSPECIFIED.,.F.,.F.,(4,3,3,3,3,3,3,3,3,3,3,3,3,3,3,3,3,3,3,3,
3,3,3,3,3,3,3,3,3,3,3,3,3,3,3,3,3,3,3,3,3,3,3,3,3,3,3,3,3,3,3,3,3,3,3,3,
3,3,3,3,3,3,3,3,4),(120.497141070234,120.595677943242,120.696824165945,
120.795132645144,120.893392568864,120.991635696353,121.094938703481,121.193304234699,
121.291735213299,121.390318471888,121.404847724867,121.50457634676,121.604162715137,
121.703638554186,121.803047299858,121.902423582258,122.001797796676,122.101340704389,
122.200858750203,122.300557356647,122.399969427529,122.499698049419,122.599284417793,
122.698760256843,122.798169002511,122.897545284908,122.996919499321,123.096462407039,
123.195980452849,123.295679059289,123.395091130192,123.494819752138,123.594406120569,
123.693881959605,123.793290705331,123.892666987784,123.992041202254,124.091584109904,
124.19110215577,124.290800762264,124.390212832855,124.489941454693,124.589527823017,
124.689003662079,124.788412407698,124.887788690045,124.987162904411,125.086705812187,
125.186223857951,125.285922464346,125.385334535518,125.485063157369,125.584649525705,
125.684125364764,125.783534110393,125.882910392748,125.982284607121,126.081827514886,
126.181345560654,126.281044167052,126.380456238181,126.49102766556,126.601262124105,
126.710922081326,126.780326376994),.UNSPECIFIED.);
#632=B_SPLINE_CURVE_WITH_KNOTS('',3,(#57387,#57388,#57389,#57390,#57391,
#57392,#57393,#57394,#57395,#57396,#57397,#57398,#57399,#57400,#57401,#57402,
#57403,#57404,#57405,#57406,#57407,#57408,#57409,#57410,#57411,#57412,#57413,
#57414,#57415,#57416,#57417,#57418,#57419,#57420,#57421,#57422,#57423,#57424,
#57425,#57426,#57427,#57428,#57429,#57430,#57431,#57432,#57433,#57434,#57435,
#57436,#57437,#57438,#57439,#57440,#57441,#57442,#57443,#57444,#57445,#57446,
#57447,#57448,#57449,#57450,#57451,#57452,#57453,#57454,#57455,#57456,#57457,
#57458,#57459,#57460,#57461,#57462,#57463,#57464,#57465,#57466,#57467,#57468,
#57469,#57470,#57471,#57472,#57473,#57474,#57475,#57476,#57477,#57478,#57479,
#57480,#57481,#57482,#57483,#57484,#57485,#57486,#57487,#57488,#57489,#57490,
#57491,#57492,#57493,#57494,#57495,#57496,#57497,#57498,#57499,#57500,#57501,
#57502,#57503,#57504,#57505,#57506,#57507,#57508,#57509,#57510,#57511,#57512,
#57513,#57514,#57515,#57516,#57517,#57518,#57519,#57520,#57521,#57522,#57523,
#57524,#57525,#57526,#57527,#57528,#57529,#57530,#57531,#57532,#57533,#57534,
#57535,#57536,#57537,#57538,#57539,#57540,#57541,#57542,#57543,#57544,#57545,
#57546,#57547,#57548,#57549,#57550,#57551,#57552,#57553,#57554,#57555,#57556,
#57557,#57558,#57559,#57560,#57561,#57562,#57563,#57564,#57565,#57566,#57567,
#57568,#57569,#57570,#57571,#57572,#57573,#57574,#57575,#57576,#57577,#57578,
#57579),.UNSPECIFIED.,.F.,.F.,(4,3,3,3,3,3,3,3,3,3,3,3,3,3,3,3,3,3,3,3,
3,3,3,3,3,3,3,3,3,3,3,3,3,3,3,3,3,3,3,3,3,3,3,3,3,3,3,3,3,3,3,3,3,3,3,3,
3,3,3,3,3,3,3,3,4),(126.780326377198,126.881078545404,126.9818657866,127.082797177342,
127.183801456351,127.285014187782,127.375577940844,127.475306562208,127.574892930058,
127.674368769239,127.773777514391,127.873153796274,127.972528010178,128.07207091851,
128.171588963827,128.271287569787,128.370699643506,128.470428265251,128.570014633474,
128.669490472561,128.768899218066,128.868275500294,128.967649714534,129.067192622443,
129.166710668072,129.266409274327,129.365821346169,129.465549970453,129.565136341231,
129.664612179681,129.764020927755,129.863397212554,129.962771429362,130.062314334229,
130.161832382391,130.261530991139,130.360943048832,130.460671666238,130.560258030133,
130.659733870304,130.759142611539,130.858518889529,130.957893099569,131.057436012551,
131.156954054111,131.256652656409,131.356064751495,131.455793373826,131.555379742598,
131.654855581543,131.754264327501,131.853640610147,131.953014824768,132.052557732116,
132.152075778033,132.25177438452,132.351186454158,132.450099816114,132.548881393724,
132.647562789345,132.746175488395,132.844770428116,132.94335698319,133.041995581221,
133.063511684378),.UNSPECIFIED.);
#633=B_SPLINE_CURVE_WITH_KNOTS('',3,(#57581,#57582,#57583,#57584,#57585,
#57586,#57587,#57588,#57589,#57590,#57591),.UNSPECIFIED.,.F.,.F.,(4,1,1,
1,1,1,1,1,4),(133.063516053725,133.346308156821,134.341429859484,135.336551562146,
136.331673264809,137.326794967472,138.321916670135,139.317038372798,139.346696991558),
 .UNSPECIFIED.);
#634=B_SPLINE_CURVE_WITH_KNOTS('',3,(#57593,#57594,#57595,#57596,#57597,
#57598,#57599,#57600,#57601,#57602,#57603,#57604,#57605,#57606,#57607,#57608,
#57609,#57610,#57611,#57612,#57613,#57614,#57615,#57616,#57617,#57618,#57619,
#57620,#57621,#57622,#57623,#57624,#57625,#57626,#57627,#57628,#57629,#57630,
#57631,#57632,#57633,#57634,#57635,#57636,#57637,#57638,#57639,#57640,#57641,
#57642,#57643,#57644,#57645,#57646,#57647,#57648,#57649,#57650,#57651,#57652,
#57653,#57654,#57655,#57656,#57657,#57658,#57659,#57660,#57661,#57662,#57663,
#57664,#57665,#57666,#57667,#57668,#57669,#57670,#57671,#57672,#57673,#57674,
#57675,#57676,#57677,#57678,#57679,#57680,#57681,#57682,#57683,#57684,#57685,
#57686,#57687,#57688,#57689,#57690,#57691,#57692,#57693,#57694,#57695,#57696,
#57697,#57698,#57699,#57700,#57701,#57702,#57703,#57704,#57705,#57706,#57707,
#57708,#57709,#57710,#57711,#57712,#57713,#57714,#57715,#57716,#57717,#57718,
#57719,#57720,#57721,#57722,#57723,#57724,#57725,#57726,#57727,#57728,#57729,
#57730,#57731,#57732,#57733,#57734,#57735,#57736,#57737,#57738,#57739,#57740,
#57741,#57742,#57743,#57744,#57745,#57746,#57747,#57748,#57749,#57750,#57751,
#57752,#57753,#57754,#57755,#57756,#57757,#57758,#57759,#57760,#57761,#57762,
#57763,#57764,#57765,#57766,#57767,#57768,#57769,#57770,#57771,#57772,#57773,
#57774,#57775,#57776,#57777,#57778,#57779,#57780,#57781,#57782),
 .UNSPECIFIED.,.F.,.F.,(4,3,3,3,3,3,3,3,3,3,3,3,3,3,3,3,3,3,3,3,3,3,3,3,
3,3,3,3,3,3,3,3,3,3,3,3,3,3,3,3,3,3,3,3,3,3,3,3,3,3,3,3,3,3,3,3,3,3,3,3,
3,3,3,4),(139.346696991558,139.445932219988,139.545026998055,139.644010661625,
139.742934364386,139.841829171499,139.940726110939,140.03972202176,140.138769074976,
140.237987522751,140.312160075461,140.411890830886,140.511479319214,140.610954626578,
140.710365444305,140.809743776229,140.909120014983,141.008660455768,141.108180444377,
141.207880929671,141.307281778123,141.40701438211,141.506604770947,141.606080477375,
141.70549330576,141.804873685462,141.904252006059,142.00378987474,142.103312005716,
142.203014651642,142.302403480786,142.402115418057,142.501685072281,142.601165086177,
142.700557167953,142.799916842311,142.899274526842,142.998837190994,143.098339064789,
143.198021841211,143.297525183449,143.39727413812,143.496880755207,143.596372432096,
143.695801067961,143.795197072117,143.894590813936,143.99410483198,144.093641727075,
144.193358620266,144.292646886112,144.392396271959,144.492003698188,144.591496744217,
144.690927087346,144.790325131506,144.889721240998,144.989233077942,145.088773106491,
145.188493561045,145.287768588775,145.403528113215,145.518253671831,145.629882298513),
 .UNSPECIFIED.);
#635=B_SPLINE_CURVE_WITH_KNOTS('',3,(#57784,#57785,#57786,#57787,#57788,
#57789,#57790,#57791,#57792,#57793,#57794,#57795,#57796,#57797,#57798,#57799,
#57800,#57801,#57802,#57803,#57804,#57805,#57806,#57807,#57808,#57809,#57810,
#57811,#57812,#57813,#57814,#57815,#57816,#57817,#57818,#57819,#57820,#57821,
#57822,#57823,#57824,#57825,#57826,#57827,#57828,#57829,#57830,#57831,#57832,
#57833,#57834,#57835,#57836,#57837,#57838,#57839,#57840,#57841,#57842,#57843,
#57844,#57845,#57846,#57847,#57848,#57849,#57850,#57851,#57852,#57853,#57854,
#57855,#57856,#57857,#57858,#57859,#57860,#57861,#57862,#57863,#57864,#57865),
 .UNSPECIFIED.,.F.,.F.,(4,3,3,3,3,3,3,3,3,3,3,3,3,3,3,3,3,3,3,3,3,3,3,3,
3,3,3,4),(145.629882298737,145.729225833863,145.828559651808,145.927914037052,
146.027388172392,146.126928281348,146.226647384157,146.282890291438,146.382800769648,
146.482568504997,146.582219937219,146.681807426266,146.78136116726,146.880911314415,
146.98055545124,147.080244052822,147.180108308869,147.2780119941,147.376723895628,
147.479230747624,147.577691171678,147.676094980091,147.774473804444,147.872859241564,
147.971339333989,148.069875915663,148.168560926324,148.196778711597),
 .UNSPECIFIED.);
#636=B_SPLINE_CURVE_WITH_KNOTS('',3,(#57869,#57870,#57871,#57872,#57873),
 .UNSPECIFIED.,.F.,.F.,(4,1,4),(-150.263377102089,-149.268255399426,-148.604832135738),
 .UNSPECIFIED.);
#637=B_SPLINE_CURVE_WITH_KNOTS('',3,(#57875,#57876,#57877,#57878,#57879,
#57880,#57881,#57882,#57883,#57884,#57885,#57886,#57887,#57888,#57889,#57890,
#57891,#57892,#57893,#57894,#57895,#57896,#57897,#57898,#57899,#57900,#57901,
#57902,#57903,#57904,#57905,#57906,#57907,#57908,#57909,#57910,#57911,#57912,
#57913,#57914,#57915,#57916,#57917,#57918,#57919,#57920,#57921,#57922,#57923,
#57924,#57925,#57926,#57927,#57928,#57929,#57930,#57931,#57932,#57933,#57934,
#57935,#57936,#57937,#57938,#57939,#57940,#57941,#57942,#57943,#57944,#57945,
#57946,#57947,#57948,#57949,#57950,#57951,#57952,#57953,#57954,#57955,#57956,
#57957,#57958,#57959,#57960,#57961,#57962,#57963,#57964,#57965,#57966,#57967,
#57968,#57969,#57970,#57971,#57972,#57973,#57974,#57975,#57976,#57977,#57978,
#57979,#57980,#57981,#57982,#57983,#57984,#57985,#57986,#57987,#57988,#57989,
#57990,#57991,#57992,#57993,#57994,#57995,#57996,#57997,#57998,#57999,#58000,
#58001,#58002,#58003,#58004,#58005,#58006,#58007,#58008,#58009,#58010,#58011,
#58012,#58013,#58014,#58015,#58016,#58017,#58018,#58019,#58020,#58021,#58022,
#58023,#58024,#58025,#58026,#58027,#58028,#58029,#58030,#58031,#58032,#58033,
#58034,#58035,#58036,#58037,#58038,#58039,#58040,#58041,#58042,#58043,#58044,
#58045,#58046,#58047,#58048,#58049,#58050,#58051,#58052,#58053,#58054,#58055,
#58056,#58057,#58058,#58059,#58060,#58061,#58062,#58063,#58064),
 .UNSPECIFIED.,.F.,.F.,(4,3,3,3,3,3,3,3,3,3,3,3,3,3,3,3,3,3,3,3,3,3,3,3,
3,3,3,3,3,3,3,3,3,3,3,3,3,3,3,3,3,3,3,3,3,3,3,3,3,3,3,3,3,3,3,3,3,3,3,3,
3,3,3,4),(-148.604831860765,-148.489732428586,-148.373417351629,-148.273133696763,
-148.173295902649,-148.073600655269,-147.974021123327,-147.87450514929,
-147.775022455839,-147.675542806154,-147.575967854218,-147.476347831078,
-147.376550353737,-147.2780119941,-147.17811920322,-147.078365323309,-146.978721908316,
-146.879138890514,-146.779586080743,-146.680033327426,-146.580381021796,
-146.480681212858,-146.380800683946,-146.282890291438,-146.183277645322,
-146.083808884829,-145.984303847822,-145.885015818526,-145.785761158351,
-145.68650930955,-145.586824129357,-145.487429037174,-145.387598812974,
-145.287768588775,-145.188018109967,-145.088409816086,-144.98891624613,
-144.889485587712,-144.790087436618,-144.69069142846,-144.591180292873,
-144.491640873192,-144.391921327373,-144.292646886112,-144.192900134702,
-144.093295242875,-143.993804562555,-143.894376481006,-143.794980589667,
-143.69558651951,-143.596071185495,-143.496532888165,-143.396813959209,
-143.297525183449,-143.198138538548,-143.098894126518,-142.999763678427,
-142.900695176485,-142.801657730765,-142.702620490327,-142.603485859914,
-142.504302501737,-142.404945286647,-142.321646828853),.UNSPECIFIED.);
#638=B_SPLINE_CURVE_WITH_KNOTS('',3,(#58066,#58067,#58068,#58069,#58070,
#58071,#58072,#58073,#58074,#58075,#58076,#58077,#58078,#58079,#58080,#58081,
#58082,#58083,#58084,#58085,#58086,#58087,#58088,#58089,#58090,#58091,#58092,
#58093,#58094,#58095,#58096,#58097,#58098,#58099,#58100,#58101,#58102,#58103,
#58104,#58105,#58106,#58107,#58108,#58109,#58110,#58111,#58112,#58113,#58114,
#58115,#58116,#58117,#58118,#58119,#58120,#58121,#58122,#58123,#58124,#58125,
#58126,#58127,#58128,#58129,#58130,#58131,#58132,#58133,#58134,#58135,#58136,
#58137,#58138,#58139,#58140,#58141,#58142,#58143,#58144,#58145,#58146,#58147,
#58148,#58149,#58150,#58151,#58152,#58153,#58154,#58155,#58156,#58157,#58158,
#58159,#58160,#58161,#58162,#58163,#58164,#58165,#58166,#58167,#58168,#58169,
#58170,#58171,#58172,#58173,#58174,#58175,#58176,#58177,#58178,#58179,#58180,
#58181,#58182,#58183,#58184,#58185,#58186,#58187,#58188,#58189,#58190,#58191,
#58192,#58193,#58194,#58195,#58196,#58197,#58198,#58199,#58200,#58201,#58202,
#58203,#58204,#58205,#58206,#58207,#58208,#58209,#58210,#58211,#58212,#58213,
#58214,#58215,#58216,#58217,#58218,#58219,#58220,#58221,#58222,#58223,#58224,
#58225,#58226,#58227,#58228,#58229,#58230,#58231,#58232,#58233,#58234,#58235,
#58236,#58237,#58238,#58239,#58240,#58241,#58242,#58243,#58244,#58245,#58246,
#58247,#58248,#58249,#58250,#58251,#58252,#58253,#58254,#58255,#58256,#58257,
#58258),.UNSPECIFIED.,.F.,.F.,(4,3,3,3,3,3,3,3,3,3,3,3,3,3,3,3,3,3,3,3,
3,3,3,3,3,3,3,3,3,3,3,3,3,3,3,3,3,3,3,3,3,3,3,3,3,3,3,3,3,3,3,3,3,3,3,3,
3,3,3,3,3,3,3,3,4),(-142.321646828558,-142.302403480786,-142.202670823123,
-142.103080390128,-142.003604654099,-141.904191804951,-141.804811413322,
-141.705433089642,-141.605895261762,-141.506373149337,-141.406670534806,
-141.307281778123,-141.207551294656,-141.107963019226,-141.008487651255,
-140.909076901832,-140.809698583607,-140.710322303991,-140.610781746858,
-140.511261584617,-140.411560847445,-140.312160075461,-140.212433538771,
-140.112849288359,-140.013372923913,-139.913966360139,-139.814592278875,
-139.715220281847,-139.615674804585,-139.516158993442,-139.416462614439,
-139.317038372798,-139.217309077004,-139.117722028356,-139.018246358578,
-138.918836922281,-138.819459946916,-138.720085038149,-138.620542946145,
-138.521024209718,-138.421324920405,-138.321916670135,-138.222187879593,
-138.12260133757,-138.023125541308,-137.923716611089,-137.824340140432,
-137.724965734292,-137.625423042587,-137.525904798474,-137.426205991313,
-137.326794967472,-137.227066614779,-137.127480520035,-137.028004613132,
-136.928596149847,-136.829220152506,-136.729846225434,-136.630302985278,
-136.53078522949,-136.4310869124,-136.331673264809,-136.209562139173,-136.089134680719,
-136.03846168399),.UNSPECIFIED.);
#639=B_SPLINE_CURVE_WITH_KNOTS('',3,(#58260,#58261,#58262,#58263,#58264,
#58265,#58266,#58267,#58268,#58269),.UNSPECIFIED.,.F.,.F.,(4,1,1,1,1,1,
1,4),(-136.038461521379,-135.336551562146,-134.341429859484,-133.346308156821,
-132.351186454158,-131.356064751495,-130.360943048832,-129.755276214199),
 .UNSPECIFIED.);
#640=B_SPLINE_CURVE_WITH_KNOTS('',3,(#58271,#58272,#58273,#58274,#58275,
#58276,#58277,#58278,#58279,#58280),.UNSPECIFIED.,.F.,.F.,(4,1,1,1,1,1,
1,4),(-129.755276214199,-129.365821346169,-128.370699643506,-127.375577940844,
-126.380456238181,-125.385334535518,-124.390212832855,-123.47209090702),
 .UNSPECIFIED.);
#641=B_SPLINE_CURVE_WITH_KNOTS('',3,(#58282,#58283,#58284,#58285,#58286,
#58287,#58288,#58289,#58290,#58291,#58292),.UNSPECIFIED.,.F.,.F.,(4,1,1,
1,1,1,1,1,4),(-123.47209090702,-123.395091130192,-122.399969427529,-121.404847724867,
-120.409726022204,-119.414604319541,-118.419482616878,-117.424360914215,
-117.18890559984),.UNSPECIFIED.);
#642=B_SPLINE_CURVE_WITH_KNOTS('',3,(#58294,#58295,#58296,#58297,#58298,
#58299,#58300,#58301,#58302,#58303),.UNSPECIFIED.,.F.,.F.,(4,1,1,1,1,1,
1,4),(-117.18890559984,-116.429239211552,-115.43411750889,-114.438995806227,
-113.443874103564,-112.448752400901,-111.453630698238,-110.905720292661),
 .UNSPECIFIED.);
#643=B_SPLINE_CURVE_WITH_KNOTS('',3,(#58305,#58306,#58307,#58308,#58309,
#58310,#58311,#58312,#58313,#58314),.UNSPECIFIED.,.F.,.F.,(4,1,1,1,1,1,
1,4),(-110.905720292661,-110.458508995575,-109.463387292913,-108.46826559025,
-107.473143887587,-106.478022184924,-105.482900482261,-104.622534985481),
 .UNSPECIFIED.);
#644=B_SPLINE_CURVE_WITH_KNOTS('',3,(#58316,#58317,#58318,#58319,#58320,
#58321,#58322,#58323,#58324,#58325,#58326),.UNSPECIFIED.,.F.,.F.,(4,1,1,
1,1,1,1,1,4),(-104.622534985481,-104.487778779598,-103.492657076935,-102.497535374273,
-101.50241367161,-100.507291968947,-99.5121702662841,-98.5170485636213,
-98.3393496783013),.UNSPECIFIED.);
#645=B_SPLINE_CURVE_WITH_KNOTS('',3,(#58328,#58329,#58330,#58331,#58332,
#58333,#58334,#58335,#58336,#58337,#58338,#58339,#58340,#58341,#58342,#58343,
#58344,#58345,#58346,#58347,#58348,#58349,#58350,#58351,#58352,#58353,#58354,
#58355,#58356,#58357,#58358,#58359,#58360,#58361,#58362,#58363,#58364,#58365,
#58366,#58367,#58368,#58369,#58370,#58371,#58372,#58373,#58374,#58375,#58376,
#58377,#58378,#58379,#58380,#58381,#58382,#58383,#58384,#58385,#58386,#58387,
#58388,#58389,#58390,#58391,#58392,#58393,#58394,#58395,#58396,#58397,#58398,
#58399,#58400,#58401,#58402,#58403,#58404,#58405,#58406,#58407,#58408,#58409,
#58410,#58411,#58412,#58413,#58414,#58415,#58416,#58417,#58418,#58419,#58420,
#58421,#58422,#58423,#58424,#58425,#58426,#58427,#58428,#58429,#58430,#58431,
#58432,#58433,#58434,#58435,#58436,#58437,#58438,#58439,#58440,#58441,#58442,
#58443,#58444,#58445,#58446,#58447,#58448,#58449,#58450,#58451,#58452,#58453,
#58454,#58455,#58456,#58457,#58458,#58459,#58460,#58461,#58462,#58463,#58464,
#58465,#58466,#58467,#58468,#58469,#58470,#58471,#58472,#58473,#58474,#58475,
#58476,#58477,#58478,#58479,#58480,#58481,#58482,#58483,#58484,#58485,#58486,
#58487,#58488,#58489,#58490,#58491,#58492,#58493,#58494,#58495,#58496,#58497,
#58498,#58499,#58500,#58501,#58502,#58503,#58504,#58505,#58506,#58507,#58508,
#58509,#58510,#58511,#58512,#58513,#58514,#58515,#58516,#58517,#58518,#58519,
#58520),.UNSPECIFIED.,.F.,.F.,(4,3,3,3,3,3,3,3,3,3,3,3,3,3,3,3,3,3,3,3,
3,3,3,3,3,3,3,3,3,3,3,3,3,3,3,3,3,3,3,3,3,3,3,3,3,3,3,3,3,3,3,3,3,3,3,3,
3,3,3,3,3,3,3,3,4),(-98.3393496783013,-98.2371718261334,-98.1391759064278,
-98.0412345205147,-97.9433155993773,-97.8453871071087,-97.7473580989926,
-97.649269359905,-97.5510258427676,-97.5219268609584,-97.4221982390589,
-97.3226118706745,-97.2231360316271,-97.1237272859484,-97.0243510035417,
-96.9249767891178,-96.8254338814122,-96.7259158355919,-96.6262172291419,
-96.5268051582956,-96.4270765363961,-96.3274901680115,-96.2280143289642,
-96.1286055832853,-96.0292293008786,-95.9298550864547,-95.8303121787492,
-95.7307941329288,-95.6310955264786,-95.5316834556327,-95.4319548337332,
-95.3323684653489,-95.2328926263015,-95.1334838806227,-95.034107598216,
-94.934733383792,-94.8351904760865,-94.735672430266,-94.6359738238159,-94.5365617529699,
-94.4368331310704,-94.3372467626859,-94.2377709236385,-94.1383621779598,
-94.0389858955531,-93.939611681129,-93.8400687734235,-93.7405507276031,
-93.640852121153,-93.541440050307,-93.4417114284074,-93.342125060023,-93.2426492209756,
-93.1432404752967,-93.04386419289,-92.9444899784661,-92.8449470707606,-92.7454290249403,
-92.6457304184902,-92.5463183476442,-92.4411448192608,-92.3362751483011,
-92.2315886854005,-92.1271417501303,-92.0561643714314),.UNSPECIFIED.);
#646=B_SPLINE_CURVE_WITH_KNOTS('',3,(#58522,#58523,#58524,#58525,#58526,
#58527,#58528,#58529,#58530,#58531,#58532,#58533,#58534,#58535,#58536,#58537,
#58538,#58539,#58540,#58541,#58542,#58543,#58544,#58545,#58546,#58547,#58548,
#58549,#58550,#58551,#58552,#58553,#58554,#58555,#58556,#58557,#58558,#58559,
#58560,#58561,#58562,#58563,#58564,#58565,#58566,#58567,#58568,#58569,#58570,
#58571,#58572,#58573,#58574,#58575,#58576,#58577,#58578,#58579,#58580,#58581,
#58582,#58583,#58584,#58585,#58586,#58587,#58588,#58589,#58590,#58591,#58592,
#58593,#58594,#58595,#58596,#58597,#58598,#58599,#58600,#58601,#58602,#58603,
#58604,#58605,#58606,#58607,#58608,#58609,#58610,#58611,#58612,#58613,#58614,
#58615,#58616,#58617,#58618,#58619,#58620,#58621,#58622,#58623,#58624,#58625,
#58626,#58627,#58628,#58629,#58630,#58631,#58632,#58633,#58634,#58635,#58636,
#58637,#58638,#58639,#58640,#58641,#58642,#58643,#58644,#58645,#58646,#58647,
#58648,#58649,#58650,#58651,#58652,#58653,#58654,#58655,#58656,#58657,#58658,
#58659,#58660,#58661,#58662,#58663,#58664,#58665,#58666,#58667,#58668,#58669,
#58670,#58671,#58672,#58673,#58674,#58675,#58676,#58677,#58678,#58679,#58680,
#58681,#58682,#58683,#58684,#58685,#58686,#58687,#58688,#58689,#58690,#58691,
#58692,#58693,#58694,#58695,#58696,#58697,#58698,#58699,#58700,#58701,#58702,
#58703,#58704,#58705,#58706,#58707,#58708,#58709,#58710,#58711,#58712,#58713,
#58714),.UNSPECIFIED.,.F.,.F.,(4,3,3,3,3,3,3,3,3,3,3,3,3,3,3,3,3,3,3,3,
3,3,3,3,3,3,3,3,3,3,3,3,3,3,3,3,3,3,3,3,3,3,3,3,3,3,3,3,3,3,3,3,3,3,3,3,
3,3,3,3,3,3,3,3,4),(-92.0561643711217,-91.9524176251218,-91.8484056440974,
-91.7442589618222,-91.6398339023725,-91.5511966449814,-91.4514680230817,
-91.3518816546971,-91.2524058156498,-91.1529970699709,-91.0536207875641,
-90.9542465731401,-90.8547036654347,-90.7551856196142,-90.655487013164,
-90.5560749423185,-90.4563463204189,-90.3567599520346,-90.2572841129873,
-90.1578753673086,-90.0584990849019,-89.9591248704779,-89.8595819627723,
-89.7600639169519,-89.6603653105018,-89.5609532396557,-89.4612246177562,
-89.3616382493717,-89.2621624103243,-89.1627536646456,-89.0633773822388,
-88.9640031678151,-88.8644602601095,-88.7649422142889,-88.6652436078388,
-88.5658315369928,-88.4661029150933,-88.3665165467089,-88.2670407076616,
-88.1676319619828,-88.0682556795761,-87.9688814651524,-87.8693385574468,
-87.7698205116263,-87.6701219051763,-87.57070983433,-87.4709812124306,-87.3713948440464,
-87.271919004999,-87.1725102593205,-87.073133976914,-86.9737597624899,-86.8742168547842,
-86.7746988089636,-86.6750002025136,-86.5755881316672,-86.4752619982512,
-86.3771456961652,-86.2791215528277,-86.181157433619,-86.079112841299,-85.9811338363746,
-85.8831260217789,-85.7850175359975,-85.7729790643388),.UNSPECIFIED.);
#647=B_SPLINE_CURVE_WITH_KNOTS('',3,(#58716,#58717,#58718,#58719,#58720,
#58721,#58722,#58723,#58724,#58725,#58726,#58727,#58728,#58729,#58730,#58731,
#58732,#58733,#58734,#58735,#58736,#58737,#58738,#58739,#58740,#58741,#58742,
#58743,#58744,#58745,#58746,#58747,#58748,#58749,#58750,#58751,#58752,#58753,
#58754,#58755,#58756,#58757,#58758,#58759,#58760,#58761,#58762,#58763,#58764,
#58765,#58766,#58767,#58768,#58769,#58770,#58771,#58772,#58773,#58774,#58775,
#58776,#58777,#58778,#58779,#58780,#58781,#58782,#58783,#58784,#58785,#58786,
#58787,#58788,#58789,#58790,#58791,#58792,#58793,#58794,#58795,#58796,#58797,
#58798,#58799,#58800,#58801,#58802,#58803,#58804,#58805,#58806,#58807,#58808,
#58809,#58810,#58811,#58812,#58813,#58814,#58815,#58816,#58817,#58818,#58819,
#58820,#58821,#58822,#58823,#58824,#58825,#58826,#58827,#58828,#58829,#58830,
#58831,#58832,#58833,#58834,#58835,#58836,#58837,#58838,#58839,#58840,#58841,
#58842,#58843,#58844,#58845,#58846,#58847,#58848,#58849,#58850,#58851,#58852,
#58853,#58854,#58855,#58856,#58857,#58858,#58859,#58860,#58861,#58862,#58863,
#58864,#58865,#58866,#58867,#58868,#58869,#58870,#58871,#58872,#58873,#58874,
#58875,#58876,#58877,#58878,#58879,#58880,#58881,#58882,#58883,#58884,#58885,
#58886,#58887,#58888,#58889,#58890,#58891,#58892,#58893,#58894,#58895,#58896,
#58897,#58898,#58899,#58900,#58901,#58902,#58903,#58904,#58905),
 .UNSPECIFIED.,.F.,.F.,(4,3,3,3,3,3,3,3,3,3,3,3,3,3,3,3,3,3,3,3,3,3,3,3,
3,3,3,3,3,3,3,3,3,3,3,3,3,3,3,3,3,3,3,3,3,3,3,3,3,3,3,3,3,3,3,3,3,3,3,3,
3,3,3,4),(-85.7729790639421,-85.628162953706,-85.5804664290043,-85.4807378071048,
-85.3811514387203,-85.281675599673,-85.1822668539941,-85.0828905715872,
-84.9835163571633,-84.8839734494578,-84.7844554036373,-84.6847567971871,
-84.5853447263415,-84.485616104442,-84.3860297360576,-84.2865538970102,
-84.1871451513315,-84.0877688689248,-83.9883946545009,-83.8888517467954,
-83.789333700975,-83.6896350945249,-83.5902230236786,-83.4904944017791,
-83.3909080333946,-83.2914321943472,-83.1920234486684,-83.0926471662617,
-82.9932729518379,-82.8937300441323,-82.7942119983119,-82.6945133918618,
-82.5951013210158,-82.4953726991163,-82.3957863307319,-82.2963104916845,
-82.1969017460058,-82.0975254635991,-81.9981512491754,-81.8986083414698,
-81.7990902956494,-81.6993916891993,-81.599979618353,-81.5002509964534,
-81.4006646280689,-81.3011887890216,-81.2017800433427,-81.102403760936,
-81.003029546512,-80.9034866388065,-80.8039685929861,-80.7042699865359,
-80.6048579156901,-80.5051292937906,-80.4055429254061,-80.3060670863588,
-80.20665834068,-80.1072820582732,-80.0079078438493,-79.9083649361438,-79.8088468903234,
-79.7091482838733,-79.6097362130273,-79.4897937567626),.UNSPECIFIED.);
#648=B_SPLINE_CURVE_WITH_KNOTS('',3,(#58907,#58908,#58909,#58910,#58911,
#58912,#58913,#58914,#58915,#58916,#58917,#58918,#58919,#58920,#58921,#58922,
#58923,#58924,#58925,#58926,#58927,#58928,#58929,#58930,#58931,#58932,#58933,
#58934,#58935,#58936,#58937,#58938,#58939,#58940,#58941,#58942,#58943,#58944,
#58945,#58946,#58947,#58948,#58949,#58950,#58951,#58952,#58953,#58954,#58955,
#58956,#58957,#58958,#58959,#58960,#58961,#58962,#58963,#58964,#58965,#58966,
#58967,#58968,#58969,#58970,#58971,#58972,#58973,#58974,#58975,#58976,#58977,
#58978,#58979,#58980,#58981,#58982,#58983,#58984,#58985,#58986,#58987,#58988,
#58989,#58990,#58991,#58992,#58993,#58994,#58995,#58996,#58997,#58998,#58999,
#59000,#59001,#59002,#59003,#59004,#59005,#59006,#59007,#59008,#59009,#59010,
#59011,#59012,#59013,#59014,#59015,#59016,#59017,#59018,#59019,#59020,#59021,
#59022,#59023,#59024,#59025,#59026,#59027,#59028,#59029,#59030,#59031,#59032,
#59033,#59034,#59035,#59036,#59037,#59038,#59039,#59040,#59041,#59042,#59043,
#59044,#59045,#59046,#59047,#59048,#59049,#59050,#59051,#59052,#59053,#59054,
#59055,#59056,#59057,#59058,#59059,#59060,#59061,#59062,#59063,#59064,#59065,
#59066,#59067,#59068,#59069,#59070,#59071,#59072,#59073,#59074,#59075,#59076,
#59077,#59078,#59079,#59080,#59081,#59082,#59083,#59084,#59085,#59086,#59087,
#59088,#59089,#59090,#59091,#59092,#59093,#59094,#59095,#59096),
 .UNSPECIFIED.,.F.,.F.,(4,3,3,3,3,3,3,3,3,3,3,3,3,3,3,3,3,3,3,3,3,3,3,3,
3,3,3,3,3,3,3,3,3,3,3,3,3,3,3,3,3,3,3,3,3,3,3,3,3,3,3,3,3,3,3,3,3,3,3,3,
3,3,3,4),(-79.4897937565462,-79.3915052515549,-79.2933497704462,-79.1952676454984,
-79.0972268719541,-78.9991954992728,-78.9010754287433,-78.8029128620371,
-78.7045773066325,-78.6146145103644,-78.5148858884649,-78.4152995200804,
-78.3158236810331,-78.2164149353542,-78.1170386529475,-78.0176644385236,
-77.9181215308181,-77.8186034849976,-77.7189048785475,-77.6194928077016,
-77.5197641858021,-77.4201778174178,-77.3207019783704,-77.2212932326916,
-77.121916950285,-77.0225427358611,-76.9229998281555,-76.8234817823351,
-76.723783175885,-76.6243711050388,-76.5246424831393,-76.4250561147545,
-76.3255802757072,-76.2261715300284,-76.1267952476215,-76.0274210331978,
-75.9278781254923,-75.8283600796719,-75.7286614732218,-75.6292494023759,
-75.5295207804764,-75.4299344120921,-75.3304585730447,-75.231049827366,
-75.1316735449592,-75.0322993305357,-74.93275642283,-74.8332383770095,-74.7335397705595,
-74.6341276997131,-74.5343990778136,-74.4348127094288,-74.3353368703815,
-74.2359281247027,-74.1365518422962,-74.0371776278724,-73.9376347201669,
-73.8381166743464,-73.7384180678963,-73.6390059970502,-73.530724223929,
-73.4227099506246,-73.3146592002585,-73.2066084498924),.UNSPECIFIED.);
#649=B_SPLINE_CURVE_WITH_KNOTS('',3,(#59098,#59099,#59100,#59101,#59102,
#59103,#59104,#59105,#59106,#59107,#59108,#59109,#59110,#59111,#59112,#59113,
#59114,#59115,#59116,#59117,#59118,#59119,#59120,#59121,#59122,#59123,#59124,
#59125,#59126,#59127,#59128,#59129,#59130,#59131,#59132,#59133,#59134,#59135,
#59136,#59137,#59138,#59139,#59140,#59141,#59142,#59143,#59144,#59145,#59146,
#59147,#59148,#59149,#59150,#59151,#59152,#59153,#59154,#59155,#59156,#59157,
#59158,#59159,#59160,#59161,#59162,#59163,#59164,#59165,#59166,#59167,#59168,
#59169,#59170,#59171,#59172,#59173,#59174,#59175,#59176,#59177,#59178,#59179,
#59180,#59181,#59182,#59183,#59184,#59185,#59186,#59187,#59188,#59189,#59190,
#59191,#59192,#59193,#59194,#59195,#59196,#59197,#59198,#59199,#59200,#59201,
#59202,#59203,#59204,#59205,#59206,#59207,#59208,#59209,#59210,#59211,#59212,
#59213,#59214,#59215,#59216,#59217,#59218,#59219,#59220,#59221,#59222,#59223,
#59224,#59225,#59226,#59227,#59228,#59229,#59230,#59231,#59232,#59233,#59234,
#59235,#59236,#59237,#59238,#59239,#59240,#59241,#59242,#59243,#59244,#59245,
#59246,#59247,#59248,#59249,#59250,#59251,#59252,#59253,#59254,#59255,#59256,
#59257,#59258,#59259,#59260,#59261,#59262,#59263,#59264,#59265,#59266,#59267,
#59268,#59269,#59270,#59271,#59272,#59273,#59274,#59275,#59276,#59277,#59278,
#59279,#59280,#59281,#59282,#59283,#59284,#59285,#59286,#59287,#59288,#59289,
#59290),.UNSPECIFIED.,.F.,.F.,(4,3,3,3,3,3,3,3,3,3,3,3,3,3,3,3,3,3,3,3,
3,3,3,3,3,3,3,3,3,3,3,3,3,3,3,3,3,3,3,3,3,3,3,3,3,3,3,3,3,3,3,3,3,3,3,3,
3,3,3,3,3,3,3,3,4),(-73.2066084495829,-73.1049365946532,-73.0031968130311,
-72.9012812821807,-72.7992691365912,-72.6970464527663,-72.6438842943874,
-72.5441556724878,-72.4445693041034,-72.345093465056,-72.2456847193772,
-72.1463084369706,-72.0469342225469,-71.9473913148413,-71.8478732690209,
-71.7481746625708,-71.6487625917245,-71.5490339698249,-71.4494476014406,
-71.3499717623932,-71.2505630167144,-71.1511867343078,-71.051812519884,
-70.9522696121784,-70.852751566358,-70.753052959908,-70.6536408890617,-70.5539122671622,
-70.4543258987778,-70.3548500597304,-70.2554413140517,-70.1560650316449,
-70.056690817221,-69.9571479095155,-69.8576298636952,-69.7579312572451,
-69.6585191863989,-69.5587905644993,-69.4592041961149,-69.3597283570676,
-69.2603196113887,-69.1609433289821,-69.0615691145583,-68.9620262068527,
-68.8625081610323,-68.7628095545821,-68.663397483736,-68.5636688618365,
-68.4640824934516,-68.3646066544043,-68.2651979087256,-68.1658216263188,
-68.0664474118948,-67.9669045041894,-67.8673864583689,-67.7676878519188,
-67.6682757810732,-67.5697064345155,-67.4712656835002,-67.3729215659591,
-67.2746422391412,-67.1763679415933,-67.0780985404751,-66.9797543738717,
-66.9234231424034),.UNSPECIFIED.);
#650=B_SPLINE_CURVE_WITH_KNOTS('',3,(#59292,#59293,#59294,#59295,#59296,
#59297,#59298,#59299,#59300,#59301,#59302,#59303,#59304,#59305,#59306,#59307,
#59308,#59309,#59310,#59311,#59312,#59313,#59314,#59315,#59316,#59317,#59318,
#59319,#59320,#59321,#59322,#59323,#59324,#59325,#59326,#59327,#59328,#59329,
#59330,#59331,#59332,#59333,#59334,#59335,#59336,#59337,#59338,#59339,#59340,
#59341,#59342,#59343,#59344,#59345,#59346,#59347,#59348,#59349,#59350,#59351,
#59352,#59353,#59354,#59355,#59356,#59357,#59358,#59359,#59360,#59361,#59362,
#59363,#59364,#59365,#59366,#59367,#59368,#59369,#59370,#59371,#59372,#59373,
#59374,#59375,#59376,#59377,#59378,#59379,#59380,#59381,#59382,#59383,#59384,
#59385,#59386,#59387,#59388,#59389,#59390,#59391,#59392,#59393,#59394,#59395,
#59396,#59397,#59398,#59399,#59400,#59401,#59402,#59403,#59404,#59405,#59406,
#59407,#59408,#59409,#59410,#59411,#59412,#59413,#59414,#59415,#59416,#59417,
#59418,#59419,#59420,#59421,#59422,#59423,#59424,#59425,#59426,#59427,#59428,
#59429,#59430,#59431,#59432,#59433,#59434,#59435,#59436,#59437,#59438,#59439,
#59440,#59441,#59442,#59443,#59444,#59445,#59446,#59447,#59448,#59449,#59450,
#59451,#59452,#59453,#59454,#59455,#59456,#59457,#59458,#59459,#59460,#59461,
#59462,#59463,#59464,#59465,#59466,#59467,#59468,#59469,#59470,#59471,#59472,
#59473,#59474,#59475,#59476,#59477,#59478,#59479,#59480,#59481),
 .UNSPECIFIED.,.F.,.F.,(4,3,3,3,3,3,3,3,3,3,3,3,3,3,3,3,3,3,3,3,3,3,3,3,
3,3,3,3,3,3,3,3,3,3,3,3,3,3,3,3,3,3,3,3,3,3,3,3,3,3,3,3,3,3,3,3,3,3,3,3,
3,3,3,4),(-66.923423141999,-66.7948298962433,-66.6731540784103,-66.5734254565109,
-66.4738390881268,-66.3743632490794,-66.2749545034008,-66.1755782209942,
-66.0762040065706,-65.9766610988649,-65.8771430530446,-65.7774444465947,
-65.6780323757475,-65.5783037538479,-65.4787173854634,-65.3792415464161,
-65.2798328007373,-65.1804565183305,-65.0810823039066,-64.9815393962011,
-64.8820213503807,-64.7823227439305,-64.6829106730847,-64.5831820511851,
-64.4835956828006,-64.3841198437533,-64.2847110980744,-64.1853348156677,
-64.0859606012438,-63.9864176935383,-63.8868996477178,-63.7872010412677,
-63.6877889704218,-63.5880603485223,-63.4884739801379,-63.3889981410905,
-63.2895893954118,-63.1902131130051,-63.0908388985813,-62.9912959908757,
-62.8917779450553,-62.7920793386053,-62.692667267759,-62.5929386458595,
-62.493352277475,-62.3938764384277,-62.2944676927489,-62.1950914103422,
-62.0957171959183,-61.9961742882127,-61.8966562423923,-61.7969576359422,
-61.6975455650961,-61.5978169431966,-61.4982305748122,-61.3987547357648,
-61.299345990086,-61.1999697076793,-61.1005954932555,-61.0010525855499,
-60.9015345397295,-60.8018359332794,-60.7024238624333,-60.6402378352238),
 .UNSPECIFIED.);
#651=B_SPLINE_CURVE_WITH_KNOTS('',3,(#59483,#59484,#59485,#59486,#59487,
#59488,#59489,#59490,#59491,#59492,#59493,#59494,#59495,#59496,#59497,#59498,
#59499,#59500,#59501,#59502,#59503,#59504,#59505,#59506,#59507,#59508,#59509,
#59510,#59511,#59512,#59513,#59514,#59515,#59516,#59517,#59518,#59519,#59520,
#59521,#59522,#59523,#59524,#59525,#59526,#59527,#59528,#59529,#59530,#59531,
#59532,#59533,#59534,#59535,#59536,#59537,#59538,#59539,#59540,#59541,#59542,
#59543,#59544,#59545,#59546,#59547,#59548,#59549,#59550,#59551,#59552,#59553,
#59554,#59555,#59556,#59557,#59558,#59559,#59560,#59561,#59562,#59563,#59564,
#59565,#59566,#59567,#59568,#59569,#59570,#59571,#59572,#59573,#59574,#59575,
#59576,#59577,#59578,#59579,#59580,#59581,#59582,#59583,#59584,#59585,#59586,
#59587,#59588,#59589,#59590,#59591,#59592,#59593,#59594,#59595,#59596,#59597,
#59598,#59599,#59600,#59601,#59602,#59603,#59604,#59605,#59606,#59607,#59608,
#59609,#59610,#59611,#59612,#59613,#59614,#59615,#59616,#59617,#59618,#59619,
#59620,#59621,#59622,#59623,#59624,#59625,#59626,#59627,#59628,#59629,#59630,
#59631,#59632,#59633,#59634,#59635,#59636,#59637,#59638,#59639,#59640,#59641,
#59642,#59643,#59644,#59645,#59646,#59647,#59648,#59649,#59650,#59651,#59652,
#59653,#59654,#59655,#59656,#59657,#59658,#59659,#59660,#59661,#59662,#59663,
#59664,#59665,#59666,#59667,#59668,#59669,#59670,#59671,#59672,#59673,#59674,
#59675),.UNSPECIFIED.,.F.,.F.,(4,3,3,3,3,3,3,3,3,3,3,3,3,3,3,3,3,3,3,3,
3,3,3,3,3,3,3,3,3,3,3,3,3,3,3,3,3,3,3,3,3,3,3,3,3,3,3,3,3,3,3,3,3,3,3,3,
3,3,3,3,3,3,3,3,4),(-60.6402378348566,-60.5414360827456,-60.442769991876,
-60.3442076929065,-60.2457001038484,-60.1472157017466,-60.0487229960321,
-59.9501286902306,-59.8514768227107,-59.7526634030564,-59.7073021597704,
-59.6075735378709,-59.5079871694863,-59.408511330439,-59.3091025847602,
-59.2097263023535,-59.1103520879298,-59.0108091802242,-58.9112911344038,
-58.8115925279537,-58.7121804571076,-58.6124518352081,-58.5128654668237,
-58.4133896277763,-58.3139808820975,-58.2146045996908,-58.1152303852671,
-58.0156874775615,-57.9161694317411,-57.8164708252911,-57.7170587544448,
-57.6173301325453,-57.517743764161,-57.4182679251136,-57.3188591794348,
-57.219482897028,-57.1201086826042,-57.0205657748986,-56.9210477290781,
-56.821349122628,-56.7219370517819,-56.6222084298823,-56.5226220614979,
-56.4231462224505,-56.3237374767719,-56.2243611943652,-56.1249869799411,
-56.0254440722356,-55.9259260264153,-55.8262274199651,-55.7268153491191,
-55.6270867272197,-55.5275003588357,-55.4280245197883,-55.3286157741095,
-55.2292394917031,-55.1298652772792,-55.0303223695735,-54.9308043237532,
-54.8311057173032,-54.7316936464563,-54.6190397884431,-54.5068020959542,
-54.3952724464623,-54.357052528268),.UNSPECIFIED.);
#652=B_SPLINE_CURVE_WITH_KNOTS('',3,(#59677,#59678,#59679,#59680,#59681,
#59682,#59683,#59684,#59685,#59686,#59687,#59688,#59689,#59690,#59691,#59692,
#59693,#59694,#59695,#59696,#59697,#59698,#59699,#59700,#59701,#59702,#59703,
#59704,#59705,#59706,#59707,#59708,#59709,#59710,#59711,#59712,#59713,#59714,
#59715,#59716,#59717,#59718,#59719,#59720,#59721,#59722,#59723,#59724,#59725,
#59726,#59727,#59728,#59729,#59730,#59731,#59732,#59733,#59734,#59735,#59736,
#59737,#59738,#59739,#59740,#59741,#59742,#59743,#59744,#59745,#59746,#59747,
#59748,#59749,#59750,#59751,#59752,#59753,#59754,#59755,#59756,#59757,#59758,
#59759,#59760,#59761,#59762,#59763,#59764,#59765,#59766,#59767,#59768,#59769,
#59770,#59771,#59772,#59773,#59774,#59775,#59776,#59777,#59778,#59779,#59780,
#59781,#59782,#59783,#59784,#59785,#59786,#59787,#59788,#59789,#59790,#59791,
#59792,#59793,#59794,#59795,#59796,#59797,#59798,#59799,#59800,#59801,#59802,
#59803,#59804,#59805,#59806,#59807,#59808,#59809,#59810,#59811,#59812,#59813,
#59814,#59815,#59816,#59817,#59818,#59819,#59820,#59821,#59822,#59823,#59824,
#59825,#59826,#59827,#59828,#59829,#59830,#59831,#59832,#59833,#59834,#59835,
#59836,#59837,#59838,#59839,#59840,#59841,#59842,#59843,#59844,#59845,#59846,
#59847,#59848,#59849,#59850,#59851,#59852,#59853,#59854,#59855,#59856,#59857,
#59858,#59859,#59860,#59861,#59862,#59863,#59864,#59865,#59866,#59867,#59868,
#59869),.UNSPECIFIED.,.F.,.F.,(4,3,3,3,3,3,3,3,3,3,3,3,3,3,3,3,3,3,3,3,
3,3,3,3,3,3,3,3,3,3,3,3,3,3,3,3,3,3,3,3,3,3,3,3,3,3,3,3,3,3,3,3,3,3,3,3,
3,3,3,3,3,3,3,3,4),(-54.3570525280442,-54.2569055163465,-54.1567447379845,
-54.0517015394367,-53.951357160527,-53.8509287440537,-53.7503282601737,
-53.7365719437934,-53.6368433218939,-53.5372569535095,-53.4377811144622,
-53.3383723687834,-53.2389960863768,-53.1396218719531,-53.0400789642475,
-52.9405609184271,-52.8408623119771,-52.7414502411306,-52.641721619231,
-52.5421352508463,-52.442659411799,-52.3432506661202,-52.2438743837134,
-52.1445001692895,-52.0449572615841,-51.9454392157635,-51.8457406093134,
-51.7463285384677,-51.6465999165682,-51.5470135481838,-51.4475377091365,
-51.3481289634577,-51.2487526810511,-51.1493784666272,-51.0498355589216,
-50.9503175131012,-50.8506189066511,-50.7512068358049,-50.6514782139054,
-50.5518918455211,-50.4524160064737,-50.353007260795,-50.2536309783884,
-50.1542567639646,-50.054713856259,-49.9551958104385,-49.8554972039884,
-49.7560851331421,-49.6563565112426,-49.556770142858,-49.4572943038106,
-49.3578855581318,-49.258509275725,-49.1591350613011,-49.0595921535956,
-48.960074107775,-48.8603755013249,-48.7609634304792,-48.6616990220686,
-48.5625696821931,-48.4635442241765,-48.3645802249587,-48.2656562064993,
-48.1666968095702,-48.0738672208646),.UNSPECIFIED.);
#653=B_SPLINE_CURVE_WITH_KNOTS('',3,(#59871,#59872,#59873,#59874,#59875,
#59876,#59877,#59878,#59879,#59880,#59881,#59882,#59883,#59884,#59885,#59886,
#59887,#59888,#59889,#59890,#59891,#59892,#59893,#59894,#59895,#59896,#59897,
#59898,#59899,#59900,#59901,#59902,#59903,#59904,#59905,#59906,#59907,#59908,
#59909,#59910,#59911,#59912,#59913,#59914,#59915,#59916,#59917,#59918,#59919,
#59920,#59921,#59922,#59923,#59924,#59925,#59926,#59927,#59928,#59929,#59930,
#59931,#59932,#59933,#59934,#59935,#59936,#59937,#59938,#59939,#59940,#59941,
#59942,#59943,#59944,#59945,#59946,#59947,#59948,#59949,#59950,#59951,#59952,
#59953,#59954,#59955,#59956,#59957,#59958,#59959,#59960,#59961,#59962,#59963,
#59964,#59965,#59966,#59967,#59968,#59969,#59970,#59971,#59972,#59973,#59974,
#59975,#59976,#59977,#59978,#59979,#59980,#59981,#59982,#59983,#59984,#59985,
#59986,#59987,#59988,#59989,#59990,#59991,#59992,#59993,#59994,#59995,#59996,
#59997,#59998,#59999,#60000,#60001,#60002,#60003,#60004,#60005,#60006,#60007,
#60008,#60009,#60010,#60011,#60012,#60013,#60014,#60015,#60016,#60017,#60018,
#60019,#60020,#60021,#60022,#60023,#60024,#60025,#60026,#60027,#60028,#60029,
#60030,#60031,#60032,#60033,#60034,#60035,#60036,#60037,#60038,#60039,#60040,
#60041,#60042,#60043,#60044,#60045,#60046,#60047,#60048,#60049,#60050,#60051,
#60052,#60053,#60054,#60055,#60056,#60057,#60058,#60059,#60060,#60061,#60062,
#60063),.UNSPECIFIED.,.F.,.F.,(4,3,3,3,3,3,3,3,3,3,3,3,3,3,3,3,3,3,3,3,
3,3,3,3,3,3,3,3,3,3,3,3,3,3,3,3,3,3,3,3,3,3,3,3,3,3,3,3,3,3,3,3,3,3,3,3,
3,3,3,3,3,3,3,3,4),(-48.073867220502,-47.9555291228368,-47.8357144863554,
-47.7658417278164,-47.6661131059167,-47.5665267375321,-47.4670508984848,
-47.3676421528058,-47.268265870399,-47.1688916559749,-47.0693487482695,
-46.9698307024489,-46.8701320959987,-46.7707200251535,-46.670991403254,
-46.5714050348696,-46.4719291958222,-46.3725204501435,-46.2731441677368,
-46.173769953313,-46.0742270456074,-45.974708999787,-45.8750103933369,-45.7755983224907,
-45.6758697005912,-45.5762833322068,-45.4768074931594,-45.3773987474807,
-45.2780224650739,-45.1786482506501,-45.0791053429445,-44.9795872971241,
-44.8798886906741,-44.7804766198278,-44.6807479979282,-44.5811616295438,
-44.4816857904964,-44.3822770448176,-44.2829007624109,-44.1835265479871,
-44.0839836402816,-43.9844655944611,-43.884766988011,-43.785354917165,-43.6856262952655,
-43.586039926881,-43.4865640878337,-43.3871553421549,-43.2877790597482,
-43.1884048453244,-43.0888619376189,-42.9893438917984,-42.8896452853484,
-42.7902332145022,-42.6905045926026,-42.5909182242181,-42.4914423851708,
-42.392033639492,-42.2926573570853,-42.1932831426614,-42.0937402349559,
-41.9942221891355,-41.8945235826853,-41.7951115118393,-41.790681913685),
 .UNSPECIFIED.);
#654=B_SPLINE_CURVE_WITH_KNOTS('',3,(#60065,#60066,#60067,#60068,#60069,
#60070,#60071,#60072,#60073,#60074,#60075,#60076,#60077,#60078,#60079,#60080,
#60081,#60082,#60083,#60084,#60085,#60086,#60087,#60088,#60089,#60090,#60091,
#60092,#60093,#60094,#60095,#60096,#60097,#60098,#60099,#60100,#60101,#60102,
#60103,#60104,#60105,#60106,#60107,#60108,#60109,#60110,#60111,#60112,#60113,
#60114,#60115,#60116,#60117,#60118,#60119,#60120,#60121,#60122,#60123,#60124,
#60125,#60126,#60127,#60128,#60129,#60130,#60131,#60132,#60133,#60134,#60135,
#60136,#60137,#60138,#60139,#60140,#60141,#60142,#60143,#60144,#60145,#60146,
#60147,#60148,#60149,#60150,#60151,#60152,#60153,#60154,#60155,#60156,#60157,
#60158,#60159,#60160,#60161,#60162,#60163,#60164,#60165,#60166,#60167,#60168,
#60169,#60170,#60171,#60172,#60173,#60174,#60175,#60176,#60177,#60178,#60179,
#60180,#60181,#60182,#60183,#60184,#60185,#60186,#60187,#60188,#60189,#60190,
#60191,#60192,#60193,#60194,#60195,#60196,#60197,#60198,#60199,#60200,#60201,
#60202,#60203,#60204,#60205,#60206,#60207,#60208,#60209,#60210,#60211,#60212,
#60213,#60214,#60215,#60216,#60217,#60218,#60219,#60220,#60221,#60222,#60223,
#60224,#60225,#60226,#60227,#60228,#60229,#60230,#60231,#60232,#60233,#60234,
#60235,#60236,#60237,#60238,#60239,#60240,#60241,#60242,#60243,#60244,#60245,
#60246,#60247,#60248,#60249,#60250,#60251,#60252,#60253,#60254),
 .UNSPECIFIED.,.F.,.F.,(4,3,3,3,3,3,3,3,3,3,3,3,3,3,3,3,3,3,3,3,3,3,3,3,
3,3,3,3,3,3,3,3,3,3,3,3,3,3,3,3,3,3,3,3,3,3,3,3,3,3,3,3,3,3,3,3,3,3,3,3,
3,3,3,4),(-41.7906819134384,-41.6910324087699,-41.5915250724781,-41.4921321462826,
-41.3928018135445,-41.2935035298061,-41.1942067901162,-41.0948123126013,
-40.9953709872715,-40.8957504652476,-40.7999898091765,-40.700261187277,
-40.6006748188926,-40.5011989798453,-40.4017902341665,-40.3024139517598,
-40.203039737336,-40.1034968296304,-40.0039787838099,-39.9042801773598,
-39.8048681065136,-39.705139484614,-39.6055531162297,-39.5060772771823,
-39.4066685315035,-39.3072922490968,-39.2079180346731,-39.1083751269675,
-39.0088570811471,-38.909158474697,-38.8097464038508,-38.7100177819513,
-38.6104314135668,-38.5109555745195,-38.4115468288407,-38.3121705464341,
-38.2127963320103,-38.1132534243047,-38.0137353784843,-37.9140367720343,
-37.814624701188,-37.7148960792884,-37.615309710904,-37.5158338718566,-37.4164251261779,
-37.3170488437712,-37.2176746293474,-37.1181317216418,-37.0186136758213,
-36.9189150693711,-36.8195029985251,-36.7197743766256,-36.6201880082412,
-36.5207121691938,-36.421303423515,-36.3219271411085,-36.2225529266847,
-36.1230100189791,-36.0234919731587,-35.9237933667087,-35.8243812958623,
-35.7055742237464,-35.5880755367551,-35.5074966068939),.UNSPECIFIED.);
#655=B_SPLINE_CURVE_WITH_KNOTS('',3,(#60256,#60257,#60258,#60259,#60260,
#60261,#60262,#60263,#60264,#60265,#60266,#60267,#60268,#60269,#60270,#60271,
#60272,#60273,#60274,#60275,#60276,#60277,#60278,#60279,#60280,#60281,#60282,
#60283,#60284,#60285,#60286,#60287,#60288,#60289,#60290,#60291,#60292,#60293,
#60294,#60295,#60296,#60297,#60298,#60299,#60300,#60301,#60302,#60303,#60304,
#60305,#60306,#60307,#60308,#60309,#60310,#60311,#60312,#60313,#60314,#60315,
#60316,#60317,#60318,#60319,#60320,#60321,#60322,#60323,#60324,#60325,#60326,
#60327,#60328,#60329,#60330,#60331,#60332,#60333,#60334,#60335,#60336,#60337,
#60338,#60339,#60340,#60341,#60342,#60343,#60344,#60345,#60346,#60347,#60348,
#60349,#60350,#60351,#60352,#60353,#60354,#60355,#60356,#60357,#60358,#60359,
#60360,#60361,#60362,#60363,#60364,#60365,#60366,#60367,#60368,#60369,#60370,
#60371,#60372,#60373,#60374,#60375,#60376,#60377,#60378,#60379,#60380,#60381,
#60382,#60383,#60384,#60385,#60386,#60387,#60388,#60389,#60390,#60391,#60392,
#60393,#60394,#60395,#60396,#60397,#60398,#60399,#60400,#60401,#60402,#60403,
#60404,#60405,#60406,#60407,#60408,#60409,#60410,#60411,#60412,#60413,#60414,
#60415,#60416,#60417,#60418,#60419,#60420,#60421,#60422,#60423,#60424,#60425,
#60426,#60427,#60428,#60429,#60430,#60431,#60432,#60433,#60434,#60435,#60436,
#60437,#60438,#60439,#60440,#60441,#60442,#60443,#60444,#60445,#60446,#60447,
#60448),.UNSPECIFIED.,.F.,.F.,(4,3,3,3,3,3,3,3,3,3,3,3,3,3,3,3,3,3,3,3,
3,3,3,3,3,3,3,3,3,3,3,3,3,3,3,3,3,3,3,3,3,3,3,3,3,3,3,3,3,3,3,3,3,3,3,3,
3,3,3,3,3,3,3,3,4),(-35.5074966065054,-35.4084154446817,-35.3093596833664,
-35.2102985815147,-35.1111318234569,-35.0119117474664,-34.9125107445922,
-34.8292595931994,-34.7295309712999,-34.6299446029154,-34.530468763868,
-34.4310600181895,-34.3316837357827,-34.232309521359,-34.1327666136534,
-34.033248567833,-33.933549961383,-33.8341378905366,-33.7344092686374,-33.6348229002533,
-33.5353470612059,-33.4359383155274,-33.3365620331209,-33.2371878186972,
-33.1376449109914,-33.0381268651713,-32.9384282587215,-32.8390161878738,
-32.7392875659734,-32.6397011975882,-32.540225358541,-32.4408166128614,
-32.3414403304539,-32.2420661160294,-32.1425232083248,-32.0430051625036,
-31.9433065560527,-31.8438944852109,-31.744165863312,-31.6445794949281,
-31.5451036558806,-31.4456949102025,-31.3463186277965,-31.2469444133734,
-31.1474015056671,-31.0478834598473,-30.9481848533977,-30.8487727825481,
-30.7490441606503,-30.6494577922679,-30.54998195322,-30.4505732075431,-30.3511969251383,
-30.251822710716,-30.1522798030083,-30.0527617571894,-29.953063150741,-29.8536510798852,
-29.7532833659848,-29.6530619260124,-29.5529572423997,-29.4529450306602,
-29.3529859149049,-29.2530399000807,-29.2243112993258),.UNSPECIFIED.);
#656=B_SPLINE_CURVE_WITH_KNOTS('',3,(#60450,#60451,#60452,#60453,#60454,
#60455,#60456,#60457,#60458,#60459,#60460,#60461,#60462,#60463,#60464,#60465,
#60466,#60467,#60468,#60469,#60470,#60471,#60472,#60473,#60474,#60475,#60476,
#60477,#60478,#60479,#60480,#60481,#60482,#60483,#60484,#60485,#60486,#60487,
#60488,#60489,#60490,#60491,#60492,#60493,#60494,#60495,#60496,#60497,#60498,
#60499,#60500,#60501,#60502,#60503,#60504,#60505,#60506,#60507,#60508,#60509,
#60510,#60511,#60512,#60513,#60514,#60515,#60516,#60517,#60518,#60519,#60520,
#60521,#60522,#60523,#60524,#60525,#60526,#60527,#60528,#60529,#60530,#60531,
#60532,#60533,#60534,#60535,#60536,#60537,#60538,#60539,#60540,#60541,#60542,
#60543,#60544,#60545,#60546,#60547,#60548,#60549,#60550,#60551,#60552,#60553,
#60554,#60555,#60556,#60557,#60558,#60559,#60560,#60561,#60562,#60563,#60564,
#60565,#60566,#60567,#60568,#60569,#60570,#60571,#60572,#60573,#60574,#60575,
#60576,#60577,#60578,#60579,#60580,#60581,#60582,#60583,#60584,#60585,#60586,
#60587,#60588,#60589,#60590,#60591,#60592,#60593,#60594,#60595,#60596,#60597,
#60598,#60599,#60600,#60601,#60602,#60603,#60604,#60605,#60606,#60607,#60608,
#60609,#60610,#60611,#60612,#60613,#60614,#60615,#60616,#60617,#60618,#60619,
#60620,#60621,#60622,#60623,#60624,#60625,#60626,#60627,#60628,#60629,#60630,
#60631,#60632,#60633,#60634,#60635,#60636,#60637,#60638,#60639,#60640,#60641,
#60642),.UNSPECIFIED.,.F.,.F.,(4,3,3,3,3,3,3,3,3,3,3,3,3,3,3,3,3,3,3,3,
3,3,3,3,3,3,3,3,3,3,3,3,3,3,3,3,3,3,3,3,3,3,3,3,3,3,3,3,3,3,3,3,3,3,3,3,
3,3,3,3,3,3,3,3,4),(-29.2243112990994,-29.1119176126332,-28.9989879022127,
-28.8854264210957,-28.8585293772224,-28.7588007553295,-28.6592143869515,
-28.5597385479025,-28.4603298022301,-28.3609535198297,-28.2615793054121,
-28.1620363976989,-28.0625183518846,-27.9628197454403,-27.8634076745595,
-27.76367905267,-27.6640926842956,-27.5646168452457,-27.4652080995772,-27.3658318171809,
-27.2664576027674,-27.1669146950497,-27.0673966492396,-26.9676980427998,
-26.8682859718967,-26.7685573499505,-26.6689709815193,-26.5694951424836,
-26.4700863967582,-26.370710114305,-26.2713358998348,-26.1717929921846,
-26.0722749463188,-25.9725763398244,-25.8731642692339,-25.7734356473956,
-25.6738492790722,-25.5743734400096,-25.4749646943909,-25.3755884120438,
-25.2762141976789,-25.176671289902,-25.0771532441386,-24.9774546377439,
-24.878042566571,-24.77831394472,-24.6787275763848,-24.5792517373252,-24.4798429916974,
-24.3804667093421,-24.2810924949701,-24.1815495872046,-24.0820315414365,
-23.9823329350386,-23.8829208639082,-23.7839919713175,-23.6852046011585,
-23.5865297484849,-23.4879152047942,-23.3893295469522,-23.2907413898845,
-23.1920584636559,-23.0933232402924,-22.9944290368006,-22.9411259924852),
 .UNSPECIFIED.);
#657=B_SPLINE_CURVE_WITH_KNOTS('',3,(#60644,#60645,#60646,#60647,#60648,
#60649,#60650,#60651,#60652,#60653,#60654,#60655,#60656,#60657,#60658,#60659,
#60660,#60661,#60662,#60663,#60664,#60665,#60666,#60667,#60668,#60669,#60670,
#60671,#60672,#60673,#60674,#60675,#60676,#60677,#60678,#60679,#60680,#60681,
#60682,#60683,#60684,#60685,#60686,#60687,#60688,#60689,#60690,#60691,#60692,
#60693,#60694,#60695,#60696,#60697,#60698,#60699,#60700,#60701,#60702,#60703,
#60704,#60705,#60706,#60707,#60708,#60709,#60710,#60711,#60712,#60713,#60714,
#60715,#60716,#60717,#60718,#60719,#60720,#60721,#60722,#60723,#60724,#60725,
#60726,#60727,#60728,#60729,#60730,#60731,#60732,#60733,#60734,#60735,#60736,
#60737,#60738,#60739,#60740,#60741,#60742,#60743,#60744,#60745,#60746,#60747,
#60748,#60749,#60750,#60751,#60752,#60753,#60754,#60755,#60756,#60757,#60758,
#60759,#60760,#60761,#60762,#60763,#60764,#60765,#60766,#60767,#60768,#60769,
#60770,#60771,#60772,#60773,#60774,#60775,#60776,#60777,#60778,#60779,#60780,
#60781,#60782,#60783,#60784,#60785,#60786,#60787,#60788,#60789,#60790,#60791,
#60792,#60793,#60794,#60795,#60796,#60797,#60798,#60799,#60800,#60801,#60802,
#60803,#60804,#60805,#60806,#60807,#60808,#60809,#60810,#60811,#60812,#60813,
#60814,#60815,#60816,#60817,#60818,#60819,#60820,#60821,#60822,#60823,#60824,
#60825,#60826,#60827,#60828,#60829,#60830,#60831,#60832,#60833),
 .UNSPECIFIED.,.F.,.F.,(4,3,3,3,3,3,3,3,3,3,3,3,3,3,3,3,3,3,3,3,3,3,3,3,
3,3,3,3,3,3,3,3,3,3,3,3,3,3,3,3,3,3,3,3,3,3,3,3,3,3,3,3,3,3,3,3,3,3,3,3,
3,3,3,4),(-22.9411259921462,-22.8877991612453,-22.7880705398818,-22.6884841720323,
-22.589008332851,-22.4895995877004,-22.3902233058181,-22.2908490919144,
-22.1913061835814,-22.0917881382652,-21.9920895323057,-21.8926774585825,
-21.792948836839,-21.6933624686168,-21.5938866295297,-21.4944778840265,
-21.3951016018,-21.2957273875606,-21.1961844796504,-21.0966664340231,-20.9969678277697,
-20.8975557559197,-20.7978271316268,-20.6982407608406,-20.5987649223926,
-20.4993561743092,-20.3999798895022,-20.3006056726855,-20.2010627678284,
-20.1015447196579,-20.001846110902,-19.9024340532568,-19.8027054358651,
-19.7031190719831,-19.6036432318095,-19.5042344905878,-19.4048582126111,
-19.3054840025846,-19.2059410895869,-19.1064230480395,-19.0067244457544,
-18.907312350594,-18.8075837282666,-18.7079973594981,-18.6085215205522,
-18.5091127745974,-18.4097364919555,-18.3103622773375,-18.2108193699859,
-18.1113013240723,-18.0116027175897,-17.9121906479311,-17.8124620096355,
-17.7128756247817,-17.6133997898425,-17.5139910276388,-17.4146147287232,
-17.315240497829,-17.2156976096888,-17.1161795476597,-17.0164809252863,
-16.9170689452683,-16.7875048152669,-16.6579406852656),.UNSPECIFIED.);
#658=B_SPLINE_CURVE_WITH_KNOTS('',3,(#60835,#60836,#60837,#60838,#60839,
#60840,#60841,#60842,#60843,#60844,#60845,#60846,#60847,#60848,#60849,#60850,
#60851,#60852,#60853,#60854,#60855,#60856,#60857,#60858,#60859,#60860,#60861,
#60862,#60863,#60864,#60865,#60866,#60867,#60868,#60869,#60870,#60871,#60872,
#60873,#60874,#60875,#60876,#60877,#60878,#60879,#60880,#60881,#60882,#60883,
#60884,#60885,#60886,#60887,#60888,#60889,#60890,#60891,#60892,#60893,#60894,
#60895,#60896,#60897,#60898,#60899,#60900,#60901,#60902,#60903,#60904,#60905,
#60906,#60907,#60908,#60909,#60910,#60911,#60912,#60913,#60914,#60915,#60916,
#60917,#60918,#60919,#60920,#60921,#60922,#60923,#60924,#60925,#60926,#60927,
#60928,#60929,#60930,#60931,#60932,#60933,#60934,#60935,#60936,#60937,#60938,
#60939,#60940,#60941,#60942,#60943,#60944,#60945,#60946,#60947,#60948,#60949,
#60950,#60951,#60952,#60953,#60954,#60955,#60956,#60957,#60958,#60959,#60960,
#60961,#60962,#60963,#60964,#60965,#60966,#60967,#60968,#60969,#60970,#60971,
#60972,#60973,#60974,#60975,#60976,#60977,#60978,#60979,#60980,#60981,#60982,
#60983,#60984,#60985,#60986,#60987,#60988,#60989,#60990,#60991,#60992,#60993,
#60994,#60995,#60996,#60997,#60998,#60999,#61000,#61001,#61002,#61003,#61004,
#61005,#61006,#61007,#61008,#61009,#61010,#61011,#61012,#61013,#61014,#61015,
#61016,#61017,#61018,#61019,#61020,#61021,#61022,#61023,#61024,#61025,#61026,
#61027),.UNSPECIFIED.,.F.,.F.,(4,3,3,3,3,3,3,3,3,3,3,3,3,3,3,3,3,3,3,3,
3,3,3,3,3,3,3,3,3,3,3,3,3,3,3,3,3,3,3,3,3,3,3,3,3,3,3,3,3,3,3,3,3,3,3,3,
3,3,3,3,3,3,3,3,4),(-16.6579406849666,-16.5595254138767,-16.4611656545462,
-16.3628297431378,-16.2644860491586,-16.1660406753646,-16.0675379808886,
-15.9688725793384,-15.9219472426055,-15.8222186055224,-15.722632222262,
-15.6231563869721,-15.5237476272617,-15.4243713311703,-15.324997103425,
-15.2254542125544,-15.1259361544264,-15.0262375363684,-14.9268255399426,
-14.8270968098077,-14.7275103325797,-14.6280345206672,-14.528625665478,
-14.4292492735555,-14.3298749497611,-14.2303321716408,-14.1308140179199,
-14.0311153053082,-13.9317038372798,-13.8319755046024,-13.7323894255564,
-13.6329135141889,-13.5335050560296,-13.434129059821,-13.3347551298906,
-13.2352118810722,-13.1356941127167,-13.0359957773353,-12.9365821346169,
-12.8368533112414,-12.7372667434675,-12.6377909545283,-12.5383820159022,
-12.4390055433873,-12.3396311419351,-12.2400884644398,-12.1405702409433,
-12.0408714637876,-11.9414604319541,-11.8417311293534,-11.7421440753674,
-11.6426684071079,-11.5432589690684,-11.4438819933176,-11.3445070855228,
-11.2449649964649,-11.1454462643122,-11.0457469812194,-10.9463387292913,
-10.8443976736582,-10.7426219664132,-10.6410185584271,-10.5395165541003,
-10.4380999037676,-10.3747553777871),.UNSPECIFIED.);
#659=B_SPLINE_CURVE_WITH_KNOTS('',3,(#61028,#61029,#61030,#61031,#61032,
#61033,#61034,#61035,#61036,#61037,#61038,#61039,#61040,#61041,#61042,#61043,
#61044,#61045,#61046,#61047,#61048,#61049,#61050,#61051,#61052,#61053,#61054,
#61055,#61056,#61057,#61058,#61059,#61060,#61061,#61062,#61063,#61064,#61065,
#61066,#61067,#61068,#61069,#61070,#61071,#61072,#61073,#61074,#61075,#61076,
#61077,#61078,#61079,#61080,#61081,#61082,#61083,#61084,#61085,#61086,#61087,
#61088,#61089,#61090,#61091,#61092,#61093,#61094,#61095,#61096,#61097,#61098,
#61099,#61100,#61101,#61102,#61103,#61104,#61105,#61106,#61107,#61108,#61109,
#61110,#61111,#61112,#61113,#61114,#61115,#61116,#61117,#61118,#61119,#61120,
#61121,#61122,#61123,#61124,#61125,#61126,#61127,#61128,#61129,#61130,#61131,
#61132,#61133,#61134,#61135,#61136,#61137,#61138,#61139,#61140,#61141,#61142,
#61143,#61144,#61145,#61146,#61147,#61148,#61149,#61150,#61151,#61152,#61153,
#61154,#61155,#61156,#61157,#61158,#61159,#61160,#61161,#61162,#61163,#61164,
#61165,#61166,#61167,#61168,#61169,#61170,#61171,#61172,#61173,#61174,#61175,
#61176,#61177,#61178,#61179,#61180,#61181,#61182,#61183,#61184,#61185,#61186,
#61187,#61188,#61189,#61190,#61191,#61192,#61193,#61194,#61195,#61196,#61197,
#61198,#61199,#61200,#61201,#61202,#61203,#61204,#61205,#61206,#61207,#61208,
#61209,#61210,#61211,#61212,#61213,#61214,#61215,#61216,#61217),
 .UNSPECIFIED.,.F.,.F.,(4,3,3,3,3,3,3,3,3,3,3,3,3,3,3,3,3,3,3,3,3,3,3,3,
3,3,3,3,3,3,3,3,3,3,3,3,3,3,3,3,3,3,3,3,3,3,3,3,3,3,3,3,3,3,3,3,3,3,3,3,
3,3,3,4),(-10.374755377445,-10.2666403402494,-10.1582341426202,-10.0493640278324,
-9.95121702662841,-9.85148626928268,-9.75189777905866,-9.65242247217202,
-9.55301165262249,-9.45363331890765,-9.35425707839538,-9.25471663978792,
-9.15519664952035,-9.05549616263931,-8.95609532396556,-8.85636271069546,
-8.75677231251689,-8.65729659670131,-8.55788375890536,-8.4585033697821,
-8.35912503976698,-8.25958718515092,-8.16006504486301,-8.06036238976783,
-7.96097362130273,-7.86126170701285,-7.76169207580455,-7.66221205615897,
-7.56281999731274,-7.46346034580379,-7.36410268400977,-7.2645399926673,
-7.16503814110849,-7.06535538645003,-6.96585191863989,-6.86610295137288,
-6.76649632180622,-6.66700463266673,-6.56757598469549,-6.46817996859153,
-6.3687862149989,-6.26927221524343,-6.16973530891784,-6.0700184049135,-5.97073021597704,
-5.87098078279411,-5.7713733089186,-5.67188021499968,-5.57244982385309,
-5.47305173161607,-5.37365557405361,-5.27414380886876,-5.17460373277934,
-5.07488323140633,-4.9756085133142,-4.87730205406189,-4.77908555613009,
-4.68103283919324,-4.58303928543698,-4.48507287255004,-4.3866971720644,
-4.28863976403018,-4.19010491731883,-4.09157007060747),.UNSPECIFIED.);
#660=B_SPLINE_CURVE_WITH_KNOTS('',3,(#61220,#61221,#61222,#61223,#61224,
#61225,#61226,#61227,#61228,#61229,#61230,#61231,#61232,#61233,#61234,#61235,
#61236,#61237,#61238,#61239,#61240,#61241,#61242,#61243,#61244,#61245,#61246,
#61247,#61248,#61249,#61250,#61251,#61252,#61253,#61254,#61255,#61256,#61257,
#61258,#61259,#61260,#61261,#61262,#61263,#61264,#61265,#61266,#61267,#61268,
#61269,#61270,#61271,#61272,#61273,#61274,#61275,#61276,#61277,#61278,#61279,
#61280,#61281,#61282,#61283,#61284,#61285,#61286,#61287,#61288,#61289,#61290,
#61291,#61292,#61293,#61294,#61295,#61296,#61297,#61298,#61299,#61300,#61301,
#61302,#61303,#61304,#61305,#61306,#61307,#61308,#61309,#61310,#61311,#61312,
#61313,#61314,#61315,#61316,#61317,#61318,#61319,#61320,#61321,#61322,#61323,
#61324,#61325,#61326,#61327,#61328,#61329,#61330,#61331,#61332,#61333,#61334,
#61335,#61336,#61337,#61338,#61339,#61340,#61341,#61342,#61343,#61344,#61345,
#61346,#61347,#61348,#61349,#61350,#61351,#61352,#61353,#61354,#61355,#61356,
#61357,#61358,#61359,#61360,#61361,#61362,#61363,#61364,#61365,#61366,#61367,
#61368,#61369,#61370,#61371,#61372,#61373,#61374,#61375,#61376,#61377,#61378,
#61379,#61380,#61381,#61382,#61383,#61384,#61385,#61386,#61387,#61388,#61389,
#61390,#61391,#61392,#61393,#61394,#61395,#61396,#61397,#61398,#61399,#61400,
#61401,#61402,#61403,#61404,#61405,#61406,#61407,#61408,#61409,#61410,#61411,
#61412,#61413,#61414,#61415,#61416,#61417,#61418,#61419,#61420,#61421,#61422,
#61423,#61424,#61425,#61426,#61427),.UNSPECIFIED.,.F.,.F.,(4,2,2,2,2,2,
2,2,2,2,2,2,2,2,2,2,2,2,2,2,2,2,2,2,2,2,2,2,2,2,2,2,2,2,2,2,2,2,2,2,2,2,
2,2,2,2,2,2,2,2,2,2,2,2,2,2,2,2,2,2,2,2,2,2,2,2,2,2,2,2,2,2,2,2,2,2,2,2,
2,2,2,2,2,2,2,2,2,2,2,2,2,2,2,2,2,2,2,2,2,2,2,2,2,4),(-1.21637204632693,
-1.18714290050887,-1.18252519076056,-1.1807942159484,-1.17956280411588,
-1.17823552312567,-1.17635158849732,-1.17162079875575,-1.14705039224846,
-1.14077796097892,-1.09197684086135,-1.08562311062903,-1.08220436766822,
-1.08005044700325,-1.07767787536863,-1.07436663504098,-1.06627092900157,
-1.05480887089881,-1.02102482040869,-0.988400361083974,-0.983570737553261,
-0.981615366171339,-0.98040759960187,-0.979057449006166,-0.97706100749205,
-0.971584919014512,-0.963185823572804,-0.933150358345562,-0.893530921537853,
-0.886213997454938,-0.883268847552423,-0.881096495416968,-0.878734576904006,
-0.875494868267652,-0.867849289884309,-0.857216314838179,-0.826216218525186,
-0.789262848239083,-0.784525102245509,-0.782582789002447,-0.781255367233748,
-0.779867817589057,-0.77771389121137,-0.771065412169405,-0.719245851386342,
-0.691239192782983,-0.686615884965941,-0.683684931943939,-0.681364583094547,
-0.678757827789386,-0.674367145504357,-0.656577561987564,-0.619456587063486,
-0.604213643902452,-0.587749283738322,-0.585041466858672,-0.583372101564736,
-0.582078570779847,-0.580584735903522,-0.57790246127404,-0.564608816748289,
-0.532983242490501,-0.495442277149877,-0.488137580459467,-0.485206205622946,
-0.483047363281574,-0.480703500033383,-0.477494910782589,-0.469954775086192,
-0.459493944316976,-0.429284366138851,-0.39109259755817,-0.38642283744968,
-0.384498988020802,-0.383180349796379,-0.381794201598762,-0.379639079791357,
-0.372961981016016,-0.321531606930985,-0.292543961380232,-0.287876426142365,
-0.284927377224576,-0.28259902175302,-0.279989859276483,-0.27561079366892,
-0.258079541803134,-0.223670634633327,-0.192200716316426,-0.187380329325498,
-0.185443294449896,-0.184115233500877,-0.182741261833012,-0.180638789586354,
-0.174620664136115,-0.133055970605354,-0.127524992631861,-0.0961719537331771,
-0.0914419738928427,-0.0884601980251379,-0.0861092523711643,-0.0834777457465266,
-0.0790673926692267,-0.0614849840781803,-0.00328557036190819),
 .UNSPECIFIED.);
#661=B_SPLINE_CURVE_WITH_KNOTS('',3,(#61431,#61432,#61433,#61434,#61435,
#61436,#61437,#61438,#61439,#61440,#61441,#61442,#61443,#61444,#61445,#61446,
#61447,#61448,#61449,#61450,#61451,#61452,#61453,#61454,#61455,#61456,#61457,
#61458,#61459,#61460,#61461,#61462,#61463,#61464,#61465,#61466,#61467,#61468,
#61469,#61470,#61471,#61472,#61473,#61474,#61475,#61476,#61477,#61478,#61479,
#61480,#61481,#61482,#61483,#61484,#61485,#61486,#61487,#61488,#61489,#61490,
#61491,#61492,#61493,#61494,#61495,#61496,#61497,#61498,#61499,#61500,#61501,
#61502,#61503,#61504,#61505,#61506,#61507,#61508,#61509,#61510,#61511,#61512,
#61513,#61514,#61515,#61516,#61517,#61518,#61519,#61520,#61521,#61522,#61523,
#61524,#61525,#61526,#61527,#61528,#61529,#61530,#61531,#61532,#61533,#61534,
#61535,#61536,#61537,#61538,#61539,#61540,#61541,#61542,#61543,#61544,#61545,
#61546,#61547,#61548,#61549,#61550,#61551,#61552,#61553,#61554,#61555,#61556,
#61557,#61558,#61559,#61560,#61561,#61562,#61563,#61564,#61565,#61566,#61567,
#61568,#61569,#61570,#61571,#61572),.UNSPECIFIED.,.F.,.F.,(4,3,3,3,3,3,
3,3,3,3,3,3,3,3,3,3,3,3,3,3,3,3,3,3,3,3,3,3,3,3,3,3,3,3,3,3,3,3,3,3,3,3,
3,3,3,3,3,4),(153.9380400259,154.042627859806,154.147205809574,154.251809213478,
154.35654362196,154.461356730466,154.566354309905,154.5910480186,154.696232724251,
154.801260196385,154.906163563652,155.011000480753,155.115806173648,155.220615823419,
155.325531863438,155.430507489867,155.535658420593,155.586169721263,155.691265762231,
155.796207481203,155.901029752881,156.005788504605,156.11051905473,156.215256679851,
156.320105840498,156.425017425559,156.530109315656,156.581291423926,156.685242476528,
156.789036407253,156.892712029041,156.996325266124,157.099912973806,157.203511967393,
157.307236501764,157.411029514324,157.515024345921,157.576413126589,157.684260599358,
157.795169878095,157.902660840125,158.010050857761,158.117368959288,158.22464408008,
158.331934949153,158.439234198118,158.546606884271,158.571534829252),
 .UNSPECIFIED.);
#662=B_SPLINE_CURVE_WITH_KNOTS('',3,(#61573,#61574,#61575,#61576),
 .UNSPECIFIED.,.F.,.F.,(4,4),(-2.51360796055909,-2.47288460460841),
 .UNSPECIFIED.);
#663=B_SPLINE_CURVE_WITH_KNOTS('',3,(#61581,#61582,#61583,#61584,#61585,
#61586,#61587,#61588,#61589,#61590,#61591,#61592,#61593,#61594,#61595,#61596,
#61597,#61598,#61599,#61600,#61601,#61602,#61603,#61604,#61605,#61606,#61607,
#61608,#61609,#61610,#61611,#61612,#61613,#61614,#61615,#61616,#61617,#61618,
#61619,#61620,#61621,#61622,#61623,#61624,#61625,#61626,#61627,#61628,#61629,
#61630,#61631,#61632,#61633,#61634,#61635,#61636,#61637,#61638,#61639,#61640,
#61641,#61642,#61643,#61644,#61645,#61646,#61647,#61648,#61649,#61650,#61651,
#61652,#61653,#61654,#61655,#61656,#61657,#61658,#61659,#61660,#61661,#61662,
#61663,#61664,#61665,#61666,#61667,#61668),.UNSPECIFIED.,.F.,.F.,(4,3,3,
3,3,3,3,3,3,3,3,3,3,3,3,3,3,3,3,3,3,3,3,3,3,3,3,3,3,4),(-0.45720120831918,
-0.443119064139232,-0.417479433866563,-0.404574804592397,-0.39832007975076,
-0.393505561949894,-0.368121979410151,-0.348481872316771,-0.338772362600017,
-0.332900697228815,-0.308156868840611,-0.283671164875764,-0.259896194857207,
-0.251236675637993,-0.247397000158282,-0.24318973513902,-0.219712589842507,
-0.211005365479902,-0.186944794736734,-0.163659385060356,-0.158785883220003,
-0.135404476683544,-0.112094332640347,-0.089146627335351,-0.0803319464901571,
-0.0766177528090602,-0.0541139355306132,-0.0322370316722101,-0.0106664437314021,
0.),.UNSPECIFIED.);
#664=B_SPLINE_CURVE_WITH_KNOTS('',3,(#61670,#61671,#61672,#61673),
 .UNSPECIFIED.,.F.,.F.,(4,4),(0.,0.013548856899879),.UNSPECIFIED.);
#665=B_SPLINE_CURVE_WITH_KNOTS('',3,(#61674,#61675,#61676,#61677,#61678,
#61679,#61680,#61681,#61682,#61683,#61684,#61685,#61686,#61687,#61688,#61689,
#61690,#61691,#61692,#61693,#61694,#61695,#61696,#61697,#61698,#61699,#61700,
#61701,#61702,#61703,#61704,#61705,#61706,#61707,#61708,#61709,#61710,#61711,
#61712,#61713,#61714,#61715,#61716,#61717,#61718,#61719,#61720,#61721,#61722,
#61723,#61724,#61725,#61726,#61727,#61728,#61729,#61730,#61731,#61732,#61733,
#61734,#61735,#61736,#61737,#61738,#61739,#61740,#61741,#61742,#61743,#61744,
#61745,#61746,#61747,#61748,#61749,#61750,#61751,#61752,#61753,#61754,#61755,
#61756,#61757,#61758),.UNSPECIFIED.,.F.,.F.,(4,3,3,3,3,3,3,3,3,3,3,3,3,
3,3,3,3,3,3,3,3,3,3,3,3,3,3,3,4),(-0.463803050843757,-0.448342324914894,
-0.426613591771729,-0.414011063870098,-0.409959849332504,-0.387413304468716,
-0.368330462284901,-0.359247061418826,-0.354808316317046,-0.331546268178802,
-0.307399571530292,-0.283764191523977,-0.275707032179122,-0.27179436159638,
-0.267658923961038,-0.243231654365683,-0.23495948158476,-0.211119300050522,
-0.187279118516284,-0.181503918087659,-0.157189728431955,-0.132120535354269,
-0.107051342276583,-0.0964113535606421,-0.0910152568088142,-0.0653193769800867,
-0.0396389090410066,-0.0142617177111558,0.),.UNSPECIFIED.);
#666=B_SPLINE_CURVE_WITH_KNOTS('',3,(#62376,#62377,#62378,#62379),
 .UNSPECIFIED.,.F.,.F.,(4,4),(-0.0456416910700171,0.),.UNSPECIFIED.);
#667=B_SPLINE_CURVE_WITH_KNOTS('',3,(#62381,#62382,#62383,#62384,#62385,
#62386,#62387,#62388,#62389,#62390,#62391,#62392,#62393,#62394,#62395,#62396,
#62397,#62398,#62399,#62400,#62401,#62402,#62403,#62404,#62405,#62406,#62407,
#62408,#62409,#62410,#62411,#62412,#62413,#62414,#62415,#62416,#62417,#62418,
#62419,#62420,#62421,#62422,#62423,#62424,#62425,#62426,#62427,#62428,#62429,
#62430,#62431,#62432,#62433,#62434,#62435,#62436,#62437,#62438,#62439,#62440,
#62441,#62442,#62443,#62444,#62445,#62446,#62447,#62448,#62449,#62450,#62451,
#62452,#62453,#62454,#62455,#62456,#62457,#62458,#62459,#62460,#62461,#62462,
#62463,#62464,#62465),.UNSPECIFIED.,.F.,.F.,(4,3,3,3,3,3,3,3,3,3,3,3,3,
3,3,3,3,3,3,3,3,3,3,3,3,3,3,3,4),(-0.463803050843767,-0.448342324914899,
-0.426613580872991,-0.414011043992197,-0.409959831578531,-0.387383433778229,
-0.368330439754046,-0.359247027935732,-0.354808278989149,-0.331103908693188,
-0.307399538397226,-0.283764158765723,-0.275707013541777,-0.2717942090871,
-0.267658891500947,-0.243231622613926,-0.234959481584771,-0.211363092564089,
-0.187279108106858,-0.181503921086847,-0.157189726180108,-0.13212052996401,
-0.107051333747913,-0.0964113400410272,-0.0904420396421145,-0.0646992370938577,
-0.0389224220676543,-0.0136952256569932,0.),.UNSPECIFIED.);
#668=B_SPLINE_CURVE_WITH_KNOTS('',3,(#62466,#62467,#62468,#62469),
 .UNSPECIFIED.,.F.,.F.,(4,4),(-0.0133434464393684,0.),.UNSPECIFIED.);
#669=B_SPLINE_CURVE_WITH_KNOTS('',3,(#62475,#62476,#62477,#62478,#62479,
#62480,#62481,#62482,#62483,#62484,#62485,#62486,#62487,#62488,#62489,#62490,
#62491,#62492,#62493,#62494,#62495,#62496,#62497,#62498,#62499,#62500,#62501,
#62502,#62503,#62504,#62505,#62506,#62507,#62508,#62509,#62510,#62511,#62512,
#62513,#62514,#62515,#62516,#62517,#62518,#62519,#62520,#62521,#62522,#62523,
#62524,#62525,#62526,#62527,#62528,#62529,#62530,#62531,#62532,#62533,#62534,
#62535,#62536,#62537,#62538,#62539,#62540,#62541,#62542,#62543,#62544,#62545,
#62546,#62547,#62548,#62549,#62550,#62551,#62552,#62553,#62554,#62555,#62556,
#62557,#62558,#62559,#62560,#62561,#62562),.UNSPECIFIED.,.F.,.F.,(4,3,3,
3,3,3,3,3,3,3,3,3,3,3,3,3,3,3,3,3,3,3,3,3,3,3,3,3,3,4),(-0.457201133310259,
-0.443119064139323,-0.41747943419836,-0.404574804903458,-0.398320120175313,
-0.393505569481669,-0.368121987119509,-0.348481879064538,-0.338772374950317,
-0.332900696925308,-0.308144898687338,-0.283887995601292,-0.2601352143991,
-0.251236713711485,-0.247397146482524,-0.243189764173982,-0.219712628371478,
-0.211005365479924,-0.186944796986518,-0.163659390555148,-0.158785882880634,
-0.135457646099974,-0.112205379051171,-0.0891466107339279,-0.0803319444019404,
-0.0766177517214363,-0.0541139253004491,-0.0322370044393299,-0.0106663968464944,
0.),.UNSPECIFIED.);
#670=B_SPLINE_CURVE_WITH_KNOTS('',3,(#63179,#63180,#63181,#63182),
 .UNSPECIFIED.,.F.,.F.,(4,4),(0.,0.0463476257986535),.UNSPECIFIED.);
#818=SHAPE_REPRESENTATION_RELATIONSHIP('SRR','None',#81137,#828);
#828=ADVANCED_BREP_SHAPE_REPRESENTATION('',(#848),#81037);
#838=STYLED_ITEM('',(#81196),#848);
#848=MANIFOLD_SOLID_BREP('Body1',#15091);
#1024=CYLINDRICAL_SURFACE('',#16364,1.99475);
#1025=CYLINDRICAL_SURFACE('',#16366,1.99475);
#1026=CYLINDRICAL_SURFACE('',#16367,1.99475);
#1027=CYLINDRICAL_SURFACE('',#16368,1.99475);
#1028=CYLINDRICAL_SURFACE('',#16369,1.99475);
#1029=CYLINDRICAL_SURFACE('',#16370,1.99475);
#1030=CYLINDRICAL_SURFACE('',#16371,1.99475);
#1031=CYLINDRICAL_SURFACE('',#16372,1.99475);
#1032=CYLINDRICAL_SURFACE('',#16373,1.99475);
#1033=CYLINDRICAL_SURFACE('',#16374,1.99475);
#1034=CYLINDRICAL_SURFACE('',#16375,1.99475);
#1035=CYLINDRICAL_SURFACE('',#16376,1.99475);
#1036=CYLINDRICAL_SURFACE('',#16377,1.99475);
#1037=CYLINDRICAL_SURFACE('',#16378,1.99475);
#1038=CYLINDRICAL_SURFACE('',#16379,1.99475);
#1039=CYLINDRICAL_SURFACE('',#16380,1.99475);
#1040=CYLINDRICAL_SURFACE('',#16381,1.99475);
#1041=CYLINDRICAL_SURFACE('',#16382,1.99475);
#1042=CYLINDRICAL_SURFACE('',#16383,1.99475);
#1043=CYLINDRICAL_SURFACE('',#16384,1.99475);
#1044=CYLINDRICAL_SURFACE('',#16385,1.99475);
#1045=CYLINDRICAL_SURFACE('',#16386,1.99475);
#1046=CYLINDRICAL_SURFACE('',#16387,1.99475);
#1047=CYLINDRICAL_SURFACE('',#16388,2.4505);
#1048=CYLINDRICAL_SURFACE('',#16391,1.99475);
#1049=CYLINDRICAL_SURFACE('',#16407,1.39337567297407);
#1050=CYLINDRICAL_SURFACE('',#16409,1.39337567297407);
#1051=CYLINDRICAL_SURFACE('',#16411,1.39337567297407);
#1052=CYLINDRICAL_SURFACE('',#16413,1.39337567297407);
#1053=CYLINDRICAL_SURFACE('',#16415,1.39337567297407);
#1054=CYLINDRICAL_SURFACE('',#16417,1.39337567297407);
#1208=FACE_BOUND('',#3150,.T.);
#1561=PLANE('',#16393);
#1562=PLANE('',#16396);
#1563=PLANE('',#16419);
#1564=PLANE('',#16420);
#1565=PLANE('',#16421);
#1566=PLANE('',#16422);
#1567=PLANE('',#16423);
#1568=PLANE('',#16424);
#1569=PLANE('',#16425);
#1570=PLANE('',#16426);
#1571=PLANE('',#16427);
#1572=PLANE('',#16428);
#1573=PLANE('',#16430);
#1574=PLANE('',#16432);
#1575=PLANE('',#16434);
#1576=PLANE('',#16436);
#1577=PLANE('',#16438);
#1578=PLANE('',#16441);
#1579=PLANE('',#16442);
#1580=PLANE('',#16443);
#1581=PLANE('',#16444);
#1582=PLANE('',#16449);
#2226=FACE_OUTER_BOUND('',#3094,.T.);
#2227=FACE_OUTER_BOUND('',#3095,.T.);
#2228=FACE_OUTER_BOUND('',#3096,.T.);
#2229=FACE_OUTER_BOUND('',#3097,.T.);
#2230=FACE_OUTER_BOUND('',#3098,.T.);
#2231=FACE_OUTER_BOUND('',#3099,.T.);
#2232=FACE_OUTER_BOUND('',#3100,.T.);
#2233=FACE_OUTER_BOUND('',#3101,.T.);
#2234=FACE_OUTER_BOUND('',#3102,.T.);
#2235=FACE_OUTER_BOUND('',#3103,.T.);
#2236=FACE_OUTER_BOUND('',#3104,.T.);
#2237=FACE_OUTER_BOUND('',#3105,.T.);
#2238=FACE_OUTER_BOUND('',#3106,.T.);
#2239=FACE_OUTER_BOUND('',#3107,.T.);
#2240=FACE_OUTER_BOUND('',#3108,.T.);
#2241=FACE_OUTER_BOUND('',#3109,.T.);
#2242=FACE_OUTER_BOUND('',#3110,.T.);
#2243=FACE_OUTER_BOUND('',#3111,.T.);
#2244=FACE_OUTER_BOUND('',#3112,.T.);
#2245=FACE_OUTER_BOUND('',#3113,.T.);
#2246=FACE_OUTER_BOUND('',#3114,.T.);
#2247=FACE_OUTER_BOUND('',#3115,.T.);
#2248=FACE_OUTER_BOUND('',#3116,.T.);
#2249=FACE_OUTER_BOUND('',#3117,.T.);
#2250=FACE_OUTER_BOUND('',#3118,.T.);
#2251=FACE_OUTER_BOUND('',#3119,.T.);
#2252=FACE_OUTER_BOUND('',#3120,.T.);
#2253=FACE_OUTER_BOUND('',#3121,.T.);
#2254=FACE_OUTER_BOUND('',#3122,.T.);
#2255=FACE_OUTER_BOUND('',#3123,.T.);
#2256=FACE_OUTER_BOUND('',#3124,.T.);
#2257=FACE_OUTER_BOUND('',#3125,.T.);
#2258=FACE_OUTER_BOUND('',#3126,.T.);
#2259=FACE_OUTER_BOUND('',#3127,.T.);
#2260=FACE_OUTER_BOUND('',#3128,.T.);
#2261=FACE_OUTER_BOUND('',#3129,.T.);
#2262=FACE_OUTER_BOUND('',#3130,.T.);
#2263=FACE_OUTER_BOUND('',#3131,.T.);
#2264=FACE_OUTER_BOUND('',#3132,.T.);
#2265=FACE_OUTER_BOUND('',#3133,.T.);
#2266=FACE_OUTER_BOUND('',#3134,.T.);
#2267=FACE_OUTER_BOUND('',#3135,.T.);
#2268=FACE_OUTER_BOUND('',#3136,.T.);
#2269=FACE_OUTER_BOUND('',#3137,.T.);
#2270=FACE_OUTER_BOUND('',#3138,.T.);
#2271=FACE_OUTER_BOUND('',#3139,.T.);
#2272=FACE_OUTER_BOUND('',#3140,.T.);
#2273=FACE_OUTER_BOUND('',#3141,.T.);
#2274=FACE_OUTER_BOUND('',#3142,.T.);
#2275=FACE_OUTER_BOUND('',#3143,.T.);
#2276=FACE_OUTER_BOUND('',#3144,.T.);
#2277=FACE_OUTER_BOUND('',#3145,.T.);
#2278=FACE_OUTER_BOUND('',#3146,.T.);
#2279=FACE_OUTER_BOUND('',#3147,.T.);
#2280=FACE_OUTER_BOUND('',#3148,.T.);
#2281=FACE_OUTER_BOUND('',#3149,.T.);
#2282=FACE_OUTER_BOUND('',#3151,.T.);
#2283=FACE_OUTER_BOUND('',#3152,.T.);
#2284=FACE_OUTER_BOUND('',#3153,.T.);
#3094=EDGE_LOOP('',(#13312,#13313,#13314,#13315));
#3095=EDGE_LOOP('',(#13316,#13317,#13318,#13319,#13320));
#3096=EDGE_LOOP('',(#13321,#13322,#13323,#13324));
#3097=EDGE_LOOP('',(#13325,#13326,#13327,#13328,#13329));
#3098=EDGE_LOOP('',(#13330,#13331,#13332,#13333,#13334,#13335));
#3099=EDGE_LOOP('',(#13336,#13337,#13338,#13339));
#3100=EDGE_LOOP('',(#13340,#13341,#13342,#13343,#13344,#13345));
#3101=EDGE_LOOP('',(#13346,#13347,#13348,#13349));
#3102=EDGE_LOOP('',(#13350,#13351,#13352,#13353,#13354,#13355));
#3103=EDGE_LOOP('',(#13356,#13357,#13358,#13359));
#3104=EDGE_LOOP('',(#13360,#13361,#13362,#13363,#13364,#13365));
#3105=EDGE_LOOP('',(#13366,#13367,#13368,#13369,#13370));
#3106=EDGE_LOOP('',(#13371,#13372,#13373,#13374,#13375));
#3107=EDGE_LOOP('',(#13376,#13377,#13378,#13379,#13380));
#3108=EDGE_LOOP('',(#13381,#13382,#13383,#13384,#13385));
#3109=EDGE_LOOP('',(#13386,#13387,#13388,#13389,#13390));
#3110=EDGE_LOOP('',(#13391,#13392,#13393,#13394,#13395));
#3111=EDGE_LOOP('',(#13396,#13397,#13398,#13399,#13400));
#3112=EDGE_LOOP('',(#13401,#13402,#13403,#13404,#13405));
#3113=EDGE_LOOP('',(#13406,#13407,#13408,#13409,#13410));
#3114=EDGE_LOOP('',(#13411,#13412,#13413,#13414,#13415));
#3115=EDGE_LOOP('',(#13416,#13417,#13418,#13419,#13420));
#3116=EDGE_LOOP('',(#13421,#13422,#13423,#13424));
#3117=EDGE_LOOP('',(#13425,#13426,#13427,#13428,#13429,#13430,#13431,#13432,
#13433,#13434,#13435,#13436,#13437,#13438,#13439,#13440,#13441,#13442,#13443,
#13444,#13445,#13446,#13447,#13448,#13449,#13450,#13451,#13452,#13453,#13454,
#13455,#13456,#13457,#13458,#13459,#13460,#13461,#13462,#13463,#13464,#13465,
#13466,#13467,#13468,#13469,#13470,#13471,#13472,#13473,#13474,#13475,#13476));
#3118=EDGE_LOOP('',(#13477,#13478,#13479,#13480,#13481));
#3119=EDGE_LOOP('',(#13482,#13483,#13484,#13485,#13486,#13487));
#3120=EDGE_LOOP('',(#13488,#13489,#13490,#13491,#13492,#13493,#13494,#13495,
#13496,#13497,#13498,#13499,#13500,#13501,#13502,#13503,#13504,#13505,#13506,
#13507,#13508,#13509,#13510,#13511,#13512,#13513,#13514,#13515,#13516,#13517,
#13518,#13519,#13520,#13521,#13522,#13523,#13524,#13525,#13526,#13527,#13528,
#13529,#13530,#13531,#13532,#13533,#13534,#13535,#13536,#13537,#13538,#13539,
#13540,#13541,#13542,#13543,#13544,#13545,#13546,#13547,#13548,#13549,#13550,
#13551));
#3121=EDGE_LOOP('',(#13552,#13553,#13554,#13555,#13556,#13557));
#3122=EDGE_LOOP('',(#13558,#13559,#13560,#13561,#13562,#13563,#13564,#13565,
#13566,#13567,#13568,#13569,#13570,#13571,#13572,#13573,#13574,#13575,#13576,
#13577,#13578,#13579,#13580,#13581,#13582,#13583,#13584,#13585,#13586,#13587,
#13588,#13589,#13590,#13591,#13592,#13593,#13594,#13595,#13596,#13597,#13598,
#13599,#13600,#13601,#13602,#13603,#13604,#13605,#13606,#13607,#13608,#13609,
#13610,#13611,#13612,#13613,#13614,#13615,#13616,#13617,#13618,#13619,#13620,
#13621));
#3123=EDGE_LOOP('',(#13622,#13623,#13624,#13625,#13626,#13627,#13628,#13629,
#13630,#13631,#13632,#13633,#13634,#13635,#13636,#13637,#13638,#13639,#13640,
#13641,#13642));
#3124=EDGE_LOOP('',(#13643,#13644,#13645,#13646));
#3125=EDGE_LOOP('',(#13647,#13648,#13649,#13650));
#3126=EDGE_LOOP('',(#13651,#13652,#13653,#13654));
#3127=EDGE_LOOP('',(#13655,#13656,#13657,#13658));
#3128=EDGE_LOOP('',(#13659,#13660,#13661,#13662));
#3129=EDGE_LOOP('',(#13663,#13664,#13665,#13666));
#3130=EDGE_LOOP('',(#13667,#13668,#13669,#13670,#13671,#13672,#13673,#13674));
#3131=EDGE_LOOP('',(#13675,#13676,#13677,#13678,#13679,#13680,#13681,#13682));
#3132=EDGE_LOOP('',(#13683,#13684,#13685,#13686,#13687,#13688,#13689,#13690));
#3133=EDGE_LOOP('',(#13691,#13692));
#3134=EDGE_LOOP('',(#13693,#13694));
#3135=EDGE_LOOP('',(#13695,#13696));
#3136=EDGE_LOOP('',(#13697,#13698));
#3137=EDGE_LOOP('',(#13699,#13700));
#3138=EDGE_LOOP('',(#13701,#13702));
#3139=EDGE_LOOP('',(#13703,#13704));
#3140=EDGE_LOOP('',(#13705,#13706));
#3141=EDGE_LOOP('',(#13707,#13708));
#3142=EDGE_LOOP('',(#13709,#13710));
#3143=EDGE_LOOP('',(#13711,#13712));
#3144=EDGE_LOOP('',(#13713,#13714));
#3145=EDGE_LOOP('',(#13715,#13716,#13717,#13718,#13719,#13720,#13721,#13722));
#3146=EDGE_LOOP('',(#13723,#13724,#13725,#13726,#13727,#13728,#13729,#13730));
#3147=EDGE_LOOP('',(#13731,#13732,#13733,#13734,#13735,#13736,#13737,#13738));
#3148=EDGE_LOOP('',(#13739,#13740,#13741,#13742,#13743,#13744,#13745,#13746));
#3149=EDGE_LOOP('',(#13747));
#3150=EDGE_LOOP('',(#13748));
#3151=EDGE_LOOP('',(#13749,#13750,#13751,#13752,#13753,#13754,#13755));
#3152=EDGE_LOOP('',(#13756,#13757,#13758,#13759,#13760,#13761,#13762));
#3153=EDGE_LOOP('',(#13763));
#4228=LINE('',#43210,#5340);
#4229=LINE('',#43509,#5341);
#4230=LINE('',#43953,#5342);
#4231=LINE('',#44385,#5343);
#4232=LINE('',#44805,#5344);
#4233=LINE('',#45307,#5345);
#4234=LINE('',#45737,#5346);
#4235=LINE('',#46191,#5347);
#4236=LINE('',#46635,#5348);
#4237=LINE('',#47117,#5349);
#4238=LINE('',#47583,#5350);
#4239=LINE('',#48007,#5351);
#4240=LINE('',#48471,#5352);
#4241=LINE('',#48910,#5353);
#4242=LINE('',#49349,#5354);
#4243=LINE('',#49798,#5355);
#4244=LINE('',#50301,#5356);
#4245=LINE('',#50804,#5357);
#4246=LINE('',#51283,#5358);
#4247=LINE('',#51716,#5359);
#4248=LINE('',#52161,#5360);
#4249=LINE('',#52610,#5361);
#4250=LINE('',#53053,#5362);
#4251=LINE('',#63245,#5363);
#4252=LINE('',#63249,#5364);
#4253=LINE('',#63251,#5365);
#4254=LINE('',#63255,#5366);
#4255=LINE('',#63257,#5367);
#4256=LINE('',#63261,#5368);
#4257=LINE('',#63264,#5369);
#4258=LINE('',#63267,#5370);
#4259=LINE('',#63269,#5371);
#4260=LINE('',#63273,#5372);
#4261=LINE('',#63276,#5373);
#4262=LINE('',#63279,#5374);
#4263=LINE('',#63282,#5375);
#4264=LINE('',#63284,#5376);
#4265=LINE('',#63286,#5377);
#4266=LINE('',#63288,#5378);
#4267=LINE('',#63289,#5379);
#4268=LINE('',#63291,#5380);
#4269=LINE('',#63293,#5381);
#4270=LINE('',#63294,#5382);
#4271=LINE('',#63296,#5383);
#4272=LINE('',#63298,#5384);
#4273=LINE('',#63299,#5385);
#4274=LINE('',#63303,#5386);
#4275=LINE('',#63306,#5387);
#4276=LINE('',#63308,#5388);
#4277=LINE('',#63311,#5389);
#4278=LINE('',#63321,#5390);
#4279=LINE('',#63324,#5391);
#4280=LINE('',#63328,#5392);
#4281=LINE('',#63330,#5393);
#4282=LINE('',#63332,#5394);
#4283=LINE('',#63338,#5395);
#4284=LINE('',#63341,#5396);
#5340=VECTOR('',#19948,1.99475);
#5341=VECTOR('',#19953,1.99475);
#5342=VECTOR('',#19956,1.99475);
#5343=VECTOR('',#19959,1.99475);
#5344=VECTOR('',#19962,1.99475);
#5345=VECTOR('',#19965,1.99475);
#5346=VECTOR('',#19968,1.99475);
#5347=VECTOR('',#19971,1.99475);
#5348=VECTOR('',#19974,1.99475);
#5349=VECTOR('',#19977,1.99475);
#5350=VECTOR('',#19980,1.99475);
#5351=VECTOR('',#19983,1.99475);
#5352=VECTOR('',#19986,1.99475);
#5353=VECTOR('',#19989,1.99475);
#5354=VECTOR('',#19992,1.99475);
#5355=VECTOR('',#19995,1.99475);
#5356=VECTOR('',#19998,1.99475);
#5357=VECTOR('',#20001,1.99475);
#5358=VECTOR('',#20004,1.99475);
#5359=VECTOR('',#20007,1.99475);
#5360=VECTOR('',#20010,1.99475);
#5361=VECTOR('',#20013,1.99475);
#5362=VECTOR('',#20016,1.99475);
#5363=VECTOR('',#20053,1.49337567297406);
#5364=VECTOR('',#20058,10.);
#5365=VECTOR('',#20059,10.);
#5366=VECTOR('',#20064,10.);
#5367=VECTOR('',#20065,10.);
#5368=VECTOR('',#20070,10.);
#5369=VECTOR('',#20073,10.);
#5370=VECTOR('',#20076,10.);
#5371=VECTOR('',#20077,10.);
#5372=VECTOR('',#20082,10.);
#5373=VECTOR('',#20085,10.);
#5374=VECTOR('',#20088,10.);
#5375=VECTOR('',#20091,10.);
#5376=VECTOR('',#20094,10.);
#5377=VECTOR('',#20095,10.);
#5378=VECTOR('',#20096,10.);
#5379=VECTOR('',#20097,10.);
#5380=VECTOR('',#20100,10.);
#5381=VECTOR('',#20101,10.);
#5382=VECTOR('',#20102,10.);
#5383=VECTOR('',#20105,10.);
#5384=VECTOR('',#20106,10.);
#5385=VECTOR('',#20107,10.);
#5386=VECTOR('',#20114,10.);
#5387=VECTOR('',#20119,10.);
#5388=VECTOR('',#20122,10.);
#5389=VECTOR('',#20125,10.);
#5390=VECTOR('',#20142,10.);
#5391=VECTOR('',#20147,10.);
#5392=VECTOR('',#20152,1.44337567297407);
#5393=VECTOR('',#20155,10.);
#5394=VECTOR('',#20158,10.);
#5395=VECTOR('',#20167,2.26);
#5396=VECTOR('',#20170,2.125);
#5948=CIRCLE('',#16365,1.99475);
#5949=CIRCLE('',#16389,2.4505);
#5950=CIRCLE('',#16390,2.4505);
#5951=CIRCLE('',#16392,1.99475);
#5952=CIRCLE('',#16394,2.4505);
#5953=CIRCLE('',#16395,2.4505);
#5954=CIRCLE('',#16397,2.4505);
#5955=CIRCLE('',#16398,2.4505);
#5956=CIRCLE('',#16400,1.39337567297407);
#5957=CIRCLE('',#16401,1.39337567297407);
#5958=CIRCLE('',#16402,1.39337567297407);
#5959=CIRCLE('',#16403,1.39337567297407);
#5960=CIRCLE('',#16404,1.39337567297407);
#5961=CIRCLE('',#16405,1.39337567297407);
#5962=CIRCLE('',#16406,1.59337567297406);
#5963=CIRCLE('',#16408,1.39337567297407);
#5964=CIRCLE('',#16410,1.39337567297407);
#5965=CIRCLE('',#16412,1.39337567297407);
#5966=CIRCLE('',#16414,1.39337567297407);
#5967=CIRCLE('',#16416,1.39337567297407);
#5968=CIRCLE('',#16418,1.39337567297407);
#5969=CIRCLE('',#16429,1.44337567297407);
#5970=CIRCLE('',#16431,1.44337567297407);
#5971=CIRCLE('',#16433,1.44337567297407);
#5972=CIRCLE('',#16435,1.44337567297407);
#5973=CIRCLE('',#16437,1.44337567297407);
#5974=CIRCLE('',#16439,1.44337567297407);
#5975=CIRCLE('',#16445,2.02);
#5976=CIRCLE('',#16448,1.75);
#7205=VERTEX_POINT('',#43208);
#7206=VERTEX_POINT('',#43209);
#7207=VERTEX_POINT('',#43211);
#7208=VERTEX_POINT('',#43386);
#7209=VERTEX_POINT('',#43507);
#7210=VERTEX_POINT('',#43508);
#7211=VERTEX_POINT('',#43728);
#7212=VERTEX_POINT('',#43951);
#7213=VERTEX_POINT('',#43952);
#7214=VERTEX_POINT('',#44383);
#7215=VERTEX_POINT('',#44384);
#7216=VERTEX_POINT('',#44614);
#7217=VERTEX_POINT('',#44803);
#7218=VERTEX_POINT('',#44804);
#7219=VERTEX_POINT('',#44806);
#7220=VERTEX_POINT('',#45067);
#7221=VERTEX_POINT('',#45305);
#7222=VERTEX_POINT('',#45306);
#7223=VERTEX_POINT('',#45735);
#7224=VERTEX_POINT('',#45736);
#7225=VERTEX_POINT('',#45738);
#7226=VERTEX_POINT('',#45967);
#7227=VERTEX_POINT('',#46189);
#7228=VERTEX_POINT('',#46190);
#7229=VERTEX_POINT('',#46633);
#7230=VERTEX_POINT('',#46634);
#7231=VERTEX_POINT('',#46636);
#7232=VERTEX_POINT('',#46869);
#7233=VERTEX_POINT('',#47115);
#7234=VERTEX_POINT('',#47116);
#7235=VERTEX_POINT('',#47581);
#7236=VERTEX_POINT('',#47582);
#7237=VERTEX_POINT('',#47584);
#7238=VERTEX_POINT('',#47773);
#7239=VERTEX_POINT('',#48005);
#7240=VERTEX_POINT('',#48006);
#7241=VERTEX_POINT('',#48008);
#7242=VERTEX_POINT('',#48469);
#7243=VERTEX_POINT('',#48470);
#7244=VERTEX_POINT('',#48684);
#7245=VERTEX_POINT('',#48908);
#7246=VERTEX_POINT('',#48909);
#7247=VERTEX_POINT('',#48911);
#7248=VERTEX_POINT('',#49347);
#7249=VERTEX_POINT('',#49348);
#7250=VERTEX_POINT('',#49572);
#7251=VERTEX_POINT('',#49796);
#7252=VERTEX_POINT('',#49797);
#7253=VERTEX_POINT('',#49799);
#7254=VERTEX_POINT('',#50299);
#7255=VERTEX_POINT('',#50300);
#7256=VERTEX_POINT('',#50534);
#7257=VERTEX_POINT('',#50802);
#7258=VERTEX_POINT('',#50803);
#7259=VERTEX_POINT('',#50805);
#7260=VERTEX_POINT('',#51281);
#7261=VERTEX_POINT('',#51282);
#7262=VERTEX_POINT('',#51488);
#7263=VERTEX_POINT('',#51714);
#7264=VERTEX_POINT('',#51715);
#7265=VERTEX_POINT('',#51717);
#7266=VERTEX_POINT('',#52159);
#7267=VERTEX_POINT('',#52160);
#7268=VERTEX_POINT('',#52378);
#7269=VERTEX_POINT('',#52608);
#7270=VERTEX_POINT('',#52609);
#7271=VERTEX_POINT('',#52611);
#7272=VERTEX_POINT('',#53051);
#7273=VERTEX_POINT('',#53052);
#7274=VERTEX_POINT('',#53517);
#7275=VERTEX_POINT('',#53518);
#7276=VERTEX_POINT('',#53525);
#7277=VERTEX_POINT('',#53527);
#7278=VERTEX_POINT('',#53533);
#7279=VERTEX_POINT('',#53724);
#7280=VERTEX_POINT('',#53918);
#7281=VERTEX_POINT('',#54109);
#7282=VERTEX_POINT('',#54303);
#7283=VERTEX_POINT('',#54497);
#7284=VERTEX_POINT('',#54691);
#7285=VERTEX_POINT('',#54882);
#7286=VERTEX_POINT('',#55076);
#7287=VERTEX_POINT('',#55270);
#7288=VERTEX_POINT('',#55461);
#7289=VERTEX_POINT('',#55655);
#7290=VERTEX_POINT('',#55846);
#7291=VERTEX_POINT('',#56037);
#7292=VERTEX_POINT('',#56228);
#7293=VERTEX_POINT('',#56422);
#7294=VERTEX_POINT('',#56613);
#7295=VERTEX_POINT('',#56807);
#7296=VERTEX_POINT('',#57001);
#7297=VERTEX_POINT('',#57192);
#7298=VERTEX_POINT('',#57386);
#7299=VERTEX_POINT('',#57580);
#7300=VERTEX_POINT('',#57592);
#7301=VERTEX_POINT('',#57783);
#7302=VERTEX_POINT('',#57866);
#7303=VERTEX_POINT('',#57868);
#7304=VERTEX_POINT('',#57874);
#7305=VERTEX_POINT('',#58065);
#7306=VERTEX_POINT('',#58259);
#7307=VERTEX_POINT('',#58270);
#7308=VERTEX_POINT('',#58281);
#7309=VERTEX_POINT('',#58293);
#7310=VERTEX_POINT('',#58304);
#7311=VERTEX_POINT('',#58315);
#7312=VERTEX_POINT('',#58327);
#7313=VERTEX_POINT('',#58521);
#7314=VERTEX_POINT('',#58715);
#7315=VERTEX_POINT('',#58906);
#7316=VERTEX_POINT('',#59097);
#7317=VERTEX_POINT('',#59291);
#7318=VERTEX_POINT('',#59482);
#7319=VERTEX_POINT('',#59676);
#7320=VERTEX_POINT('',#59870);
#7321=VERTEX_POINT('',#60064);
#7322=VERTEX_POINT('',#60255);
#7323=VERTEX_POINT('',#60449);
#7324=VERTEX_POINT('',#60643);
#7325=VERTEX_POINT('',#60834);
#7326=VERTEX_POINT('',#61219);
#7327=VERTEX_POINT('',#61428);
#7328=VERTEX_POINT('',#61430);
#7329=VERTEX_POINT('',#61578);
#7330=VERTEX_POINT('',#61579);
#7331=VERTEX_POINT('',#61669);
#7332=VERTEX_POINT('',#62380);
#7333=VERTEX_POINT('',#62471);
#7334=VERTEX_POINT('',#62473);
#7335=VERTEX_POINT('',#63184);
#7336=VERTEX_POINT('',#63185);
#7337=VERTEX_POINT('',#63189);
#7338=VERTEX_POINT('',#63191);
#7339=VERTEX_POINT('',#63195);
#7340=VERTEX_POINT('',#63199);
#7341=VERTEX_POINT('',#63201);
#7342=VERTEX_POINT('',#63205);
#7343=VERTEX_POINT('',#63209);
#7344=VERTEX_POINT('',#63211);
#7345=VERTEX_POINT('',#63215);
#7346=VERTEX_POINT('',#63219);
#7347=VERTEX_POINT('',#63221);
#7348=VERTEX_POINT('',#63225);
#7349=VERTEX_POINT('',#63229);
#7350=VERTEX_POINT('',#63231);
#7351=VERTEX_POINT('',#63235);
#7352=VERTEX_POINT('',#63239);
#7353=VERTEX_POINT('',#63244);
#7354=VERTEX_POINT('',#63248);
#7355=VERTEX_POINT('',#63250);
#7356=VERTEX_POINT('',#63254);
#7357=VERTEX_POINT('',#63256);
#7358=VERTEX_POINT('',#63260);
#7359=VERTEX_POINT('',#63262);
#7360=VERTEX_POINT('',#63266);
#7361=VERTEX_POINT('',#63268);
#7362=VERTEX_POINT('',#63272);
#7363=VERTEX_POINT('',#63274);
#7364=VERTEX_POINT('',#63278);
#7365=VERTEX_POINT('',#63280);
#7366=VERTEX_POINT('',#63285);
#7367=VERTEX_POINT('',#63287);
#7368=VERTEX_POINT('',#63292);
#7369=VERTEX_POINT('',#63297);
#7370=VERTEX_POINT('',#63310);
#7371=VERTEX_POINT('',#63320);
#7372=VERTEX_POINT('',#63327);
#7373=VERTEX_POINT('',#63335);
#7374=VERTEX_POINT('',#63340);
#9319=EDGE_CURVE('',#7205,#7206,#4228,.T.);
#9320=EDGE_CURVE('',#7207,#7205,#543,.F.);
#9321=EDGE_CURVE('',#7208,#7207,#5948,.T.);
#9322=EDGE_CURVE('',#7208,#7206,#544,.T.);
#9323=EDGE_CURVE('',#7209,#7210,#4229,.T.);
#9324=EDGE_CURVE('',#7205,#7209,#545,.F.);
#9325=EDGE_CURVE('',#7206,#7211,#546,.T.);
#9326=EDGE_CURVE('',#7211,#7210,#547,.T.);
#9327=EDGE_CURVE('',#7212,#7213,#4230,.T.);
#9328=EDGE_CURVE('',#7209,#7212,#548,.F.);
#9329=EDGE_CURVE('',#7210,#7213,#549,.T.);
#9330=EDGE_CURVE('',#7214,#7215,#4231,.T.);
#9331=EDGE_CURVE('',#7212,#7214,#550,.F.);
#9332=EDGE_CURVE('',#7213,#7216,#551,.T.);
#9333=EDGE_CURVE('',#7216,#7215,#552,.T.);
#9334=EDGE_CURVE('',#7217,#7218,#4232,.T.);
#9335=EDGE_CURVE('',#7219,#7217,#553,.F.);
#9336=EDGE_CURVE('',#7214,#7219,#554,.F.);
#9337=EDGE_CURVE('',#7215,#7220,#555,.T.);
#9338=EDGE_CURVE('',#7220,#7218,#556,.T.);
#9339=EDGE_CURVE('',#7221,#7222,#4233,.T.);
#9340=EDGE_CURVE('',#7217,#7221,#557,.F.);
#9341=EDGE_CURVE('',#7218,#7222,#558,.T.);
#9342=EDGE_CURVE('',#7223,#7224,#4234,.T.);
#9343=EDGE_CURVE('',#7225,#7223,#559,.F.);
#9344=EDGE_CURVE('',#7221,#7225,#560,.F.);
#9345=EDGE_CURVE('',#7222,#7226,#561,.T.);
#9346=EDGE_CURVE('',#7226,#7224,#562,.T.);
#9347=EDGE_CURVE('',#7227,#7228,#4235,.T.);
#9348=EDGE_CURVE('',#7223,#7227,#563,.F.);
#9349=EDGE_CURVE('',#7224,#7228,#564,.T.);
#9350=EDGE_CURVE('',#7229,#7230,#4236,.T.);
#9351=EDGE_CURVE('',#7231,#7229,#565,.F.);
#9352=EDGE_CURVE('',#7227,#7231,#566,.F.);
#9353=EDGE_CURVE('',#7228,#7232,#567,.T.);
#9354=EDGE_CURVE('',#7232,#7230,#568,.T.);
#9355=EDGE_CURVE('',#7233,#7234,#4237,.T.);
#9356=EDGE_CURVE('',#7229,#7233,#569,.F.);
#9357=EDGE_CURVE('',#7230,#7234,#570,.T.);
#9358=EDGE_CURVE('',#7235,#7236,#4238,.T.);
#9359=EDGE_CURVE('',#7237,#7235,#571,.T.);
#9360=EDGE_CURVE('',#7233,#7237,#572,.F.);
#9361=EDGE_CURVE('',#7234,#7238,#573,.T.);
#9362=EDGE_CURVE('',#7238,#7236,#574,.T.);
#9363=EDGE_CURVE('',#7239,#7240,#4239,.T.);
#9364=EDGE_CURVE('',#7241,#7239,#575,.F.);
#9365=EDGE_CURVE('',#7235,#7241,#576,.T.);
#9366=EDGE_CURVE('',#7236,#7240,#577,.T.);
#9367=EDGE_CURVE('',#7242,#7243,#4240,.T.);
#9368=EDGE_CURVE('',#7239,#7242,#578,.F.);
#9369=EDGE_CURVE('',#7240,#7244,#579,.T.);
#9370=EDGE_CURVE('',#7244,#7243,#580,.T.);
#9371=EDGE_CURVE('',#7245,#7246,#4241,.T.);
#9372=EDGE_CURVE('',#7247,#7245,#581,.F.);
#9373=EDGE_CURVE('',#7242,#7247,#582,.F.);
#9374=EDGE_CURVE('',#7243,#7246,#583,.T.);
#9375=EDGE_CURVE('',#7248,#7249,#4242,.T.);
#9376=EDGE_CURVE('',#7245,#7248,#584,.F.);
#9377=EDGE_CURVE('',#7246,#7250,#585,.T.);
#9378=EDGE_CURVE('',#7250,#7249,#586,.T.);
#9379=EDGE_CURVE('',#7251,#7252,#4243,.T.);
#9380=EDGE_CURVE('',#7253,#7251,#587,.F.);
#9381=EDGE_CURVE('',#7248,#7253,#588,.F.);
#9382=EDGE_CURVE('',#7249,#7252,#589,.T.);
#9383=EDGE_CURVE('',#7254,#7255,#4244,.T.);
#9384=EDGE_CURVE('',#7251,#7254,#590,.F.);
#9385=EDGE_CURVE('',#7252,#7256,#591,.T.);
#9386=EDGE_CURVE('',#7256,#7255,#592,.T.);
#9387=EDGE_CURVE('',#7257,#7258,#4245,.T.);
#9388=EDGE_CURVE('',#7259,#7257,#593,.F.);
#9389=EDGE_CURVE('',#7254,#7259,#594,.F.);
#9390=EDGE_CURVE('',#7255,#7258,#595,.T.);
#9391=EDGE_CURVE('',#7260,#7261,#4246,.T.);
#9392=EDGE_CURVE('',#7257,#7260,#596,.F.);
#9393=EDGE_CURVE('',#7258,#7262,#597,.T.);
#9394=EDGE_CURVE('',#7262,#7261,#598,.T.);
#9395=EDGE_CURVE('',#7263,#7264,#4247,.T.);
#9396=EDGE_CURVE('',#7265,#7263,#599,.F.);
#9397=EDGE_CURVE('',#7260,#7265,#600,.F.);
#9398=EDGE_CURVE('',#7261,#7264,#601,.T.);
#9399=EDGE_CURVE('',#7266,#7267,#4248,.T.);
#9400=EDGE_CURVE('',#7263,#7266,#602,.F.);
#9401=EDGE_CURVE('',#7264,#7268,#603,.T.);
#9402=EDGE_CURVE('',#7268,#7267,#604,.T.);
#9403=EDGE_CURVE('',#7269,#7270,#4249,.T.);
#9404=EDGE_CURVE('',#7271,#7269,#605,.F.);
#9405=EDGE_CURVE('',#7266,#7271,#606,.F.);
#9406=EDGE_CURVE('',#7267,#7270,#607,.T.);
#9407=EDGE_CURVE('',#7272,#7273,#4250,.T.);
#9408=EDGE_CURVE('',#7269,#7272,#608,.F.);
#9409=EDGE_CURVE('',#7270,#7273,#609,.T.);
#9410=EDGE_CURVE('',#7274,#7275,#610,.T.);
#9411=EDGE_CURVE('',#7275,#7276,#5949,.T.);
#9412=EDGE_CURVE('',#7276,#7277,#611,.T.);
#9413=EDGE_CURVE('',#7277,#7278,#612,.T.);
#9414=EDGE_CURVE('',#7278,#7279,#613,.T.);
#9415=EDGE_CURVE('',#7279,#7280,#614,.T.);
#9416=EDGE_CURVE('',#7280,#7281,#615,.T.);
#9417=EDGE_CURVE('',#7281,#7282,#616,.T.);
#9418=EDGE_CURVE('',#7282,#7283,#617,.T.);
#9419=EDGE_CURVE('',#7283,#7284,#618,.T.);
#9420=EDGE_CURVE('',#7284,#7285,#619,.T.);
#9421=EDGE_CURVE('',#7285,#7286,#620,.T.);
#9422=EDGE_CURVE('',#7286,#7287,#621,.T.);
#9423=EDGE_CURVE('',#7287,#7288,#622,.T.);
#9424=EDGE_CURVE('',#7288,#7289,#623,.T.);
#9425=EDGE_CURVE('',#7289,#7290,#624,.T.);
#9426=EDGE_CURVE('',#7290,#7291,#625,.T.);
#9427=EDGE_CURVE('',#7291,#7292,#626,.T.);
#9428=EDGE_CURVE('',#7292,#7293,#627,.T.);
#9429=EDGE_CURVE('',#7293,#7294,#628,.T.);
#9430=EDGE_CURVE('',#7294,#7295,#629,.T.);
#9431=EDGE_CURVE('',#7295,#7296,#630,.T.);
#9432=EDGE_CURVE('',#7296,#7297,#631,.T.);
#9433=EDGE_CURVE('',#7297,#7298,#632,.T.);
#9434=EDGE_CURVE('',#7298,#7299,#633,.T.);
#9435=EDGE_CURVE('',#7299,#7300,#634,.T.);
#9436=EDGE_CURVE('',#7300,#7301,#635,.T.);
#9437=EDGE_CURVE('',#7302,#7301,#5950,.F.);
#9438=EDGE_CURVE('',#7302,#7303,#636,.T.);
#9439=EDGE_CURVE('',#7303,#7304,#637,.T.);
#9440=EDGE_CURVE('',#7304,#7305,#638,.T.);
#9441=EDGE_CURVE('',#7305,#7306,#639,.T.);
#9442=EDGE_CURVE('',#7306,#7307,#640,.T.);
#9443=EDGE_CURVE('',#7307,#7308,#641,.T.);
#9444=EDGE_CURVE('',#7308,#7309,#642,.T.);
#9445=EDGE_CURVE('',#7309,#7310,#643,.T.);
#9446=EDGE_CURVE('',#7310,#7311,#644,.T.);
#9447=EDGE_CURVE('',#7311,#7312,#645,.T.);
#9448=EDGE_CURVE('',#7312,#7313,#646,.T.);
#9449=EDGE_CURVE('',#7313,#7314,#647,.T.);
#9450=EDGE_CURVE('',#7314,#7315,#648,.T.);
#9451=EDGE_CURVE('',#7315,#7316,#649,.T.);
#9452=EDGE_CURVE('',#7316,#7317,#650,.T.);
#9453=EDGE_CURVE('',#7317,#7318,#651,.T.);
#9454=EDGE_CURVE('',#7318,#7319,#652,.T.);
#9455=EDGE_CURVE('',#7319,#7320,#653,.T.);
#9456=EDGE_CURVE('',#7320,#7321,#654,.T.);
#9457=EDGE_CURVE('',#7321,#7322,#655,.T.);
#9458=EDGE_CURVE('',#7322,#7323,#656,.T.);
#9459=EDGE_CURVE('',#7323,#7324,#657,.T.);
#9460=EDGE_CURVE('',#7324,#7325,#658,.T.);
#9461=EDGE_CURVE('',#7325,#7274,#659,.T.);
#9462=EDGE_CURVE('',#7273,#7326,#660,.T.);
#9463=EDGE_CURVE('',#7327,#7326,#5951,.T.);
#9464=EDGE_CURVE('',#7328,#7327,#661,.T.);
#9465=EDGE_CURVE('',#7272,#7328,#662,.F.);
#9466=EDGE_CURVE('',#7329,#7330,#5952,.F.);
#9467=EDGE_CURVE('',#7329,#7327,#663,.T.);
#9468=EDGE_CURVE('',#7326,#7331,#664,.T.);
#9469=EDGE_CURVE('',#7331,#7302,#665,.T.);
#9470=EDGE_CURVE('',#7330,#7302,#5953,.F.);
#9471=EDGE_CURVE('',#7301,#7329,#666,.T.);
#9472=EDGE_CURVE('',#7332,#7276,#667,.T.);
#9473=EDGE_CURVE('',#7332,#7207,#668,.T.);
#9474=EDGE_CURVE('',#7276,#7333,#5954,.T.);
#9475=EDGE_CURVE('',#7333,#7334,#5955,.T.);
#9476=EDGE_CURVE('',#7334,#7208,#669,.T.);
#9477=EDGE_CURVE('',#7334,#7275,#670,.T.);
#9478=EDGE_CURVE('',#7335,#7336,#344,.T.);
#9479=EDGE_CURVE('',#7335,#7337,#5956,.T.);
#9480=EDGE_CURVE('',#7338,#7337,#345,.T.);
#9481=EDGE_CURVE('',#7339,#7338,#346,.T.);
#9482=EDGE_CURVE('',#7339,#7340,#5957,.T.);
#9483=EDGE_CURVE('',#7341,#7340,#347,.T.);
#9484=EDGE_CURVE('',#7342,#7341,#348,.T.);
#9485=EDGE_CURVE('',#7342,#7343,#5958,.T.);
#9486=EDGE_CURVE('',#7344,#7343,#349,.T.);
#9487=EDGE_CURVE('',#7345,#7344,#350,.T.);
#9488=EDGE_CURVE('',#7345,#7346,#5959,.T.);
#9489=EDGE_CURVE('',#7347,#7346,#351,.T.);
#9490=EDGE_CURVE('',#7348,#7347,#352,.T.);
#9491=EDGE_CURVE('',#7348,#7349,#5960,.T.);
#9492=EDGE_CURVE('',#7350,#7349,#353,.T.);
#9493=EDGE_CURVE('',#7351,#7350,#354,.T.);
#9494=EDGE_CURVE('',#7351,#7352,#5961,.T.);
#9495=EDGE_CURVE('',#7336,#7352,#355,.T.);
#9496=EDGE_CURVE('',#7336,#7353,#4251,.T.);
#9497=EDGE_CURVE('',#7353,#7353,#5962,.T.);
#9498=EDGE_CURVE('',#7343,#7354,#4252,.T.);
#9499=EDGE_CURVE('',#7355,#7342,#4253,.T.);
#9500=EDGE_CURVE('',#7354,#7355,#5963,.T.);
#9501=EDGE_CURVE('',#7346,#7356,#4254,.T.);
#9502=EDGE_CURVE('',#7357,#7345,#4255,.T.);
#9503=EDGE_CURVE('',#7356,#7357,#5964,.T.);
#9504=EDGE_CURVE('',#7358,#7339,#4256,.T.);
#9505=EDGE_CURVE('',#7359,#7358,#5965,.T.);
#9506=EDGE_CURVE('',#7340,#7359,#4257,.T.);
#9507=EDGE_CURVE('',#7349,#7360,#4258,.T.);
#9508=EDGE_CURVE('',#7361,#7348,#4259,.T.);
#9509=EDGE_CURVE('',#7360,#7361,#5966,.T.);
#9510=EDGE_CURVE('',#7362,#7335,#4260,.T.);
#9511=EDGE_CURVE('',#7363,#7362,#5967,.T.);
#9512=EDGE_CURVE('',#7337,#7363,#4261,.T.);
#9513=EDGE_CURVE('',#7364,#7351,#4262,.T.);
#9514=EDGE_CURVE('',#7365,#7364,#5968,.T.);
#9515=EDGE_CURVE('',#7352,#7365,#4263,.T.);
#9516=EDGE_CURVE('',#7361,#7360,#4264,.T.);
#9517=EDGE_CURVE('',#7347,#7366,#4265,.T.);
#9518=EDGE_CURVE('',#7366,#7367,#4266,.T.);
#9519=EDGE_CURVE('',#7350,#7367,#4267,.T.);
#9520=EDGE_CURVE('',#7357,#7356,#4268,.T.);
#9521=EDGE_CURVE('',#7344,#7368,#4269,.T.);
#9522=EDGE_CURVE('',#7368,#7366,#4270,.T.);
#9523=EDGE_CURVE('',#7355,#7354,#4271,.T.);
#9524=EDGE_CURVE('',#7341,#7369,#4272,.T.);
#9525=EDGE_CURVE('',#7369,#7368,#4273,.T.);
#9526=EDGE_CURVE('',#7358,#7359,#4274,.T.);
#9527=EDGE_CURVE('',#7362,#7363,#4275,.T.);
#9528=EDGE_CURVE('',#7364,#7365,#4276,.T.);
#9529=EDGE_CURVE('',#7370,#7369,#4277,.T.);
#9530=EDGE_CURVE('',#7370,#7369,#5969,.T.);
#9531=EDGE_CURVE('',#7369,#7368,#5970,.T.);
#9532=EDGE_CURVE('',#7368,#7366,#5971,.T.);
#9533=EDGE_CURVE('',#7366,#7367,#5972,.T.);
#9534=EDGE_CURVE('',#7367,#7371,#4278,.T.);
#9535=EDGE_CURVE('',#7367,#7371,#5973,.T.);
#9536=EDGE_CURVE('',#7371,#7370,#4279,.T.);
#9537=EDGE_CURVE('',#7371,#7370,#5974,.T.);
#9538=EDGE_CURVE('',#7372,#7371,#4280,.T.);
#9539=EDGE_CURVE('',#7338,#7370,#4281,.T.);
#9540=EDGE_CURVE('',#7336,#7371,#4282,.T.);
#9541=EDGE_CURVE('',#7373,#7373,#5975,.T.);
#9542=EDGE_CURVE('',#7333,#7373,#4283,.T.);
#9543=EDGE_CURVE('',#7330,#7374,#4284,.T.);
#9544=EDGE_CURVE('',#7374,#7374,#5976,.T.);
#13312=ORIENTED_EDGE('',*,*,#9319,.F.);
#13313=ORIENTED_EDGE('',*,*,#9320,.F.);
#13314=ORIENTED_EDGE('',*,*,#9321,.F.);
#13315=ORIENTED_EDGE('',*,*,#9322,.T.);
#13316=ORIENTED_EDGE('',*,*,#9323,.F.);
#13317=ORIENTED_EDGE('',*,*,#9324,.F.);
#13318=ORIENTED_EDGE('',*,*,#9319,.T.);
#13319=ORIENTED_EDGE('',*,*,#9325,.T.);
#13320=ORIENTED_EDGE('',*,*,#9326,.T.);
#13321=ORIENTED_EDGE('',*,*,#9327,.F.);
#13322=ORIENTED_EDGE('',*,*,#9328,.F.);
#13323=ORIENTED_EDGE('',*,*,#9323,.T.);
#13324=ORIENTED_EDGE('',*,*,#9329,.T.);
#13325=ORIENTED_EDGE('',*,*,#9330,.F.);
#13326=ORIENTED_EDGE('',*,*,#9331,.F.);
#13327=ORIENTED_EDGE('',*,*,#9327,.T.);
#13328=ORIENTED_EDGE('',*,*,#9332,.T.);
#13329=ORIENTED_EDGE('',*,*,#9333,.T.);
#13330=ORIENTED_EDGE('',*,*,#9334,.F.);
#13331=ORIENTED_EDGE('',*,*,#9335,.F.);
#13332=ORIENTED_EDGE('',*,*,#9336,.F.);
#13333=ORIENTED_EDGE('',*,*,#9330,.T.);
#13334=ORIENTED_EDGE('',*,*,#9337,.T.);
#13335=ORIENTED_EDGE('',*,*,#9338,.T.);
#13336=ORIENTED_EDGE('',*,*,#9339,.F.);
#13337=ORIENTED_EDGE('',*,*,#9340,.F.);
#13338=ORIENTED_EDGE('',*,*,#9334,.T.);
#13339=ORIENTED_EDGE('',*,*,#9341,.T.);
#13340=ORIENTED_EDGE('',*,*,#9342,.F.);
#13341=ORIENTED_EDGE('',*,*,#9343,.F.);
#13342=ORIENTED_EDGE('',*,*,#9344,.F.);
#13343=ORIENTED_EDGE('',*,*,#9339,.T.);
#13344=ORIENTED_EDGE('',*,*,#9345,.T.);
#13345=ORIENTED_EDGE('',*,*,#9346,.T.);
#13346=ORIENTED_EDGE('',*,*,#9347,.F.);
#13347=ORIENTED_EDGE('',*,*,#9348,.F.);
#13348=ORIENTED_EDGE('',*,*,#9342,.T.);
#13349=ORIENTED_EDGE('',*,*,#9349,.T.);
#13350=ORIENTED_EDGE('',*,*,#9350,.F.);
#13351=ORIENTED_EDGE('',*,*,#9351,.F.);
#13352=ORIENTED_EDGE('',*,*,#9352,.F.);
#13353=ORIENTED_EDGE('',*,*,#9347,.T.);
#13354=ORIENTED_EDGE('',*,*,#9353,.T.);
#13355=ORIENTED_EDGE('',*,*,#9354,.T.);
#13356=ORIENTED_EDGE('',*,*,#9355,.F.);
#13357=ORIENTED_EDGE('',*,*,#9356,.F.);
#13358=ORIENTED_EDGE('',*,*,#9350,.T.);
#13359=ORIENTED_EDGE('',*,*,#9357,.T.);
#13360=ORIENTED_EDGE('',*,*,#9358,.F.);
#13361=ORIENTED_EDGE('',*,*,#9359,.F.);
#13362=ORIENTED_EDGE('',*,*,#9360,.F.);
#13363=ORIENTED_EDGE('',*,*,#9355,.T.);
#13364=ORIENTED_EDGE('',*,*,#9361,.T.);
#13365=ORIENTED_EDGE('',*,*,#9362,.T.);
#13366=ORIENTED_EDGE('',*,*,#9363,.F.);
#13367=ORIENTED_EDGE('',*,*,#9364,.F.);
#13368=ORIENTED_EDGE('',*,*,#9365,.F.);
#13369=ORIENTED_EDGE('',*,*,#9358,.T.);
#13370=ORIENTED_EDGE('',*,*,#9366,.T.);
#13371=ORIENTED_EDGE('',*,*,#9367,.F.);
#13372=ORIENTED_EDGE('',*,*,#9368,.F.);
#13373=ORIENTED_EDGE('',*,*,#9363,.T.);
#13374=ORIENTED_EDGE('',*,*,#9369,.T.);
#13375=ORIENTED_EDGE('',*,*,#9370,.T.);
#13376=ORIENTED_EDGE('',*,*,#9371,.F.);
#13377=ORIENTED_EDGE('',*,*,#9372,.F.);
#13378=ORIENTED_EDGE('',*,*,#9373,.F.);
#13379=ORIENTED_EDGE('',*,*,#9367,.T.);
#13380=ORIENTED_EDGE('',*,*,#9374,.T.);
#13381=ORIENTED_EDGE('',*,*,#9375,.F.);
#13382=ORIENTED_EDGE('',*,*,#9376,.F.);
#13383=ORIENTED_EDGE('',*,*,#9371,.T.);
#13384=ORIENTED_EDGE('',*,*,#9377,.T.);
#13385=ORIENTED_EDGE('',*,*,#9378,.T.);
#13386=ORIENTED_EDGE('',*,*,#9379,.F.);
#13387=ORIENTED_EDGE('',*,*,#9380,.F.);
#13388=ORIENTED_EDGE('',*,*,#9381,.F.);
#13389=ORIENTED_EDGE('',*,*,#9375,.T.);
#13390=ORIENTED_EDGE('',*,*,#9382,.T.);
#13391=ORIENTED_EDGE('',*,*,#9383,.F.);
#13392=ORIENTED_EDGE('',*,*,#9384,.F.);
#13393=ORIENTED_EDGE('',*,*,#9379,.T.);
#13394=ORIENTED_EDGE('',*,*,#9385,.T.);
#13395=ORIENTED_EDGE('',*,*,#9386,.T.);
#13396=ORIENTED_EDGE('',*,*,#9387,.F.);
#13397=ORIENTED_EDGE('',*,*,#9388,.F.);
#13398=ORIENTED_EDGE('',*,*,#9389,.F.);
#13399=ORIENTED_EDGE('',*,*,#9383,.T.);
#13400=ORIENTED_EDGE('',*,*,#9390,.T.);
#13401=ORIENTED_EDGE('',*,*,#9391,.F.);
#13402=ORIENTED_EDGE('',*,*,#9392,.F.);
#13403=ORIENTED_EDGE('',*,*,#9387,.T.);
#13404=ORIENTED_EDGE('',*,*,#9393,.T.);
#13405=ORIENTED_EDGE('',*,*,#9394,.T.);
#13406=ORIENTED_EDGE('',*,*,#9395,.F.);
#13407=ORIENTED_EDGE('',*,*,#9396,.F.);
#13408=ORIENTED_EDGE('',*,*,#9397,.F.);
#13409=ORIENTED_EDGE('',*,*,#9391,.T.);
#13410=ORIENTED_EDGE('',*,*,#9398,.T.);
#13411=ORIENTED_EDGE('',*,*,#9399,.F.);
#13412=ORIENTED_EDGE('',*,*,#9400,.F.);
#13413=ORIENTED_EDGE('',*,*,#9395,.T.);
#13414=ORIENTED_EDGE('',*,*,#9401,.T.);
#13415=ORIENTED_EDGE('',*,*,#9402,.T.);
#13416=ORIENTED_EDGE('',*,*,#9403,.F.);
#13417=ORIENTED_EDGE('',*,*,#9404,.F.);
#13418=ORIENTED_EDGE('',*,*,#9405,.F.);
#13419=ORIENTED_EDGE('',*,*,#9399,.T.);
#13420=ORIENTED_EDGE('',*,*,#9406,.T.);
#13421=ORIENTED_EDGE('',*,*,#9407,.F.);
#13422=ORIENTED_EDGE('',*,*,#9408,.F.);
#13423=ORIENTED_EDGE('',*,*,#9403,.T.);
#13424=ORIENTED_EDGE('',*,*,#9409,.T.);
#13425=ORIENTED_EDGE('',*,*,#9410,.T.);
#13426=ORIENTED_EDGE('',*,*,#9411,.T.);
#13427=ORIENTED_EDGE('',*,*,#9412,.T.);
#13428=ORIENTED_EDGE('',*,*,#9413,.T.);
#13429=ORIENTED_EDGE('',*,*,#9414,.T.);
#13430=ORIENTED_EDGE('',*,*,#9415,.T.);
#13431=ORIENTED_EDGE('',*,*,#9416,.T.);
#13432=ORIENTED_EDGE('',*,*,#9417,.T.);
#13433=ORIENTED_EDGE('',*,*,#9418,.T.);
#13434=ORIENTED_EDGE('',*,*,#9419,.T.);
#13435=ORIENTED_EDGE('',*,*,#9420,.T.);
#13436=ORIENTED_EDGE('',*,*,#9421,.T.);
#13437=ORIENTED_EDGE('',*,*,#9422,.T.);
#13438=ORIENTED_EDGE('',*,*,#9423,.T.);
#13439=ORIENTED_EDGE('',*,*,#9424,.T.);
#13440=ORIENTED_EDGE('',*,*,#9425,.T.);
#13441=ORIENTED_EDGE('',*,*,#9426,.T.);
#13442=ORIENTED_EDGE('',*,*,#9427,.T.);
#13443=ORIENTED_EDGE('',*,*,#9428,.T.);
#13444=ORIENTED_EDGE('',*,*,#9429,.T.);
#13445=ORIENTED_EDGE('',*,*,#9430,.T.);
#13446=ORIENTED_EDGE('',*,*,#9431,.T.);
#13447=ORIENTED_EDGE('',*,*,#9432,.T.);
#13448=ORIENTED_EDGE('',*,*,#9433,.T.);
#13449=ORIENTED_EDGE('',*,*,#9434,.T.);
#13450=ORIENTED_EDGE('',*,*,#9435,.T.);
#13451=ORIENTED_EDGE('',*,*,#9436,.T.);
#13452=ORIENTED_EDGE('',*,*,#9437,.F.);
#13453=ORIENTED_EDGE('',*,*,#9438,.T.);
#13454=ORIENTED_EDGE('',*,*,#9439,.T.);
#13455=ORIENTED_EDGE('',*,*,#9440,.T.);
#13456=ORIENTED_EDGE('',*,*,#9441,.T.);
#13457=ORIENTED_EDGE('',*,*,#9442,.T.);
#13458=ORIENTED_EDGE('',*,*,#9443,.T.);
#13459=ORIENTED_EDGE('',*,*,#9444,.T.);
#13460=ORIENTED_EDGE('',*,*,#9445,.T.);
#13461=ORIENTED_EDGE('',*,*,#9446,.T.);
#13462=ORIENTED_EDGE('',*,*,#9447,.T.);
#13463=ORIENTED_EDGE('',*,*,#9448,.T.);
#13464=ORIENTED_EDGE('',*,*,#9449,.T.);
#13465=ORIENTED_EDGE('',*,*,#9450,.T.);
#13466=ORIENTED_EDGE('',*,*,#9451,.T.);
#13467=ORIENTED_EDGE('',*,*,#9452,.T.);
#13468=ORIENTED_EDGE('',*,*,#9453,.T.);
#13469=ORIENTED_EDGE('',*,*,#9454,.T.);
#13470=ORIENTED_EDGE('',*,*,#9455,.T.);
#13471=ORIENTED_EDGE('',*,*,#9456,.T.);
#13472=ORIENTED_EDGE('',*,*,#9457,.T.);
#13473=ORIENTED_EDGE('',*,*,#9458,.T.);
#13474=ORIENTED_EDGE('',*,*,#9459,.T.);
#13475=ORIENTED_EDGE('',*,*,#9460,.T.);
#13476=ORIENTED_EDGE('',*,*,#9461,.T.);
#13477=ORIENTED_EDGE('',*,*,#9407,.T.);
#13478=ORIENTED_EDGE('',*,*,#9462,.T.);
#13479=ORIENTED_EDGE('',*,*,#9463,.F.);
#13480=ORIENTED_EDGE('',*,*,#9464,.F.);
#13481=ORIENTED_EDGE('',*,*,#9465,.F.);
#13482=ORIENTED_EDGE('',*,*,#9466,.F.);
#13483=ORIENTED_EDGE('',*,*,#9467,.T.);
#13484=ORIENTED_EDGE('',*,*,#9463,.T.);
#13485=ORIENTED_EDGE('',*,*,#9468,.T.);
#13486=ORIENTED_EDGE('',*,*,#9469,.T.);
#13487=ORIENTED_EDGE('',*,*,#9470,.F.);
#13488=ORIENTED_EDGE('',*,*,#9467,.F.);
#13489=ORIENTED_EDGE('',*,*,#9471,.F.);
#13490=ORIENTED_EDGE('',*,*,#9436,.F.);
#13491=ORIENTED_EDGE('',*,*,#9435,.F.);
#13492=ORIENTED_EDGE('',*,*,#9434,.F.);
#13493=ORIENTED_EDGE('',*,*,#9433,.F.);
#13494=ORIENTED_EDGE('',*,*,#9432,.F.);
#13495=ORIENTED_EDGE('',*,*,#9431,.F.);
#13496=ORIENTED_EDGE('',*,*,#9430,.F.);
#13497=ORIENTED_EDGE('',*,*,#9429,.F.);
#13498=ORIENTED_EDGE('',*,*,#9428,.F.);
#13499=ORIENTED_EDGE('',*,*,#9427,.F.);
#13500=ORIENTED_EDGE('',*,*,#9426,.F.);
#13501=ORIENTED_EDGE('',*,*,#9425,.F.);
#13502=ORIENTED_EDGE('',*,*,#9424,.F.);
#13503=ORIENTED_EDGE('',*,*,#9423,.F.);
#13504=ORIENTED_EDGE('',*,*,#9422,.F.);
#13505=ORIENTED_EDGE('',*,*,#9421,.F.);
#13506=ORIENTED_EDGE('',*,*,#9420,.F.);
#13507=ORIENTED_EDGE('',*,*,#9419,.F.);
#13508=ORIENTED_EDGE('',*,*,#9418,.F.);
#13509=ORIENTED_EDGE('',*,*,#9417,.F.);
#13510=ORIENTED_EDGE('',*,*,#9416,.F.);
#13511=ORIENTED_EDGE('',*,*,#9415,.F.);
#13512=ORIENTED_EDGE('',*,*,#9414,.F.);
#13513=ORIENTED_EDGE('',*,*,#9413,.F.);
#13514=ORIENTED_EDGE('',*,*,#9412,.F.);
#13515=ORIENTED_EDGE('',*,*,#9472,.F.);
#13516=ORIENTED_EDGE('',*,*,#9473,.T.);
#13517=ORIENTED_EDGE('',*,*,#9320,.T.);
#13518=ORIENTED_EDGE('',*,*,#9324,.T.);
#13519=ORIENTED_EDGE('',*,*,#9328,.T.);
#13520=ORIENTED_EDGE('',*,*,#9331,.T.);
#13521=ORIENTED_EDGE('',*,*,#9336,.T.);
#13522=ORIENTED_EDGE('',*,*,#9335,.T.);
#13523=ORIENTED_EDGE('',*,*,#9340,.T.);
#13524=ORIENTED_EDGE('',*,*,#9344,.T.);
#13525=ORIENTED_EDGE('',*,*,#9343,.T.);
#13526=ORIENTED_EDGE('',*,*,#9348,.T.);
#13527=ORIENTED_EDGE('',*,*,#9352,.T.);
#13528=ORIENTED_EDGE('',*,*,#9351,.T.);
#13529=ORIENTED_EDGE('',*,*,#9356,.T.);
#13530=ORIENTED_EDGE('',*,*,#9360,.T.);
#13531=ORIENTED_EDGE('',*,*,#9359,.T.);
#13532=ORIENTED_EDGE('',*,*,#9365,.T.);
#13533=ORIENTED_EDGE('',*,*,#9364,.T.);
#13534=ORIENTED_EDGE('',*,*,#9368,.T.);
#13535=ORIENTED_EDGE('',*,*,#9373,.T.);
#13536=ORIENTED_EDGE('',*,*,#9372,.T.);
#13537=ORIENTED_EDGE('',*,*,#9376,.T.);
#13538=ORIENTED_EDGE('',*,*,#9381,.T.);
#13539=ORIENTED_EDGE('',*,*,#9380,.T.);
#13540=ORIENTED_EDGE('',*,*,#9384,.T.);
#13541=ORIENTED_EDGE('',*,*,#9389,.T.);
#13542=ORIENTED_EDGE('',*,*,#9388,.T.);
#13543=ORIENTED_EDGE('',*,*,#9392,.T.);
#13544=ORIENTED_EDGE('',*,*,#9397,.T.);
#13545=ORIENTED_EDGE('',*,*,#9396,.T.);
#13546=ORIENTED_EDGE('',*,*,#9400,.T.);
#13547=ORIENTED_EDGE('',*,*,#9405,.T.);
#13548=ORIENTED_EDGE('',*,*,#9404,.T.);
#13549=ORIENTED_EDGE('',*,*,#9408,.T.);
#13550=ORIENTED_EDGE('',*,*,#9465,.T.);
#13551=ORIENTED_EDGE('',*,*,#9464,.T.);
#13552=ORIENTED_EDGE('',*,*,#9474,.T.);
#13553=ORIENTED_EDGE('',*,*,#9475,.T.);
#13554=ORIENTED_EDGE('',*,*,#9476,.T.);
#13555=ORIENTED_EDGE('',*,*,#9321,.T.);
#13556=ORIENTED_EDGE('',*,*,#9473,.F.);
#13557=ORIENTED_EDGE('',*,*,#9472,.T.);
#13558=ORIENTED_EDGE('',*,*,#9469,.F.);
#13559=ORIENTED_EDGE('',*,*,#9468,.F.);
#13560=ORIENTED_EDGE('',*,*,#9462,.F.);
#13561=ORIENTED_EDGE('',*,*,#9409,.F.);
#13562=ORIENTED_EDGE('',*,*,#9406,.F.);
#13563=ORIENTED_EDGE('',*,*,#9402,.F.);
#13564=ORIENTED_EDGE('',*,*,#9401,.F.);
#13565=ORIENTED_EDGE('',*,*,#9398,.F.);
#13566=ORIENTED_EDGE('',*,*,#9394,.F.);
#13567=ORIENTED_EDGE('',*,*,#9393,.F.);
#13568=ORIENTED_EDGE('',*,*,#9390,.F.);
#13569=ORIENTED_EDGE('',*,*,#9386,.F.);
#13570=ORIENTED_EDGE('',*,*,#9385,.F.);
#13571=ORIENTED_EDGE('',*,*,#9382,.F.);
#13572=ORIENTED_EDGE('',*,*,#9378,.F.);
#13573=ORIENTED_EDGE('',*,*,#9377,.F.);
#13574=ORIENTED_EDGE('',*,*,#9374,.F.);
#13575=ORIENTED_EDGE('',*,*,#9370,.F.);
#13576=ORIENTED_EDGE('',*,*,#9369,.F.);
#13577=ORIENTED_EDGE('',*,*,#9366,.F.);
#13578=ORIENTED_EDGE('',*,*,#9362,.F.);
#13579=ORIENTED_EDGE('',*,*,#9361,.F.);
#13580=ORIENTED_EDGE('',*,*,#9357,.F.);
#13581=ORIENTED_EDGE('',*,*,#9354,.F.);
#13582=ORIENTED_EDGE('',*,*,#9353,.F.);
#13583=ORIENTED_EDGE('',*,*,#9349,.F.);
#13584=ORIENTED_EDGE('',*,*,#9346,.F.);
#13585=ORIENTED_EDGE('',*,*,#9345,.F.);
#13586=ORIENTED_EDGE('',*,*,#9341,.F.);
#13587=ORIENTED_EDGE('',*,*,#9338,.F.);
#13588=ORIENTED_EDGE('',*,*,#9337,.F.);
#13589=ORIENTED_EDGE('',*,*,#9333,.F.);
#13590=ORIENTED_EDGE('',*,*,#9332,.F.);
#13591=ORIENTED_EDGE('',*,*,#9329,.F.);
#13592=ORIENTED_EDGE('',*,*,#9326,.F.);
#13593=ORIENTED_EDGE('',*,*,#9325,.F.);
#13594=ORIENTED_EDGE('',*,*,#9322,.F.);
#13595=ORIENTED_EDGE('',*,*,#9476,.F.);
#13596=ORIENTED_EDGE('',*,*,#9477,.T.);
#13597=ORIENTED_EDGE('',*,*,#9410,.F.);
#13598=ORIENTED_EDGE('',*,*,#9461,.F.);
#13599=ORIENTED_EDGE('',*,*,#9460,.F.);
#13600=ORIENTED_EDGE('',*,*,#9459,.F.);
#13601=ORIENTED_EDGE('',*,*,#9458,.F.);
#13602=ORIENTED_EDGE('',*,*,#9457,.F.);
#13603=ORIENTED_EDGE('',*,*,#9456,.F.);
#13604=ORIENTED_EDGE('',*,*,#9455,.F.);
#13605=ORIENTED_EDGE('',*,*,#9454,.F.);
#13606=ORIENTED_EDGE('',*,*,#9453,.F.);
#13607=ORIENTED_EDGE('',*,*,#9452,.F.);
#13608=ORIENTED_EDGE('',*,*,#9451,.F.);
#13609=ORIENTED_EDGE('',*,*,#9450,.F.);
#13610=ORIENTED_EDGE('',*,*,#9449,.F.);
#13611=ORIENTED_EDGE('',*,*,#9448,.F.);
#13612=ORIENTED_EDGE('',*,*,#9447,.F.);
#13613=ORIENTED_EDGE('',*,*,#9446,.F.);
#13614=ORIENTED_EDGE('',*,*,#9445,.F.);
#13615=ORIENTED_EDGE('',*,*,#9444,.F.);
#13616=ORIENTED_EDGE('',*,*,#9443,.F.);
#13617=ORIENTED_EDGE('',*,*,#9442,.F.);
#13618=ORIENTED_EDGE('',*,*,#9441,.F.);
#13619=ORIENTED_EDGE('',*,*,#9440,.F.);
#13620=ORIENTED_EDGE('',*,*,#9439,.F.);
#13621=ORIENTED_EDGE('',*,*,#9438,.F.);
#13622=ORIENTED_EDGE('',*,*,#9478,.F.);
#13623=ORIENTED_EDGE('',*,*,#9479,.T.);
#13624=ORIENTED_EDGE('',*,*,#9480,.F.);
#13625=ORIENTED_EDGE('',*,*,#9481,.F.);
#13626=ORIENTED_EDGE('',*,*,#9482,.T.);
#13627=ORIENTED_EDGE('',*,*,#9483,.F.);
#13628=ORIENTED_EDGE('',*,*,#9484,.F.);
#13629=ORIENTED_EDGE('',*,*,#9485,.T.);
#13630=ORIENTED_EDGE('',*,*,#9486,.F.);
#13631=ORIENTED_EDGE('',*,*,#9487,.F.);
#13632=ORIENTED_EDGE('',*,*,#9488,.T.);
#13633=ORIENTED_EDGE('',*,*,#9489,.F.);
#13634=ORIENTED_EDGE('',*,*,#9490,.F.);
#13635=ORIENTED_EDGE('',*,*,#9491,.T.);
#13636=ORIENTED_EDGE('',*,*,#9492,.F.);
#13637=ORIENTED_EDGE('',*,*,#9493,.F.);
#13638=ORIENTED_EDGE('',*,*,#9494,.T.);
#13639=ORIENTED_EDGE('',*,*,#9495,.F.);
#13640=ORIENTED_EDGE('',*,*,#9496,.T.);
#13641=ORIENTED_EDGE('',*,*,#9497,.F.);
#13642=ORIENTED_EDGE('',*,*,#9496,.F.);
#13643=ORIENTED_EDGE('',*,*,#9498,.F.);
#13644=ORIENTED_EDGE('',*,*,#9485,.F.);
#13645=ORIENTED_EDGE('',*,*,#9499,.F.);
#13646=ORIENTED_EDGE('',*,*,#9500,.F.);
#13647=ORIENTED_EDGE('',*,*,#9501,.F.);
#13648=ORIENTED_EDGE('',*,*,#9488,.F.);
#13649=ORIENTED_EDGE('',*,*,#9502,.F.);
#13650=ORIENTED_EDGE('',*,*,#9503,.F.);
#13651=ORIENTED_EDGE('',*,*,#9504,.F.);
#13652=ORIENTED_EDGE('',*,*,#9505,.F.);
#13653=ORIENTED_EDGE('',*,*,#9506,.F.);
#13654=ORIENTED_EDGE('',*,*,#9482,.F.);
#13655=ORIENTED_EDGE('',*,*,#9507,.F.);
#13656=ORIENTED_EDGE('',*,*,#9491,.F.);
#13657=ORIENTED_EDGE('',*,*,#9508,.F.);
#13658=ORIENTED_EDGE('',*,*,#9509,.F.);
#13659=ORIENTED_EDGE('',*,*,#9510,.F.);
#13660=ORIENTED_EDGE('',*,*,#9511,.F.);
#13661=ORIENTED_EDGE('',*,*,#9512,.F.);
#13662=ORIENTED_EDGE('',*,*,#9479,.F.);
#13663=ORIENTED_EDGE('',*,*,#9513,.F.);
#13664=ORIENTED_EDGE('',*,*,#9514,.F.);
#13665=ORIENTED_EDGE('',*,*,#9515,.F.);
#13666=ORIENTED_EDGE('',*,*,#9494,.F.);
#13667=ORIENTED_EDGE('',*,*,#9492,.T.);
#13668=ORIENTED_EDGE('',*,*,#9507,.T.);
#13669=ORIENTED_EDGE('',*,*,#9516,.F.);
#13670=ORIENTED_EDGE('',*,*,#9508,.T.);
#13671=ORIENTED_EDGE('',*,*,#9490,.T.);
#13672=ORIENTED_EDGE('',*,*,#9517,.T.);
#13673=ORIENTED_EDGE('',*,*,#9518,.T.);
#13674=ORIENTED_EDGE('',*,*,#9519,.F.);
#13675=ORIENTED_EDGE('',*,*,#9489,.T.);
#13676=ORIENTED_EDGE('',*,*,#9501,.T.);
#13677=ORIENTED_EDGE('',*,*,#9520,.F.);
#13678=ORIENTED_EDGE('',*,*,#9502,.T.);
#13679=ORIENTED_EDGE('',*,*,#9487,.T.);
#13680=ORIENTED_EDGE('',*,*,#9521,.T.);
#13681=ORIENTED_EDGE('',*,*,#9522,.T.);
#13682=ORIENTED_EDGE('',*,*,#9517,.F.);
#13683=ORIENTED_EDGE('',*,*,#9486,.T.);
#13684=ORIENTED_EDGE('',*,*,#9498,.T.);
#13685=ORIENTED_EDGE('',*,*,#9523,.F.);
#13686=ORIENTED_EDGE('',*,*,#9499,.T.);
#13687=ORIENTED_EDGE('',*,*,#9484,.T.);
#13688=ORIENTED_EDGE('',*,*,#9524,.T.);
#13689=ORIENTED_EDGE('',*,*,#9525,.T.);
#13690=ORIENTED_EDGE('',*,*,#9521,.F.);
#13691=ORIENTED_EDGE('',*,*,#9500,.T.);
#13692=ORIENTED_EDGE('',*,*,#9523,.T.);
#13693=ORIENTED_EDGE('',*,*,#9503,.T.);
#13694=ORIENTED_EDGE('',*,*,#9520,.T.);
#13695=ORIENTED_EDGE('',*,*,#9505,.T.);
#13696=ORIENTED_EDGE('',*,*,#9526,.T.);
#13697=ORIENTED_EDGE('',*,*,#9509,.T.);
#13698=ORIENTED_EDGE('',*,*,#9516,.T.);
#13699=ORIENTED_EDGE('',*,*,#9511,.T.);
#13700=ORIENTED_EDGE('',*,*,#9527,.T.);
#13701=ORIENTED_EDGE('',*,*,#9514,.T.);
#13702=ORIENTED_EDGE('',*,*,#9528,.T.);
#13703=ORIENTED_EDGE('',*,*,#9529,.F.);
#13704=ORIENTED_EDGE('',*,*,#9530,.T.);
#13705=ORIENTED_EDGE('',*,*,#9525,.F.);
#13706=ORIENTED_EDGE('',*,*,#9531,.T.);
#13707=ORIENTED_EDGE('',*,*,#9522,.F.);
#13708=ORIENTED_EDGE('',*,*,#9532,.T.);
#13709=ORIENTED_EDGE('',*,*,#9518,.F.);
#13710=ORIENTED_EDGE('',*,*,#9533,.T.);
#13711=ORIENTED_EDGE('',*,*,#9534,.F.);
#13712=ORIENTED_EDGE('',*,*,#9535,.T.);
#13713=ORIENTED_EDGE('',*,*,#9536,.F.);
#13714=ORIENTED_EDGE('',*,*,#9537,.T.);
#13715=ORIENTED_EDGE('',*,*,#9538,.T.);
#13716=ORIENTED_EDGE('',*,*,#9535,.F.);
#13717=ORIENTED_EDGE('',*,*,#9533,.F.);
#13718=ORIENTED_EDGE('',*,*,#9532,.F.);
#13719=ORIENTED_EDGE('',*,*,#9531,.F.);
#13720=ORIENTED_EDGE('',*,*,#9530,.F.);
#13721=ORIENTED_EDGE('',*,*,#9537,.F.);
#13722=ORIENTED_EDGE('',*,*,#9538,.F.);
#13723=ORIENTED_EDGE('',*,*,#9481,.T.);
#13724=ORIENTED_EDGE('',*,*,#9539,.T.);
#13725=ORIENTED_EDGE('',*,*,#9529,.T.);
#13726=ORIENTED_EDGE('',*,*,#9524,.F.);
#13727=ORIENTED_EDGE('',*,*,#9483,.T.);
#13728=ORIENTED_EDGE('',*,*,#9506,.T.);
#13729=ORIENTED_EDGE('',*,*,#9526,.F.);
#13730=ORIENTED_EDGE('',*,*,#9504,.T.);
#13731=ORIENTED_EDGE('',*,*,#9478,.T.);
#13732=ORIENTED_EDGE('',*,*,#9540,.T.);
#13733=ORIENTED_EDGE('',*,*,#9536,.T.);
#13734=ORIENTED_EDGE('',*,*,#9539,.F.);
#13735=ORIENTED_EDGE('',*,*,#9480,.T.);
#13736=ORIENTED_EDGE('',*,*,#9512,.T.);
#13737=ORIENTED_EDGE('',*,*,#9527,.F.);
#13738=ORIENTED_EDGE('',*,*,#9510,.T.);
#13739=ORIENTED_EDGE('',*,*,#9493,.T.);
#13740=ORIENTED_EDGE('',*,*,#9519,.T.);
#13741=ORIENTED_EDGE('',*,*,#9534,.T.);
#13742=ORIENTED_EDGE('',*,*,#9540,.F.);
#13743=ORIENTED_EDGE('',*,*,#9495,.T.);
#13744=ORIENTED_EDGE('',*,*,#9515,.T.);
#13745=ORIENTED_EDGE('',*,*,#9528,.F.);
#13746=ORIENTED_EDGE('',*,*,#9513,.T.);
#13747=ORIENTED_EDGE('',*,*,#9541,.F.);
#13748=ORIENTED_EDGE('',*,*,#9497,.T.);
#13749=ORIENTED_EDGE('',*,*,#9477,.F.);
#13750=ORIENTED_EDGE('',*,*,#9475,.F.);
#13751=ORIENTED_EDGE('',*,*,#9542,.T.);
#13752=ORIENTED_EDGE('',*,*,#9541,.T.);
#13753=ORIENTED_EDGE('',*,*,#9542,.F.);
#13754=ORIENTED_EDGE('',*,*,#9474,.F.);
#13755=ORIENTED_EDGE('',*,*,#9411,.F.);
#13756=ORIENTED_EDGE('',*,*,#9466,.T.);
#13757=ORIENTED_EDGE('',*,*,#9543,.T.);
#13758=ORIENTED_EDGE('',*,*,#9544,.F.);
#13759=ORIENTED_EDGE('',*,*,#9543,.F.);
#13760=ORIENTED_EDGE('',*,*,#9470,.T.);
#13761=ORIENTED_EDGE('',*,*,#9437,.T.);
#13762=ORIENTED_EDGE('',*,*,#9471,.T.);
#13763=ORIENTED_EDGE('',*,*,#9544,.T.);
#14331=CONICAL_SURFACE('',#16399,1.49337567297406,0.785398163397437);
#14332=CONICAL_SURFACE('',#16440,1.44337567297407,1.02974425867665);
#14333=CONICAL_SURFACE('',#16446,2.26,0.785398163397448);
#14334=CONICAL_SURFACE('',#16447,2.125,0.785398163397448);
#14961=ADVANCED_FACE('',(#2226),#1024,.T.);
#14962=ADVANCED_FACE('',(#2227),#1025,.T.);
#14963=ADVANCED_FACE('',(#2228),#1026,.T.);
#14964=ADVANCED_FACE('',(#2229),#1027,.T.);
#14965=ADVANCED_FACE('',(#2230),#1028,.T.);
#14966=ADVANCED_FACE('',(#2231),#1029,.T.);
#14967=ADVANCED_FACE('',(#2232),#1030,.T.);
#14968=ADVANCED_FACE('',(#2233),#1031,.T.);
#14969=ADVANCED_FACE('',(#2234),#1032,.T.);
#14970=ADVANCED_FACE('',(#2235),#1033,.T.);
#14971=ADVANCED_FACE('',(#2236),#1034,.T.);
#14972=ADVANCED_FACE('',(#2237),#1035,.T.);
#14973=ADVANCED_FACE('',(#2238),#1036,.T.);
#14974=ADVANCED_FACE('',(#2239),#1037,.T.);
#14975=ADVANCED_FACE('',(#2240),#1038,.T.);
#14976=ADVANCED_FACE('',(#2241),#1039,.T.);
#14977=ADVANCED_FACE('',(#2242),#1040,.T.);
#14978=ADVANCED_FACE('',(#2243),#1041,.T.);
#14979=ADVANCED_FACE('',(#2244),#1042,.T.);
#14980=ADVANCED_FACE('',(#2245),#1043,.T.);
#14981=ADVANCED_FACE('',(#2246),#1044,.T.);
#14982=ADVANCED_FACE('',(#2247),#1045,.T.);
#14983=ADVANCED_FACE('',(#2248),#1046,.T.);
#14984=ADVANCED_FACE('',(#2249),#1047,.T.);
#14985=ADVANCED_FACE('',(#2250),#1048,.T.);
#14986=ADVANCED_FACE('',(#2251),#1561,.F.);
#14987=ADVANCED_FACE('',(#2252),#366,.F.);
#14988=ADVANCED_FACE('',(#2253),#1562,.T.);
#14989=ADVANCED_FACE('',(#2254),#367,.F.);
#14990=ADVANCED_FACE('',(#2255),#14331,.F.);
#14991=ADVANCED_FACE('',(#2256),#1049,.T.);
#14992=ADVANCED_FACE('',(#2257),#1050,.T.);
#14993=ADVANCED_FACE('',(#2258),#1051,.T.);
#14994=ADVANCED_FACE('',(#2259),#1052,.T.);
#14995=ADVANCED_FACE('',(#2260),#1053,.T.);
#14996=ADVANCED_FACE('',(#2261),#1054,.T.);
#14997=ADVANCED_FACE('',(#2262),#1563,.F.);
#14998=ADVANCED_FACE('',(#2263),#1564,.F.);
#14999=ADVANCED_FACE('',(#2264),#1565,.F.);
#15000=ADVANCED_FACE('',(#2265),#1566,.T.);
#15001=ADVANCED_FACE('',(#2266),#1567,.T.);
#15002=ADVANCED_FACE('',(#2267),#1568,.T.);
#15003=ADVANCED_FACE('',(#2268),#1569,.T.);
#15004=ADVANCED_FACE('',(#2269),#1570,.T.);
#15005=ADVANCED_FACE('',(#2270),#1571,.T.);
#15006=ADVANCED_FACE('',(#2271),#1572,.F.);
#15007=ADVANCED_FACE('',(#2272),#1573,.F.);
#15008=ADVANCED_FACE('',(#2273),#1574,.F.);
#15009=ADVANCED_FACE('',(#2274),#1575,.F.);
#15010=ADVANCED_FACE('',(#2275),#1576,.F.);
#15011=ADVANCED_FACE('',(#2276),#1577,.F.);
#15012=ADVANCED_FACE('',(#2277),#14332,.F.);
#15013=ADVANCED_FACE('',(#2278),#1578,.F.);
#15014=ADVANCED_FACE('',(#2279),#1579,.F.);
#15015=ADVANCED_FACE('',(#2280),#1580,.F.);
#15016=ADVANCED_FACE('',(#2281,#1208),#1581,.T.);
#15017=ADVANCED_FACE('',(#2282),#14333,.T.);
#15018=ADVANCED_FACE('',(#2283),#14334,.T.);
#15019=ADVANCED_FACE('',(#2284),#1582,.T.);
#15091=CLOSED_SHELL('',(#14961,#14962,#14963,#14964,#14965,#14966,#14967,
#14968,#14969,#14970,#14971,#14972,#14973,#14974,#14975,#14976,#14977,#14978,
#14979,#14980,#14981,#14982,#14983,#14984,#14985,#14986,#14987,#14988,#14989,
#14990,#14991,#14992,#14993,#14994,#14995,#14996,#14997,#14998,#14999,#15000,
#15001,#15002,#15003,#15004,#15005,#15006,#15007,#15008,#15009,#15010,#15011,
#15012,#15013,#15014,#15015,#15016,#15017,#15018,#15019));
#16363=AXIS2_PLACEMENT_3D('',#43206,#19944,#19945);
#16364=AXIS2_PLACEMENT_3D('',#43207,#19946,#19947);
#16365=AXIS2_PLACEMENT_3D('',#43387,#19949,#19950);
#16366=AXIS2_PLACEMENT_3D('',#43506,#19951,#19952);
#16367=AXIS2_PLACEMENT_3D('',#43950,#19954,#19955);
#16368=AXIS2_PLACEMENT_3D('',#44382,#19957,#19958);
#16369=AXIS2_PLACEMENT_3D('',#44802,#19960,#19961);
#16370=AXIS2_PLACEMENT_3D('',#45304,#19963,#19964);
#16371=AXIS2_PLACEMENT_3D('',#45734,#19966,#19967);
#16372=AXIS2_PLACEMENT_3D('',#46188,#19969,#19970);
#16373=AXIS2_PLACEMENT_3D('',#46632,#19972,#19973);
#16374=AXIS2_PLACEMENT_3D('',#47114,#19975,#19976);
#16375=AXIS2_PLACEMENT_3D('',#47580,#19978,#19979);
#16376=AXIS2_PLACEMENT_3D('',#48004,#19981,#19982);
#16377=AXIS2_PLACEMENT_3D('',#48468,#19984,#19985);
#16378=AXIS2_PLACEMENT_3D('',#48907,#19987,#19988);
#16379=AXIS2_PLACEMENT_3D('',#49346,#19990,#19991);
#16380=AXIS2_PLACEMENT_3D('',#49795,#19993,#19994);
#16381=AXIS2_PLACEMENT_3D('',#50298,#19996,#19997);
#16382=AXIS2_PLACEMENT_3D('',#50801,#19999,#20000);
#16383=AXIS2_PLACEMENT_3D('',#51280,#20002,#20003);
#16384=AXIS2_PLACEMENT_3D('',#51713,#20005,#20006);
#16385=AXIS2_PLACEMENT_3D('',#52158,#20008,#20009);
#16386=AXIS2_PLACEMENT_3D('',#52607,#20011,#20012);
#16387=AXIS2_PLACEMENT_3D('',#53050,#20014,#20015);
#16388=AXIS2_PLACEMENT_3D('',#53516,#20017,#20018);
#16389=AXIS2_PLACEMENT_3D('',#53526,#20019,#20020);
#16390=AXIS2_PLACEMENT_3D('',#57867,#20021,#20022);
#16391=AXIS2_PLACEMENT_3D('',#61218,#20023,#20024);
#16392=AXIS2_PLACEMENT_3D('',#61429,#20025,#20026);
#16393=AXIS2_PLACEMENT_3D('',#61577,#20027,#20028);
#16394=AXIS2_PLACEMENT_3D('',#61580,#20029,#20030);
#16395=AXIS2_PLACEMENT_3D('',#61759,#20031,#20032);
#16396=AXIS2_PLACEMENT_3D('',#62470,#20033,#20034);
#16397=AXIS2_PLACEMENT_3D('',#62472,#20035,#20036);
#16398=AXIS2_PLACEMENT_3D('',#62474,#20037,#20038);
#16399=AXIS2_PLACEMENT_3D('',#63183,#20039,#20040);
#16400=AXIS2_PLACEMENT_3D('',#63190,#20041,#20042);
#16401=AXIS2_PLACEMENT_3D('',#63200,#20043,#20044);
#16402=AXIS2_PLACEMENT_3D('',#63210,#20045,#20046);
#16403=AXIS2_PLACEMENT_3D('',#63220,#20047,#20048);
#16404=AXIS2_PLACEMENT_3D('',#63230,#20049,#20050);
#16405=AXIS2_PLACEMENT_3D('',#63240,#20051,#20052);
#16406=AXIS2_PLACEMENT_3D('',#63246,#20054,#20055);
#16407=AXIS2_PLACEMENT_3D('',#63247,#20056,#20057);
#16408=AXIS2_PLACEMENT_3D('',#63252,#20060,#20061);
#16409=AXIS2_PLACEMENT_3D('',#63253,#20062,#20063);
#16410=AXIS2_PLACEMENT_3D('',#63258,#20066,#20067);
#16411=AXIS2_PLACEMENT_3D('',#63259,#20068,#20069);
#16412=AXIS2_PLACEMENT_3D('',#63263,#20071,#20072);
#16413=AXIS2_PLACEMENT_3D('',#63265,#20074,#20075);
#16414=AXIS2_PLACEMENT_3D('',#63270,#20078,#20079);
#16415=AXIS2_PLACEMENT_3D('',#63271,#20080,#20081);
#16416=AXIS2_PLACEMENT_3D('',#63275,#20083,#20084);
#16417=AXIS2_PLACEMENT_3D('',#63277,#20086,#20087);
#16418=AXIS2_PLACEMENT_3D('',#63281,#20089,#20090);
#16419=AXIS2_PLACEMENT_3D('',#63283,#20092,#20093);
#16420=AXIS2_PLACEMENT_3D('',#63290,#20098,#20099);
#16421=AXIS2_PLACEMENT_3D('',#63295,#20103,#20104);
#16422=AXIS2_PLACEMENT_3D('',#63300,#20108,#20109);
#16423=AXIS2_PLACEMENT_3D('',#63301,#20110,#20111);
#16424=AXIS2_PLACEMENT_3D('',#63302,#20112,#20113);
#16425=AXIS2_PLACEMENT_3D('',#63304,#20115,#20116);
#16426=AXIS2_PLACEMENT_3D('',#63305,#20117,#20118);
#16427=AXIS2_PLACEMENT_3D('',#63307,#20120,#20121);
#16428=AXIS2_PLACEMENT_3D('',#63309,#20123,#20124);
#16429=AXIS2_PLACEMENT_3D('',#63312,#20126,#20127);
#16430=AXIS2_PLACEMENT_3D('',#63313,#20128,#20129);
#16431=AXIS2_PLACEMENT_3D('',#63314,#20130,#20131);
#16432=AXIS2_PLACEMENT_3D('',#63315,#20132,#20133);
#16433=AXIS2_PLACEMENT_3D('',#63316,#20134,#20135);
#16434=AXIS2_PLACEMENT_3D('',#63317,#20136,#20137);
#16435=AXIS2_PLACEMENT_3D('',#63318,#20138,#20139);
#16436=AXIS2_PLACEMENT_3D('',#63319,#20140,#20141);
#16437=AXIS2_PLACEMENT_3D('',#63322,#20143,#20144);
#16438=AXIS2_PLACEMENT_3D('',#63323,#20145,#20146);
#16439=AXIS2_PLACEMENT_3D('',#63325,#20148,#20149);
#16440=AXIS2_PLACEMENT_3D('',#63326,#20150,#20151);
#16441=AXIS2_PLACEMENT_3D('',#63329,#20153,#20154);
#16442=AXIS2_PLACEMENT_3D('',#63331,#20156,#20157);
#16443=AXIS2_PLACEMENT_3D('',#63333,#20159,#20160);
#16444=AXIS2_PLACEMENT_3D('',#63334,#20161,#20162);
#16445=AXIS2_PLACEMENT_3D('',#63336,#20163,#20164);
#16446=AXIS2_PLACEMENT_3D('',#63337,#20165,#20166);
#16447=AXIS2_PLACEMENT_3D('',#63339,#20168,#20169);
#16448=AXIS2_PLACEMENT_3D('',#63342,#20171,#20172);
#16449=AXIS2_PLACEMENT_3D('',#63343,#20173,#20174);
#19944=DIRECTION('axis',(0.,0.,1.));
#19945=DIRECTION('refdir',(1.,0.,0.));
#19946=DIRECTION('center_axis',(0.,0.,1.));
#19947=DIRECTION('ref_axis',(0.979226971796874,-0.202767200763645,0.));
#19948=DIRECTION('',(0.,0.,-1.));
#19949=DIRECTION('center_axis',(0.,0.,-1.));
#19950=DIRECTION('ref_axis',(1.,6.67887018197865E-15,0.));
#19951=DIRECTION('center_axis',(0.,0.,1.));
#19952=DIRECTION('ref_axis',(0.979226971796874,-0.202767200763645,0.));
#19953=DIRECTION('',(0.,0.,-1.));
#19954=DIRECTION('center_axis',(0.,0.,1.));
#19955=DIRECTION('ref_axis',(0.979226971796874,-0.202767200763645,0.));
#19956=DIRECTION('',(0.,0.,-1.));
#19957=DIRECTION('center_axis',(0.,0.,1.));
#19958=DIRECTION('ref_axis',(0.979226971796874,-0.202767200763645,0.));
#19959=DIRECTION('',(0.,0.,-1.));
#19960=DIRECTION('center_axis',(0.,0.,1.));
#19961=DIRECTION('ref_axis',(0.979226971796874,-0.202767200763645,0.));
#19962=DIRECTION('',(0.,0.,-1.));
#19963=DIRECTION('center_axis',(0.,0.,1.));
#19964=DIRECTION('ref_axis',(0.979226971796874,-0.202767200763645,0.));
#19965=DIRECTION('',(0.,0.,-1.));
#19966=DIRECTION('center_axis',(0.,0.,1.));
#19967=DIRECTION('ref_axis',(0.979226971796874,-0.202767200763645,0.));
#19968=DIRECTION('',(0.,0.,-1.));
#19969=DIRECTION('center_axis',(0.,0.,1.));
#19970=DIRECTION('ref_axis',(0.979226971796874,-0.202767200763645,0.));
#19971=DIRECTION('',(0.,0.,-1.));
#19972=DIRECTION('center_axis',(0.,0.,1.));
#19973=DIRECTION('ref_axis',(0.979226971796874,-0.202767200763645,0.));
#19974=DIRECTION('',(0.,0.,-1.));
#19975=DIRECTION('center_axis',(0.,0.,1.));
#19976=DIRECTION('ref_axis',(0.979226971796874,-0.202767200763645,0.));
#19977=DIRECTION('',(0.,0.,-1.));
#19978=DIRECTION('center_axis',(0.,0.,1.));
#19979=DIRECTION('ref_axis',(0.979226971796874,-0.202767200763645,0.));
#19980=DIRECTION('',(0.,0.,-1.));
#19981=DIRECTION('center_axis',(0.,0.,1.));
#19982=DIRECTION('ref_axis',(0.979226971796874,-0.202767200763645,0.));
#19983=DIRECTION('',(0.,0.,-1.));
#19984=DIRECTION('center_axis',(0.,0.,1.));
#19985=DIRECTION('ref_axis',(0.979226971796874,-0.202767200763645,0.));
#19986=DIRECTION('',(0.,0.,-1.));
#19987=DIRECTION('center_axis',(0.,0.,1.));
#19988=DIRECTION('ref_axis',(0.979226971796874,-0.202767200763645,0.));
#19989=DIRECTION('',(0.,0.,-1.));
#19990=DIRECTION('center_axis',(0.,0.,1.));
#19991=DIRECTION('ref_axis',(0.979226971796874,-0.202767200763645,0.));
#19992=DIRECTION('',(0.,0.,-1.));
#19993=DIRECTION('center_axis',(0.,0.,1.));
#19994=DIRECTION('ref_axis',(0.979226971796874,-0.202767200763645,0.));
#19995=DIRECTION('',(0.,0.,-1.));
#19996=DIRECTION('center_axis',(0.,0.,1.));
#19997=DIRECTION('ref_axis',(0.979226971796874,-0.202767200763645,0.));
#19998=DIRECTION('',(0.,0.,-1.));
#19999=DIRECTION('center_axis',(0.,0.,1.));
#20000=DIRECTION('ref_axis',(0.979226971796874,-0.202767200763645,0.));
#20001=DIRECTION('',(0.,0.,-1.));
#20002=DIRECTION('center_axis',(0.,0.,1.));
#20003=DIRECTION('ref_axis',(0.979226971796874,-0.202767200763645,0.));
#20004=DIRECTION('',(0.,0.,-1.));
#20005=DIRECTION('center_axis',(0.,0.,1.));
#20006=DIRECTION('ref_axis',(0.979226971796874,-0.202767200763645,0.));
#20007=DIRECTION('',(0.,0.,-1.));
#20008=DIRECTION('center_axis',(0.,0.,1.));
#20009=DIRECTION('ref_axis',(0.979226971796874,-0.202767200763645,0.));
#20010=DIRECTION('',(0.,0.,-1.));
#20011=DIRECTION('center_axis',(0.,0.,1.));
#20012=DIRECTION('ref_axis',(0.979226971796874,-0.202767200763645,0.));
#20013=DIRECTION('',(0.,0.,-1.));
#20014=DIRECTION('center_axis',(0.,0.,1.));
#20015=DIRECTION('ref_axis',(0.979226971796874,-0.202767200763645,0.));
#20016=DIRECTION('',(0.,0.,-1.));
#20017=DIRECTION('center_axis',(0.,0.,1.));
#20018=DIRECTION('ref_axis',(1.,0.,0.));
#20019=DIRECTION('center_axis',(0.,0.,1.));
#20020=DIRECTION('ref_axis',(1.,0.,0.));
#20021=DIRECTION('center_axis',(0.,0.,-1.));
#20022=DIRECTION('ref_axis',(1.,0.,0.));
#20023=DIRECTION('center_axis',(0.,0.,1.));
#20024=DIRECTION('ref_axis',(0.979226971796874,-0.202767200763645,0.));
#20025=DIRECTION('center_axis',(0.,0.,1.));
#20026=DIRECTION('ref_axis',(1.,6.67887018197865E-15,0.));
#20027=DIRECTION('center_axis',(0.,0.,1.));
#20028=DIRECTION('ref_axis',(1.,0.,0.));
#20029=DIRECTION('center_axis',(0.,0.,-1.));
#20030=DIRECTION('ref_axis',(1.,0.,0.));
#20031=DIRECTION('center_axis',(0.,0.,-1.));
#20032=DIRECTION('ref_axis',(1.,0.,0.));
#20033=DIRECTION('center_axis',(0.,0.,1.));
#20034=DIRECTION('ref_axis',(1.,0.,0.));
#20035=DIRECTION('center_axis',(0.,0.,1.));
#20036=DIRECTION('ref_axis',(1.,0.,0.));
#20037=DIRECTION('center_axis',(0.,0.,1.));
#20038=DIRECTION('ref_axis',(1.,0.,0.));
#20039=DIRECTION('center_axis',(0.,0.,-1.));
#20040=DIRECTION('ref_axis',(1.,0.,0.));
#20041=DIRECTION('center_axis',(0.,0.,1.));
#20042=DIRECTION('ref_axis',(1.,0.,0.));
#20043=DIRECTION('center_axis',(0.,0.,1.));
#20044=DIRECTION('ref_axis',(1.,0.,0.));
#20045=DIRECTION('center_axis',(0.,0.,1.));
#20046=DIRECTION('ref_axis',(1.,0.,0.));
#20047=DIRECTION('center_axis',(0.,0.,1.));
#20048=DIRECTION('ref_axis',(1.,0.,0.));
#20049=DIRECTION('center_axis',(0.,0.,1.));
#20050=DIRECTION('ref_axis',(1.,0.,0.));
#20051=DIRECTION('center_axis',(0.,0.,1.));
#20052=DIRECTION('ref_axis',(1.,0.,0.));
#20053=DIRECTION('',(-0.707106781186539,8.65956056235484E-17,-0.707106781186556));
#20054=DIRECTION('center_axis',(0.,0.,1.));
#20055=DIRECTION('ref_axis',(1.,0.,0.));
#20056=DIRECTION('center_axis',(0.,0.,1.));
#20057=DIRECTION('ref_axis',(1.,0.,0.));
#20058=DIRECTION('',(0.,0.,-1.));
#20059=DIRECTION('',(0.,0.,1.));
#20060=DIRECTION('center_axis',(0.,0.,-1.));
#20061=DIRECTION('ref_axis',(1.,0.,0.));
#20062=DIRECTION('center_axis',(0.,0.,1.));
#20063=DIRECTION('ref_axis',(1.,0.,0.));
#20064=DIRECTION('',(0.,0.,-1.));
#20065=DIRECTION('',(0.,0.,1.));
#20066=DIRECTION('center_axis',(0.,0.,-1.));
#20067=DIRECTION('ref_axis',(1.,0.,0.));
#20068=DIRECTION('center_axis',(0.,0.,1.));
#20069=DIRECTION('ref_axis',(1.,0.,0.));
#20070=DIRECTION('',(0.,0.,1.));
#20071=DIRECTION('center_axis',(0.,0.,-1.));
#20072=DIRECTION('ref_axis',(1.,0.,0.));
#20073=DIRECTION('',(0.,0.,-1.));
#20074=DIRECTION('center_axis',(0.,0.,1.));
#20075=DIRECTION('ref_axis',(1.,0.,0.));
#20076=DIRECTION('',(0.,0.,-1.));
#20077=DIRECTION('',(0.,0.,1.));
#20078=DIRECTION('center_axis',(0.,0.,-1.));
#20079=DIRECTION('ref_axis',(1.,0.,0.));
#20080=DIRECTION('center_axis',(0.,0.,1.));
#20081=DIRECTION('ref_axis',(1.,0.,0.));
#20082=DIRECTION('',(0.,0.,1.));
#20083=DIRECTION('center_axis',(0.,0.,-1.));
#20084=DIRECTION('ref_axis',(1.,0.,0.));
#20085=DIRECTION('',(0.,0.,-1.));
#20086=DIRECTION('center_axis',(0.,0.,1.));
#20087=DIRECTION('ref_axis',(1.,0.,0.));
#20088=DIRECTION('',(0.,0.,1.));
#20089=DIRECTION('center_axis',(0.,0.,-1.));
#20090=DIRECTION('ref_axis',(1.,0.,0.));
#20091=DIRECTION('',(0.,0.,-1.));
#20092=DIRECTION('center_axis',(0.,1.,0.));
#20093=DIRECTION('ref_axis',(-1.,0.,0.));
#20094=DIRECTION('',(-1.,0.,0.));
#20095=DIRECTION('',(0.,0.,1.));
#20096=DIRECTION('',(-1.,0.,0.));
#20097=DIRECTION('',(0.,0.,1.));
#20098=DIRECTION('center_axis',(0.86602540378444,0.499999999999998,0.));
#20099=DIRECTION('ref_axis',(-0.499999999999998,0.86602540378444,0.));
#20100=DIRECTION('',(-0.499999999999998,0.86602540378444,0.));
#20101=DIRECTION('',(0.,0.,1.));
#20102=DIRECTION('',(-0.499999999999998,0.86602540378444,0.));
#20103=DIRECTION('center_axis',(0.86602540378444,-0.499999999999998,0.));
#20104=DIRECTION('ref_axis',(0.499999999999998,0.86602540378444,0.));
#20105=DIRECTION('',(0.499999999999998,0.86602540378444,0.));
#20106=DIRECTION('',(0.,0.,1.));
#20107=DIRECTION('',(0.499999999999998,0.86602540378444,0.));
#20108=DIRECTION('center_axis',(0.,0.,-1.));
#20109=DIRECTION('ref_axis',(-1.,0.,0.));
#20110=DIRECTION('center_axis',(0.,0.,-1.));
#20111=DIRECTION('ref_axis',(-1.,0.,0.));
#20112=DIRECTION('center_axis',(0.,0.,-1.));
#20113=DIRECTION('ref_axis',(-1.,0.,0.));
#20114=DIRECTION('',(1.,0.,0.));
#20115=DIRECTION('center_axis',(0.,0.,-1.));
#20116=DIRECTION('ref_axis',(-1.,0.,0.));
#20117=DIRECTION('center_axis',(0.,0.,-1.));
#20118=DIRECTION('ref_axis',(-1.,0.,0.));
#20119=DIRECTION('',(0.499999999999998,-0.86602540378444,0.));
#20120=DIRECTION('center_axis',(0.,0.,-1.));
#20121=DIRECTION('ref_axis',(-1.,0.,0.));
#20122=DIRECTION('',(-0.499999999999998,-0.86602540378444,0.));
#20123=DIRECTION('center_axis',(0.,0.,-1.));
#20124=DIRECTION('ref_axis',(-1.,0.,0.));
#20125=DIRECTION('',(1.,0.,0.));
#20126=DIRECTION('center_axis',(0.,0.,1.));
#20127=DIRECTION('ref_axis',(1.,0.,0.));
#20128=DIRECTION('center_axis',(0.,0.,-1.));
#20129=DIRECTION('ref_axis',(-1.,0.,0.));
#20130=DIRECTION('center_axis',(0.,0.,1.));
#20131=DIRECTION('ref_axis',(1.,0.,0.));
#20132=DIRECTION('center_axis',(0.,0.,-1.));
#20133=DIRECTION('ref_axis',(-1.,0.,0.));
#20134=DIRECTION('center_axis',(0.,0.,1.));
#20135=DIRECTION('ref_axis',(1.,0.,0.));
#20136=DIRECTION('center_axis',(0.,0.,-1.));
#20137=DIRECTION('ref_axis',(-1.,0.,0.));
#20138=DIRECTION('center_axis',(0.,0.,1.));
#20139=DIRECTION('ref_axis',(1.,0.,0.));
#20140=DIRECTION('center_axis',(0.,0.,-1.));
#20141=DIRECTION('ref_axis',(-1.,0.,0.));
#20142=DIRECTION('',(-0.499999999999998,-0.86602540378444,0.));
#20143=DIRECTION('center_axis',(0.,0.,1.));
#20144=DIRECTION('ref_axis',(1.,0.,0.));
#20145=DIRECTION('center_axis',(0.,0.,-1.));
#20146=DIRECTION('ref_axis',(-1.,0.,0.));
#20147=DIRECTION('',(0.499999999999998,-0.86602540378444,0.));
#20148=DIRECTION('center_axis',(0.,0.,1.));
#20149=DIRECTION('ref_axis',(1.,0.,0.));
#20150=DIRECTION('center_axis',(0.,0.,-1.));
#20151=DIRECTION('ref_axis',(1.,0.,0.));
#20152=DIRECTION('',(-0.85716730070211,1.04972719113862E-16,-0.515038074910058));
#20153=DIRECTION('center_axis',(0.,-1.,0.));
#20154=DIRECTION('ref_axis',(1.,0.,0.));
#20155=DIRECTION('',(0.,0.,1.));
#20156=DIRECTION('center_axis',(-0.86602540378444,-0.499999999999998,0.));
#20157=DIRECTION('ref_axis',(0.499999999999998,-0.86602540378444,0.));
#20158=DIRECTION('',(0.,0.,1.));
#20159=DIRECTION('center_axis',(-0.86602540378444,0.499999999999998,0.));
#20160=DIRECTION('ref_axis',(-0.499999999999998,-0.86602540378444,0.));
#20161=DIRECTION('center_axis',(0.,0.,-1.));
#20162=DIRECTION('ref_axis',(-1.,0.,0.));
#20163=DIRECTION('center_axis',(0.,0.,1.));
#20164=DIRECTION('ref_axis',(1.,0.,0.));
#20165=DIRECTION('center_axis',(0.,0.,1.));
#20166=DIRECTION('ref_axis',(1.,0.,0.));
#20167=DIRECTION('',(0.707106781186547,8.65956056235493E-17,-0.707106781186548));
#20168=DIRECTION('center_axis',(0.,0.,-1.));
#20169=DIRECTION('ref_axis',(1.,0.,0.));
#20170=DIRECTION('',(0.707106781186547,-8.65956056235493E-17,0.707106781186548));
#20171=DIRECTION('center_axis',(0.,0.,1.));
#20172=DIRECTION('ref_axis',(1.,0.,0.));
#20173=DIRECTION('center_axis',(0.,0.,1.));
#20174=DIRECTION('ref_axis',(1.,0.,0.));
#43206=CARTESIAN_POINT('',(0.,0.,0.));
#43207=CARTESIAN_POINT('Origin',(55.,29.,3.45145488139523));
#43208=CARTESIAN_POINT('',(53.0466869980211,29.4044698737854,5.5836423751603));
#43209=CARTESIAN_POINT('',(53.0466869980082,29.4044698737233,5.42540812064255));
#43210=CARTESIAN_POINT('',(53.0466869980082,29.4044698737233,3.45145488139523));
#43211=CARTESIAN_POINT('',(53.8611373905627,27.3623127528964,4.93049999999996));
#43212=CARTESIAN_POINT('Ctrl Pts',(53.0466869980211,29.4044698737854,5.5836423751603));
#43213=CARTESIAN_POINT('Ctrl Pts',(53.0467598410346,29.4048216557467,5.58361735794786));
#43214=CARTESIAN_POINT('Ctrl Pts',(53.0468327795955,29.4051734205221,5.58359234005539));
#43215=CARTESIAN_POINT('Ctrl Pts',(53.052944084167,29.4346067439485,5.58149885155498));
#43216=CARTESIAN_POINT('Ctrl Pts',(53.0596311359168,29.463549813269,5.57942719964456));
#43217=CARTESIAN_POINT('Ctrl Pts',(53.079658569571,29.5421832070144,5.57377511658151));
#43218=CARTESIAN_POINT('Ctrl Pts',(53.0942792715992,29.591525759737,5.57020181656668));
#43219=CARTESIAN_POINT('Ctrl Pts',(53.1281561119192,29.6914874381887,5.56296689427717));
#43220=CARTESIAN_POINT('Ctrl Pts',(53.1475996330664,29.7420029867334,5.5593130896378));
#43221=CARTESIAN_POINT('Ctrl Pts',(53.1726367106895,29.7999071888819,5.55517541185005));
#43222=CARTESIAN_POINT('Ctrl Pts',(53.1762540609445,29.808120571997,5.55458973206913));
#43223=CARTESIAN_POINT('Ctrl Pts',(53.182194225425,29.8213649786112,5.55364761522522));
#43224=CARTESIAN_POINT('Ctrl Pts',(53.1844827387612,29.8264111192952,5.55328921441833));
#43225=CARTESIAN_POINT('Ctrl Pts',(53.1885888050893,29.8353655621017,5.55265428753538));
#43226=CARTESIAN_POINT('Ctrl Pts',(53.1903980261385,29.8392775683841,5.55237726763184));
#43227=CARTESIAN_POINT('Ctrl Pts',(53.1943395988275,29.8477282720442,5.55177965573117));
#43228=CARTESIAN_POINT('Ctrl Pts',(53.1964763867749,29.8522647977318,5.55145933871332));
#43229=CARTESIAN_POINT('Ctrl Pts',(53.2025062824284,29.8649423848354,5.55056544773773));
#43230=CARTESIAN_POINT('Ctrl Pts',(53.2064376176204,29.8730652791062,5.54999415888182));
#43231=CARTESIAN_POINT('Ctrl Pts',(53.2304006381325,29.921732465328,5.54657846256867));
#43232=CARTESIAN_POINT('Ctrl Pts',(53.251752897287,29.9616160414764,5.54380892718374));
#43233=CARTESIAN_POINT('Ctrl Pts',(53.329544218408,30.0957497024807,5.53448041500691));
#43234=CARTESIAN_POINT('Ctrl Pts',(53.3924003014302,30.186050862637,5.52816720503428));
#43235=CARTESIAN_POINT('Ctrl Pts',(53.5448870745863,30.3705658375547,5.51424720056297));
#43236=CARTESIAN_POINT('Ctrl Pts',(53.6369149972079,30.4621207901423,5.50663231156854));
#43237=CARTESIAN_POINT('Ctrl Pts',(53.7493859359876,30.5541047281784,5.49761556419157));
#43238=CARTESIAN_POINT('Ctrl Pts',(53.7617306247401,30.5639584314487,5.49662983864366));
#43239=CARTESIAN_POINT('Ctrl Pts',(53.7819752865071,30.5797280550832,5.49501890204659));
#43240=CARTESIAN_POINT('Ctrl Pts',(53.7898045849945,30.5857338940074,5.49439723334141));
#43241=CARTESIAN_POINT('Ctrl Pts',(53.8038390539862,30.596335231447,5.49328505327765));
#43242=CARTESIAN_POINT('Ctrl Pts',(53.8100269952484,30.60095328638,5.49279543238884));
#43243=CARTESIAN_POINT('Ctrl Pts',(53.8231477326398,30.6106271843221,5.4917587472129));
#43244=CARTESIAN_POINT('Ctrl Pts',(53.8300866354468,30.6156744417553,5.49121136580214));
#43245=CARTESIAN_POINT('Ctrl Pts',(53.8486189765485,30.6289726161707,5.48975159847759));
#43246=CARTESIAN_POINT('Ctrl Pts',(53.8602683376335,30.6371443937267,5.48883622855343));
#43247=CARTESIAN_POINT('Ctrl Pts',(53.917026817361,30.6760598494534,5.48438620008985));
#43248=CARTESIAN_POINT('Ctrl Pts',(53.9632939445138,30.7050651429083,5.4807876177965));
#43249=CARTESIAN_POINT('Ctrl Pts',(54.1864074481192,30.8324967499752,5.46355530959757));
#43250=CARTESIAN_POINT('Ctrl Pts',(54.3763344630289,30.9055173440879,5.4490750849697));
#43251=CARTESIAN_POINT('Ctrl Pts',(54.6071992840641,30.9559887464049,5.43311035353166));
#43252=CARTESIAN_POINT('Ctrl Pts',(54.6406092752949,30.9624023569689,5.43084241964906));
#43253=CARTESIAN_POINT('Ctrl Pts',(54.6826361309647,30.9693606555478,5.42805556969599));
#43254=CARTESIAN_POINT('Ctrl Pts',(54.6911122263776,30.9707078846567,5.42749685439508));
#43255=CARTESIAN_POINT('Ctrl Pts',(54.7045122685035,30.9727491691074,5.42661912461067));
#43256=CARTESIAN_POINT('Ctrl Pts',(54.7094304506579,30.9734795722214,5.42629815312209));
#43257=CARTESIAN_POINT('Ctrl Pts',(54.7182092058252,30.974749782946,5.42572739671727));
#43258=CARTESIAN_POINT('Ctrl Pts',(54.7220686017681,30.9752966600293,5.42547722671951));
#43259=CARTESIAN_POINT('Ctrl Pts',(54.7312869635949,30.9765753512837,5.42488144691789));
#43260=CARTESIAN_POINT('Ctrl Pts',(54.7366473251915,30.9772966862746,5.42453642454854));
#43261=CARTESIAN_POINT('Ctrl Pts',(54.7527691377047,30.9793994487664,5.42350281170371));
#43262=CARTESIAN_POINT('Ctrl Pts',(54.7635391977724,30.9807149159857,5.42281776693858));
#43263=CARTESIAN_POINT('Ctrl Pts',(54.7884146505401,30.9835474395462,5.42124699119317));
#43264=CARTESIAN_POINT('Ctrl Pts',(54.8025267166315,30.9850020483384,5.42036435897924));
#43265=CARTESIAN_POINT('Ctrl Pts',(54.8505508508856,30.9894349280911,5.41738588508356));
#43266=CARTESIAN_POINT('Ctrl Pts',(54.8845246747252,30.991695783145,5.41532137063713));
#43267=CARTESIAN_POINT('Ctrl Pts',(55.0714430634789,30.9993352333717,5.40411637916261));
#43268=CARTESIAN_POINT('Ctrl Pts',(55.2245620306993,30.9879696561106,5.39546385208552));
#43269=CARTESIAN_POINT('Ctrl Pts',(55.4541103597074,30.9440468197256,5.38164807919455));
#43270=CARTESIAN_POINT('Ctrl Pts',(55.5323361852893,30.9240972383442,5.37679113269101));
#43271=CARTESIAN_POINT('Ctrl Pts',(55.6233625220245,30.8949063304474,5.37085166486203));
#43272=CARTESIAN_POINT('Ctrl Pts',(55.6375390683028,30.8901837880418,5.36991830345721));
#43273=CARTESIAN_POINT('Ctrl Pts',(55.6607512822745,30.8821604110354,5.36837565747547));
#43274=CARTESIAN_POINT('Ctrl Pts',(55.6698186621453,30.8789526403198,5.36776941374951));
#43275=CARTESIAN_POINT('Ctrl Pts',(55.6861101445537,30.8730562841087,5.36667343529993));
#43276=CARTESIAN_POINT('Ctrl Pts',(55.6933425761252,30.8703911471479,5.36618448088078));
#43277=CARTESIAN_POINT('Ctrl Pts',(55.7087608854888,30.8646078139443,5.36513687648532));
#43278=CARTESIAN_POINT('Ctrl Pts',(55.7169420106464,30.8614774889824,5.36457783302405));
#43279=CARTESIAN_POINT('Ctrl Pts',(55.739078260069,30.8528399714588,5.36305642212925));
#43280=CARTESIAN_POINT('Ctrl Pts',(55.7529920806579,30.8472291521559,5.36209062484586));
#43281=CARTESIAN_POINT('Ctrl Pts',(55.8266105715767,30.8165721662778,5.35692870868625));
#43282=CARTESIAN_POINT('Ctrl Pts',(55.8851266732236,30.7887897270671,5.35264132666126));
#43283=CARTESIAN_POINT('Ctrl Pts',(56.073780504631,30.6876947972367,5.33819064714519));
#43284=CARTESIAN_POINT('Ctrl Pts',(56.1970357929047,30.6026273879261,5.3276712881522));
#43285=CARTESIAN_POINT('Ctrl Pts',(56.3642577387813,30.4570770415889,5.31234294664548));
#43286=CARTESIAN_POINT('Ctrl Pts',(56.4162624191764,30.4065830171306,5.30740241716296));
#43287=CARTESIAN_POINT('Ctrl Pts',(56.4725126533723,30.3456759060381,5.30195848867342));
#43288=CARTESIAN_POINT('Ctrl Pts',(56.4795548969886,30.3379291747173,5.30127503966523));
#43289=CARTESIAN_POINT('Ctrl Pts',(56.4901298431912,30.3261107270354,5.30024632671909));
#43290=CARTESIAN_POINT('Ctrl Pts',(56.49370743987,30.3220796858166,5.29989787794448));
#43291=CARTESIAN_POINT('Ctrl Pts',(56.5001030722091,30.3148143351866,5.29927426986947));
#43292=CARTESIAN_POINT('Ctrl Pts',(56.50292706706,30.3115853749136,5.29899867453789));
#43293=CARTESIAN_POINT('Ctrl Pts',(56.509081239888,30.3045027073592,5.29839757829528));
#43294=CARTESIAN_POINT('Ctrl Pts',(56.5124070841153,30.300645345744,5.29807239454115));
#43295=CARTESIAN_POINT('Ctrl Pts',(56.5218920686168,30.2895589501389,5.2971438845272));
#43296=CARTESIAN_POINT('Ctrl Pts',(56.5280145066089,30.2822984950842,5.29654318056524));
#43297=CARTESIAN_POINT('Ctrl Pts',(56.5701565504473,30.2315928007642,5.29239662327045));
#43298=CARTESIAN_POINT('Ctrl Pts',(56.6043737659093,30.1866754107808,5.28896915328454));
#43299=CARTESIAN_POINT('Ctrl Pts',(56.6916579319223,30.061405626217,5.2798726688626));
#43300=CARTESIAN_POINT('Ctrl Pts',(56.7408899672203,29.9785665924262,5.27433457303476));
#43301=CARTESIAN_POINT('Ctrl Pts',(56.8430593123045,29.7743464179482,5.26107390515525));
#43302=CARTESIAN_POINT('Ctrl Pts',(56.8902762318413,29.6506374369867,5.25332224917714));
#43303=CARTESIAN_POINT('Ctrl Pts',(56.9290370954948,29.5080256231801,5.24415279051811));
#43304=CARTESIAN_POINT('Ctrl Pts',(56.9329764961587,29.4928245051462,5.24317297793125));
#43305=CARTESIAN_POINT('Ctrl Pts',(56.939083418211,29.4680589679658,5.24157201103533));
#43306=CARTESIAN_POINT('Ctrl Pts',(56.9413606503824,29.4585221040407,5.24095438625694));
#43307=CARTESIAN_POINT('Ctrl Pts',(56.945293374306,29.4414975107157,5.23984969389446));
#43308=CARTESIAN_POINT('Ctrl Pts',(56.9469761840545,29.434016244084,5.23936351328078));
#43309=CARTESIAN_POINT('Ctrl Pts',(56.9504368739863,29.4182058075239,5.23833441584678));
#43310=CARTESIAN_POINT('Ctrl Pts',(56.9522046266746,29.409874601229,5.23779118574829));
#43311=CARTESIAN_POINT('Ctrl Pts',(56.9567594439886,29.387710155499,5.23634331369595));
#43312=CARTESIAN_POINT('Ctrl Pts',(56.9594531239508,29.3738584282556,5.2354357188024));
#43313=CARTESIAN_POINT('Ctrl Pts',(56.9717284256869,29.3069542533562,5.23103799203724));
#43314=CARTESIAN_POINT('Ctrl Pts',(56.9793028575019,29.253560994094,5.22748509753295));
#43315=CARTESIAN_POINT('Ctrl Pts',(56.9951861160448,29.0958882609151,5.21686009187886));
#43316=CARTESIAN_POINT('Ctrl Pts',(56.997468429701,28.9911941364029,5.20962594995398));
#43317=CARTESIAN_POINT('Ctrl Pts',(56.9895148154999,28.8512465375254,5.19985609716229));
#43318=CARTESIAN_POINT('Ctrl Pts',(56.9865408023446,28.8157380861126,5.19736989327771));
#43319=CARTESIAN_POINT('Ctrl Pts',(56.9806418946041,28.7624983000686,5.19364326420605));
#43320=CARTESIAN_POINT('Ctrl Pts',(56.9784259039746,28.7446956152318,5.19239733976931));
#43321=CARTESIAN_POINT('Ctrl Pts',(56.9656162085244,28.6520046695348,5.1859177104549));
#43322=CARTESIAN_POINT('Ctrl Pts',(56.9510084677251,28.5777247394624,5.18074811658668));
#43323=CARTESIAN_POINT('Ctrl Pts',(56.9296209819756,28.4943326688822,5.17509414251862));
#43324=CARTESIAN_POINT('Ctrl Pts',(56.9269476164077,28.4842389324896,5.17441236899198));
#43325=CARTESIAN_POINT('Ctrl Pts',(56.922780346937,28.4689895471189,5.17338675935825));
#43326=CARTESIAN_POINT('Ctrl Pts',(56.9213447398797,28.4638183555879,5.17303973582239));
#43327=CARTESIAN_POINT('Ctrl Pts',(56.9187227990959,28.4545196380427,5.17241719114263));
#43328=CARTESIAN_POINT('Ctrl Pts',(56.9175440065505,28.4503901486285,5.17214125254017));
#43329=CARTESIAN_POINT('Ctrl Pts',(56.9149256185164,28.4413285089472,5.17153688741819));
#43330=CARTESIAN_POINT('Ctrl Pts',(56.9134803030432,28.4363981097868,5.17120879469745));
#43331=CARTESIAN_POINT('Ctrl Pts',(56.9092889252682,28.4223020596539,5.17027274960637));
#43332=CARTESIAN_POINT('Ctrl Pts',(56.9064959004578,28.413150359488,5.16966742812156));
#43333=CARTESIAN_POINT('Ctrl Pts',(56.8867265109213,28.3500044937226,5.16550510092732));
#43334=CARTESIAN_POINT('Ctrl Pts',(56.867522923147,28.2967287121739,5.16206583302436));
#43335=CARTESIAN_POINT('Ctrl Pts',(56.8096549510096,28.1553578307649,5.15295800487276));
#43336=CARTESIAN_POINT('Ctrl Pts',(56.7668454527477,28.0691237814998,5.14741794081993));
#43337=CARTESIAN_POINT('Ctrl Pts',(56.65092522318,27.8726645194238,5.13415503046321));
#43338=CARTESIAN_POINT('Ctrl Pts',(56.5727684096054,27.7659690937386,5.12640349020351));
#43339=CARTESIAN_POINT('Ctrl Pts',(56.4740858556187,27.6559951531108,5.1172318081291));
#43340=CARTESIAN_POINT('Ctrl Pts',(56.4633742118408,27.6443400013257,5.11624370547335));
#43341=CARTESIAN_POINT('Ctrl Pts',(56.4457379630333,27.6256029071172,5.11462805256785));
#43342=CARTESIAN_POINT('Ctrl Pts',(56.4388972015588,27.6184427393707,5.11400403940678));
#43343=CARTESIAN_POINT('Ctrl Pts',(56.426603127475,27.6057649925271,5.11288712632583));
#43344=CARTESIAN_POINT('Ctrl Pts',(56.4211703721253,27.6002276935041,5.11239511613917));
#43345=CARTESIAN_POINT('Ctrl Pts',(56.4096259472681,27.5885976037271,5.11135278914394));
#43346=CARTESIAN_POINT('Ctrl Pts',(56.403506775353,27.5825125174658,5.11080215025016));
#43347=CARTESIAN_POINT('Ctrl Pts',(56.3871189647084,27.5664261412988,5.10933224400521));
#43348=CARTESIAN_POINT('Ctrl Pts',(56.3767818306701,27.5564956516279,5.10840995972341));
#43349=CARTESIAN_POINT('Ctrl Pts',(56.3260199437685,27.5087719415706,5.10390369762393));
#43350=CARTESIAN_POINT('Ctrl Pts',(56.2841447678497,27.4725638307195,5.10025437425244));
#43351=CARTESIAN_POINT('Ctrl Pts',(56.0734505989827,27.3051769295966,5.08220053443745));
#43352=CARTESIAN_POINT('Ctrl Pts',(55.8858329932664,27.2000006483006,5.06684547522726));
#43353=CARTESIAN_POINT('Ctrl Pts',(55.6634479072121,27.1186713946938,5.05102880771687));
#43354=CARTESIAN_POINT('Ctrl Pts',(55.6416308196626,27.1111192608178,5.04950276410035));
#43355=CARTESIAN_POINT('Ctrl Pts',(55.6126294895628,27.101640763293,5.04751226900416));
#43356=CARTESIAN_POINT('Ctrl Pts',(55.6055595562046,27.0993737055664,5.04702998956829));
#43357=CARTESIAN_POINT('Ctrl Pts',(55.5940210191816,27.0957446570491,5.04624788457996));
#43358=CARTESIAN_POINT('Ctrl Pts',(55.5895600618636,27.0943588172985,5.04594672550576));
#43359=CARTESIAN_POINT('Ctrl Pts',(55.5808893885261,27.0916985495937,5.04536377671824));
#43360=CARTESIAN_POINT('Ctrl Pts',(55.5766802665595,27.0904223560222,5.04508188391851));
#43361=CARTESIAN_POINT('Ctrl Pts',(55.5666610625676,27.087420711204,5.04441340645468));
#43362=CARTESIAN_POINT('Ctrl Pts',(55.5608472302511,27.0857077855469,5.04402752588487));
#43363=CARTESIAN_POINT('Ctrl Pts',(55.5412450761933,27.0800293834263,5.04273297309114));
#43364=CARTESIAN_POINT('Ctrl Pts',(55.5274214394433,27.076186065855,5.04183083974647));
#43365=CARTESIAN_POINT('Ctrl Pts',(55.4492052358708,27.0553464697595,5.03678092316811));
#43366=CARTESIAN_POINT('Ctrl Pts',(55.3840284318532,27.0414325067611,5.0327797115616));
#43367=CARTESIAN_POINT('Ctrl Pts',(55.1460042396163,27.0029617864523,5.01851942570968));
#43368=CARTESIAN_POINT('Ctrl Pts',(54.9708367400101,26.9978438435076,5.00861485645763));
#43369=CARTESIAN_POINT('Ctrl Pts',(54.7611181533047,27.0192725900574,4.99576917198283));
#43370=CARTESIAN_POINT('Ctrl Pts',(54.7251106133381,27.0239480808233,4.99353136743136));
#43371=CARTESIAN_POINT('Ctrl Pts',(54.6765202248454,27.0316111829569,4.99045846631094));
#43372=CARTESIAN_POINT('Ctrl Pts',(54.6638081538849,27.0337424557005,4.98964960337045));
#43373=CARTESIAN_POINT('Ctrl Pts',(54.6437047885457,27.0373135827476,4.98836222373275));
#43374=CARTESIAN_POINT('Ctrl Pts',(54.6362993164737,27.0386723729802,4.98788622068686));
#43375=CARTESIAN_POINT('Ctrl Pts',(54.6211783414933,27.0415354218614,4.9869105777871));
#43376=CARTESIAN_POINT('Ctrl Pts',(54.6134636908624,27.043043426221,4.98641082930076));
#43377=CARTESIAN_POINT('Ctrl Pts',(54.5957260146967,27.0466196366109,4.98525713768923));
#43378=CARTESIAN_POINT('Ctrl Pts',(54.5857096563399,27.048719445059,4.98460221884103));
#43379=CARTESIAN_POINT('Ctrl Pts',(54.5543373009053,27.0555487248541,4.98253989138371));
#43380=CARTESIAN_POINT('Ctrl Pts',(54.5330432515918,27.0605523116497,4.98112394801785));
#43381=CARTESIAN_POINT('Ctrl Pts',(54.4280885468073,27.0870427671995,4.97406211674203));
#43382=CARTESIAN_POINT('Ctrl Pts',(54.3458130270717,27.1135949456928,4.9682581280078));
#43383=CARTESIAN_POINT('Ctrl Pts',(54.1227950888987,27.2019159713303,4.95180333239948));
#43384=CARTESIAN_POINT('Ctrl Pts',(53.9871081654211,27.2747115301222,4.94091516715197));
#43385=CARTESIAN_POINT('Ctrl Pts',(53.8611373905627,27.3623127528964,4.93049999999996));
#43386=CARTESIAN_POINT('',(56.1603489846691,27.3774656255483,4.9305));
#43387=CARTESIAN_POINT('Origin',(55.,29.,4.9305));
#43388=CARTESIAN_POINT('Ctrl Pts',(56.1603489846691,27.3774656255483,4.9305));
#43389=CARTESIAN_POINT('Ctrl Pts',(56.2184216902281,27.4189960892435,4.93505709699294));
#43390=CARTESIAN_POINT('Ctrl Pts',(56.2743063157546,27.4636793687382,4.93961419398587));
#43391=CARTESIAN_POINT('Ctrl Pts',(56.3276577251371,27.5112580722691,4.9441712909788));
#43392=CARTESIAN_POINT('Ctrl Pts',(56.382795092379,27.5604294902287,4.94888093845325));
#43393=CARTESIAN_POINT('Ctrl Pts',(56.4352261996819,27.6126933573083,4.95359058592769));
#43394=CARTESIAN_POINT('Ctrl Pts',(56.484606964112,27.6677201027524,4.95830023340213));
#43395=CARTESIAN_POINT('Ctrl Pts',(56.5323524863125,27.7209246395096,4.96285392107065));
#43396=CARTESIAN_POINT('Ctrl Pts',(56.5772462315824,27.7767115451888,4.96740760873917));
#43397=CARTESIAN_POINT('Ctrl Pts',(56.6190157492701,27.834746565714,4.97196129640769));
#43398=CARTESIAN_POINT('Ctrl Pts',(56.6607857488445,27.8927822557777,4.97651503661119));
#43399=CARTESIAN_POINT('Ctrl Pts',(56.6994311820518,27.9530657412654,4.98106877681469));
#43400=CARTESIAN_POINT('Ctrl Pts',(56.7347219369901,28.0152323300263,4.9856225170182));
#43401=CARTESIAN_POINT('Ctrl Pts',(56.770022593053,28.0774163601582,4.99017753481266));
#43402=CARTESIAN_POINT('Ctrl Pts',(56.8019664744604,28.1414841461348,4.99473255260713));
#43403=CARTESIAN_POINT('Ctrl Pts',(56.8303692593991,28.2070460689631,4.99928757040159));
#43404=CARTESIAN_POINT('Ctrl Pts',(56.8587876569103,28.2726440301685,5.00384509201904));
#43405=CARTESIAN_POINT('Ctrl Pts',(56.8836609071208,28.3397373416821,5.00840261363649));
#43406=CARTESIAN_POINT('Ctrl Pts',(56.9048531997708,28.4079173623362,5.01296013525394));
#43407=CARTESIAN_POINT('Ctrl Pts',(56.9260780688309,28.4762021880885,5.01752466261144));
#43408=CARTESIAN_POINT('Ctrl Pts',(56.9436105518529,28.5455766198122,5.02208918996893));
#43409=CARTESIAN_POINT('Ctrl Pts',(56.9573651317897,28.6156182843135,5.02665371732643));
#43410=CARTESIAN_POINT('Ctrl Pts',(56.9711320025852,28.6857225368555,5.03122232346797));
#43411=CARTESIAN_POINT('Ctrl Pts',(56.9811141820617,28.7564947577038,5.03579092960952));
#43412=CARTESIAN_POINT('Ctrl Pts',(56.9872779160048,28.8275063854523,5.04035953575106));
#43413=CARTESIAN_POINT('Ctrl Pts',(56.9934529543083,28.8986482493601,5.04493652076993));
#43414=CARTESIAN_POINT('Ctrl Pts',(56.9957955514951,28.970029940603,5.0495135057888));
#43415=CARTESIAN_POINT('Ctrl Pts',(56.9943240157816,29.0412223553015,5.05409049080767));
#43416=CARTESIAN_POINT('Ctrl Pts',(56.9939904687856,29.0573592494626,5.05512793732693));
#43417=CARTESIAN_POINT('Ctrl Pts',(56.9934611719914,29.0734864424386,5.05616538384619));
#43418=CARTESIAN_POINT('Ctrl Pts',(56.9927367071262,29.0895989875611,5.05720283036545));
#43419=CARTESIAN_POINT('Ctrl Pts',(56.9896539144736,29.1581621962148,5.0616174440485));
#43420=CARTESIAN_POINT('Ctrl Pts',(56.9830210524896,29.2267271840215,5.06603205773156));
#43421=CARTESIAN_POINT('Ctrl Pts',(56.9728321611652,29.29489121108,5.07044667141461));
#43422=CARTESIAN_POINT('Ctrl Pts',(56.9626601262909,29.362942467918,5.07485398158319));
#43423=CARTESIAN_POINT('Ctrl Pts',(56.948943803451,29.4305935908549,5.07926129175177));
#43424=CARTESIAN_POINT('Ctrl Pts',(56.9317292042771,29.4974433071647,5.08366860192035));
#43425=CARTESIAN_POINT('Ctrl Pts',(56.9145379279213,29.5642024536182,5.08806994094245));
#43426=CARTESIAN_POINT('Ctrl Pts',(56.8938579080394,29.6301618682264,5.09247127996455));
#43427=CARTESIAN_POINT('Ctrl Pts',(56.8697864793689,29.6949288338162,5.09687261898666));
#43428=CARTESIAN_POINT('Ctrl Pts',(56.8457327381214,29.7596482093469,5.10127072395289));
#43429=CARTESIAN_POINT('Ctrl Pts',(56.8182927014435,29.8231764060104,5.10566882891913));
#43430=CARTESIAN_POINT('Ctrl Pts',(56.7876135306692,29.8851358243052,5.11006693388537));
#43431=CARTESIAN_POINT('Ctrl Pts',(56.7569460005025,29.947071733318,5.11446337007723));
#43432=CARTESIAN_POINT('Ctrl Pts',(56.7230419956251,30.0074395973588,5.11885980626908));
#43433=CARTESIAN_POINT('Ctrl Pts',(56.6860960352171,30.0658835407892,5.12325624246093));
#43434=CARTESIAN_POINT('Ctrl Pts',(56.6491509646711,30.1243260765678,5.12765257276241));
#43435=CARTESIAN_POINT('Ctrl Pts',(56.6091643529584,30.1808443626743,5.13204890306389));
#43436=CARTESIAN_POINT('Ctrl Pts',(56.5663747139411,30.2351104477034,5.13644523336537));
#43437=CARTESIAN_POINT('Ctrl Pts',(56.5235418517711,30.2894313486022,5.14084600453759));
#43438=CARTESIAN_POINT('Ctrl Pts',(56.4779006207076,30.3414951143212,5.1452467757098));
#43439=CARTESIAN_POINT('Ctrl Pts',(56.4297299175529,30.3910068027707,5.14964754688202));
#43440=CARTESIAN_POINT('Ctrl Pts',(56.3815329085139,30.4405455294126,5.15405072130288));
#43441=CARTESIAN_POINT('Ctrl Pts',(56.3308040462454,30.4875290668789,5.15845389572373));
#43442=CARTESIAN_POINT('Ctrl Pts',(56.2778570511968,30.5317013152722,5.16285707014459));
#43443=CARTESIAN_POINT('Ctrl Pts',(56.2248163567507,30.575951734543,5.16726803678841));
#43444=CARTESIAN_POINT('Ctrl Pts',(56.1695500948677,30.6173806359082,5.17167900343223));
#43445=CARTESIAN_POINT('Ctrl Pts',(56.112402083768,30.6557744914476,5.17608997007605));
#43446=CARTESIAN_POINT('Ctrl Pts',(56.0786490002709,30.6784508888735,5.17869520029434));
#43447=CARTESIAN_POINT('Ctrl Pts',(56.0442399981255,30.7000693996835,5.18130043051263));
#43448=CARTESIAN_POINT('Ctrl Pts',(56.0092496154507,30.7205937278197,5.18390566073091));
#43449=CARTESIAN_POINT('Ctrl Pts',(55.9493356610869,30.7557374891994,5.18836659063431));
#43450=CARTESIAN_POINT('Ctrl Pts',(55.8874677711289,30.7878161804688,5.19282752053772));
#43451=CARTESIAN_POINT('Ctrl Pts',(55.8239917835498,30.8166081314203,5.19728845044112));
#43452=CARTESIAN_POINT('Ctrl Pts',(55.7606106181105,30.84535707218,5.20174271648729));
#43453=CARTESIAN_POINT('Ctrl Pts',(55.6956265641001,30.8708288185757,5.20619698253345));
#43454=CARTESIAN_POINT('Ctrl Pts',(55.6294115023349,30.8928467247055,5.21065124857962));
#43455=CARTESIAN_POINT('Ctrl Pts',(55.5632743336875,30.9148387297291,5.21510027478065));
#43456=CARTESIAN_POINT('Ctrl Pts',(55.4959094944692,30.9333848118939,5.21954930098167));
#43457=CARTESIAN_POINT('Ctrl Pts',(55.4277087213242,30.9483564386947,5.2239983271827));
#43458=CARTESIAN_POINT('Ctrl Pts',(55.3595508949386,30.9633186377014,5.22844455178415));
#43459=CARTESIAN_POINT('Ctrl Pts',(55.290558654364,30.9747107428247,5.23289077638559));
#43460=CARTESIAN_POINT('Ctrl Pts',(55.221137323565,30.9824545005186,5.23733700098703));
#43461=CARTESIAN_POINT('Ctrl Pts',(55.1517363292538,30.9901959897335,5.24178192309844));
#43462=CARTESIAN_POINT('Ctrl Pts',(55.0819069788018,30.99429119944,5.24622684520984));
#43463=CARTESIAN_POINT('Ctrl Pts',(55.0120614315314,30.9947135344128,5.25067176732124));
#43464=CARTESIAN_POINT('Ctrl Pts',(54.9422128242487,30.9951358878885,5.2551168841697));
#43465=CARTESIAN_POINT('Ctrl Pts',(54.8723485065069,30.9918850466157,5.25956200101816));
#43466=CARTESIAN_POINT('Ctrl Pts',(54.8028805958103,30.9849865246374,5.26400711786662));
#43467=CARTESIAN_POINT('Ctrl Pts',(54.7333411857832,30.9780809024066,5.26845680981853));
#43468=CARTESIAN_POINT('Ctrl Pts',(54.6641994834418,30.9675201544059,5.27290650177045));
#43469=CARTESIAN_POINT('Ctrl Pts',(54.5958614759773,30.9533815848167,5.27735619372237));
#43470=CARTESIAN_POINT('Ctrl Pts',(54.5274841733299,30.9392348853784,5.28180844430111));
#43471=CARTESIAN_POINT('Ctrl Pts',(54.4599119575084,30.9215063926186,5.28626069487986));
#43472=CARTESIAN_POINT('Ctrl Pts',(54.3935369530285,30.9003236922056,5.2907129454586));
#43473=CARTESIAN_POINT('Ctrl Pts',(54.3270498994079,30.8791052327988,5.29517271198187));
#43474=CARTESIAN_POINT('Ctrl Pts',(54.2617645475404,30.8544210985306,5.29963247850514));
#43475=CARTESIAN_POINT('Ctrl Pts',(54.1980535338539,30.8264472146591,5.30409224502841));
#43476=CARTESIAN_POINT('Ctrl Pts',(54.1670237598173,30.8128228309735,5.30626432705105));
#43477=CARTESIAN_POINT('Ctrl Pts',(54.1363670647112,30.7984187939596,5.3084364090737));
#43478=CARTESIAN_POINT('Ctrl Pts',(54.106124189597,30.7832592627199,5.31060849109635));
#43479=CARTESIAN_POINT('Ctrl Pts',(54.0439745802264,30.7521061748859,5.31507215563614));
#43480=CARTESIAN_POINT('Ctrl Pts',(53.9833383728733,30.717641484113,5.31953582017592));
#43481=CARTESIAN_POINT('Ctrl Pts',(53.9245898534785,30.6800358863008,5.3239994847157));
#43482=CARTESIAN_POINT('Ctrl Pts',(53.86594127085,30.6424942591534,5.32845555614157));
#43483=CARTESIAN_POINT('Ctrl Pts',(53.809174402341,30.6018226028416,5.33291162756744));
#43484=CARTESIAN_POINT('Ctrl Pts',(53.7546395290766,30.5582377417972,5.3373676989933));
#43485=CARTESIAN_POINT('Ctrl Pts',(53.7001568729434,30.5146946132494,5.34181950373159));
#43486=CARTESIAN_POINT('Ctrl Pts',(53.6479023507712,30.468244116519,5.34627130846988));
#43487=CARTESIAN_POINT('Ctrl Pts',(53.5981967552725,30.4191459493552,5.35072311320817));
#43488=CARTESIAN_POINT('Ctrl Pts',(53.5485220701845,30.3700783148608,5.35517214950336));
#43489=CARTESIAN_POINT('Ctrl Pts',(53.5013935113704,30.3183666195505,5.35962118579854));
#43490=CARTESIAN_POINT('Ctrl Pts',(53.4570969576199,30.2643092043936,5.36407022209372));
#43491=CARTESIAN_POINT('Ctrl Pts',(53.4128130845098,30.2102672640893,5.36851798477676));
#43492=CARTESIAN_POINT('Ctrl Pts',(53.3713599140202,30.1538813147802,5.37296574745979));
#43493=CARTESIAN_POINT('Ctrl Pts',(53.3329836074857,30.0954834136529,5.37741351014282));
#43494=CARTESIAN_POINT('Ctrl Pts',(53.2945859321945,30.0370529953124,5.38186374943623));
#43495=CARTESIAN_POINT('Ctrl Pts',(53.2592688143221,29.9766087928291,5.38631398872963));
#43496=CARTESIAN_POINT('Ctrl Pts',(53.2272349024942,29.9145116027504,5.39076422802304));
#43497=CARTESIAN_POINT('Ctrl Pts',(53.1951917413346,29.8523964830007,5.39521575225907));
#43498=CARTESIAN_POINT('Ctrl Pts',(53.166433881358,29.7886278665477,5.3996672764951));
#43499=CARTESIAN_POINT('Ctrl Pts',(53.1411167183624,29.7235886315776,5.40411880073113));
#43500=CARTESIAN_POINT('Ctrl Pts',(53.1157659750434,29.6584631294949,5.40857622940534));
#43501=CARTESIAN_POINT('Ctrl Pts',(53.0938652001118,29.5920641048668,5.41303365807955));
#43502=CARTESIAN_POINT('Ctrl Pts',(53.0755203145486,29.5247909133979,5.41749108675376));
#43503=CARTESIAN_POINT('Ctrl Pts',(53.0646592635329,29.4849619615071,5.42013009805002));
#43504=CARTESIAN_POINT('Ctrl Pts',(53.0550436614939,29.4448268458996,5.42276910934629));
#43505=CARTESIAN_POINT('Ctrl Pts',(53.0466869980082,29.4044698737233,5.42540812064255));
#43506=CARTESIAN_POINT('Origin',(55.,29.,3.45145488139523));
#43507=CARTESIAN_POINT('',(53.046686998162,29.4044698744659,6.38531629657044));
#43508=CARTESIAN_POINT('',(53.0466869743493,29.404469759467,6.22571516850574));
#43509=CARTESIAN_POINT('',(53.0466869980082,29.4044698737233,3.45145488139523));
#43510=CARTESIAN_POINT('Ctrl Pts',(53.046686998162,29.404469874466,6.38531629657044));
#43511=CARTESIAN_POINT('Ctrl Pts',(53.0475577577059,29.4086750478202,6.3850495438278));
#43512=CARTESIAN_POINT('Ctrl Pts',(53.0484421144563,29.4128774942598,6.38478237233183));
#43513=CARTESIAN_POINT('Ctrl Pts',(53.0523440964602,29.4311269716662,6.38361954233214));
#43514=CARTESIAN_POINT('Ctrl Pts',(53.0554997775915,29.4451436311797,6.38271967662396));
#43515=CARTESIAN_POINT('Ctrl Pts',(53.0607878336167,29.4675016961701,6.3812729657046));
#43516=CARTESIAN_POINT('Ctrl Pts',(53.0628233126949,29.4758656749478,6.3807292136261));
#43517=CARTESIAN_POINT('Ctrl Pts',(53.0665974895298,29.4909485293677,6.37974394047379));
#43518=CARTESIAN_POINT('Ctrl Pts',(53.0683172448876,29.4976720381938,6.37930303275358));
#43519=CARTESIAN_POINT('Ctrl Pts',(53.0724552326884,29.5135051750495,6.3782606605891));
#43520=CARTESIAN_POINT('Ctrl Pts',(53.0749029962216,29.5226068463296,6.37765825571887));
#43521=CARTESIAN_POINT('Ctrl Pts',(53.0822629929287,29.5492204737721,6.37588723677603));
#43522=CARTESIAN_POINT('Ctrl Pts',(53.0873502347284,29.5666826240363,6.37471301778809));
#43523=CARTESIAN_POINT('Ctrl Pts',(53.1331129653527,29.7161236791144,6.36455608905531));
#43524=CARTESIAN_POINT('Ctrl Pts',(53.1871467797638,29.8435935797991,6.35512532152846));
#43525=CARTESIAN_POINT('Ctrl Pts',(53.3193420074771,30.0829309865168,6.33610672863624));
#43526=CARTESIAN_POINT('Ctrl Pts',(53.3966842572105,30.1944601285966,6.32658202078836));
#43527=CARTESIAN_POINT('Ctrl Pts',(53.4945899246505,30.3088154226263,6.31662114456524));
#43528=CARTESIAN_POINT('Ctrl Pts',(53.5045788510581,30.3202169995012,6.31562595680132));
#43529=CARTESIAN_POINT('Ctrl Pts',(53.5185227850067,30.3357715641854,6.31426673347779));
#43530=CARTESIAN_POINT('Ctrl Pts',(53.5223668791216,30.3400226760234,6.3138950921806));
#43531=CARTESIAN_POINT('Ctrl Pts',(53.5289848395267,30.3472782488259,6.3132606075992));
#43532=CARTESIAN_POINT('Ctrl Pts',(53.5317496932293,30.3502908277484,6.31299710819081));
#43533=CARTESIAN_POINT('Ctrl Pts',(53.5375254534981,30.3565453691546,6.31244996991303));
#43534=CARTESIAN_POINT('Ctrl Pts',(53.5405379022808,30.3597858373589,6.31216646076998));
#43535=CARTESIAN_POINT('Ctrl Pts',(53.5478677253153,30.3676180542884,6.31148105351671));
#43536=CARTESIAN_POINT('Ctrl Pts',(53.5521961763001,30.3721994666395,6.31107998818048));
#43537=CARTESIAN_POINT('Ctrl Pts',(53.5675487818023,30.3882957861287,6.30967005721075));
#43538=CARTESIAN_POINT('Ctrl Pts',(53.5786895164332,30.3996993352801,6.30866967152245));
#43539=CARTESIAN_POINT('Ctrl Pts',(53.606500431757,30.4274918274352,6.30622402887145));
#43540=CARTESIAN_POINT('Ctrl Pts',(53.6233246014926,30.4437239724474,6.30478901517503));
#43541=CARTESIAN_POINT('Ctrl Pts',(53.693921730673,30.5094802770394,6.29892825857359));
#43542=CARTESIAN_POINT('Ctrl Pts',(53.7501151197452,30.556329200335,6.29463669068409));
#43543=CARTESIAN_POINT('Ctrl Pts',(53.9444795087286,30.7010395168376,6.28051916701322));
#43544=CARTESIAN_POINT('Ctrl Pts',(54.0924900601227,30.7843987763376,6.27082727671733));
#43545=CARTESIAN_POINT('Ctrl Pts',(54.2703416742453,30.8566488662321,6.25898423167699));
#43546=CARTESIAN_POINT('Ctrl Pts',(54.2915870353529,30.8648585175939,6.25756793671175));
#43547=CARTESIAN_POINT('Ctrl Pts',(54.3225435101036,30.8762154208556,6.25549990560979));
#43548=CARTESIAN_POINT('Ctrl Pts',(54.3321460265683,30.8796549324716,6.25485781939521));
#43549=CARTESIAN_POINT('Ctrl Pts',(54.349126735079,30.8855906815297,6.25372114505847));
#43550=CARTESIAN_POINT('Ctrl Pts',(54.3564940141228,30.8881176522166,6.25322757878406));
#43551=CARTESIAN_POINT('Ctrl Pts',(54.3717748255173,30.8932591345568,6.25220292337203));
#43552=CARTESIAN_POINT('Ctrl Pts',(54.3796903100954,30.8958673227831,6.25167163843889));
#43553=CARTESIAN_POINT('Ctrl Pts',(54.4001079112635,30.9024534604454,6.25029978465087));
#43554=CARTESIAN_POINT('Ctrl Pts',(54.4126331911631,30.9063577590828,6.24945683764299));
#43555=CARTESIAN_POINT('Ctrl Pts',(54.4662363949388,30.9224881866546,6.24584289566559));
#43556=CARTESIAN_POINT('Ctrl Pts',(54.5076614810664,30.9335115029647,6.24303353913215));
#43557=CARTESIAN_POINT('Ctrl Pts',(54.6200143082666,30.9595642119622,6.23536469466131));
#43558=CARTESIAN_POINT('Ctrl Pts',(54.6914547175895,30.9720747947637,6.230434387143));
#43559=CARTESIAN_POINT('Ctrl Pts',(54.8476731469693,30.9907349035604,6.21958026410742));
#43560=CARTESIAN_POINT('Ctrl Pts',(54.9324898441911,30.9954123754082,6.21364027235125));
#43561=CARTESIAN_POINT('Ctrl Pts',(55.106568590734,30.9938988192544,6.20154404726113));
#43562=CARTESIAN_POINT('Ctrl Pts',(55.195652684769,30.9871369211181,6.19540606022436));
#43563=CARTESIAN_POINT('Ctrl Pts',(55.2945143044327,30.9729170952118,6.18884583894524));
#43564=CARTESIAN_POINT('Ctrl Pts',(55.3050231372263,30.9713197198053,6.18815177029238));
#43565=CARTESIAN_POINT('Ctrl Pts',(55.3208738186932,30.9687805782239,6.187110345199));
#43566=CARTESIAN_POINT('Ctrl Pts',(55.3262252224566,30.9679009321158,6.18675968708387));
#43567=CARTESIAN_POINT('Ctrl Pts',(55.3358167149142,30.966284113986,6.18613296086047));
#43568=CARTESIAN_POINT('Ctrl Pts',(55.3400580499016,30.9655550378235,6.1858564511367));
#43569=CARTESIAN_POINT('Ctrl Pts',(55.3493268409547,30.9639308530502,6.18525355846166));
#43570=CARTESIAN_POINT('Ctrl Pts',(55.3543532240828,30.9630301656761,6.18492749189933));
#43571=CARTESIAN_POINT('Ctrl Pts',(55.368670060394,30.9604079226805,6.18400110237566));
#43572=CARTESIAN_POINT('Ctrl Pts',(55.3779519649456,30.9586396190321,6.18340333903162));
#43573=CARTESIAN_POINT('Ctrl Pts',(55.4402296428418,30.9463158410065,6.17940953647328));
#43574=CARTESIAN_POINT('Ctrl Pts',(55.4927953112126,30.9336756221015,6.17612093106042));
#43575=CARTESIAN_POINT('Ctrl Pts',(55.7230093482689,30.8683169486861,6.16182789922688));
#43576=CARTESIAN_POINT('Ctrl Pts',(55.8933151965619,30.7931387684466,6.15146135865577));
#43577=CARTESIAN_POINT('Ctrl Pts',(56.0933143678857,30.6691890199001,6.13729124872138));
#43578=CARTESIAN_POINT('Ctrl Pts',(56.1348117795988,30.6412586292119,6.13423393558637));
#43579=CARTESIAN_POINT('Ctrl Pts',(56.1868396443677,30.6033234988697,6.13022193770194));
#43580=CARTESIAN_POINT('Ctrl Pts',(56.1983733308368,30.5947212691795,6.12932078455072));
#43581=CARTESIAN_POINT('Ctrl Pts',(56.2166608143533,30.5807713970762,6.12787246908252));
#43582=CARTESIAN_POINT('Ctrl Pts',(56.2234749190573,30.5755033689872,6.1273284116399));
#43583=CARTESIAN_POINT('Ctrl Pts',(56.2357172707347,30.5659114114955,6.12634285411743));
#43584=CARTESIAN_POINT('Ctrl Pts',(56.2411575042861,30.5616029487089,6.12590196942683));
#43585=CARTESIAN_POINT('Ctrl Pts',(56.253928376632,30.5513800009336,6.12486001076704));
#43586=CARTESIAN_POINT('Ctrl Pts',(56.2612397745039,30.5454418485448,6.12425799898747));
#43587=CARTESIAN_POINT('Ctrl Pts',(56.2825211524651,30.5279059915603,6.12248938950158));
#43588=CARTESIAN_POINT('Ctrl Pts',(56.2963748692234,30.5161693137892,6.12131721077876));
#43589=CARTESIAN_POINT('Ctrl Pts',(56.4169083904272,30.4111951722558,6.11093020929373));
#43590=CARTESIAN_POINT('Ctrl Pts',(56.5135127305351,30.3070447673084,6.10124183258951));
#43591=CARTESIAN_POINT('Ctrl Pts',(56.6770293303521,30.0880859772198,6.08222299174596));
#43592=CARTESIAN_POINT('Ctrl Pts',(56.7451713177668,29.9750595243364,6.07297227009244));
#43593=CARTESIAN_POINT('Ctrl Pts',(56.808250511512,29.8423133853931,6.06324569867088));
#43594=CARTESIAN_POINT('Ctrl Pts',(56.8146595391249,29.8284156822456,6.06224078732908));
#43595=CARTESIAN_POINT('Ctrl Pts',(56.8232561111802,29.8091957635382,6.06087073666968));
#43596=CARTESIAN_POINT('Ctrl Pts',(56.8255813300257,29.8039362164424,6.06049783235387));
#43597=CARTESIAN_POINT('Ctrl Pts',(56.8295230486201,29.7949149258377,6.05986174674027));
#43598=CARTESIAN_POINT('Ctrl Pts',(56.8311507549924,29.7911581624284,6.05959790227346));
#43599=CARTESIAN_POINT('Ctrl Pts',(56.8345116429221,29.7833352610723,6.05905069108301));
#43600=CARTESIAN_POINT('Ctrl Pts',(56.8362428868957,29.7792683491474,6.05876745098275));
#43601=CARTESIAN_POINT('Ctrl Pts',(56.8404014108947,29.7694086408904,6.05808369670317));
#43602=CARTESIAN_POINT('Ctrl Pts',(56.8428149040626,29.7636100063569,6.05768400566394));
#43603=CARTESIAN_POINT('Ctrl Pts',(56.8512049999241,29.7431805872103,6.05628405327668));
#43604=CARTESIAN_POINT('Ctrl Pts',(56.8570352585872,29.7284898228396,6.0552921147949));
#43605=CARTESIAN_POINT('Ctrl Pts',(56.8921764506903,29.6367785409774,6.04918175999137));
#43606=CARTESIAN_POINT('Ctrl Pts',(56.9168689473078,29.5580637745161,6.04429321371887));
#43607=CARTESIAN_POINT('Ctrl Pts',(56.9689901415571,29.346911362959,6.03156764190196));
#43608=CARTESIAN_POINT('Ctrl Pts',(56.9879556947468,29.2128408072602,6.02385372205077));
#43609=CARTESIAN_POINT('Ctrl Pts',(56.9955874830295,29.0175227669985,6.01216657970325));
#43610=CARTESIAN_POINT('Ctrl Pts',(56.9952028185878,28.9570919116139,6.00849340824957));
#43611=CARTESIAN_POINT('Ctrl Pts',(56.9912942792531,28.8816629345709,6.00379313353684));
#43612=CARTESIAN_POINT('Ctrl Pts',(56.9903392482068,28.8665600324685,6.00284628793918));
#43613=CARTESIAN_POINT('Ctrl Pts',(56.9885525216129,28.8426310381501,6.00133641452591));
#43614=CARTESIAN_POINT('Ctrl Pts',(56.9878336578241,28.8337969130465,6.0007769004887));
#43615=CARTESIAN_POINT('Ctrl Pts',(56.9863822791434,28.817320095069,5.9997292917177));
#43616=CARTESIAN_POINT('Ctrl Pts',(56.9856644662942,28.8096762464264,5.99924166446368));
#43617=CARTESIAN_POINT('Ctrl Pts',(56.9839673074789,28.7926594717303,5.99815239866943));
#43618=CARTESIAN_POINT('Ctrl Pts',(56.9829656355396,28.7832890056479,5.99755007337295));
#43619=CARTESIAN_POINT('Ctrl Pts',(56.9798367055823,28.7558589513339,5.99577935751434));
#43620=CARTESIAN_POINT('Ctrl Pts',(56.977528896779,28.7378213229256,5.99460536384981));
#43621=CARTESIAN_POINT('Ctrl Pts',(56.9556456152207,28.5835681260892,5.98448052866964));
#43622=CARTESIAN_POINT('Ctrl Pts',(56.9222727988645,28.4497098063835,5.97508500323398));
#43623=CARTESIAN_POINT('Ctrl Pts',(56.8291016025179,28.1926071917617,5.95606468749601));
#43624=CARTESIAN_POINT('Ctrl Pts',(56.7698616905146,28.0698973296001,5.94650046650399));
#43625=CARTESIAN_POINT('Ctrl Pts',(56.6906676757398,27.9412746936394,5.93650639913881));
#43626=CARTESIAN_POINT('Ctrl Pts',(56.6825887179724,27.9284815899359,5.93551305842408));
#43627=CARTESIAN_POINT('Ctrl Pts',(56.671251670743,27.9109737293185,5.93415591001705));
#43628=CARTESIAN_POINT('Ctrl Pts',(56.6681179045737,27.9061796200582,5.93378452604483));
#43629=CARTESIAN_POINT('Ctrl Pts',(56.6627122098043,27.8979871239202,5.93315038071906));
#43630=CARTESIAN_POINT('Ctrl Pts',(56.6604504252254,27.8945821343139,5.9328869645658));
#43631=CARTESIAN_POINT('Ctrl Pts',(56.6557185142516,27.8875058005912,5.93233987817836));
#43632=CARTESIAN_POINT('Ctrl Pts',(56.6532466223867,27.8838356984093,5.9320563382285));
#43633=CARTESIAN_POINT('Ctrl Pts',(56.6472223431152,27.8749551643968,5.9313706782385));
#43634=CARTESIAN_POINT('Ctrl Pts',(56.6436573809517,27.8697532365046,5.93096939263456));
#43635=CARTESIAN_POINT('Ctrl Pts',(56.6309806228752,27.8514423679364,5.92955777384316));
#43636=CARTESIAN_POINT('Ctrl Pts',(56.6217359096769,27.8384255928387,5.92855594811371));
#43637=CARTESIAN_POINT('Ctrl Pts',(56.5985458493377,27.8065900718251,5.92610611475485));
#43638=CARTESIAN_POINT('Ctrl Pts',(56.5844231661395,27.7879028844157,5.92466839662416));
#43639=CARTESIAN_POINT('Ctrl Pts',(56.5247348862797,27.7117496067061,5.91879102854432));
#43640=CARTESIAN_POINT('Ctrl Pts',(56.4763435904853,27.6565652956145,5.91448635577703));
#43641=CARTESIAN_POINT('Ctrl Pts',(56.3068538569417,27.4835314533684,5.90037613600066));
#43642=CARTESIAN_POINT('Ctrl Pts',(56.173863119453,27.3784009282983,5.89070219568259));
#43643=CARTESIAN_POINT('Ctrl Pts',(56.0096781102839,27.2795063715418,5.87887804894824));
#43644=CARTESIAN_POINT('Ctrl Pts',(55.989932314196,27.2680698168799,5.877459165992));
#43645=CARTESIAN_POINT('Ctrl Pts',(55.961075773484,27.2520111223426,5.87538802600159));
#43646=CARTESIAN_POINT('Ctrl Pts',(55.9521184228187,27.2471160159493,5.87474545992219));
#43647=CARTESIAN_POINT('Ctrl Pts',(55.9362596749008,27.2386067819257,5.8736082153047));
#43648=CARTESIAN_POINT('Ctrl Pts',(55.9293738867726,27.2349639031118,5.8731145617548));
#43649=CARTESIAN_POINT('Ctrl Pts',(55.915080062402,27.2275086874467,5.87209000016603));
#43650=CARTESIAN_POINT('Ctrl Pts',(55.9076691379463,27.2237022472976,5.8715588979476));
#43651=CARTESIAN_POINT('Ctrl Pts',(55.8885391944048,27.214027594944,5.87018810232118));
#43652=CARTESIAN_POINT('Ctrl Pts',(55.8767859406093,27.2082283258026,5.86934603801476));
#43653=CARTESIAN_POINT('Ctrl Pts',(55.8264725725348,27.1840163722682,5.86574130897188));
#43654=CARTESIAN_POINT('Ctrl Pts',(55.7873857472753,27.1667306052127,5.8629405285689));
#43655=CARTESIAN_POINT('Ctrl Pts',(55.6808782788926,27.1236632922674,5.85530227752049));
#43656=CARTESIAN_POINT('Ctrl Pts',(55.6125680720841,27.1002649630747,5.85039469938749));
#43657=CARTESIAN_POINT('Ctrl Pts',(55.4845628845463,27.0640420375499,5.84121842712118));
#43658=CARTESIAN_POINT('Ctrl Pts',(55.4252526805483,27.0501553485057,5.83697496078905));
#43659=CARTESIAN_POINT('Ctrl Pts',(55.2617105768291,27.0196817382267,5.8253810476877));
#43660=CARTESIAN_POINT('Ctrl Pts',(55.1566391858276,27.008613197887,5.81804295730451));
#43661=CARTESIAN_POINT('Ctrl Pts',(55.035125726017,27.0054946607225,5.80999018001432));
#43662=CARTESIAN_POINT('Ctrl Pts',(55.0190697773188,27.0052765235279,5.80893503327229));
#43663=CARTESIAN_POINT('Ctrl Pts',(54.9965058790845,27.0052424488411,5.80746629805671));
#43664=CARTESIAN_POINT('Ctrl Pts',(54.9899992872413,27.005264457284,5.8070444162579));
#43665=CARTESIAN_POINT('Ctrl Pts',(54.9794723796783,27.0053515737654,5.80636465061021));
#43666=CARTESIAN_POINT('Ctrl Pts',(54.9754520144618,27.0053970007593,5.80610569755592));
#43667=CARTESIAN_POINT('Ctrl Pts',(54.966936811138,27.0055189655325,5.80555866414862));
#43668=CARTESIAN_POINT('Ctrl Pts',(54.9624420376718,27.0055985430264,5.805270758795));
#43669=CARTESIAN_POINT('Ctrl Pts',(54.9512979714052,27.005833529729,5.80455896162135));
#43670=CARTESIAN_POINT('Ctrl Pts',(54.9446490464113,27.0060070025999,5.80413606072854));
#43671=CARTESIAN_POINT('Ctrl Pts',(54.9197422397878,27.0067815074211,5.80255813815024));
#43672=CARTESIAN_POINT('Ctrl Pts',(54.901491377328,27.0076000968734,5.80141449466457));
#43673=CARTESIAN_POINT('Ctrl Pts',(54.8552563327153,27.0103107343628,5.7985434660906));
#43674=CARTESIAN_POINT('Ctrl Pts',(54.8272953755409,27.0125424849386,5.79683152648397));
#43675=CARTESIAN_POINT('Ctrl Pts',(54.6992571707259,27.0254848122089,5.7890665801158));
#43676=CARTESIAN_POINT('Ctrl Pts',(54.6000267391681,27.0431706865036,5.78325205005792));
#43677=CARTESIAN_POINT('Ctrl Pts',(54.3760734205213,27.1008422786077,5.76981948414682));
#43678=CARTESIAN_POINT('Ctrl Pts',(54.2531177754162,27.1457492363395,5.76219700707953));
#43679=CARTESIAN_POINT('Ctrl Pts',(54.1134998649133,27.212896830897,5.75265944960527));
#43680=CARTESIAN_POINT('Ctrl Pts',(54.0917563790041,27.2238486348719,5.75114807200526));
#43681=CARTESIAN_POINT('Ctrl Pts',(54.0615508456732,27.2397623029425,5.74900912771438));
#43682=CARTESIAN_POINT('Ctrl Pts',(54.0529161107412,27.2443930774059,5.74839308955682));
#43683=CARTESIAN_POINT('Ctrl Pts',(54.0379725150755,27.2525495977891,5.74731878244174));
#43684=CARTESIAN_POINT('Ctrl Pts',(54.0316479982493,27.2560463915509,5.74686154023548));
#43685=CARTESIAN_POINT('Ctrl Pts',(54.018487193125,27.2634165987734,5.74590460938088));
#43686=CARTESIAN_POINT('Ctrl Pts',(54.0116545216558,27.2672961845632,5.74540470690573));
#43687=CARTESIAN_POINT('Ctrl Pts',(53.9955048697496,27.2765925491261,5.74421568460849));
#43688=CARTESIAN_POINT('Ctrl Pts',(53.9862085911298,27.2820446221659,5.74352530770837));
#43689=CARTESIAN_POINT('Ctrl Pts',(53.9551242679141,27.3006150906336,5.74119654131422));
#43690=CARTESIAN_POINT('Ctrl Pts',(53.9335437623622,27.3140743312885,5.73954588508074));
#43691=CARTESIAN_POINT('Ctrl Pts',(53.8825847818005,27.3472261651163,5.73556440955052));
#43692=CARTESIAN_POINT('Ctrl Pts',(53.8534619597361,27.3672941512569,5.73322037865256));
#43693=CARTESIAN_POINT('Ctrl Pts',(53.7416250368162,27.4488269815449,5.72394489698141));
#43694=CARTESIAN_POINT('Ctrl Pts',(53.6631983210278,27.5158833566747,5.71682370772235));
#43695=CARTESIAN_POINT('Ctrl Pts',(53.5031638095426,27.6757340626276,5.70106756344419));
#43696=CARTESIAN_POINT('Ctrl Pts',(53.4242602921459,27.7706715172439,5.69243888993308));
#43697=CARTESIAN_POINT('Ctrl Pts',(53.3457078404214,27.8852833528123,5.68323763011562));
#43698=CARTESIAN_POINT('Ctrl Pts',(53.3369553689962,27.8983837578626,5.68220265405569));
#43699=CARTESIAN_POINT('Ctrl Pts',(53.3248360932572,27.9169971711783,5.68075707727969));
#43700=CARTESIAN_POINT('Ctrl Pts',(53.3213397072533,27.9224245427696,5.6803385187077));
#43701=CARTESIAN_POINT('Ctrl Pts',(53.3154995188614,27.9315875619623,5.67963694126219));
#43702=CARTESIAN_POINT('Ctrl Pts',(53.3131416647818,27.9353141464132,5.67935301321466));
#43703=CARTESIAN_POINT('Ctrl Pts',(53.3083534486854,27.9429377500027,5.67877507718099));
#43704=CARTESIAN_POINT('Ctrl Pts',(53.3059241555526,27.9468353930945,5.6784811390642));
#43705=CARTESIAN_POINT('Ctrl Pts',(53.2997610064949,27.956800268785,5.67773346563248));
#43706=CARTESIAN_POINT('Ctrl Pts',(53.2960461141464,27.9628792390494,5.6772809509678));
#43707=CARTESIAN_POINT('Ctrl Pts',(53.2810231671461,27.9877610847784,5.67544283002364));
#43708=CARTESIAN_POINT('Ctrl Pts',(53.2699926520123,28.006730830547,5.67407405642454));
#43709=CARTESIAN_POINT('Ctrl Pts',(53.2416492387349,28.0573796381182,5.67049436836086));
#43710=CARTESIAN_POINT('Ctrl Pts',(53.2248788409193,28.0893542271402,5.6683103904162));
#43711=CARTESIAN_POINT('Ctrl Pts',(53.1290871143118,28.2847063557645,5.65531361808838));
#43712=CARTESIAN_POINT('Ctrl Pts',(53.0717955771144,28.4577865181362,5.64515089894356));
#43713=CARTESIAN_POINT('Ctrl Pts',(53.0289208880002,28.6889544034501,5.63102947708381));
#43714=CARTESIAN_POINT('Ctrl Pts',(53.0212736085615,28.7420400547309,5.62775792800331));
#43715=CARTESIAN_POINT('Ctrl Pts',(53.0142632273663,28.8100159591008,5.62350212513587));
#43716=CARTESIAN_POINT('Ctrl Pts',(53.0129146975151,28.824681865257,5.62258006504534));
#43717=CARTESIAN_POINT('Ctrl Pts',(53.0110294845188,28.8480156521577,5.62110635272926));
#43718=CARTESIAN_POINT('Ctrl Pts',(53.0103867758722,28.856674608041,5.62055801017592));
#43719=CARTESIAN_POINT('Ctrl Pts',(53.0093333416006,28.8722434730398,5.61956935016476));
#43720=CARTESIAN_POINT('Ctrl Pts',(53.0089020099433,28.8791518842997,5.61912968257287));
#43721=CARTESIAN_POINT('Ctrl Pts',(53.007975516364,28.8953458771206,5.61809672794307));
#43722=CARTESIAN_POINT('Ctrl Pts',(53.0075093127419,28.9046328923534,5.6175025489317));
#43723=CARTESIAN_POINT('Ctrl Pts',(53.0063486368736,28.9315052685148,5.61577790630032));
#43724=CARTESIAN_POINT('Ctrl Pts',(53.0058219486616,28.94909663331,5.61464226610543));
#43725=CARTESIAN_POINT('Ctrl Pts',(53.0030727676453,29.1137177129465,5.60394993500629));
#43726=CARTESIAN_POINT('Ctrl Pts',(53.0168824057165,29.2605340668433,5.59387846756103));
#43727=CARTESIAN_POINT('Ctrl Pts',(53.0466869980211,29.4044698737854,5.5836423751603));
#43728=CARTESIAN_POINT('',(53.0052504464614,29.0013346002041,5.45145488139523));
#43729=CARTESIAN_POINT('Ctrl Pts',(53.0466869980082,29.4044698737233,5.42540812064255));
#43730=CARTESIAN_POINT('Ctrl Pts',(53.0341228174013,29.3437934700324,5.42937585424897));
#43731=CARTESIAN_POINT('Ctrl Pts',(53.0244059665824,29.2826156364975,5.43334358785539));
#43732=CARTESIAN_POINT('Ctrl Pts',(53.0175552112802,29.2212243706688,5.43731132146181));
#43733=CARTESIAN_POINT('Ctrl Pts',(53.009415042121,29.1482783571704,5.44202584143961));
#43734=CARTESIAN_POINT('Ctrl Pts',(53.0052996465098,29.0748710602292,5.44674036141742));
#43735=CARTESIAN_POINT('Ctrl Pts',(53.0052504464614,29.0013346002041,5.45145488139523));
#43736=CARTESIAN_POINT('Ctrl Pts',(53.0052504994822,29.0014116246202,5.45274812801779));
#43737=CARTESIAN_POINT('Ctrl Pts',(53.0051243702486,28.823179945905,5.46336349765806));
#43738=CARTESIAN_POINT('Ctrl Pts',(53.0288844422315,28.6457246371508,5.47335752524397));
#43739=CARTESIAN_POINT('Ctrl Pts',(53.0853141557639,28.4393971371445,5.48620705734885));
#43740=CARTESIAN_POINT('Ctrl Pts',(53.0956340276698,28.4052837002946,5.48837053488748));
#43741=CARTESIAN_POINT('Ctrl Pts',(53.1149113918893,28.3472204307118,5.49213320198773));
#43742=CARTESIAN_POINT('Ctrl Pts',(53.1234259273877,28.3231322993833,5.49371838887516));
#43743=CARTESIAN_POINT('Ctrl Pts',(53.1361781117867,28.289147583295,5.49599245218247));
#43744=CARTESIAN_POINT('Ctrl Pts',(53.140037078361,28.2791108877255,5.49666876644954));
#43745=CARTESIAN_POINT('Ctrl Pts',(53.1468394832641,28.261836945149,5.49784114265779));
#43746=CARTESIAN_POINT('Ctrl Pts',(53.1497446665786,28.254584817264,5.49833591375741));
#43747=CARTESIAN_POINT('Ctrl Pts',(53.1553962697641,28.2407134956761,5.4992872989044));
#43748=CARTESIAN_POINT('Ctrl Pts',(53.1581359101351,28.2340916572393,5.49974367781418));
#43749=CARTESIAN_POINT('Ctrl Pts',(53.1646621936556,28.2185548558603,5.50081975660486));
#43750=CARTESIAN_POINT('Ctrl Pts',(53.1684781785465,28.2096524886123,5.50144044466351));
#43751=CARTESIAN_POINT('Ctrl Pts',(53.1819369172502,28.1788753608719,5.50360079200397));
#43752=CARTESIAN_POINT('Ctrl Pts',(53.1919076432231,28.1571471108125,5.50515157542793));
#43753=CARTESIAN_POINT('Ctrl Pts',(53.2670189394738,28.0009338336864,5.5164924795253));
#43754=CARTESIAN_POINT('Ctrl Pts',(53.3466873599294,27.8739902781695,5.52680393141826));
#43755=CARTESIAN_POINT('Ctrl Pts',(53.4941863319689,27.6888233574931,5.54331678543631));
#43756=CARTESIAN_POINT('Ctrl Pts',(53.5530483972595,27.624139638695,5.54941695053602));
#43757=CARTESIAN_POINT('Ctrl Pts',(53.6346300899288,27.545536385824,5.55710080103722));
#43758=CARTESIAN_POINT('Ctrl Pts',(53.6536453904161,27.5279168520392,5.55884242915338));
#43759=CARTESIAN_POINT('Ctrl Pts',(53.6817359458982,27.5028879927363,5.56133829437962));
#43760=CARTESIAN_POINT('Ctrl Pts',(53.6905408397385,27.4951806749556,5.56210999418487));
#43761=CARTESIAN_POINT('Ctrl Pts',(53.7063212244745,27.4816107893552,5.56347352690025));
#43762=CARTESIAN_POINT('Ctrl Pts',(53.7132699465959,27.475717760212,5.56406733786493));
#43763=CARTESIAN_POINT('Ctrl Pts',(53.724123124669,27.466640571138,5.56498427985308));
#43764=CARTESIAN_POINT('Ctrl Pts',(53.7279995710887,27.463423334391,5.56530972473934));
#43765=CARTESIAN_POINT('Ctrl Pts',(53.7319064934698,27.4602057209625,5.56563562782453));
#43766=CARTESIAN_POINT('Ctrl Pts',(53.7319247720948,27.4601906678313,5.56563715252347));
#43767=CARTESIAN_POINT('Ctrl Pts',(53.7319614874054,27.4601604324972,5.56564021501336));
#43768=CARTESIAN_POINT('Ctrl Pts',(53.7319799240775,27.4601452503149,5.56564175280239));
#43769=CARTESIAN_POINT('Ctrl Pts',(53.732016958123,27.4601147547324,5.56564484169033));
#43770=CARTESIAN_POINT('Ctrl Pts',(53.7320355556297,27.4600994412323,5.56564639279954));
#43771=CARTESIAN_POINT('Ctrl Pts',(53.735364856519,27.4573581400278,5.56592406177133));
#43772=CARTESIAN_POINT('Ctrl Pts',(53.7386842826977,27.4546428840048,5.56619938894165));
#43773=CARTESIAN_POINT('Ctrl Pts',(53.7461805916915,27.448551225902,5.56681779141259));
#43774=CARTESIAN_POINT('Ctrl Pts',(53.7503623684838,27.4451809755419,5.56716042735255));
#43775=CARTESIAN_POINT('Ctrl Pts',(53.7626669133761,27.435345991954,5.56816194603189));
#43776=CARTESIAN_POINT('Ctrl Pts',(53.7708267416976,27.4289276133442,5.56881765231527));
#43777=CARTESIAN_POINT('Ctrl Pts',(53.8341825194713,27.3798888338048,5.57384716914853));
#43778=CARTESIAN_POINT('Ctrl Pts',(53.8915354636155,27.3401207356254,5.57804272504762));
#43779=CARTESIAN_POINT('Ctrl Pts',(54.0429511921845,27.2464866546377,5.58855820432079));
#43780=CARTESIAN_POINT('Ctrl Pts',(54.1395283222239,27.1971296729067,5.59476105051674));
#43781=CARTESIAN_POINT('Ctrl Pts',(54.3046189887543,27.1290608273355,5.60520978789602));
#43782=CARTESIAN_POINT('Ctrl Pts',(54.3709673988639,27.1057231059785,5.60936884213672));
#43783=CARTESIAN_POINT('Ctrl Pts',(54.4787135949044,27.0741099043881,5.61617737858332));
#43784=CARTESIAN_POINT('Ctrl Pts',(54.5193828199309,27.0635602469462,5.61875872796345));
#43785=CARTESIAN_POINT('Ctrl Pts',(54.5730770201309,27.0514275718044,5.62219545391431));
#43786=CARTESIAN_POINT('Ctrl Pts',(54.5858290390408,27.0486773354919,5.62301371825951));
#43787=CARTESIAN_POINT('Ctrl Pts',(54.6067665328694,27.0443762139883,5.62436098548788));
#43788=CARTESIAN_POINT('Ctrl Pts',(54.6149365019882,27.04275115246,5.62488763294647));
#43789=CARTESIAN_POINT('Ctrl Pts',(54.6307908632533,27.0397007231144,5.62591153718839));
#43790=CARTESIAN_POINT('Ctrl Pts',(54.6384739360747,27.0382692478609,5.62640859085829));
#43791=CARTESIAN_POINT('Ctrl Pts',(54.6562816734196,27.0350595572168,5.6275627499452));
#43792=CARTESIAN_POINT('Ctrl Pts',(54.6664119969846,27.0333143948594,5.62822088223868));
#43793=CARTESIAN_POINT('Ctrl Pts',(54.6993976136719,27.0278941122551,5.63036916625568));
#43794=CARTESIAN_POINT('Ctrl Pts',(54.7223027995737,27.0245386316445,5.63186924780907));
#43795=CARTESIAN_POINT('Ctrl Pts',(54.9086468084579,27.000545113172,5.64414509551553));
#43796=CARTESIAN_POINT('Ctrl Pts',(55.0739811408788,26.999832187681,5.65556413672351));
#43797=CARTESIAN_POINT('Ctrl Pts',(55.3122225787306,27.0283988556418,5.67227205711633));
#43798=CARTESIAN_POINT('Ctrl Pts',(55.3864006372345,27.0415848314658,5.67749720673242));
#43799=CARTESIAN_POINT('Ctrl Pts',(55.482818101896,27.0644172383239,5.68419592114564));
#43800=CARTESIAN_POINT('Ctrl Pts',(55.5058775449852,27.0703155800818,5.68579061934464));
#43801=CARTESIAN_POINT('Ctrl Pts',(55.5444164403186,27.0809117510184,5.6884374127566));
#43802=CARTESIAN_POINT('Ctrl Pts',(55.5599538682012,27.0853875919484,5.68949941407683));
#43803=CARTESIAN_POINT('Ctrl Pts',(55.5815177858884,27.0918844436673,5.6909646053593));
#43804=CARTESIAN_POINT('Ctrl Pts',(55.587591150264,27.0937459365562,5.69137629788698));
#43805=CARTESIAN_POINT('Ctrl Pts',(55.5978990541474,27.0969592647107,5.69207326035051));
#43806=CARTESIAN_POINT('Ctrl Pts',(55.6021381252689,27.0982962905482,5.69235937013802));
#43807=CARTESIAN_POINT('Ctrl Pts',(55.6102681678322,27.1008904599946,5.69290706460656));
#43808=CARTESIAN_POINT('Ctrl Pts',(55.6141597810002,27.1021454097484,5.69316877830027));
#43809=CARTESIAN_POINT('Ctrl Pts',(55.623484977232,27.1051842435332,5.69379488152643));
#43810=CARTESIAN_POINT('Ctrl Pts',(55.6289148385437,27.1069795575434,5.69415861312416));
#43811=CARTESIAN_POINT('Ctrl Pts',(55.6485755332966,27.1135740446853,5.69547285275241));
#43812=CARTESIAN_POINT('Ctrl Pts',(55.6627601933935,27.1185106790596,5.69641575326356));
#43813=CARTESIAN_POINT('Ctrl Pts',(55.8055803419602,27.1700314902501,5.70586866119001));
#43814=CARTESIAN_POINT('Ctrl Pts',(55.9291744147149,27.2295790814892,5.71372933708038));
#43815=CARTESIAN_POINT('Ctrl Pts',(56.1621867233661,27.3730220832878,5.72962830695051));
#43816=CARTESIAN_POINT('Ctrl Pts',(56.2709618187409,27.4565025581736,5.73763538125252));
#43817=CARTESIAN_POINT('Ctrl Pts',(56.3835069639838,27.5628971745225,5.74724001182875));
#43818=CARTESIAN_POINT('Ctrl Pts',(56.3965069076698,27.5755265977855,5.74837123807565));
#43819=CARTESIAN_POINT('Ctrl Pts',(56.4159953581795,27.5949827954121,5.75010169420315));
#43820=CARTESIAN_POINT('Ctrl Pts',(56.4226108175827,27.6016814896445,5.7506953355887));
#43821=CARTESIAN_POINT('Ctrl Pts',(56.4340211459099,27.6134001650665,5.75173028634165));
#43822=CARTESIAN_POINT('Ctrl Pts',(56.4388377279617,27.6183988492438,5.75217064420853));
#43823=CARTESIAN_POINT('Ctrl Pts',(56.4495781877454,27.6296624573515,5.75316050320812));
#43824=CARTESIAN_POINT('Ctrl Pts',(56.4554877061842,27.63594082368,5.7537106063262));
#43825=CARTESIAN_POINT('Ctrl Pts',(56.471170774334,27.6528207145162,5.75518535941987));
#43826=CARTESIAN_POINT('Ctrl Pts',(56.4808702423791,27.6634900742106,5.7561131031886));
#43827=CARTESIAN_POINT('Ctrl Pts',(56.523867797224,27.7118298689125,5.76029767083468));
#43828=CARTESIAN_POINT('Ctrl Pts',(56.5558476892036,27.7506431352072,5.7636078502144));
#43829=CARTESIAN_POINT('Ctrl Pts',(56.698622549301,27.9379187621129,5.77936465902168));
#43830=CARTESIAN_POINT('Ctrl Pts',(56.7898488000355,28.1001350618055,5.79252054339303));
#43831=CARTESIAN_POINT('Ctrl Pts',(56.8706229093093,28.3063741604563,5.80769572840009));
#43832=CARTESIAN_POINT('Ctrl Pts',(56.8829435403619,28.3405526460518,5.81015935008419));
#43833=CARTESIAN_POINT('Ctrl Pts',(56.9012306551285,28.3959838897776,5.81405391619489));
#43834=CARTESIAN_POINT('Ctrl Pts',(56.9077896145335,28.4170314339323,5.81550974967522));
#43835=CARTESIAN_POINT('Ctrl Pts',(56.9160096185182,28.4450354202302,5.8174126542167));
#43836=CARTESIAN_POINT('Ctrl Pts',(56.9179838361426,28.4518973170305,5.81787623902597));
#43837=CARTESIAN_POINT('Ctrl Pts',(56.9211689660514,28.4631960182846,5.8186349887387));
#43838=CARTESIAN_POINT('Ctrl Pts',(56.9224014349827,28.4676266021654,5.81893136447483));
#43839=CARTESIAN_POINT('Ctrl Pts',(56.9247844722703,28.476309534921,5.81950988132743));
#43840=CARTESIAN_POINT('Ctrl Pts',(56.9259362902992,28.4805614818496,5.81979208906304));
#43841=CARTESIAN_POINT('Ctrl Pts',(56.928737956676,28.4910412939383,5.82048505301578));
#43842=CARTESIAN_POINT('Ctrl Pts',(56.9303717548881,28.4972734732787,5.82089489565217));
#43843=CARTESIAN_POINT('Ctrl Pts',(56.9358812590743,28.5187125811551,5.8222973990816));
#43844=CARTESIAN_POINT('Ctrl Pts',(56.9396078098455,28.5339577180397,5.82328197444759));
#43845=CARTESIAN_POINT('Ctrl Pts',(56.9712177999448,28.6702250760193,5.83198231632844));
#43846=CARTESIAN_POINT('Ctrl Pts',(56.9879260019381,28.7935783999363,5.83916693255887));
#43847=CARTESIAN_POINT('Ctrl Pts',(56.9972739877713,29.0199539569346,5.85232212985626));
#43848=CARTESIAN_POINT('Ctrl Pts',(56.9936206220023,29.1223778672296,5.85826414135199));
#43849=CARTESIAN_POINT('Ctrl Pts',(56.9781703031958,29.2590559335216,5.86653324549573));
#43850=CARTESIAN_POINT('Ctrl Pts',(56.9732888401537,29.2939365033879,5.86867263638917));
#43851=CARTESIAN_POINT('Ctrl Pts',(56.9633109329982,29.3536666583885,5.87239869362057));
#43852=CARTESIAN_POINT('Ctrl Pts',(56.9586590426868,29.3785823418286,5.87397184714782));
#43853=CARTESIAN_POINT('Ctrl Pts',(56.9513588776086,29.4139344894648,5.87623382647598));
#43854=CARTESIAN_POINT('Ctrl Pts',(56.9490987794719,29.4244492566038,5.87691039112654));
#43855=CARTESIAN_POINT('Ctrl Pts',(56.9450429424901,29.4426026202448,5.87808523221383));
#43856=CARTESIAN_POINT('Ctrl Pts',(56.9432869413356,29.4502499176697,5.87858223550771));
#43857=CARTESIAN_POINT('Ctrl Pts',(56.9398284883154,29.4649141122475,5.87953937129112));
#43858=CARTESIAN_POINT('Ctrl Pts',(56.9381329629381,29.4719325286272,5.87999927546284));
#43859=CARTESIAN_POINT('Ctrl Pts',(56.9340476970148,29.4884495902442,5.88108595046646));
#43860=CARTESIAN_POINT('Ctrl Pts',(56.9316260430119,29.4979400775795,5.88171373521028));
#43861=CARTESIAN_POINT('Ctrl Pts',(56.9229374349614,29.5309733676697,5.88391093414111));
#43862=CARTESIAN_POINT('Ctrl Pts',(56.9163093613801,29.5544181100595,5.88549186943257));
#43863=CARTESIAN_POINT('Ctrl Pts',(56.8715252443568,29.7024172484047,5.89561314582776));
#43864=CARTESIAN_POINT('Ctrl Pts',(56.821680662501,29.8230829147425,5.90453613215046));
#43865=CARTESIAN_POINT('Ctrl Pts',(56.7128934658764,30.0272530140889,5.92063535153886));
#43866=CARTESIAN_POINT('Ctrl Pts',(56.6586242518417,30.112753321118,5.92772458299025));
#43867=CARTESIAN_POINT('Ctrl Pts',(56.5812801946533,30.216293863772,5.93650921685234));
#43868=CARTESIAN_POINT('Ctrl Pts',(56.5639815868616,30.2384585484714,5.9384018088601));
#43869=CARTESIAN_POINT('Ctrl Pts',(56.5346609473686,30.2744324394118,5.94148428674759));
#43870=CARTESIAN_POINT('Ctrl Pts',(56.5229074713133,30.2884545613956,5.94268858793973));
#43871=CARTESIAN_POINT('Ctrl Pts',(56.506621268824,30.3073500391843,5.9443130027469));
#43872=CARTESIAN_POINT('Ctrl Pts',(56.5022550572408,30.3123648572918,5.94474427130239));
#43873=CARTESIAN_POINT('Ctrl Pts',(56.4948980868386,30.3207298885599,5.94546377260231));
#43874=CARTESIAN_POINT('Ctrl Pts',(56.4919209725298,30.3240919686844,5.94575298735202));
#43875=CARTESIAN_POINT('Ctrl Pts',(56.4862582925413,30.3304435345939,5.9462993786686));
#43876=CARTESIAN_POINT('Ctrl Pts',(56.4835750153007,30.3334349948763,5.94655672566556));
#43877=CARTESIAN_POINT('Ctrl Pts',(56.4765294703774,30.3412421500516,5.94722843739487));
#43878=CARTESIAN_POINT('Ctrl Pts',(56.4721526374619,30.3460447231754,5.94764172506316));
#43879=CARTESIAN_POINT('Ctrl Pts',(56.4569143420002,30.3626020336426,5.94906722204481));
#43880=CARTESIAN_POINT('Ctrl Pts',(56.4459346074727,30.374247739958,5.95007099988089));
#43881=CARTESIAN_POINT('Ctrl Pts',(56.3554621189796,30.4679228967994,5.95816708621102));
#43882=CARTESIAN_POINT('Ctrl Pts',(56.2691868783676,30.5431288965373,5.96481328119672));
#43883=CARTESIAN_POINT('Ctrl Pts',(56.089622460271,30.6743493260088,5.97773281715732));
#43884=CARTESIAN_POINT('Ctrl Pts',(55.9972692535995,30.7309462415362,5.98398857887714));
#43885=CARTESIAN_POINT('Ctrl Pts',(55.8674839124194,30.7966336459837,5.99271437211588));
#43886=CARTESIAN_POINT('Ctrl Pts',(55.833715520682,30.8125504077134,5.99497783683222));
#43887=CARTESIAN_POINT('Ctrl Pts',(55.7752379966984,30.8381338879296,5.99890084547824));
#43888=CARTESIAN_POINT('Ctrl Pts',(55.7507456702286,30.8482724306315,6.0005448468812));
#43889=CARTESIAN_POINT('Ctrl Pts',(55.71585599014,30.8619070262258,6.00289136577377));
#43890=CARTESIAN_POINT('Ctrl Pts',(55.7056200106054,30.8658102706184,6.00358033635454));
#43891=CARTESIAN_POINT('Ctrl Pts',(55.6879581041119,30.8723790884211,6.00477030318122));
#43892=CARTESIAN_POINT('Ctrl Pts',(55.6805474863075,30.8750853099943,6.00526994212671));
#43893=CARTESIAN_POINT('Ctrl Pts',(55.6663532950211,30.8801735392379,6.0062276955104));
#43894=CARTESIAN_POINT('Ctrl Pts',(55.6595725021178,30.8825629773462,6.00668555571313));
#43895=CARTESIAN_POINT('Ctrl Pts',(55.6419401571575,30.8886693644042,6.00787706769655));
#43896=CARTESIAN_POINT('Ctrl Pts',(55.6310693180359,30.8923294216918,6.00861257155633));
#43897=CARTESIAN_POINT('Ctrl Pts',(55.593814228106,30.9045159604478,6.0111366146564));
#43898=CARTESIAN_POINT('Ctrl Pts',(55.5672850392769,30.9125856681373,6.01293986574604));
#43899=CARTESIAN_POINT('Ctrl Pts',(55.3366673240301,30.977515283591,6.02867353583479));
#43900=CARTESIAN_POINT('Ctrl Pts',(55.1249105147715,31.0020663939471,6.04371963022209));
#43901=CARTESIAN_POINT('Ctrl Pts',(54.8576520012668,30.9904452013711,6.06206383555487));
#43902=CARTESIAN_POINT('Ctrl Pts',(54.8020799479456,30.9856897895796,6.06582940817737));
#43903=CARTESIAN_POINT('Ctrl Pts',(54.7373301971144,30.9774030454849,6.07010717927522));
#43904=CARTESIAN_POINT('Ctrl Pts',(54.7278938533528,30.9761266364305,6.07072784137697));
#43905=CARTESIAN_POINT('Ctrl Pts',(54.7133946408433,30.9740595685501,6.07167688488032));
#43906=CARTESIAN_POINT('Ctrl Pts',(54.708325227481,30.9733169133662,6.07200783167734));
#43907=CARTESIAN_POINT('Ctrl Pts',(54.6990027647369,30.9719144883695,6.07261475753468));
#43908=CARTESIAN_POINT('Ctrl Pts',(54.6947490024847,30.9712604886903,6.07289104355579));
#43909=CARTESIAN_POINT('Ctrl Pts',(54.685156828082,30.969753934718,6.07351261889783));
#43910=CARTESIAN_POINT('Ctrl Pts',(54.6798197536788,30.9688934449975,6.07385746001496));
#43911=CARTESIAN_POINT('Ctrl Pts',(54.6640809465861,30.966290208159,6.07487159647397));
#43912=CARTESIAN_POINT('Ctrl Pts',(54.6536892708555,30.9644866208319,6.07553759346337));
#43913=CARTESIAN_POINT('Ctrl Pts',(54.5640058476712,30.9481873346454,6.08125805676871));
#43914=CARTESIAN_POINT('Ctrl Pts',(54.4856358216565,30.9289783568547,6.08607341876405));
#43915=CARTESIAN_POINT('Ctrl Pts',(54.3065952741266,30.8734014085041,6.09708469817586));
#43916=CARTESIAN_POINT('Ctrl Pts',(54.2072649467573,30.8335797700217,6.10320863638305));
#43917=CARTESIAN_POINT('Ctrl Pts',(54.0335066935849,30.7471479398676,6.11460409602138));
#43918=CARTESIAN_POINT('Ctrl Pts',(53.9580530074242,30.7032260891853,6.11981146278568));
#43919=CARTESIAN_POINT('Ctrl Pts',(53.8676154953236,30.642318290226,6.12654499117124));
#43920=CARTESIAN_POINT('Ctrl Pts',(53.8497124074744,30.6298289570712,6.1279033384047));
#43921=CARTESIAN_POINT('Ctrl Pts',(53.8238002977516,30.6111128435897,6.12990875840758));
#43922=CARTESIAN_POINT('Ctrl Pts',(53.8156276861906,30.6051144976518,6.13054713235738));
#43923=CARTESIAN_POINT('Ctrl Pts',(53.8012861823812,30.5944192848014,6.13167796634376));
#43924=CARTESIAN_POINT('Ctrl Pts',(53.7950982407657,30.5897482253925,6.13216942101721));
#43925=CARTESIAN_POINT('Ctrl Pts',(53.7830582056641,30.5805489494834,6.13313267118159));
#43926=CARTESIAN_POINT('Ctrl Pts',(53.7772037610154,30.5760240061703,6.13360433344885));
#43927=CARTESIAN_POINT('Ctrl Pts',(53.7614500986313,30.5637072647499,6.13488252164843));
#43928=CARTESIAN_POINT('Ctrl Pts',(53.7515994279111,30.5558541922768,6.1356914595393));
#43929=CARTESIAN_POINT('Ctrl Pts',(53.7147008787404,30.5258621934304,6.13875892187169));
#43930=CARTESIAN_POINT('Ctrl Pts',(53.6881634280438,30.5031080530749,6.14104195194072));
#43931=CARTESIAN_POINT('Ctrl Pts',(53.5118231726884,30.3436797899028,6.15675655580967));
#43932=CARTESIAN_POINT('Ctrl Pts',(53.3830373974161,30.1855572873459,6.17116159103879));
#43933=CARTESIAN_POINT('Ctrl Pts',(53.2523220195476,29.9631732114552,6.18884664082957));
#43934=CARTESIAN_POINT('Ctrl Pts',(53.2263097031231,29.9143877175651,6.19257837972626));
#43935=CARTESIAN_POINT('Ctrl Pts',(53.1982378937371,29.8560204997555,6.19682256392062));
#43936=CARTESIAN_POINT('Ctrl Pts',(53.1941820825243,29.8474310833616,6.1974416863755));
#43937=CARTESIAN_POINT('Ctrl Pts',(53.188036096121,29.8341705780667,6.19838876061404));
#43938=CARTESIAN_POINT('Ctrl Pts',(53.1859023462123,29.8295200095293,6.19871926490623));
#43939=CARTESIAN_POINT('Ctrl Pts',(53.1820074233556,29.8209440074579,6.19932565215712));
#43940=CARTESIAN_POINT('Ctrl Pts',(53.1802410617463,29.8170211009625,6.19960183975046));
#43941=CARTESIAN_POINT('Ctrl Pts',(53.1762826174932,29.808153281798,6.20022350419443));
#43942=CARTESIAN_POINT('Ctrl Pts',(53.1740979503492,29.8032051573978,6.20056853076356));
#43943=CARTESIAN_POINT('Ctrl Pts',(53.1677059792656,29.7885669161725,6.20158394798967));
#43944=CARTESIAN_POINT('Ctrl Pts',(53.1635554164891,29.7788520160157,6.20225102614816));
#43945=CARTESIAN_POINT('Ctrl Pts',(53.1278396634481,29.6933818431783,6.208064167495));
#43946=CARTESIAN_POINT('Ctrl Pts',(53.1008962968186,29.6157687884393,6.21296219580502));
#43947=CARTESIAN_POINT('Ctrl Pts',(53.0665961605006,29.4929885107095,6.22044491636916));
#43948=CARTESIAN_POINT('Ctrl Pts',(53.0558836360809,29.4488833620477,6.22308124932006));
#43949=CARTESIAN_POINT('Ctrl Pts',(53.0466869743493,29.404469759467,6.22571516850575));
#43950=CARTESIAN_POINT('Origin',(55.,29.,3.45145488139523));
#43951=CARTESIAN_POINT('',(53.0466869981335,29.4044698743284,7.18242967527062));
#43952=CARTESIAN_POINT('',(53.0466869980042,29.4044698737041,7.02360963496714));
#43953=CARTESIAN_POINT('',(53.0466869980082,29.4044698737233,3.45145488139523));
#43954=CARTESIAN_POINT('Ctrl Pts',(53.0466869981335,29.4044698743284,7.18242967527062));
#43955=CARTESIAN_POINT('Ctrl Pts',(53.0666916447592,29.5010786425753,7.17661931946525));
#43956=CARTESIAN_POINT('Ctrl Pts',(53.0938369179684,29.5960751312477,7.17095413793509));
#43957=CARTESIAN_POINT('Ctrl Pts',(53.1530599331324,29.7570666411215,7.16092930501707));
#43958=CARTESIAN_POINT('Ctrl Pts',(53.1819445957839,29.8240211123612,7.15662490802084));
#43959=CARTESIAN_POINT('Ctrl Pts',(53.233600278732,29.9277444422827,7.14960490747043));
#43960=CARTESIAN_POINT('Ctrl Pts',(53.2540144845991,29.9656147744896,7.14696331199493));
#43961=CARTESIAN_POINT('Ctrl Pts',(53.2822395067726,30.0141494034132,7.14345873691704));
#43962=CARTESIAN_POINT('Ctrl Pts',(53.2889552182893,30.0254393529079,7.14263487657998));
#43963=CARTESIAN_POINT('Ctrl Pts',(53.3001149317604,30.0437853399635,7.14128151710104));
#43964=CARTESIAN_POINT('Ctrl Pts',(53.3044926035728,30.0508814140537,7.14075443000207));
#43965=CARTESIAN_POINT('Ctrl Pts',(53.3130446597757,30.0645514939051,7.13973190469558));
#43966=CARTESIAN_POINT('Ctrl Pts',(53.3172133121716,30.0711289201349,7.13923668317857));
#43967=CARTESIAN_POINT('Ctrl Pts',(53.326926162893,30.0862575002357,7.13809006587162));
#43968=CARTESIAN_POINT('Ctrl Pts',(53.3324975556609,30.0947908535497,7.13743767277651));
#43969=CARTESIAN_POINT('Ctrl Pts',(53.3507036595188,30.1222146055288,7.13532252944452));
#43970=CARTESIAN_POINT('Ctrl Pts',(53.3635955057812,30.1409313303226,7.13385023040724));
#43971=CARTESIAN_POINT('Ctrl Pts',(53.4754177308781,30.2974828099682,7.12128492581618));
#43972=CARTESIAN_POINT('Ctrl Pts',(53.5912251323893,30.4223724427831,7.10950182275871));
#43973=CARTESIAN_POINT('Ctrl Pts',(53.7772962687928,30.5777600381371,7.09261792691267));
#43974=CARTESIAN_POINT('Ctrl Pts',(53.8357121773471,30.6213470895029,7.08756632949024));
#43975=CARTESIAN_POINT('Ctrl Pts',(53.9158119639947,30.6745470387087,7.08106784276053));
#43976=CARTESIAN_POINT('Ctrl Pts',(53.9354651670009,30.687109116457,7.07950561023867));
#43977=CARTESIAN_POINT('Ctrl Pts',(53.9688919564254,30.707658342189,7.07690775189745));
#43978=CARTESIAN_POINT('Ctrl Pts',(53.9825486509922,30.7158302951325,7.0758626004635));
#43979=CARTESIAN_POINT('Ctrl Pts',(54.0017451669593,30.7270073886353,7.07441750944381));
#43980=CARTESIAN_POINT('Ctrl Pts',(54.0072032173153,30.7301507977539,7.07400931112081));
#43981=CARTESIAN_POINT('Ctrl Pts',(54.0165198651018,30.7354578516306,7.0733171996565));
#43982=CARTESIAN_POINT('Ctrl Pts',(54.0203709131133,30.7376345945271,7.07303246319501));
#43983=CARTESIAN_POINT('Ctrl Pts',(54.0277965393561,30.7417992772045,7.07248606549673));
#43984=CARTESIAN_POINT('Ctrl Pts',(54.0313700135177,30.7437890471543,7.07222428269351));
#43985=CARTESIAN_POINT('Ctrl Pts',(54.0399689844973,30.7485425086628,7.07159707347549));
#43986=CARTESIAN_POINT('Ctrl Pts',(54.0450003643735,30.7512955642067,7.07123231311435));
#43987=CARTESIAN_POINT('Ctrl Pts',(54.0633979474697,30.7612594371632,7.0699063943199));
#43988=CARTESIAN_POINT('Ctrl Pts',(54.0768349079327,30.7683394626468,7.06895304585028));
#43989=CARTESIAN_POINT('Ctrl Pts',(54.2102501979229,30.8367016096683,7.05962200653594));
#43990=CARTESIAN_POINT('Ctrl Pts',(54.3360819729028,30.8858422229226,7.05187350183976));
#43991=CARTESIAN_POINT('Ctrl Pts',(54.5995404604579,30.9590538760853,7.0359899908337));
#43992=CARTESIAN_POINT('Ctrl Pts',(54.7366465759225,30.9821447891328,7.0278805683961));
#43993=CARTESIAN_POINT('Ctrl Pts',(54.8931849903518,30.9919711390948,7.01815480816874));
#43994=CARTESIAN_POINT('Ctrl Pts',(54.9113542428573,30.9928623537587,7.01701953450466));
#43995=CARTESIAN_POINT('Ctrl Pts',(54.9389525769092,30.9938379121207,7.0152843135652));
#43996=CARTESIAN_POINT('Ctrl Pts',(54.9483745749343,30.9941041142017,7.0146900090323));
#43997=CARTESIAN_POINT('Ctrl Pts',(54.965474619833,30.9944659730976,7.01360779829824));
#43998=CARTESIAN_POINT('Ctrl Pts',(54.9731520469343,30.9945840931025,7.01312059939424));
#43999=CARTESIAN_POINT('Ctrl Pts',(54.9896930383754,30.9947430641319,7.01206800895863));
#44000=CARTESIAN_POINT('Ctrl Pts',(54.9985565479559,30.994769169014,7.01150216965427));
#44001=CARTESIAN_POINT('Ctrl Pts',(55.0225511871177,30.9946799161412,7.00996533682697));
#44002=CARTESIAN_POINT('Ctrl Pts',(55.0376810669348,30.9944514635071,7.00899085906464));
#44003=CARTESIAN_POINT('Ctrl Pts',(55.1131586459729,30.9924526628192,7.00410144985794));
#44004=CARTESIAN_POINT('Ctrl Pts',(55.1734011806347,30.9881155033851,7.00010792318171));
#44005=CARTESIAN_POINT('Ctrl Pts',(55.3675792227355,30.9652431624853,6.986934621165));
#44006=CARTESIAN_POINT('Ctrl Pts',(55.4998431342191,30.9358316927362,6.97746544346421));
#44007=CARTESIAN_POINT('Ctrl Pts',(55.7062664672906,30.8673505024225,6.96235172744517));
#44008=CARTESIAN_POINT('Ctrl Pts',(55.7827615925344,30.836599386846,6.95668043012796));
#44009=CARTESIAN_POINT('Ctrl Pts',(55.8714098643384,30.7944141247573,6.95018158837856));
#44010=CARTESIAN_POINT('Ctrl Pts',(55.8855962028438,30.7874553436784,6.94914402786589));
#44011=CARTESIAN_POINT('Ctrl Pts',(55.9053042238755,30.7774957858713,6.94770757929789));
#44012=CARTESIAN_POINT('Ctrl Pts',(55.9108962525276,30.7746365899119,6.94730055997782));
#44013=CARTESIAN_POINT('Ctrl Pts',(55.9204008384593,30.7697201466181,6.94660984463038));
#44014=CARTESIAN_POINT('Ctrl Pts',(55.9243202063734,30.7676762311936,6.94632533319063));
#44015=CARTESIAN_POINT('Ctrl Pts',(55.9318568602372,30.7637140125621,6.94577889113273));
#44016=CARTESIAN_POINT('Ctrl Pts',(55.93547505671,30.7617975891357,6.94551684164791));
#44017=CARTESIAN_POINT('Ctrl Pts',(55.9441614424461,30.7571624314138,6.94488835405222));
#44018=CARTESIAN_POINT('Ctrl Pts',(55.9492238595146,30.7544328731092,6.94452258801589));
#44019=CARTESIAN_POINT('Ctrl Pts',(55.9677183692727,30.7443575030099,6.94318796783252));
#44020=CARTESIAN_POINT('Ctrl Pts',(55.9810779828172,30.7368787998858,6.94222706134827));
#44021=CARTESIAN_POINT('Ctrl Pts',(56.1083569115992,30.663690931769,6.93308997531943));
#44022=CARTESIAN_POINT('Ctrl Pts',(56.2156177171251,30.5870116565507,6.92551234873589));
#44023=CARTESIAN_POINT('Ctrl Pts',(56.4211406734027,30.4069353376887,6.90964278370779));
#44024=CARTESIAN_POINT('Ctrl Pts',(56.5174530236151,30.3024734430475,6.90136967346551));
#44025=CARTESIAN_POINT('Ctrl Pts',(56.6127308057256,30.1740776597263,6.89145565248301));
#44026=CARTESIAN_POINT('Ctrl Pts',(56.6233787556746,30.1593103054675,6.89031947132378));
#44027=CARTESIAN_POINT('Ctrl Pts',(56.6392321840964,30.1366768721068,6.88858314369568));
#44028=CARTESIAN_POINT('Ctrl Pts',(56.6445866469688,30.1289159493428,6.887988651114));
#44029=CARTESIAN_POINT('Ctrl Pts',(56.6537866053956,30.1153768855018,6.88695294028633));
#44030=CARTESIAN_POINT('Ctrl Pts',(56.6576573693912,30.1096160491915,6.88651268054141));
#44031=CARTESIAN_POINT('Ctrl Pts',(56.6662601879818,30.0966670459226,6.88552398070469));
#44032=CARTESIAN_POINT('Ctrl Pts',(56.6709759251847,30.0894682543865,6.88497494449933));
#44033=CARTESIAN_POINT('Ctrl Pts',(56.6834341105488,30.070179086908,6.88350530738382));
#44034=CARTESIAN_POINT('Ctrl Pts',(56.6910927470488,30.0580354368958,6.88258164662552));
#44035=CARTESIAN_POINT('Ctrl Pts',(56.7246688569936,30.0035006642109,6.87843977580195));
#44036=CARTESIAN_POINT('Ctrl Pts',(56.7491262761213,29.960235805642,6.87516951345243));
#44037=CARTESIAN_POINT('Ctrl Pts',(56.8481780066025,29.7686489562313,6.86074505841113));
#44038=CARTESIAN_POINT('Ctrl Pts',(56.9057021868245,29.6122640174991,6.84904229574597));
#44039=CARTESIAN_POINT('Ctrl Pts',(56.9543695819128,29.4023884520922,6.83414968234723));
#44040=CARTESIAN_POINT('Ctrl Pts',(56.9637519261193,29.3537738779263,6.83076027603962));
#44041=CARTESIAN_POINT('Ctrl Pts',(56.974106951383,29.2868146491723,6.82621386184849));
#44042=CARTESIAN_POINT('Ctrl Pts',(56.9766495052811,29.2687334788619,6.82499828192145));
#44043=CARTESIAN_POINT('Ctrl Pts',(56.980601837733,29.2375250145556,6.82292378136598));
#44044=CARTESIAN_POINT('Ctrl Pts',(56.9821301835058,29.2244141930124,6.8220594249982));
#44045=CARTESIAN_POINT('Ctrl Pts',(56.9841472007655,29.2054789172412,6.82082230342152));
#44046=CARTESIAN_POINT('Ctrl Pts',(56.9847405551354,29.19966629815,6.82044406323201));
#44047=CARTESIAN_POINT('Ctrl Pts',(56.9857308288667,29.1895244983226,6.81978686603181));
#44048=CARTESIAN_POINT('Ctrl Pts',(56.986139147815,29.1851965095376,6.81950728463812));
#44049=CARTESIAN_POINT('Ctrl Pts',(56.9869721599372,29.1760472153623,6.81891813525641));
#44050=CARTESIAN_POINT('Ctrl Pts',(56.9873934569634,29.1712256838819,6.81860875620718));
#44051=CARTESIAN_POINT('Ctrl Pts',(56.9884835087576,29.1582042416448,6.8177760561605));
#44052=CARTESIAN_POINT('Ctrl Pts',(56.9891190988931,29.1500015421842,6.81725454059352));
#44053=CARTESIAN_POINT('Ctrl Pts',(56.9917820281599,29.112634627375,6.81489166073638));
#44054=CARTESIAN_POINT('Ctrl Pts',(56.9932189540587,29.0834303143754,6.81308055506658));
#44055=CARTESIAN_POINT('Ctrl Pts',(56.9996543405425,28.8466870950551,6.79861136150138));
#44056=CARTESIAN_POINT('Ctrl Pts',(56.9728702123683,28.6395451713328,6.78714507927761));
#44057=CARTESIAN_POINT('Ctrl Pts',(56.9044040008753,28.40536269987,6.77249410984721));
#44058=CARTESIAN_POINT('Ctrl Pts',(56.8932558565437,28.3707701931234,6.77028858205908));
#44059=CARTESIAN_POINT('Ctrl Pts',(56.8725324854121,28.3120145856584,6.76645736062212));
#44060=CARTESIAN_POINT('Ctrl Pts',(56.8634183361255,28.2876982047568,6.76484623770607));
#44061=CARTESIAN_POINT('Ctrl Pts',(56.8498215855671,28.2534709032816,6.76253883412008));
#44062=CARTESIAN_POINT('Ctrl Pts',(56.8457283747993,28.2434074083732,6.76185549228548));
#44063=CARTESIAN_POINT('Ctrl Pts',(56.838528337522,28.2261117241772,6.76067232564928));
#44064=CARTESIAN_POINT('Ctrl Pts',(56.8354605051779,28.2188634931173,6.76017381913831));
#44065=CARTESIAN_POINT('Ctrl Pts',(56.8295024193571,28.2050154915147,6.75921619845525));
#44066=CARTESIAN_POINT('Ctrl Pts',(56.8266191429162,28.1984128396296,6.75875732664263));
#44067=CARTESIAN_POINT('Ctrl Pts',(56.8197638112604,28.1829433120279,6.75767677880472));
#44068=CARTESIAN_POINT('Ctrl Pts',(56.8157626454658,28.1740896114181,6.75705412016706));
#44069=CARTESIAN_POINT('Ctrl Pts',(56.8017069252029,28.1435832526029,6.75489380837529));
#44070=CARTESIAN_POINT('Ctrl Pts',(56.7913287749436,28.1220827897258,6.75334515240792));
#44071=CARTESIAN_POINT('Ctrl Pts',(56.7133041106098,27.9675851788973,6.74202157441482));
#44072=CARTESIAN_POINT('Ctrl Pts',(56.6313208987502,27.8423870618857,6.7317305961901));
#44073=CARTESIAN_POINT('Ctrl Pts',(56.4809338588952,27.6608359609217,6.71530008681886));
#44074=CARTESIAN_POINT('Ctrl Pts',(56.4214103009037,27.5978160551205,6.70925951483155));
#44075=CARTESIAN_POINT('Ctrl Pts',(56.3390668555281,27.5212863780906,6.70163879669598));
#44076=CARTESIAN_POINT('Ctrl Pts',(56.3198166237046,27.5040794709588,6.69990486726887));
#44077=CARTESIAN_POINT('Ctrl Pts',(56.2872115889623,27.4760548288016,6.69705347394267));
#44078=CARTESIAN_POINT('Ctrl Pts',(56.2740417133189,27.4650275833835,6.69592406751638));
#44079=CARTESIAN_POINT('Ctrl Pts',(56.2557003702374,27.4500689450035,6.69438353311118));
#44080=CARTESIAN_POINT('Ctrl Pts',(56.2506501316,27.4459910083239,6.69396266981006));
#44081=CARTESIAN_POINT('Ctrl Pts',(56.2420955459322,27.4391521155836,6.69325547774728));
#44082=CARTESIAN_POINT('Ctrl Pts',(56.2386017082338,27.4363781553091,6.69296824014254));
#44083=CARTESIAN_POINT('Ctrl Pts',(56.2319195618294,27.4311092629728,6.69242195769294));
#44084=CARTESIAN_POINT('Ctrl Pts',(56.2287329323647,27.4286122906235,6.69216276346233));
#44085=CARTESIAN_POINT('Ctrl Pts',(56.2211388849498,27.4226989881247,6.69154815191224));
#44086=CARTESIAN_POINT('Ctrl Pts',(56.2167246711969,27.4192913821079,6.69119334179756));
#44087=CARTESIAN_POINT('Ctrl Pts',(56.2010705451695,27.4073114160271,6.6899434699723));
#44088=CARTESIAN_POINT('Ctrl Pts',(56.1897535536857,27.3988398306306,6.68905509160309));
#44089=CARTESIAN_POINT('Ctrl Pts',(56.059888633158,27.3037637795336,6.67902040280405));
#44090=CARTESIAN_POINT('Ctrl Pts',(55.9321994263362,27.2303676634608,6.67063153464379));
#44091=CARTESIAN_POINT('Ctrl Pts',(55.6807491561,27.1206759602873,6.65467690049963));
#44092=CARTESIAN_POINT('Ctrl Pts',(55.5593044436243,27.0810287404708,6.64718276321157));
#44093=CARTESIAN_POINT('Ctrl Pts',(55.4168149917384,27.0491958472848,6.63813325306116));
#44094=CARTESIAN_POINT('Ctrl Pts',(55.398658487695,27.0454046572768,6.63697605028504));
#44095=CARTESIAN_POINT('Ctrl Pts',(55.3711278638344,27.0400556393345,6.63521411288293));
#44096=CARTESIAN_POINT('Ctrl Pts',(55.3617908190403,27.0383106294631,6.63461529348404));
#44097=CARTESIAN_POINT('Ctrl Pts',(55.3449491322474,27.0352873981992,6.63353276276496));
#44098=CARTESIAN_POINT('Ctrl Pts',(55.3374489177741,27.0339853162307,6.63304981430279));
#44099=CARTESIAN_POINT('Ctrl Pts',(55.3212791127767,27.0312733957904,6.63200669104536));
#44100=CARTESIAN_POINT('Ctrl Pts',(55.3126073227887,27.0298778291378,6.63144607774987));
#44101=CARTESIAN_POINT('Ctrl Pts',(55.2893172418508,27.0262873549437,6.62993709247676));
#44102=CARTESIAN_POINT('Ctrl Pts',(55.2746835239841,27.0241976278128,6.62898544564365));
#44103=CARTESIAN_POINT('Ctrl Pts',(55.2047553091895,27.0150035929815,6.62442027344402));
#44104=CARTESIAN_POINT('Ctrl Pts',(55.149206999144,27.0100573528435,6.62074028525787));
#44105=CARTESIAN_POINT('Ctrl Pts',(54.9146910730861,26.99904939898,6.60497061139637));
#44106=CARTESIAN_POINT('Ctrl Pts',(54.7355440877852,27.0147725812098,6.5922589316747));
#44107=CARTESIAN_POINT('Ctrl Pts',(54.5258768057124,27.0620817668024,6.57753820012826));
#44108=CARTESIAN_POINT('Ctrl Pts',(54.4910277200637,27.0709413159193,6.57510076611379));
#44109=CARTESIAN_POINT('Ctrl Pts',(54.4353829054125,27.0867007949842,6.57124283574848));
#44110=CARTESIAN_POINT('Ctrl Pts',(54.4144290665264,27.0930094158185,6.56979799425634));
#44111=CARTESIAN_POINT('Ctrl Pts',(54.3867985654778,27.1018265969667,6.56790710563729));
#44112=CARTESIAN_POINT('Ctrl Pts',(54.3800263772893,27.1040276958445,6.56744480404991));
#44113=CARTESIAN_POINT('Ctrl Pts',(54.3689039336888,27.1077086827692,6.56668759855882));
#44114=CARTESIAN_POINT('Ctrl Pts',(54.3645468159209,27.1091673987202,6.56639149360175));
#44115=CARTESIAN_POINT('Ctrl Pts',(54.3560163822983,27.1120561122691,6.56581285577817));
#44116=CARTESIAN_POINT('Ctrl Pts',(54.3518427176803,27.1134849162966,6.56553025937061));
#44117=CARTESIAN_POINT('Ctrl Pts',(54.3415653843125,27.1170413705552,6.56483557374667));
#44118=CARTESIAN_POINT('Ctrl Pts',(54.3354671844149,27.1191848886424,6.56442440636526));
#44119=CARTESIAN_POINT('Ctrl Pts',(54.314496113848,27.1266709514708,6.56301366317416));
#44120=CARTESIAN_POINT('Ctrl Pts',(54.2996759327407,27.1321607297954,6.56202228923762));
#44121=CARTESIAN_POINT('Ctrl Pts',(54.1720451895023,27.1811711584973,6.55352039242769));
#44122=CARTESIAN_POINT('Ctrl Pts',(54.063327025177,27.2346957053981,6.54651190223482));
#44123=CARTESIAN_POINT('Ctrl Pts',(53.8708239805844,27.3522932707182,6.53341235394136));
#44124=CARTESIAN_POINT('Ctrl Pts',(53.7859665094858,27.413779142495,6.52734426949235));
#44125=CARTESIAN_POINT('Ctrl Pts',(53.6791750329981,27.5047670868791,6.51891364981743));
#44126=CARTESIAN_POINT('Ctrl Pts',(53.6526488358274,27.5286249014816,6.51674734085933));
#44127=CARTESIAN_POINT('Ctrl Pts',(53.6082091154794,27.5708040411168,6.51297830404808));
#44128=CARTESIAN_POINT('Ctrl Pts',(53.5899823112836,27.5887831562152,6.51138950481195));
#44129=CARTESIAN_POINT('Ctrl Pts',(53.5645635303534,27.6148406542357,6.5091086013084));
#44130=CARTESIAN_POINT('Ctrl Pts',(53.5570829504477,27.6226348877839,6.50842902766213));
#44131=CARTESIAN_POINT('Ctrl Pts',(53.5442698853305,27.6362041303912,6.50725031140425));
#44132=CARTESIAN_POINT('Ctrl Pts',(53.5389074911014,27.6419506568999,6.50675246029609));
#44133=CARTESIAN_POINT('Ctrl Pts',(53.5286861607864,27.6530348012645,6.50579463984382));
#44134=CARTESIAN_POINT('Ctrl Pts',(53.5238219501723,27.6583674038567,6.50533490447229));
#44135=CARTESIAN_POINT('Ctrl Pts',(53.5124429684654,27.6709789076192,6.50425008333531));
#44136=CARTESIAN_POINT('Ctrl Pts',(53.5059525585768,27.6782794458543,6.50362399551756));
#44137=CARTESIAN_POINT('Ctrl Pts',(53.4835241172738,27.7038836853224,6.50143452880689));
#44138=CARTESIAN_POINT('Ctrl Pts',(53.467867241644,27.7224297556653,6.49985972978617));
#44139=CARTESIAN_POINT('Ctrl Pts',(53.3650790563348,27.848793239632,6.48919891931733));
#44140=CARTESIAN_POINT('Ctrl Pts',(53.289067911369,27.965136695496,6.47967469045432));
#44141=CARTESIAN_POINT('Ctrl Pts',(53.1690536038691,28.1987210393171,6.46138297595814));
#44142=CARTESIAN_POINT('Ctrl Pts',(53.1227776159862,28.3141034162764,6.45269090205674));
#44143=CARTESIAN_POINT('Ctrl Pts',(53.083052374847,28.4481067578686,6.44343585836962));
#44144=CARTESIAN_POINT('Ctrl Pts',(53.0787653008339,28.4632210738082,6.44240385757877));
#44145=CARTESIAN_POINT('Ctrl Pts',(53.0729709180718,28.4846088291476,6.44096171638683));
#44146=CARTESIAN_POINT('Ctrl Pts',(53.0713149170892,28.4908408939069,6.44054366647915));
#44147=CARTESIAN_POINT('Ctrl Pts',(53.0685777118761,28.5013468735339,6.43984269259501));
#44148=CARTESIAN_POINT('Ctrl Pts',(53.0674804124074,28.5056165046767,6.43955886279768));
#44149=CARTESIAN_POINT('Ctrl Pts',(53.0652672786344,28.5143478504738,6.43898061770297));
#44150=CARTESIAN_POINT('Ctrl Pts',(53.0641527067173,28.5188098384322,6.43868627486099));
#44151=CARTESIAN_POINT('Ctrl Pts',(53.061347076103,28.5302092073647,6.43793715635705));
#44152=CARTESIAN_POINT('Ctrl Pts',(53.0596777996614,28.537151957181,6.43748360727462));
#44153=CARTESIAN_POINT('Ctrl Pts',(53.053007619738,28.5655645201198,6.43563795798104));
#44154=CARTESIAN_POINT('Ctrl Pts',(53.0483252804419,28.5871084901867,6.43426283870236));
#44155=CARTESIAN_POINT('Ctrl Pts',(53.0368751957249,28.6443481625649,6.43066292646322));
#44156=CARTESIAN_POINT('Ctrl Pts',(53.0307235389978,28.680159792689,6.42846540700149));
#44157=CARTESIAN_POINT('Ctrl Pts',(52.9991521478969,28.8997467933963,6.41521590284308));
#44158=CARTESIAN_POINT('Ctrl Pts',(52.9984936833413,29.0861583468699,6.40483632778336));
#44159=CARTESIAN_POINT('Ctrl Pts',(53.0297639748385,29.315068056609,6.39092058868415));
#44160=CARTESIAN_POINT('Ctrl Pts',(53.0374625283022,29.359921990805,6.38814216583772));
#44161=CARTESIAN_POINT('Ctrl Pts',(53.046686998162,29.404469874466,6.38531629657044));
#44162=CARTESIAN_POINT('Ctrl Pts',(53.0466869743493,29.404469759467,6.22571516850575));
#44163=CARTESIAN_POINT('Ctrl Pts',(53.0336901222297,29.3417038296453,6.22943746026231));
#44164=CARTESIAN_POINT('Ctrl Pts',(53.0237206966933,29.2783219142394,6.23315573173925));
#44165=CARTESIAN_POINT('Ctrl Pts',(53.0091361594068,29.1435060238327,6.24113115979555));
#44166=CARTESIAN_POINT('Ctrl Pts',(53.0052742093992,29.072113868334,6.24539418151947));
#44167=CARTESIAN_POINT('Ctrl Pts',(53.0052401907627,28.9712533874548,6.25157249376068));
#44168=CARTESIAN_POINT('Ctrl Pts',(53.0058811019398,28.9418386165462,6.25339263738129));
#44169=CARTESIAN_POINT('Ctrl Pts',(53.0076881732792,28.9007058025391,6.25596817345258));
#44170=CARTESIAN_POINT('Ctrl Pts',(53.0083079180278,28.888966699742,6.25670666770735));
#44171=CARTESIAN_POINT('Ctrl Pts',(53.0094768959908,28.8700087014318,6.2579051428035));
#44172=CARTESIAN_POINT('Ctrl Pts',(53.0099617385099,28.8627860033684,6.25836311565912));
#44173=CARTESIAN_POINT('Ctrl Pts',(53.0110536867358,28.8477448833479,6.25931976776433));
#44174=CARTESIAN_POINT('Ctrl Pts',(53.0116676032664,28.8399270952741,6.25981865120777));
#44175=CARTESIAN_POINT('Ctrl Pts',(53.0132285217316,28.821446816068,6.26100195342078));
#44176=CARTESIAN_POINT('Ctrl Pts',(53.0142152779156,28.8107880116351,6.26168759915631));
#44177=CARTESIAN_POINT('Ctrl Pts',(53.0177945044293,28.7752448430209,6.26398479840446));
#44178=CARTESIAN_POINT('Ctrl Pts',(53.0207692523406,28.7504022015754,6.26560817886421));
#44179=CARTESIAN_POINT('Ctrl Pts',(53.0289725192607,28.691330454617,6.26951243235895));
#44180=CARTESIAN_POINT('Ctrl Pts',(53.0346264314697,28.6571695517108,6.2718058569667));
#44181=CARTESIAN_POINT('Ctrl Pts',(53.0752693345346,28.4458973920729,6.28621316955182));
#44182=CARTESIAN_POINT('Ctrl Pts',(53.133280930704,28.2740800025001,6.29901819537356));
#44183=CARTESIAN_POINT('Ctrl Pts',(53.2243692819676,28.090741645815,6.31306635217036));
#44184=CARTESIAN_POINT('Ctrl Pts',(53.2355504837523,28.0692297870817,6.31471932230543));
#44185=CARTESIAN_POINT('Ctrl Pts',(53.2634356470972,28.0178899494942,6.3186671259085));
#44186=CARTESIAN_POINT('Ctrl Pts',(53.2805204130662,27.9882756386985,6.32094673851372));
#44187=CARTESIAN_POINT('Ctrl Pts',(53.3028412190259,27.9517856055767,6.32374532525463));
#44188=CARTESIAN_POINT('Ctrl Pts',(53.3073707900135,27.9444869927895,6.32430455731323));
#44189=CARTESIAN_POINT('Ctrl Pts',(53.3145953143114,27.9330120400183,6.32518266545636));
#44190=CARTESIAN_POINT('Ctrl Pts',(53.3172589089077,27.9288162235464,6.32550350674239));
#44191=CARTESIAN_POINT('Ctrl Pts',(53.3220330038915,27.9213576025441,6.32607335621864));
#44192=CARTESIAN_POINT('Ctrl Pts',(53.3241373443133,27.9180910291148,6.32632275351748));
#44193=CARTESIAN_POINT('Ctrl Pts',(53.3291782237629,27.9103160540121,6.32691596757327));
#44194=CARTESIAN_POINT('Ctrl Pts',(53.3321234678105,27.9058133682551,6.32725920378033));
#44195=CARTESIAN_POINT('Ctrl Pts',(53.3410177735145,27.8923351210008,6.32828588559477));
#44196=CARTESIAN_POINT('Ctrl Pts',(53.3470214437224,27.8833955863511,6.32896582955401));
#44197=CARTESIAN_POINT('Ctrl Pts',(53.3610311003458,27.8628956838051,6.3305238017073));
#44198=CARTESIAN_POINT('Ctrl Pts',(53.3690876061914,27.8513703522526,6.33139878101936));
#44199=CARTESIAN_POINT('Ctrl Pts',(53.3968322141058,27.8125604845479,6.33434548800326));
#44200=CARTESIAN_POINT('Ctrl Pts',(53.4170893469668,27.7856879837985,6.33638644313321));
#44201=CARTESIAN_POINT('Ctrl Pts',(53.5302674964805,27.6431975546764,6.34728779310529));
#44202=CARTESIAN_POINT('Ctrl Pts',(53.6351869745191,27.5377012268036,6.35568207480793));
#44203=CARTESIAN_POINT('Ctrl Pts',(53.8183510966638,27.3905802756177,6.36952581144618));
#44204=CARTESIAN_POINT('Ctrl Pts',(53.8893146491604,27.3408130549455,6.37472402115603));
#44205=CARTESIAN_POINT('Ctrl Pts',(53.9762306293578,27.2879387888947,6.38104279747824));
#44206=CARTESIAN_POINT('Ctrl Pts',(53.9892693566838,27.2802090645124,6.38198933575541));
#44207=CARTESIAN_POINT('Ctrl Pts',(54.0107709902327,27.2677912671264,6.3835486516898));
#44208=CARTESIAN_POINT('Ctrl Pts',(54.0191823013398,27.2630147482695,6.38415825476024));
#44209=CARTESIAN_POINT('Ctrl Pts',(54.034349284701,27.2545471886746,6.38525692870694));
#44210=CARTESIAN_POINT('Ctrl Pts',(54.0410922535662,27.2508336981141,6.38574518916298));
#44211=CARTESIAN_POINT('Ctrl Pts',(54.0554930300929,27.2430111922066,6.38678763444405));
#44212=CARTESIAN_POINT('Ctrl Pts',(54.0631565136887,27.2389130160173,6.38734218921769));
#44213=CARTESIAN_POINT('Ctrl Pts',(54.0838904190425,27.2279988461721,6.388842185226));
#44214=CARTESIAN_POINT('Ctrl Pts',(54.0970098150319,27.2212775483199,6.38979091117769));
#44215=CARTESIAN_POINT('Ctrl Pts',(54.165042768132,27.1873697160483,6.39470965361494));
#44216=CARTESIAN_POINT('Ctrl Pts',(54.2211081346196,27.1625810875899,6.39876116265078));
#44217=CARTESIAN_POINT('Ctrl Pts',(54.3448144893781,27.114565736296,6.40770094927617));
#44218=CARTESIAN_POINT('Ctrl Pts',(54.412743493521,27.0923158754541,6.41261078646231));
#44219=CARTESIAN_POINT('Ctrl Pts',(54.6180500092199,27.0370749243969,6.42736632752475));
#44220=CARTESIAN_POINT('Ctrl Pts',(54.757900397643,27.0149678441298,6.43733362084736));
#44221=CARTESIAN_POINT('Ctrl Pts',(54.9181090272729,27.0068390296775,6.44800528327447));
#44222=CARTESIAN_POINT('Ctrl Pts',(54.9373134339272,27.0061426217843,6.44927185161378));
#44223=CARTESIAN_POINT('Ctrl Pts',(54.9635286872229,27.0055711417654,6.45098088704421));
#44224=CARTESIAN_POINT('Ctrl Pts',(54.9705325264032,27.0054553655684,6.451435545384));
#44225=CARTESIAN_POINT('Ctrl Pts',(54.9816518348254,27.005330142174,6.45215413122779));
#44226=CARTESIAN_POINT('Ctrl Pts',(54.9857668937531,27.0052965342396,6.45241936480779));
#44227=CARTESIAN_POINT('Ctrl Pts',(54.9942873414668,27.0052533155991,6.45296705008526));
#44228=CARTESIAN_POINT('Ctrl Pts',(54.9986926798279,27.005245563818,6.4532493870948));
#44229=CARTESIAN_POINT('Ctrl Pts',(55.0092967199724,27.0052620329449,6.4539270605146));
#44230=CARTESIAN_POINT('Ctrl Pts',(55.0154954191258,27.0053005538056,6.45432161041427));
#44231=CARTESIAN_POINT('Ctrl Pts',(55.0369815114805,27.0055342399769,6.45568400494136));
#44232=CARTESIAN_POINT('Ctrl Pts',(55.052267216231,27.0058762647386,6.4566441109457));
#44233=CARTESIAN_POINT('Ctrl Pts',(55.1444800393686,27.0090006500764,6.46238903726044));
#44234=CARTESIAN_POINT('Ctrl Pts',(55.221205637902,27.0160585720634,6.46697268475538));
#44235=CARTESIAN_POINT('Ctrl Pts',(55.3792091456557,27.0398767729622,6.47634488833364));
#44236=CARTESIAN_POINT('Ctrl Pts',(55.4602327391628,27.0573037005231,6.48111504270365));
#44237=CARTESIAN_POINT('Ctrl Pts',(55.6505259559454,27.110809784941,6.49264468816447));
#44238=CARTESIAN_POINT('Ctrl Pts',(55.7582044071864,27.1513938703551,6.49944658264577));
#44239=CARTESIAN_POINT('Ctrl Pts',(55.8760362879693,27.2078399365926,6.50755440069076));
#44240=CARTESIAN_POINT('Ctrl Pts',(55.8902056804436,27.2148358352977,6.50854053970448));
#44241=CARTESIAN_POINT('Ctrl Pts',(55.9130852470149,27.2264723691894,6.51015186086307));
#44242=CARTESIAN_POINT('Ctrl Pts',(55.9218469023253,27.2310106815912,6.51077349420613));
#44243=CARTESIAN_POINT('Ctrl Pts',(55.9374011886622,27.2392143392031,6.51188542827417));
#44244=CARTESIAN_POINT('Ctrl Pts',(55.9442069415694,27.2428544794047,6.51237483718683));
#44245=CARTESIAN_POINT('Ctrl Pts',(55.9585281550571,27.2506215815933,6.51341088182645));
#44246=CARTESIAN_POINT('Ctrl Pts',(55.9660384582823,27.2547576763717,6.51395783337311));
#44247=CARTESIAN_POINT('Ctrl Pts',(55.9859260457451,27.2658779259029,6.51541599451997));
#44248=CARTESIAN_POINT('Ctrl Pts',(55.9982555728153,27.2729460547913,6.51633018055453));
#44249=CARTESIAN_POINT('Ctrl Pts',(56.0574299104708,27.3077141971115,6.52076804559156));
#44250=CARTESIAN_POINT('Ctrl Pts',(56.103199555955,27.3371894108576,6.52435528352325));
#44251=CARTESIAN_POINT('Ctrl Pts',(56.3114313654878,27.4836729576747,6.54142850658865));
#44252=CARTESIAN_POINT('Ctrl Pts',(56.4568553056925,27.6228105563532,6.55574145577927));
#44253=CARTESIAN_POINT('Ctrl Pts',(56.6012530662405,27.8099044842397,6.57173883429098));
#44254=CARTESIAN_POINT('Ctrl Pts',(56.6225937968314,27.8391690579339,6.57415711984861));
#44255=CARTESIAN_POINT('Ctrl Pts',(56.6480926761642,27.8762140847911,6.57710046516448));
#44256=CARTESIAN_POINT('Ctrl Pts',(56.6530105022833,27.8834604626198,6.57767076282761));
#44257=CARTESIAN_POINT('Ctrl Pts',(56.6606657595944,27.8949018672549,6.5785623895592));
#44258=CARTESIAN_POINT('Ctrl Pts',(56.6634353148235,27.8990751148173,6.57888578207171));
#44259=CARTESIAN_POINT('Ctrl Pts',(56.6685379694145,27.9068271604192,6.57948305767277));
#44260=CARTESIAN_POINT('Ctrl Pts',(56.6708752733194,27.9104029946448,6.57975721022623));
#44261=CARTESIAN_POINT('Ctrl Pts',(56.6762128051163,27.9186264316481,6.58038461014332));
#44262=CARTESIAN_POINT('Ctrl Pts',(56.6792051985231,27.923279021575,6.58073734038845));
#44263=CARTESIAN_POINT('Ctrl Pts',(56.6883766432639,27.9376700662044,6.58182169911222));
#44264=CARTESIAN_POINT('Ctrl Pts',(56.6944907501909,27.947449910898,6.58254921859051));
#44265=CARTESIAN_POINT('Ctrl Pts',(56.7519559624721,28.0411672745306,6.58943732700102));
#44266=CARTESIAN_POINT('Ctrl Pts',(56.797121982662,28.1287550716496,6.59524408254966));
#44267=CARTESIAN_POINT('Ctrl Pts',(56.9040063245006,28.3800793837888,6.61117384762291));
#44268=CARTESIAN_POINT('Ctrl Pts',(56.9509534610614,28.5490931830108,6.62115320792036));
#44269=CARTESIAN_POINT('Ctrl Pts',(56.978373532884,28.7439627197549,6.63330215089091));
#44270=CARTESIAN_POINT('Ctrl Pts',(56.9810911758399,28.7659174992277,6.6346784437214));
#44271=CARTESIAN_POINT('Ctrl Pts',(56.984514997263,28.7979370559507,6.63669854124829));
#44272=CARTESIAN_POINT('Ctrl Pts',(56.9855109046531,28.8079696657671,6.63733332205234));
#44273=CARTESIAN_POINT('Ctrl Pts',(56.9871395849604,28.8257467261469,6.63846152450768));
#44274=CARTESIAN_POINT('Ctrl Pts',(56.9878032466555,28.8334881884625,6.63895397332591));
#44275=CARTESIAN_POINT('Ctrl Pts',(56.9890889809182,28.8495909413031,6.6399807647622));
#44276=CARTESIAN_POINT('Ctrl Pts',(56.9897035980167,28.8579526576323,6.64051532953499));
#44277=CARTESIAN_POINT('Ctrl Pts',(56.9911601016814,28.8796371531007,6.64190531428085));
#44278=CARTESIAN_POINT('Ctrl Pts',(56.991920985548,28.8929647791707,6.64276323400183));
#44279=CARTESIAN_POINT('Ctrl Pts',(56.9946643199461,28.9513015365321,6.64653491343137));
#44280=CARTESIAN_POINT('Ctrl Pts',(56.9952552468688,28.9963598002743,6.64949133035863));
#44281=CARTESIAN_POINT('Ctrl Pts',(56.9910417829105,29.1993473372872,6.66301427174421));
#44282=CARTESIAN_POINT('Ctrl Pts',(56.9690099202627,29.3563315039657,6.6740911748947));
#44283=CARTESIAN_POINT('Ctrl Pts',(56.9067302801766,29.5923028271303,6.69103666399445));
#44284=CARTESIAN_POINT('Ctrl Pts',(56.8793837843771,29.674064587153,6.69695138826517));
#44285=CARTESIAN_POINT('Ctrl Pts',(56.8428254438862,29.763632426481,6.70330529757384));
#44286=CARTESIAN_POINT('Ctrl Pts',(56.8387381881853,29.7734222562692,6.70399799250553));
#44287=CARTESIAN_POINT('Ctrl Pts',(56.8324454655494,29.7881627621189,6.70503776256106));
#44288=CARTESIAN_POINT('Ctrl Pts',(56.8302976830356,29.7931376406076,6.7053881243559));
#44289=CARTESIAN_POINT('Ctrl Pts',(56.8264079499274,29.8020474297157,6.70601452433708));
#44290=CARTESIAN_POINT('Ctrl Pts',(56.8246735213666,29.8059854965059,6.70629100226585));
#44291=CARTESIAN_POINT('Ctrl Pts',(56.8208517407689,29.8145873846591,6.70689405891063));
#44292=CARTESIAN_POINT('Ctrl Pts',(56.8187592114624,29.8192488030073,6.70722031972455));
#44293=CARTESIAN_POINT('Ctrl Pts',(56.8127397660176,29.8325212742388,6.70814788497766));
#44294=CARTESIAN_POINT('Ctrl Pts',(56.8087693841898,29.8411126289198,6.70874661917851));
#44295=CARTESIAN_POINT('Ctrl Pts',(56.7815584908717,29.8989094291282,6.71276524014978));
#44296=CARTESIAN_POINT('Ctrl Pts',(56.7563717584758,29.9471790880372,6.71607614452245));
#44297=CARTESIAN_POINT('Ctrl Pts',(56.6344233711701,30.1592526604831,6.73068278461686));
#44298=CARTESIAN_POINT('Ctrl Pts',(56.5165120352766,30.3097350899645,6.74131215017533));
#44299=CARTESIAN_POINT('Ctrl Pts',(56.3461242070602,30.4727715520555,6.75556125943586));
#44300=CARTESIAN_POINT('Ctrl Pts',(56.3121122501544,30.5031524818635,6.75835542897464));
#44301=CARTESIAN_POINT('Ctrl Pts',(56.2663969944422,30.5412527437503,6.7620658617992));
#44302=CARTESIAN_POINT('Ctrl Pts',(56.2556099790925,30.55005320315,6.76293820456724));
#44303=CARTESIAN_POINT('Ctrl Pts',(56.2380819762654,30.564050192361,6.76435109078169));
#44304=CARTESIAN_POINT('Ctrl Pts',(56.2313981797162,30.5693178465673,6.76488879553809));
#44305=CARTESIAN_POINT('Ctrl Pts',(56.2185771156468,30.5792900848745,6.76591833771115));
#44306=CARTESIAN_POINT('Ctrl Pts',(56.2124457847171,30.5840020755474,6.76640987093001));
#44307=CARTESIAN_POINT('Ctrl Pts',(56.1983330162123,30.5947179352342,6.76753947817042));
#44308=CARTESIAN_POINT('Ctrl Pts',(56.1903336261087,30.6006977114044,6.76817847355913));
#44309=CARTESIAN_POINT('Ctrl Pts',(56.1653516279314,30.6190816572252,6.77017029180876));
#44310=CARTESIAN_POINT('Ctrl Pts',(56.1482179736392,30.6312771863464,6.7715310438189));
#44311=CARTESIAN_POINT('Ctrl Pts',(56.0640636579724,30.6891945196858,6.77819131024342));
#44312=CARTESIAN_POINT('Ctrl Pts',(55.9944967452248,30.7310640950781,6.78363114184655));
#44313=CARTESIAN_POINT('Ctrl Pts',(55.801591535736,30.831693386752,6.7985191654965));
#44314=CARTESIAN_POINT('Ctrl Pts',(55.6744542906723,30.8822214053855,6.80815217689868));
#44315=CARTESIAN_POINT('Ctrl Pts',(55.5320360987636,30.9225240756106,6.8183257263553));
#44316=CARTESIAN_POINT('Ctrl Pts',(55.5208841018493,30.925575496297,6.81911816925973));
#44317=CARTESIAN_POINT('Ctrl Pts',(55.4628424304527,30.9409157780111,6.8232188923695));
#44318=CARTESIAN_POINT('Ctrl Pts',(55.415538488929,30.9515905786893,6.82648150993546));
#44319=CARTESIAN_POINT('Ctrl Pts',(55.3593291942646,30.9621381031396,6.83023035843789));
#44320=CARTESIAN_POINT('Ctrl Pts',(55.3507591758218,30.963688216794,6.8307984460385));
#44321=CARTESIAN_POINT('Ctrl Pts',(55.3367971022441,30.9661193042327,6.83171799691199));
#44322=CARTESIAN_POINT('Ctrl Pts',(55.3314112030415,30.9670343217051,6.83207127512843));
#44323=CARTESIAN_POINT('Ctrl Pts',(55.3217735677498,30.9686309644259,6.8327007819814));
#44324=CARTESIAN_POINT('Ctrl Pts',(55.3175233312051,30.9693209586752,6.8329774698283));
#44325=CARTESIAN_POINT('Ctrl Pts',(55.3082589982,30.9707941814143,6.83357854502291));
#44326=CARTESIAN_POINT('Ctrl Pts',(55.3032441423801,30.971572039504,6.83390263036447));
#44327=CARTESIAN_POINT('Ctrl Pts',(55.2890288955388,30.9737214561414,6.83481780275453));
#44328=CARTESIAN_POINT('Ctrl Pts',(55.2798216588205,30.9750478313412,6.83540642634461));
#44329=CARTESIAN_POINT('Ctrl Pts',(55.2203339508917,30.9831931572662,6.83918479795891));
#44330=CARTESIAN_POINT('Ctrl Pts',(55.1698134780151,30.9881565565629,6.84227996578166));
#44331=CARTESIAN_POINT('Ctrl Pts',(54.966750373323,31.0003080106511,6.85446126597659));
#44332=CARTESIAN_POINT('Ctrl Pts',(54.8137969434966,30.9919016364594,6.86308890425721));
#44333=CARTESIAN_POINT('Ctrl Pts',(54.5824862533878,30.952288621832,6.87694815961842));
#44334=CARTESIAN_POINT('Ctrl Pts',(54.5026194798947,30.9334836030646,6.8818805200862));
#44335=CARTESIAN_POINT('Ctrl Pts',(54.4097991862446,30.9054959928171,6.88790341840874));
#44336=CARTESIAN_POINT('Ctrl Pts',(54.3955059477993,30.9010099686771,6.8888390728381));
#44337=CARTESIAN_POINT('Ctrl Pts',(54.3721205180139,30.8933798984495,6.89038405413735));
#44338=CARTESIAN_POINT('Ctrl Pts',(54.3629979777129,30.8903302627229,6.8909903056809));
#44339=CARTESIAN_POINT('Ctrl Pts',(54.3466200413766,30.8847231544339,6.89208530797283));
#44340=CARTESIAN_POINT('Ctrl Pts',(54.3393566644848,30.8821894484184,6.89257327074057));
#44341=CARTESIAN_POINT('Ctrl Pts',(54.323886810592,30.8766924743355,6.89361765400438));
#44342=CARTESIAN_POINT('Ctrl Pts',(54.3156847790155,30.8737172578816,6.8941744603741));
#44343=CARTESIAN_POINT('Ctrl Pts',(54.2941746965986,30.8657545872149,6.89564295050602));
#44344=CARTESIAN_POINT('Ctrl Pts',(54.280900158583,30.8606786233721,6.89655754911394));
#44345=CARTESIAN_POINT('Ctrl Pts',(54.2177373899727,30.8357493634029,6.90095025480894));
#44346=CARTESIAN_POINT('Ctrl Pts',(54.168614092384,30.8140306193279,6.90449006303857));
#44347=CARTESIAN_POINT('Ctrl Pts',(54.0255567801739,30.7437492284303,6.91517802983858));
#44348=CARTESIAN_POINT('Ctrl Pts',(53.9345484111306,30.689677269297,6.92249227999612));
#44349=CARTESIAN_POINT('Ctrl Pts',(53.7507624052646,30.5597092602233,6.93817652536704));
#44350=CARTESIAN_POINT('Ctrl Pts',(53.6596427874565,30.4821387353655,6.94653024156676));
#44351=CARTESIAN_POINT('Ctrl Pts',(53.5648989389195,30.3855554809716,6.95549097517508));
#44352=CARTESIAN_POINT('Ctrl Pts',(53.5539287606786,30.3741022723118,6.95653290946483));
#44353=CARTESIAN_POINT('Ctrl Pts',(53.5386745821129,30.357791399461,6.95798644782903));
#44354=CARTESIAN_POINT('Ctrl Pts',(53.5342761897338,30.3530421930721,6.95840612576579));
#44355=CARTESIAN_POINT('Ctrl Pts',(53.5269180424435,30.345019176266,6.95910903860495));
#44356=CARTESIAN_POINT('Ctrl Pts',(53.5239459195698,30.3417568300958,6.95939319040541));
#44357=CARTESIAN_POINT('Ctrl Pts',(53.5179032259121,30.3350796990789,6.95997132768147));
#44358=CARTESIAN_POINT('Ctrl Pts',(53.5148335827682,30.3316641336367,6.96026524503036));
#44359=CARTESIAN_POINT('Ctrl Pts',(53.5070420201277,30.3229340769405,6.96101196056232));
#44360=CARTESIAN_POINT('Ctrl Pts',(53.5023366178853,30.3176048342012,6.96146354764638));
#44361=CARTESIAN_POINT('Ctrl Pts',(53.4853541207843,30.2981622885126,6.96309621503646));
#44362=CARTESIAN_POINT('Ctrl Pts',(53.4732467744923,30.2839011309568,6.96426560881298));
#44363=CARTESIAN_POINT('Ctrl Pts',(53.4099056700461,30.2071287384328,6.97042580200009));
#44364=CARTESIAN_POINT('Ctrl Pts',(53.3623007487888,30.1417108707432,6.97520832855291));
#44365=CARTESIAN_POINT('Ctrl Pts',(53.2740924655199,30.0035780495066,6.98478744549072));
#44366=CARTESIAN_POINT('Ctrl Pts',(53.2338075213227,29.9308544494379,6.98957257553851));
#44367=CARTESIAN_POINT('Ctrl Pts',(53.1529101035594,29.7605367969924,7.00060035072053));
#44368=CARTESIAN_POINT('Ctrl Pts',(53.1152839154119,29.6618143877731,7.00687543281817));
#44369=CARTESIAN_POINT('Ctrl Pts',(53.0812290330443,29.5455199865914,7.01439622596903));
#44370=CARTESIAN_POINT('Ctrl Pts',(53.0769947523479,29.5304006740588,7.01537614293193));
#44371=CARTESIAN_POINT('Ctrl Pts',(53.0703986791068,29.5057302329335,7.01697929839781));
#44372=CARTESIAN_POINT('Ctrl Pts',(53.0679282400433,29.4962086606766,7.01759904807972));
#44373=CARTESIAN_POINT('Ctrl Pts',(53.0636461863744,29.4791878403923,7.01870888437768));
#44374=CARTESIAN_POINT('Ctrl Pts',(53.0618074495076,29.4716955717669,7.01919809191215));
#44375=CARTESIAN_POINT('Ctrl Pts',(53.0580130530898,29.4558377625538,7.02023504060823));
#44376=CARTESIAN_POINT('Ctrl Pts',(53.0560678880824,29.4474698964312,7.02078310567221));
#44377=CARTESIAN_POINT('Ctrl Pts',(53.0522213635964,29.4304240534228,7.02190144655977));
#44378=CARTESIAN_POINT('Ctrl Pts',(53.0503238028868,29.4217454260556,7.02247182977963));
#44379=CARTESIAN_POINT('Ctrl Pts',(53.0478789049589,29.4101942714901,7.02323238708284));
#44380=CARTESIAN_POINT('Ctrl Pts',(53.047279802351,29.4073327134691,7.02342091185398));
#44381=CARTESIAN_POINT('Ctrl Pts',(53.0466869980042,29.4044698737041,7.02360963496715));
#44382=CARTESIAN_POINT('Origin',(55.,29.,3.45145488139523));
#44383=CARTESIAN_POINT('',(53.0466869993245,29.4044698800802,7.9829668504648));
#44384=CARTESIAN_POINT('',(53.0466869980082,29.4044698737233,7.82538782795618));
#44385=CARTESIAN_POINT('',(53.0466869980082,29.4044698737233,3.45145488139523));
#44386=CARTESIAN_POINT('Ctrl Pts',(53.0466869993245,29.4044698800804,7.98296685046478));
#44387=CARTESIAN_POINT('Ctrl Pts',(53.058256749032,29.4603438613858,7.97899706014529));
#44388=CARTESIAN_POINT('Ctrl Pts',(53.0722308559657,29.5157554395691,7.97504270473785));
#44389=CARTESIAN_POINT('Ctrl Pts',(53.09660062202,29.5973971457715,7.96925228785007));
#44390=CARTESIAN_POINT('Ctrl Pts',(53.1051795072496,29.6240737166142,7.96736626695004));
#44391=CARTESIAN_POINT('Ctrl Pts',(53.1202708552382,29.6678166395263,7.96429308346822));
#44392=CARTESIAN_POINT('Ctrl Pts',(53.1264605265564,29.684989503327,7.9630916300141));
#44393=CARTESIAN_POINT('Ctrl Pts',(53.1352247274185,29.7082972012562,7.961470149161));
#44394=CARTESIAN_POINT('Ctrl Pts',(53.1375952712547,29.7145070831788,7.96103903453475));
#44395=CARTESIAN_POINT('Ctrl Pts',(53.1416201433371,29.724894514447,7.96031954278676));
#44396=CARTESIAN_POINT('Ctrl Pts',(53.1432576083671,29.7290784875535,7.960030186707));
#44397=CARTESIAN_POINT('Ctrl Pts',(53.1463869130747,29.7369954180128,7.95948356681448));
#44398=CARTESIAN_POINT('Ctrl Pts',(53.147875919644,29.7407294471354,7.95922613255389));
#44399=CARTESIAN_POINT('Ctrl Pts',(53.1518041756027,29.7504945570915,7.95855383018765));
#44400=CARTESIAN_POINT('Ctrl Pts',(53.1542616834397,29.7565183111737,7.95814004299468));
#44401=CARTESIAN_POINT('Ctrl Pts',(53.1628856813414,29.7773649598123,7.95671091414849));
#44402=CARTESIAN_POINT('Ctrl Pts',(53.1692018014966,29.792125807633,7.95570406270219));
#44403=CARTESIAN_POINT('Ctrl Pts',(53.2178472440217,29.9021196906272,7.94822779975666));
#44404=CARTESIAN_POINT('Ctrl Pts',(53.2674089238648,29.9939930000087,7.94212831651028));
#44405=CARTESIAN_POINT('Ctrl Pts',(53.3723791147905,30.1566598034611,7.93086833385433));
#44406=CARTESIAN_POINT('Ctrl Pts',(53.4258172509597,30.2283972241488,7.92571049418162));
#44407=CARTESIAN_POINT('Ctrl Pts',(53.5192931652996,30.3377234201072,7.91721248782243));
#44408=CARTESIAN_POINT('Ctrl Pts',(53.55638361103,30.3776675013163,7.91395320651823));
#44409=CARTESIAN_POINT('Ctrl Pts',(53.6117569470897,30.4326067039399,7.90919672110261));
#44410=CARTESIAN_POINT('Ctrl Pts',(53.6287443882276,30.4488749846551,7.90775131565239));
#44411=CARTESIAN_POINT('Ctrl Pts',(53.6594621440349,30.4772681333704,7.90515842363056));
#44412=CARTESIAN_POINT('Ctrl Pts',(53.6730794447241,30.4895115597093,7.90401595915376));
#44413=CARTESIAN_POINT('Ctrl Pts',(53.6939505111383,30.5077635569917,7.902274263741));
#44414=CARTESIAN_POINT('Ctrl Pts',(53.7010816860669,30.5139112985939,7.90168078008074));
#44415=CARTESIAN_POINT('Ctrl Pts',(53.7138893422637,30.5247955900981,7.90061759620665));
#44416=CARTESIAN_POINT('Ctrl Pts',(53.7195491717601,30.5295515321807,7.90014869812735));
#44417=CARTESIAN_POINT('Ctrl Pts',(53.7318746572385,30.5397922554801,7.89912951003128));
#44418=CARTESIAN_POINT('Ctrl Pts',(53.7385497179463,30.5452654325582,7.89857876551159));
#44419=CARTESIAN_POINT('Ctrl Pts',(53.7565134784349,30.5598007525789,7.8970997132618));
#44420=CARTESIAN_POINT('Ctrl Pts',(53.767865483786,30.5687834881847,7.89616827652151));
#44421=CARTESIAN_POINT('Ctrl Pts',(53.8195387105894,30.6087651803162,7.89194210521781));
#44422=CARTESIAN_POINT('Ctrl Pts',(53.8609356982831,30.6383363542787,7.888592685866));
#44423=CARTESIAN_POINT('Ctrl Pts',(54.025675521768,30.7467515489523,7.87539183268403));
#44424=CARTESIAN_POINT('Ctrl Pts',(54.156408452148,30.8135025719006,7.86514014977479));
#44425=CARTESIAN_POINT('Ctrl Pts',(54.3701635191774,30.8944920781916,7.84925561106511));
#44426=CARTESIAN_POINT('Ctrl Pts',(54.4488244908911,30.9188544956094,7.84359128707348));
#44427=CARTESIAN_POINT('Ctrl Pts',(54.5441164810909,30.9420214042953,7.83709955782068));
#44428=CARTESIAN_POINT('Ctrl Pts',(54.5595048530021,30.9455695773487,7.8360625996412));
#44429=CARTESIAN_POINT('Ctrl Pts',(54.581069107399,30.9502727747297,7.834626837203));
#44430=CARTESIAN_POINT('Ctrl Pts',(54.5872102978464,30.951581833536,7.83421991175346));
#44431=CARTESIAN_POINT('Ctrl Pts',(54.5976847959668,30.9537629270249,7.83352930758292));
#44432=CARTESIAN_POINT('Ctrl Pts',(54.6020149798198,30.9546495909957,7.83324481407801));
#44433=CARTESIAN_POINT('Ctrl Pts',(54.6103623133197,30.9563299317769,7.83269836873879));
#44434=CARTESIAN_POINT('Ctrl Pts',(54.6143789842356,30.9571256377098,7.83243629825188));
#44435=CARTESIAN_POINT('Ctrl Pts',(54.6240444389855,30.9590094615944,7.83180770914746));
#44436=CARTESIAN_POINT('Ctrl Pts',(54.6296955743781,30.960085530987,7.83144186308687));
#44437=CARTESIAN_POINT('Ctrl Pts',(54.6504122947935,30.9639375429333,7.83010655575824));
#44438=CARTESIAN_POINT('Ctrl Pts',(54.665505517672,30.9665644436056,7.8291450530694));
#44439=CARTESIAN_POINT('Ctrl Pts',(54.8102424195978,30.9900405748958,7.82002007968978));
#44440=CARTESIAN_POINT('Ctrl Pts',(54.9416352029698,30.9982174090173,7.81245324320272));
#44441=CARTESIAN_POINT('Ctrl Pts',(55.2159389231107,30.9881869584236,7.79651215720499));
#44442=CARTESIAN_POINT('Ctrl Pts',(55.3579852893726,30.9675762250938,7.78815511850839));
#44443=CARTESIAN_POINT('Ctrl Pts',(55.5135038781799,30.9276011321715,7.77818948728048));
#44444=CARTESIAN_POINT('Ctrl Pts',(55.5303543803362,30.9230331663275,7.77709922981147));
#44445=CARTESIAN_POINT('Ctrl Pts',(55.5560607117063,30.9157009305978,7.77541895381105));
#44446=CARTESIAN_POINT('Ctrl Pts',(55.5649611041334,30.9130950098609,7.77483403758255));
#44447=CARTESIAN_POINT('Ctrl Pts',(55.5804748039049,30.9084350958864,7.77380886263698));
#44448=CARTESIAN_POINT('Ctrl Pts',(55.5870962387047,30.9064085390371,7.77336950003555));
#44449=CARTESIAN_POINT('Ctrl Pts',(55.6020260349922,30.90175396677,7.77237469091108));
#44450=CARTESIAN_POINT('Ctrl Pts',(55.6103279550488,30.8991059160222,7.77181859947228));
#44451=CARTESIAN_POINT('Ctrl Pts',(55.6327295148991,30.8917984645812,7.7703100337936));
#44452=CARTESIAN_POINT('Ctrl Pts',(55.6467946902029,30.8870359505526,7.76935420962558));
#44453=CARTESIAN_POINT('Ctrl Pts',(55.7122001169103,30.864072320203,7.76486803601261));
#44454=CARTESIAN_POINT('Ctrl Pts',(55.7628299557096,30.843931707293,7.76127451317597));
#44455=CARTESIAN_POINT('Ctrl Pts',(55.9773159941087,30.7482627279924,7.74551321755942));
#44456=CARTESIAN_POINT('Ctrl Pts',(56.1313262609965,30.6527713697668,7.73270425254582));
#44457=CARTESIAN_POINT('Ctrl Pts',(56.2981490696811,30.5149702224225,7.71788395938611));
#44458=CARTESIAN_POINT('Ctrl Pts',(56.325303075136,30.4912739014594,7.71544080017243));
#44459=CARTESIAN_POINT('Ctrl Pts',(56.3679177708981,30.4520016675498,7.71157486702448));
#44460=CARTESIAN_POINT('Ctrl Pts',(56.3837887632463,30.4368843462613,7.71012763146908));
#44461=CARTESIAN_POINT('Ctrl Pts',(56.4044856083783,30.4165092672847,7.708234121535));
#44462=CARTESIAN_POINT('Ctrl Pts',(56.4095363496569,30.4114834788783,7.70777153729304));
#44463=CARTESIAN_POINT('Ctrl Pts',(56.4178004033383,30.403171657022,7.70701398933276));
#44464=CARTESIAN_POINT('Ctrl Pts',(56.4210294295137,30.3999014409133,7.70671782247437));
#44465=CARTESIAN_POINT('Ctrl Pts',(56.4273353113667,30.3934708198436,7.70613916725052));
#44466=CARTESIAN_POINT('Ctrl Pts',(56.4304130250831,30.3903113302691,7.70585661477593));
#44467=CARTESIAN_POINT('Ctrl Pts',(56.4379727507325,30.3824990656663,7.70516219251697));
#44468=CARTESIAN_POINT('Ctrl Pts',(56.4424427369119,30.3778346242954,7.7047512429944));
#44469=CARTESIAN_POINT('Ctrl Pts',(56.4577544338817,30.3617006500387,7.70334201441788));
#44470=CARTESIAN_POINT('Ctrl Pts',(56.4684829630928,30.3501238733153,7.70235191383899));
#44471=CARTESIAN_POINT('Ctrl Pts',(56.5606221808058,30.2483018714429,7.6938121409686));
#44472=CARTESIAN_POINT('Ctrl Pts',(56.6337757698294,30.1509057225283,7.68676991026199));
#44473=CARTESIAN_POINT('Ctrl Pts',(56.7523250472462,29.9587704404674,7.67365987604715));
#44474=CARTESIAN_POINT('Ctrl Pts',(56.8000029196513,29.8659510928186,7.66761595955041));
#44475=CARTESIAN_POINT('Ctrl Pts',(56.853944639569,29.7370096397422,7.6592162431652));
#44476=CARTESIAN_POINT('Ctrl Pts',(56.8667968878204,29.7038203598276,7.65705498695327));
#44477=CARTESIAN_POINT('Ctrl Pts',(56.887340874969,29.6462390851212,7.65329397121755));
#44478=CARTESIAN_POINT('Ctrl Pts',(56.8954641084144,29.6220098513922,7.65170805895421));
#44479=CARTESIAN_POINT('Ctrl Pts',(56.9063536779131,29.5873327456712,7.64943058800991));
#44480=CARTESIAN_POINT('Ctrl Pts',(56.9095042425722,29.577007486723,7.64875150779693));
#44481=CARTESIAN_POINT('Ctrl Pts',(56.9148031789142,29.5591226196559,7.64757337678411));
#44482=CARTESIAN_POINT('Ctrl Pts',(56.9169909929917,29.55157487952,7.64707561401987));
#44483=CARTESIAN_POINT('Ctrl Pts',(56.9211030596698,29.5370686346339,7.64611777284123));
#44484=CARTESIAN_POINT('Ctrl Pts',(56.9230342494557,29.5301122120459,7.64565792730351));
#44485=CARTESIAN_POINT('Ctrl Pts',(56.9274913059824,29.5137123564863,7.64457255272798));
#44486=CARTESIAN_POINT('Ctrl Pts',(56.9299855849412,29.5042606034239,7.64394601908212));
#44487=CARTESIAN_POINT('Ctrl Pts',(56.9384183556305,29.4713263515948,7.64175920298449));
#44488=CARTESIAN_POINT('Ctrl Pts',(56.9439983420182,29.4477550806724,7.64018755802181));
#44489=CARTESIAN_POINT('Ctrl Pts',(56.9788106603771,29.2877547865987,7.62947109318889));
#44490=CARTESIAN_POINT('Ctrl Pts',(56.9940830311268,29.1487086161036,7.61988170300658));
#44491=CARTESIAN_POINT('Ctrl Pts',(56.9949261205005,28.9665675048193,7.60719387944647));
#44492=CARTESIAN_POINT('Ctrl Pts',(56.9937546860302,28.9239063155554,7.60421663448295));
#44493=CARTESIAN_POINT('Ctrl Pts',(56.9864011264306,28.8005329321703,7.59563092414739));
#44494=CARTESIAN_POINT('Ctrl Pts',(56.9766741263554,28.7201095840579,7.59006228582761));
#44495=CARTESIAN_POINT('Ctrl Pts',(56.9592626409828,28.6250828121043,7.58366824560303));
#44496=CARTESIAN_POINT('Ctrl Pts',(56.9562576166606,28.6097063056806,7.58263960691582));
#44497=CARTESIAN_POINT('Ctrl Pts',(56.9517988137639,28.5882377733724,7.58121332570551));
#44498=CARTESIAN_POINT('Ctrl Pts',(56.9504971323217,28.5821152311545,7.58080770055516));
#44499=CARTESIAN_POINT('Ctrl Pts',(56.9482279179279,28.5716834748861,7.58011863444908));
#44500=CARTESIAN_POINT('Ctrl Pts',(56.9472748597342,28.5673711891368,7.57983438741928));
#44501=CARTESIAN_POINT('Ctrl Pts',(56.9454094996615,28.559062082692,7.57928788634528));
#44502=CARTESIAN_POINT('Ctrl Pts',(56.9444991934145,28.555064885811,7.57902551664782));
#44503=CARTESIAN_POINT('Ctrl Pts',(56.9422778673065,28.5454479700905,7.5783954951841));
#44504=CARTESIAN_POINT('Ctrl Pts',(56.9409547627849,28.5398310391723,7.57802852274043));
#44505=CARTESIAN_POINT('Ctrl Pts',(56.9359993720645,28.5191957419056,7.57668377727222));
#44506=CARTESIAN_POINT('Ctrl Pts',(56.9322168895523,28.5042135246025,7.57571411254403));
#44507=CARTESIAN_POINT('Ctrl Pts',(56.895173697089,28.3643552824329,7.56671214152172));
#44508=CARTESIAN_POINT('Ctrl Pts',(56.8500208496504,28.2429267894257,7.55925662655601));
#44509=CARTESIAN_POINT('Ctrl Pts',(56.7301960047754,27.9968494529237,7.54336245238481));
#44510=CARTESIAN_POINT('Ctrl Pts',(56.653055936557,27.8742611389787,7.5349387361995));
#44511=CARTESIAN_POINT('Ctrl Pts',(56.5522958983302,27.7471142978037,7.52487466339645));
#44512=CARTESIAN_POINT('Ctrl Pts',(56.5410412858105,27.7332968531751,7.52376213246466));
#44513=CARTESIAN_POINT('Ctrl Pts',(56.5236022144679,27.7124631008254,7.5220546537203));
#44514=CARTESIAN_POINT('Ctrl Pts',(56.5175508505609,27.705336188094,7.52146507244251));
#44515=CARTESIAN_POINT('Ctrl Pts',(56.5069259843949,27.6929997352353,7.52043479147969));
#44516=CARTESIAN_POINT('Ctrl Pts',(56.5023749778709,27.687770965709,7.51999501829732));
#44517=CARTESIAN_POINT('Ctrl Pts',(56.4920776350535,27.6760638679754,7.51900332634028));
#44518=CARTESIAN_POINT('Ctrl Pts',(56.4863162094975,27.6695990558419,7.5184507870748));
#44519=CARTESIAN_POINT('Ctrl Pts',(56.47072759648,27.652334946948,7.51696183760949));
#44520=CARTESIAN_POINT('Ctrl Pts',(56.4608237754154,27.6416058610416,7.51602222501837));
#44521=CARTESIAN_POINT('Ctrl Pts',(56.4149657699492,27.5930081269185,7.5116993639499));
#44522=CARTESIAN_POINT('Ctrl Pts',(56.3776538449613,27.5564546024662,7.50825829588231));
#44523=CARTESIAN_POINT('Ctrl Pts',(56.2033846403688,27.3986432426049,7.49250589784078));
#44524=CARTESIAN_POINT('Ctrl Pts',(56.0515797433873,27.2951129324974,7.47951785521477));
#44525=CARTESIAN_POINT('Ctrl Pts',(55.8554481099161,27.1976279752204,7.46451448194547));
#44526=CARTESIAN_POINT('Ctrl Pts',(55.8226174920834,27.1824089685719,7.4620610661412));
#44527=CARTESIAN_POINT('Ctrl Pts',(55.7692039190095,27.1593924923555,7.45818080225043));
#44528=CARTESIAN_POINT('Ctrl Pts',(55.748875188057,27.1510282005852,7.45672928335571));
#44529=CARTESIAN_POINT('Ctrl Pts',(55.7217712387449,27.1403966237849,7.45483108397166));
#44530=CARTESIAN_POINT('Ctrl Pts',(55.7151170565212,27.1378276027448,7.45436799432134));
#44531=CARTESIAN_POINT('Ctrl Pts',(55.7041514725323,27.1336614985584,7.45360983344906));
#44532=CARTESIAN_POINT('Ctrl Pts',(55.6998481432022,27.1320435562548,7.45331355535822));
#44533=CARTESIAN_POINT('Ctrl Pts',(55.691406423735,27.1289029518435,7.45273486297223));
#44534=CARTESIAN_POINT('Ctrl Pts',(55.6872685274846,27.1273791152247,7.45245238356636));
#44535=CARTESIAN_POINT('Ctrl Pts',(55.6770615710574,27.1236586533026,7.4517584160686));
#44536=CARTESIAN_POINT('Ctrl Pts',(55.6709867704976,27.121477714559,7.45134784547262));
#44537=CARTESIAN_POINT('Ctrl Pts',(55.6500557091463,27.1140776581088,7.44994127691316));
#44538=CARTESIAN_POINT('Ctrl Pts',(55.6351478577089,27.1090048282404,7.44895341614856));
#44539=CARTESIAN_POINT('Ctrl Pts',(55.5029815265541,27.0657707830142,7.44030520854156));
#44540=CARTESIAN_POINT('Ctrl Pts',(55.382462655455,27.0383772572288,7.43316759851297));
#44541=CARTESIAN_POINT('Ctrl Pts',(55.1581317439686,27.0088660906528,7.42002900329593));
#44542=CARTESIAN_POINT('Ctrl Pts',(55.0552106473647,27.0033604080661,7.41405493492404));
#44543=CARTESIAN_POINT('Ctrl Pts',(54.9170048944666,27.006664100843,7.40574460306981));
#44544=CARTESIAN_POINT('Ctrl Pts',(54.8817093102582,27.0084470142943,7.40359805861164));
#44545=CARTESIAN_POINT('Ctrl Pts',(54.8211411944945,27.0131222916088,7.39986040500741));
#44546=CARTESIAN_POINT('Ctrl Pts',(54.795841904756,27.0155623259862,7.39828290721759));
#44547=CARTESIAN_POINT('Ctrl Pts',(54.7598963921876,27.019723792608,7.39601543578436));
#44548=CARTESIAN_POINT('Ctrl Pts',(54.7492061730232,27.0210492555022,7.39533778882544));
#44549=CARTESIAN_POINT('Ctrl Pts',(54.7307407916579,27.0234907710482,7.39416134867105));
#44550=CARTESIAN_POINT('Ctrl Pts',(54.7229604455916,27.0245662917111,7.39366383336948));
#44551=CARTESIAN_POINT('Ctrl Pts',(54.7080361239225,27.0267192665489,7.3927059062986));
#44552=CARTESIAN_POINT('Ctrl Pts',(54.7008912394898,27.0277896397483,7.3922457241843));
#44553=CARTESIAN_POINT('Ctrl Pts',(54.6840727336928,27.0304027105315,7.39115868806623));
#44554=CARTESIAN_POINT('Ctrl Pts',(54.6744044186631,27.0319778883208,7.39053082186408));
#44555=CARTESIAN_POINT('Ctrl Pts',(54.6407522096671,27.0377153278892,7.38833484031418));
#44556=CARTESIAN_POINT('Ctrl Pts',(54.61683400196,27.0422452041131,7.38675523663701));
#44557=CARTESIAN_POINT('Ctrl Pts',(54.4647426402105,27.0739436414041,7.37658623668558));
#44558=CARTESIAN_POINT('Ctrl Pts',(54.3394474144801,27.1132427693404,7.36760964848039));
#44559=CARTESIAN_POINT('Ctrl Pts',(54.1265165393998,27.2038539338081,7.35150558040402));
#44560=CARTESIAN_POINT('Ctrl Pts',(54.0372030134549,27.2501035455637,7.34446669077798));
#44561=CARTESIAN_POINT('Ctrl Pts',(53.9279170166428,27.3176057662148,7.33573691058411));
#44562=CARTESIAN_POINT('Ctrl Pts',(53.9043954342116,27.332827819907,7.33385121169732));
#44563=CARTESIAN_POINT('Ctrl Pts',(53.8660915882586,27.3587771773414,7.33077849516072));
#44564=CARTESIAN_POINT('Ctrl Pts',(53.8511225668072,27.3692206342248,7.32957719181216));
#44565=CARTESIAN_POINT('Ctrl Pts',(53.830900105809,27.3837459433206,7.32795587899305));
#44566=CARTESIAN_POINT('Ctrl Pts',(53.8255211616559,27.3876504102281,7.32752478519715));
#44567=CARTESIAN_POINT('Ctrl Pts',(53.8165390476539,27.3942391453251,7.32680531850831));
#44568=CARTESIAN_POINT('Ctrl Pts',(53.8129252892231,27.396908804733,7.32651596680101));
#44569=CARTESIAN_POINT('Ctrl Pts',(53.8060952666062,27.401990234633,7.32596934788591));
#44570=CARTESIAN_POINT('Ctrl Pts',(53.8028772308953,27.4043995490678,7.32571191027209));
#44571=CARTESIAN_POINT('Ctrl Pts',(53.7944702769207,27.4107335100226,7.32503958587472));
#44572=CARTESIAN_POINT('Ctrl Pts',(53.7892931852811,27.4146738818139,7.32462578014157));
#44573=CARTESIAN_POINT('Ctrl Pts',(53.7714068107378,27.4284262242267,7.3231965216192));
#44574=CARTESIAN_POINT('Ctrl Pts',(53.7587963943306,27.4383665587333,7.32218956108257));
#44575=CARTESIAN_POINT('Ctrl Pts',(53.6639988194956,27.5149659015489,7.31461345651484));
#44576=CARTESIAN_POINT('Ctrl Pts',(53.5871023589485,27.5879265476658,7.30842594831309));
#44577=CARTESIAN_POINT('Ctrl Pts',(53.439900501296,27.7517217911272,7.29562064378984));
#44578=CARTESIAN_POINT('Ctrl Pts',(53.3709122049121,27.8432026560081,7.28902582320648));
#44579=CARTESIAN_POINT('Ctrl Pts',(53.2791429265253,27.9895137553325,7.27867825059314));
#44580=CARTESIAN_POINT('Ctrl Pts',(53.2503279811946,28.0402717175552,7.27512389268616));
#44581=CARTESIAN_POINT('Ctrl Pts',(53.2171709388505,28.1051485949626,7.27058502461403));
#44582=CARTESIAN_POINT('Ctrl Pts',(53.210703009256,28.1181526437211,7.26967551919338));
#44583=CARTESIAN_POINT('Ctrl Pts',(53.2006137056474,28.1390056797287,7.26821695281176));
#44584=CARTESIAN_POINT('Ctrl Pts',(53.1969002701736,28.1468097419918,7.26767107610022));
#44585=CARTESIAN_POINT('Ctrl Pts',(53.1899723374444,28.1616165603018,7.26663521678136));
#44586=CARTESIAN_POINT('Ctrl Pts',(53.1867474636532,28.1686143085819,7.26614560141701));
#44587=CARTESIAN_POINT('Ctrl Pts',(53.1795343351045,28.1845078994495,7.26503333213097));
#44588=CARTESIAN_POINT('Ctrl Pts',(53.1755706138886,28.1934145967883,7.26440985640041));
#44589=CARTESIAN_POINT('Ctrl Pts',(53.1655107147186,28.2164733170062,7.26279513176812));
#44590=CARTESIAN_POINT('Ctrl Pts',(53.1595130373644,28.2306673546693,7.26180059177553));
#44591=CARTESIAN_POINT('Ctrl Pts',(53.1179166391773,28.3323799787954,7.25466830177191));
#44592=CARTESIAN_POINT('Ctrl Pts',(53.0884162205546,28.4222482280429,7.24832876228336));
#44593=CARTESIAN_POINT('Ctrl Pts',(53.023562523072,28.6803332287233,7.23006428913969));
#44594=CARTESIAN_POINT('Ctrl Pts',(53.0033931300134,28.8515035560417,7.21783037161033));
#44595=CARTESIAN_POINT('Ctrl Pts',(53.0055596025529,29.0382582085128,7.20536269312291));
#44596=CARTESIAN_POINT('Ctrl Pts',(53.0059069074542,29.0533756303228,7.20436029661958));
#44597=CARTESIAN_POINT('Ctrl Pts',(53.006817465833,29.0798804490078,7.20261646716537));
#44598=CARTESIAN_POINT('Ctrl Pts',(53.0073064990734,29.0912695268911,7.20187156670995));
#44599=CARTESIAN_POINT('Ctrl Pts',(53.008176480545,29.1081523989988,7.20077451358064));
#44600=CARTESIAN_POINT('Ctrl Pts',(53.0084825763716,29.1136495807192,7.20041843336773));
#44601=CARTESIAN_POINT('Ctrl Pts',(53.0090688051341,29.1234467780605,7.19978591454569));
#44602=CARTESIAN_POINT('Ctrl Pts',(53.0093401144347,29.1277472148095,7.19950899806007));
#44603=CARTESIAN_POINT('Ctrl Pts',(53.0099591961832,29.1370787848985,7.19890969838135));
#44604=CARTESIAN_POINT('Ctrl Pts',(53.0103121124014,29.1421094839134,7.19858760254091));
#44605=CARTESIAN_POINT('Ctrl Pts',(53.0113411716254,29.1560223544458,7.19769942173102));
#44606=CARTESIAN_POINT('Ctrl Pts',(53.0120577479138,29.1649015467617,7.19713552410449));
#44607=CARTESIAN_POINT('Ctrl Pts',(53.0161643985336,29.2118620306212,7.19416732481635));
#44608=CARTESIAN_POINT('Ctrl Pts',(53.0205895144708,29.2498475221283,7.19181566616976));
#44609=CARTESIAN_POINT('Ctrl Pts',(53.0314832209871,29.3245925942169,7.18724471848035));
#44610=CARTESIAN_POINT('Ctrl Pts',(53.0378966351962,29.3613437508665,7.18502451419171));
#44611=CARTESIAN_POINT('Ctrl Pts',(53.0457833858183,29.4000874820423,7.18269327447379));
#44612=CARTESIAN_POINT('Ctrl Pts',(53.0462333559396,29.4022790926368,7.18256143578627));
#44613=CARTESIAN_POINT('Ctrl Pts',(53.0466869981335,29.4044698743284,7.18242967527062));
#44614=CARTESIAN_POINT('',(53.0052508017986,28.9982114880629,7.05145488142717));
#44615=CARTESIAN_POINT('Ctrl Pts',(53.0466869980042,29.4044698737041,7.02360963496715));
#44616=CARTESIAN_POINT('Ctrl Pts',(53.0445976879508,29.3943799343589,7.02427478038959));
#44617=CARTESIAN_POINT('Ctrl Pts',(53.0425866133465,29.3842740735815,7.02494239072689));
#44618=CARTESIAN_POINT('Ctrl Pts',(53.0169857519414,29.2502088099897,7.03381838151229));
#44619=CARTESIAN_POINT('Ctrl Pts',(53.00513641142,29.1243248017733,7.04240020381067));
#44620=CARTESIAN_POINT('Ctrl Pts',(53.0052508205679,28.9981906755863,7.05115502780437));
#44621=CARTESIAN_POINT('Ctrl Pts',(53.0052508017986,28.9982114880629,7.05145488142717));
#44622=CARTESIAN_POINT('Ctrl Pts',(53.005330467948,28.9093588590626,7.05712256701506));
#44623=CARTESIAN_POINT('Ctrl Pts',(53.0113506355184,28.8207686812029,7.06279025260296));
#44624=CARTESIAN_POINT('Ctrl Pts',(53.0231839296303,28.7331184037289,7.06845793819085));
#44625=CARTESIAN_POINT('Ctrl Pts',(53.0343123097836,28.6506894875669,7.07378799753146));
#44626=CARTESIAN_POINT('Ctrl Pts',(53.0505813290659,28.5690913732212,7.07911805687207));
#44627=CARTESIAN_POINT('Ctrl Pts',(53.0718472890399,28.4888692087957,7.08444811621268));
#44628=CARTESIAN_POINT('Ctrl Pts',(53.0896261223019,28.4218016281651,7.0889041688155));
#44629=CARTESIAN_POINT('Ctrl Pts',(53.1109431910862,28.355531420224,7.09336022141832));
#44630=CARTESIAN_POINT('Ctrl Pts',(53.1357095494889,28.290458825273,7.09781627402114));
#44631=CARTESIAN_POINT('Ctrl Pts',(53.1604389486801,28.2254833391402,7.10226567678923));
#44632=CARTESIAN_POINT('Ctrl Pts',(53.188607248147,28.1617023720646,7.10671507955732));
#44633=CARTESIAN_POINT('Ctrl Pts',(53.2200752937475,28.0995025804746,7.1111644823254));
#44634=CARTESIAN_POINT('Ctrl Pts',(53.2515066084609,28.0373753912175,7.11560869155486));
#44635=CARTESIAN_POINT('Ctrl Pts',(53.2862297995589,27.9768261459978,7.12005290078431));
#44636=CARTESIAN_POINT('Ctrl Pts',(53.3240577194163,27.9182213559827,7.12449711001376));
#44637=CARTESIAN_POINT('Ctrl Pts',(53.3618620647527,27.8596530887227,7.12893854959307));
#44638=CARTESIAN_POINT('Ctrl Pts',(53.4027670356867,27.803027282564,7.13337998917237));
#44639=CARTESIAN_POINT('Ctrl Pts',(53.4465404238203,27.7486843293255,7.13782142875168));
#44640=CARTESIAN_POINT('Ctrl Pts',(53.4903013669552,27.6943568260673,7.14226160560693));
#44641=CARTESIAN_POINT('Ctrl Pts',(53.5369288016427,27.6423112678627,7.14670178246219));
#44642=CARTESIAN_POINT('Ctrl Pts',(53.5861492903504,27.5928561788775,7.15114195931745));
#44643=CARTESIAN_POINT('Ctrl Pts',(53.6353724656587,27.5433983904864,7.15558237853077));
#44644=CARTESIAN_POINT('Ctrl Pts',(53.687188629292,27.4965316969205,7.16002279774409));
#44645=CARTESIAN_POINT('Ctrl Pts',(53.7412876925744,27.4525275803313,7.16446321695741));
#44646=CARTESIAN_POINT('Ctrl Pts',(53.7954437835132,27.4084770775112,7.16890831696714));
#44647=CARTESIAN_POINT('Ctrl Pts',(53.8518871969525,27.3672954833691,7.17335341697686));
#44648=CARTESIAN_POINT('Ctrl Pts',(53.9102757449189,27.3292131762586,7.17779851698659));
#44649=CARTESIAN_POINT('Ctrl Pts',(53.9686986081662,27.2911084879601,7.18224622940681));
#44650=CARTESIAN_POINT('Ctrl Pts',(54.0290684581531,27.2561069574895,7.18669394182704));
#44651=CARTESIAN_POINT('Ctrl Pts',(54.0910175906236,27.2243934720935,7.19114165424727));
#44652=CARTESIAN_POINT('Ctrl Pts',(54.1530732469453,27.1926254541727,7.19559701467543));
#44653=CARTESIAN_POINT('Ctrl Pts',(54.2167131600073,27.1641569663705,7.20005237510359));
#44654=CARTESIAN_POINT('Ctrl Pts',(54.2815494725857,27.1391248289694,7.20450773553175));
#44655=CARTESIAN_POINT('Ctrl Pts',(54.3137744230974,27.1266833535543,7.20672213921387));
#44656=CARTESIAN_POINT('Ctrl Pts',(54.3462946796159,27.1150899806534,7.208936542896));
#44657=CARTESIAN_POINT('Ctrl Pts',(54.3790614983329,27.1043568532956,7.21115094657813));
#44658=CARTESIAN_POINT('Ctrl Pts',(54.4449982766341,27.0827585454103,7.21560699847377));
#44659=CARTESIAN_POINT('Ctrl Pts',(54.5121924168342,27.0645622877864,7.2200630503694));
#44660=CARTESIAN_POINT('Ctrl Pts',(54.5802597651972,27.0499113615562,7.22451910226504));
#44661=CARTESIAN_POINT('Ctrl Pts',(54.6482255355046,27.035282299151,7.22896850431904));
#44662=CARTESIAN_POINT('Ctrl Pts',(54.7170614532739,27.0241881689483,7.23341790637304));
#44663=CARTESIAN_POINT('Ctrl Pts',(54.7863674258446,27.0167227410774,7.23786730842703));
#44664=CARTESIAN_POINT('Ctrl Pts',(54.8555925013184,27.0092660271948,7.24231151693572));
#44665=CARTESIAN_POINT('Ctrl Pts',(54.9252860579139,27.0054296550877,7.24675572544441));
#44666=CARTESIAN_POINT('Ctrl Pts',(54.9950387736206,27.0052561696466,7.2511999339531));
#44667=CARTESIAN_POINT('Ctrl Pts',(55.0647480190721,27.0050827923226,7.25564137280793));
#44668=CARTESIAN_POINT('Ctrl Pts',(55.1345158625737,27.0085677742324,7.26008281166277));
#44669=CARTESIAN_POINT('Ctrl Pts',(55.203930360552,27.0157016427601,7.2645242505176));
#44670=CARTESIAN_POINT('Ctrl Pts',(55.2733251235887,27.0228334830878,7.26896442664579));
#44671=CARTESIAN_POINT('Ctrl Pts',(55.3423662543198,27.033612100505,7.27340460277399));
#44672=CARTESIAN_POINT('Ctrl Pts',(55.4106460953808,27.0479760895808,7.27784477890218));
#44673=CARTESIAN_POINT('Ctrl Pts',(55.4789296633368,27.0623408626812,7.28228519738697));
#44674=CARTESIAN_POINT('Ctrl Pts',(55.5464513810847,27.0802912929114,7.28672561587176));
#44675=CARTESIAN_POINT('Ctrl Pts',(55.6128147101192,27.1017150652335,7.29116603435654));
#44676=CARTESIAN_POINT('Ctrl Pts',(55.6792479950412,27.1231614210972,7.29561113364051));
#44677=CARTESIAN_POINT('Ctrl Pts',(55.7445199878621,27.148088276039,7.30005623292447));
#44678=CARTESIAN_POINT('Ctrl Pts',(55.8082511540919,27.1763340123781,7.30450133220844));
#44679=CARTESIAN_POINT('Ctrl Pts',(55.8720197755036,27.2045963489028,7.30894904390344));
#44680=CARTESIAN_POINT('Ctrl Pts',(55.9342453317487,27.2361812277723,7.31339675559844));
#44681=CARTESIAN_POINT('Ctrl Pts',(55.9945725563398,27.2708808622088,7.31784446729343));
#44682=CARTESIAN_POINT('Ctrl Pts',(56.0550035159831,27.3056401640412,7.32229982700486));
#44683=CARTESIAN_POINT('Ctrl Pts',(56.1135292180118,27.3435246464504,7.32675518671628));
#44684=CARTESIAN_POINT('Ctrl Pts',(56.169823744429,27.3842834501466,7.3312105464277));
#44685=CARTESIAN_POINT('Ctrl Pts',(56.1978033420369,27.404541457434,7.33342495659966));
#44686=CARTESIAN_POINT('Ctrl Pts',(56.2252322915135,27.4255088867476,7.33563936677162));
#44687=CARTESIAN_POINT('Ctrl Pts',(56.2520738704859,27.4471514609124,7.33785377694358));
#44688=CARTESIAN_POINT('Ctrl Pts',(56.306087108594,27.4907027554484,7.34230982865389));
#44689=CARTESIAN_POINT('Ctrl Pts',(56.357931130304,27.5371608355829,7.34676588036421));
#44690=CARTESIAN_POINT('Ctrl Pts',(56.4072766141824,27.5862814658939,7.35122193207452));
#44691=CARTESIAN_POINT('Ctrl Pts',(56.4565484588945,27.6353287925915,7.35567133393751));
#44692=CARTESIAN_POINT('Ctrl Pts',(56.5033288226362,27.6870304407377,7.36012073580051));
#44693=CARTESIAN_POINT('Ctrl Pts',(56.5473212378837,27.7411018511039,7.3645701376635));
#44694=CARTESIAN_POINT('Ctrl Pts',(56.5912623030984,27.7951101467564,7.3690143459737));
#44695=CARTESIAN_POINT('Ctrl Pts',(56.6324215761606,27.8514823330851,7.37345855428391));
#44696=CARTESIAN_POINT('Ctrl Pts',(56.670540534099,27.9098982219847,7.37790276259411));
#44697=CARTESIAN_POINT('Ctrl Pts',(56.7086357360648,27.9682777057374,7.38234420124593));
#44698=CARTESIAN_POINT('Ctrl Pts',(56.7436941151949,28.0286979566868,7.38678563989775));
#44699=CARTESIAN_POINT('Ctrl Pts',(56.7754993549302,28.090808269317,7.39122707854957));
#44700=CARTESIAN_POINT('Ctrl Pts',(56.8072955522221,28.1529009235678,7.39566725447052));
#44701=CARTESIAN_POINT('Ctrl Pts',(56.8358402235265,28.2166822505069,7.40010743039146));
#44702=CARTESIAN_POINT('Ctrl Pts',(56.8609629482528,28.2817768677282,7.40454760631241));
#44703=CARTESIAN_POINT('Ctrl Pts',(56.8860870442219,28.346875037929,7.40898802458603));
#44704=CARTESIAN_POINT('Ctrl Pts',(56.907788649001,28.4132861836269,7.41342844285964));
#44705=CARTESIAN_POINT('Ctrl Pts',(56.9259460993766,28.4806165339595,7.41786886113326));
#44706=CARTESIAN_POINT('Ctrl Pts',(56.9441226901329,28.548017859485,7.42231396020152));
#44707=CARTESIAN_POINT('Ctrl Pts',(56.958747542426,28.6163398504778,7.42675905926977));
#44708=CARTESIAN_POINT('Ctrl Pts',(56.9697496063415,28.6851761590708,7.43120415833803));
#44709=CARTESIAN_POINT('Ctrl Pts',(56.980758136228,28.7540529231248,7.43565186981443));
#44710=CARTESIAN_POINT('Ctrl Pts',(56.9881395881643,28.8234441200276,7.44009958129082));
#44711=CARTESIAN_POINT('Ctrl Pts',(56.9918748515594,28.8929386240275,7.44454729276721));
#44712=CARTESIAN_POINT('Ctrl Pts',(56.9956165378864,28.9625526265509,7.44900265225781));
#44713=CARTESIAN_POINT('Ctrl Pts',(56.9956995204162,29.032269801885,7.45345801174842));
#44714=CARTESIAN_POINT('Ctrl Pts',(56.9921567962098,29.1016801938195,7.45791337123902));
#44715=CARTESIAN_POINT('Ctrl Pts',(56.99039598407,29.1361786909147,7.46012778326235));
#44716=CARTESIAN_POINT('Ctrl Pts',(56.987740316033,29.1706015002951,7.46234219528569));
#44717=CARTESIAN_POINT('Ctrl Pts',(56.9841985529908,29.2048991576584,7.46455660730903));
#44718=CARTESIAN_POINT('Ctrl Pts',(56.9770714781229,29.2739161892637,7.46901265930649));
#44719=CARTESIAN_POINT('Ctrl Pts',(56.9663251945019,29.3426960836193,7.47346871130395));
#44720=CARTESIAN_POINT('Ctrl Pts',(56.9519852901646,29.4108296355923,7.47792476330141));
#44721=CARTESIAN_POINT('Ctrl Pts',(56.9376667855111,29.478861510704,7.48237416545651));
#44722=CARTESIAN_POINT('Ctrl Pts',(56.9197654043598,29.5462484831796,7.4868235676116));
#44723=CARTESIAN_POINT('Ctrl Pts',(56.8983584450676,29.6125869542691,7.4912729697667));
#44724=CARTESIAN_POINT('Ctrl Pts',(56.8769764729631,29.6788479920432,7.4957171783749));
#44725=CARTESIAN_POINT('Ctrl Pts',(56.8520971994254,29.7440624960506,7.5001613869831));
#44726=CARTESIAN_POINT('Ctrl Pts',(56.8238484662561,29.8078393000067,7.5046055955913));
#44727=CARTESIAN_POINT('Ctrl Pts',(56.7956173378504,29.8715763579129,7.5090470345446));
#44728=CARTESIAN_POINT('Ctrl Pts',(56.7640211132783,29.9338770471652,7.5134884734979));
#44729=CARTESIAN_POINT('Ctrl Pts',(56.7292362103178,29.994368991585,7.5179299124512));
#44730=CARTESIAN_POINT('Ctrl Pts',(56.6944611969147,30.0548437377807,7.52237008867666));
#44731=CARTESIAN_POINT('Ctrl Pts',(56.6564995485811,30.1135103363396,7.52681026490211));
#44732=CARTESIAN_POINT('Ctrl Pts',(56.6155733684929,30.1700214756646,7.53125044112756));
#44733=CARTESIAN_POINT('Ctrl Pts',(56.5746449545579,30.2265356995002,7.53569085970825));
#44734=CARTESIAN_POINT('Ctrl Pts',(56.5307519764274,30.2808938358961,7.54013127828894));
#44735=CARTESIAN_POINT('Ctrl Pts',(56.4841585055315,30.3327794614858,7.54457169686962));
#44736=CARTESIAN_POINT('Ctrl Pts',(56.4375159188712,30.3847197814805,7.54901679624675));
#44737=CARTESIAN_POINT('Ctrl Pts',(56.3881674852917,30.4341820242444,7.55346189562388));
#44738=CARTESIAN_POINT('Ctrl Pts',(56.3364153800509,30.480885375194,7.557906995001));
#44739=CARTESIAN_POINT('Ctrl Pts',(56.2846328598102,30.5276161739625,7.56235470678773));
#44740=CARTESIAN_POINT('Ctrl Pts',(56.2304442359862,30.5715845454544,7.56680241857447));
#44741=CARTESIAN_POINT('Ctrl Pts',(56.1741839674546,30.612550642018,7.5712501303612));
#44742=CARTESIAN_POINT('Ctrl Pts',(56.1178269572052,30.6535871813763,7.57570549016116));
#44743=CARTESIAN_POINT('Ctrl Pts',(56.0593916015765,30.6916108745887,7.58016084996113));
#44744=CARTESIAN_POINT('Ctrl Pts',(55.9992397458495,30.7264262199163,7.58461620976109));
#44745=CARTESIAN_POINT('Ctrl Pts',(55.9693429844244,30.7437301926802,7.58683061906555));
#44746=CARTESIAN_POINT('Ctrl Pts',(55.9390225525708,30.7602423352268,7.58904502837001));
#44747=CARTESIAN_POINT('Ctrl Pts',(55.9083247114548,30.7759430680798,7.59125943767448));
#44748=CARTESIAN_POINT('Ctrl Pts',(55.8465515006347,30.8075376247423,7.59571548956065));
#44749=CARTESIAN_POINT('Ctrl Pts',(55.7830069063956,30.8359672002922,7.60017154144682));
#44750=CARTESIAN_POINT('Ctrl Pts',(55.7180481104491,30.86103048701,7.60462759333299));
#44751=CARTESIAN_POINT('Ctrl Pts',(55.6531862536422,30.8860563713496,7.60907699537553));
#44752=CARTESIAN_POINT('Ctrl Pts',(55.5869148365943,30.9077257631791,7.61352639741806));
#44753=CARTESIAN_POINT('Ctrl Pts',(55.5196144893837,30.9258837828183,7.6179757994606));
#44754=CARTESIAN_POINT('Ctrl Pts',(55.4523926982567,30.9440206075756,7.62242000795491));
#44755=CARTESIAN_POINT('Ctrl Pts',(55.3841448323252,30.9586540740292,7.62686421644922));
#44756=CARTESIAN_POINT('Ctrl Pts',(55.315268608896,30.9696784678583,7.63130842494354));
#44757=CARTESIAN_POINT('Ctrl Pts',(55.2464353095155,30.9806959912235,7.63574986378219));
#44758=CARTESIAN_POINT('Ctrl Pts',(55.1769749113017,30.988108826964,7.64019130262085));
#44759=CARTESIAN_POINT('Ctrl Pts',(55.1072958147491,30.9918622368621,7.64463274145951));
#44760=CARTESIAN_POINT('Ctrl Pts',(55.037636528393,30.9956145796427,7.64907291756974));
#44761=CARTESIAN_POINT('Ctrl Pts',(54.9677591552154,30.9957095357998,7.65351309367997));
#44762=CARTESIAN_POINT('Ctrl Pts',(54.8980759420762,30.9921443343584,7.65795326979021));
#44763=CARTESIAN_POINT('Ctrl Pts',(54.8283889254701,30.9885789383203,7.66239368825527));
#44764=CARTESIAN_POINT('Ctrl Pts',(54.7588965781964,30.9813530154764,7.66683410672033));
#44765=CARTESIAN_POINT('Ctrl Pts',(54.6900080848404,30.9705158144597,7.67127452518539));
#44766=CARTESIAN_POINT('Ctrl Pts',(54.6210469737728,30.9596671895796,7.67571962444707));
#44767=CARTESIAN_POINT('Ctrl Pts',(54.5526914710745,30.9451997649612,7.68016472370876));
#44768=CARTESIAN_POINT('Ctrl Pts',(54.4853416355406,30.9272141371399,7.68460982297044));
#44769=CARTESIAN_POINT('Ctrl Pts',(54.4179522181341,30.9092179390652,7.68905753464167));
#44770=CARTESIAN_POINT('Ctrl Pts',(54.3515701095865,30.8876995731218,7.69350524631289));
#44771=CARTESIAN_POINT('Ctrl Pts',(54.2865785798249,30.8628090185887,7.69795295798412));
#44772=CARTESIAN_POINT('Ctrl Pts',(54.2214752945834,30.8378756637726,7.7024083176697));
#44773=CARTESIAN_POINT('Ctrl Pts',(54.1577678076811,30.8095587446936,7.70686367735528));
#44774=CARTESIAN_POINT('Ctrl Pts',(54.0958170997561,30.7780553549894,7.71131903704085));
#44775=CARTESIAN_POINT('Ctrl Pts',(54.0650262551444,30.7623974874749,7.71353344737388));
#44776=CARTESIAN_POINT('Ctrl Pts',(54.0346689715651,30.7459531607705,7.71574785770691));
#44777=CARTESIAN_POINT('Ctrl Pts',(54.0047868574518,30.7287505208674,7.71796226803994));
#44778=CARTESIAN_POINT('Ctrl Pts',(53.9443850958589,30.6939782236246,7.72243833303645));
#44779=CARTESIAN_POINT('Ctrl Pts',(53.8856890934857,30.6559681027548,7.72691439803296));
#44780=CARTESIAN_POINT('Ctrl Pts',(53.8290670293782,30.6149128585812,7.73139046302947));
#44781=CARTESIAN_POINT('Ctrl Pts',(53.7727928307591,30.574109842983,7.73583902870111));
#44782=CARTESIAN_POINT('Ctrl Pts',(53.7185675837773,30.530299265726,7.74028759437275));
#44783=CARTESIAN_POINT('Ctrl Pts',(53.666728108292,30.483716153879,7.74473616004438));
#44784=CARTESIAN_POINT('Ctrl Pts',(53.6149406275608,30.4371797646776,7.74918026382523));
#44785=CARTESIAN_POINT('Ctrl Pts',(53.5655345327799,30.3878766830037,7.75362436760608));
#44786=CARTESIAN_POINT('Ctrl Pts',(53.5188148507357,30.3360831246966,7.75806847138692));
#44787=CARTESIAN_POINT('Ctrl Pts',(53.4721261933883,30.2843239604471,7.76250962401386));
#44788=CARTESIAN_POINT('Ctrl Pts',(53.4281207344431,30.2300779645987,7.76695077664079));
#44789=CARTESIAN_POINT('Ctrl Pts',(53.3870665053104,30.1736580013821,7.77139192926773));
#44790=CARTESIAN_POINT('Ctrl Pts',(53.3454714476156,30.1164947888531,7.77589158749176));
#44791=CARTESIAN_POINT('Ctrl Pts',(53.3069062974652,30.0571002854678,7.7803912457158));
#44792=CARTESIAN_POINT('Ctrl Pts',(53.2716065449753,29.9958331321701,7.78489090393984));
#44793=CARTESIAN_POINT('Ctrl Pts',(53.2367637564795,29.9353590972686,7.78933231297941));
#44794=CARTESIAN_POINT('Ctrl Pts',(53.2051025141465,29.8730610744932,7.79377372201899));
#44795=CARTESIAN_POINT('Ctrl Pts',(53.1768035530877,29.8093097543378,7.79821513105856));
#44796=CARTESIAN_POINT('Ctrl Pts',(53.1479478797148,29.7443042840779,7.80274391387483));
#44797=CARTESIAN_POINT('Ctrl Pts',(53.1225884276952,29.6777881994564,7.8072726966911));
#44798=CARTESIAN_POINT('Ctrl Pts',(53.1008648448833,29.6101747496414,7.81180147950737));
#44799=CARTESIAN_POINT('Ctrl Pts',(53.0791412620714,29.5425612998265,7.81633026232364));
#44800=CARTESIAN_POINT('Ctrl Pts',(53.0610536560262,29.47385101117,7.82085904513991));
#44801=CARTESIAN_POINT('Ctrl Pts',(53.0466869980082,29.4044698737233,7.82538782795619));
#44802=CARTESIAN_POINT('Origin',(55.,29.,3.45145488139523));
#44803=CARTESIAN_POINT('',(53.0466869980092,29.404469873728,8.78541210591381));
#44804=CARTESIAN_POINT('',(53.0466869433582,29.4044696098012,8.62635914573793));
#44805=CARTESIAN_POINT('',(53.0466869980082,29.4044698737233,3.45145488139523));
#44806=CARTESIAN_POINT('',(53.0052508354721,29.0012981434294,8.01095171076546));
#44807=CARTESIAN_POINT('Ctrl Pts',(53.0466869980092,29.404469873728,8.78541210591381));
#44808=CARTESIAN_POINT('Ctrl Pts',(53.0471763476454,29.4068330979609,8.78525791073123));
#44809=CARTESIAN_POINT('Ctrl Pts',(53.0476699849055,29.4091954287619,8.78510357909714));
#44810=CARTESIAN_POINT('Ctrl Pts',(53.0511509502984,29.4257041076768,8.78402369411619));
#44811=CARTESIAN_POINT('Ctrl Pts',(53.0542876510602,29.4398181929545,8.78309341089251));
#44812=CARTESIAN_POINT('Ctrl Pts',(53.0706602313561,29.5098836375005,8.77843926933478));
#44813=CARTESIAN_POINT('Ctrl Pts',(53.0861562499064,29.5652736190893,8.77464408487961));
#44814=CARTESIAN_POINT('Ctrl Pts',(53.1386457955463,29.7258108077838,8.76329370015989));
#44815=CARTESIAN_POINT('Ctrl Pts',(53.1820782395446,29.8286110184691,8.75555879578595));
#44816=CARTESIAN_POINT('Ctrl Pts',(53.2848874775335,30.0244355553964,8.74014342331277));
#44817=CARTESIAN_POINT('Ctrl Pts',(53.3438592282766,30.1172652160646,8.73249249321695));
#44818=CARTESIAN_POINT('Ctrl Pts',(53.4198655981057,30.2175632246231,8.72415558681927));
#44819=CARTESIAN_POINT('Ctrl Pts',(53.429709300766,30.2302325360583,8.72310133076771));
#44820=CARTESIAN_POINT('Ctrl Pts',(53.4437571326641,30.2478693836482,8.72163365224335));
#44821=CARTESIAN_POINT('Ctrl Pts',(53.4478340420646,30.2529368310685,8.7212119501624));
#44822=CARTESIAN_POINT('Ctrl Pts',(53.4544706607057,30.2611037946156,8.72053242764542));
#44823=CARTESIAN_POINT('Ctrl Pts',(53.4570150411808,30.2642156212326,8.72027353898543));
#44824=CARTESIAN_POINT('Ctrl Pts',(53.4624235911971,30.2707897307754,8.71972670203542));
#44825=CARTESIAN_POINT('Ctrl Pts',(53.4652900879389,30.2742500693926,8.71943892872029));
#44826=CARTESIAN_POINT('Ctrl Pts',(53.472427082998,30.282806592206,8.71872740219586));
#44827=CARTESIAN_POINT('Ctrl Pts',(53.4767114591822,30.2878912198545,8.71830463990576));
#44828=CARTESIAN_POINT('Ctrl Pts',(53.4928616384867,30.3068646491141,8.71672688384933));
#44829=CARTESIAN_POINT('Ctrl Pts',(53.5048930387663,30.3206121617782,8.71558327535639));
#44830=CARTESIAN_POINT('Ctrl Pts',(53.5358718030092,30.3550434879406,8.7127121709201));
#44831=CARTESIAN_POINT('Ctrl Pts',(53.5550701487517,30.3754970428994,8.71100013531827));
#44832=CARTESIAN_POINT('Ctrl Pts',(53.6451182525085,30.4674657971467,8.70323415030831));
#44833=CARTESIAN_POINT('Ctrl Pts',(53.7208909775005,30.5339633712613,8.69741896197683));
#44834=CARTESIAN_POINT('Ctrl Pts',(53.905846003979,30.6730032461,8.68398018520722));
#44835=CARTESIAN_POINT('Ctrl Pts',(54.0177801684663,30.7410776957544,8.67635212630113));
#44836=CARTESIAN_POINT('Ctrl Pts',(54.1575031152611,30.808264185645,8.66680788757141));
#44837=CARTESIAN_POINT('Ctrl Pts',(54.1796362301917,30.8184123766082,8.66529635302767));
#44838=CARTESIAN_POINT('Ctrl Pts',(54.2109273303359,30.8320720127476,8.66315733592696));
#44839=CARTESIAN_POINT('Ctrl Pts',(54.2199344553071,30.8359251832365,8.66254139067008));
#44840=CARTESIAN_POINT('Ctrl Pts',(54.2356327998561,30.842504421852,8.66146730473609));
#44841=CARTESIAN_POINT('Ctrl Pts',(54.2423111783236,30.8452607968761,8.66101019123223));
#44842=CARTESIAN_POINT('Ctrl Pts',(54.2562805984109,30.850937789961,8.66005358964875));
#44843=CARTESIAN_POINT('Ctrl Pts',(54.2635741977936,30.8538517431473,8.65955388812169));
#44844=CARTESIAN_POINT('Ctrl Pts',(54.280910485703,30.8606595198192,8.65836545713902));
#44845=CARTESIAN_POINT('Ctrl Pts',(54.2909677972855,30.8645151933663,8.65767547204381));
#44846=CARTESIAN_POINT('Ctrl Pts',(54.3248541483644,30.8771923918364,8.65534859114199));
#44847=CARTESIAN_POINT('Ctrl Pts',(54.3488195995829,30.8856397282705,8.65369944859847));
#44848=CARTESIAN_POINT('Ctrl Pts',(54.4064734948597,30.9047314058389,8.6497220334942));
#44849=CARTESIAN_POINT('Ctrl Pts',(54.4402952497117,30.9149427618275,8.64738057799504));
#44850=CARTESIAN_POINT('Ctrl Pts',(54.5736023822089,30.9513571563533,8.63811953590363));
#44851=CARTESIAN_POINT('Ctrl Pts',(54.6747737088761,30.9707443300508,8.6310108081723));
#44852=CARTESIAN_POINT('Ctrl Pts',(54.8996009405477,30.9960397037425,8.61525124741179));
#44853=CARTESIAN_POINT('Ctrl Pts',(55.0232507299588,30.9984291764641,8.60660599183199));
#44854=CARTESIAN_POINT('Ctrl Pts',(55.1620370968349,30.9882201509278,8.59739066796584));
#44855=CARTESIAN_POINT('Ctrl Pts',(55.1777235629555,30.9868794028054,8.59635645810611));
#44856=CARTESIAN_POINT('Ctrl Pts',(55.1998163590217,30.9847273452906,8.59491178287156));
#44857=CARTESIAN_POINT('Ctrl Pts',(55.2062366693476,30.9840704754294,8.59449337154652));
#44858=CARTESIAN_POINT('Ctrl Pts',(55.2170380221741,30.9829123787833,8.59379196755199));
#44859=CARTESIAN_POINT('Ctrl Pts',(55.2214207578804,30.9824277677278,8.59350806660202));
#44860=CARTESIAN_POINT('Ctrl Pts',(55.2303699059257,30.9814081876884,8.59292984374982));
#44861=CARTESIAN_POINT('Ctrl Pts',(55.2349361294475,30.9808719584848,8.59263559335114));
#44862=CARTESIAN_POINT('Ctrl Pts',(55.2465823859333,30.9794634565763,8.59188700574447));
#44863=CARTESIAN_POINT('Ctrl Pts',(55.2536597404976,30.9785689749672,8.59143389165318));
#44864=CARTESIAN_POINT('Ctrl Pts',(55.2825297241546,30.974762746517,8.58959233233629));
#44865=CARTESIAN_POINT('Ctrl Pts',(55.3042792422954,30.9715286421758,8.58822077327159));
#44866=CARTESIAN_POINT('Ctrl Pts',(55.3616778719469,30.9620210440397,8.5846324839403));
#44867=CARTESIAN_POINT('Ctrl Pts',(55.3972184337046,30.955135617987,8.58244280888315));
#44868=CARTESIAN_POINT('Ctrl Pts',(55.6113225591814,30.9075763184457,8.56934198057138));
#44869=CARTESIAN_POINT('Ctrl Pts',(55.7837735871049,30.8434395724339,8.55908946026871));
#44870=CARTESIAN_POINT('Ctrl Pts',(55.9908376815435,30.7320422013397,8.54494961267907));
#44871=CARTESIAN_POINT('Ctrl Pts',(56.0356303515982,30.7056372924828,8.54177499739736));
#44872=CARTESIAN_POINT('Ctrl Pts',(56.0915982838198,30.6696266903828,8.53762933017521));
#44873=CARTESIAN_POINT('Ctrl Pts',(56.1037712780878,30.6616043591768,8.53671643313224));
#44874=CARTESIAN_POINT('Ctrl Pts',(56.1230288067323,30.6486081293023,8.53525369715432));
#44875=CARTESIAN_POINT('Ctrl Pts',(56.1301709406775,30.6437202030156,8.53470707481664));
#44876=CARTESIAN_POINT('Ctrl Pts',(56.1429764983931,30.6348334315156,8.53371942137837));
#44877=CARTESIAN_POINT('Ctrl Pts',(56.1486513424993,30.6308512243852,8.53327902471101));
#44878=CARTESIAN_POINT('Ctrl Pts',(56.1619361021709,30.6214251762926,8.5322415958891));
#44879=CARTESIAN_POINT('Ctrl Pts',(56.169528651239,30.6159572509439,8.53164365092297));
#44880=CARTESIAN_POINT('Ctrl Pts',(56.1914974008431,30.5999000935571,8.52989864322451));
#44881=CARTESIAN_POINT('Ctrl Pts',(56.2057699407662,30.5891712246786,8.52874622329895));
#44882=CARTESIAN_POINT('Ctrl Pts',(56.336317558479,30.4882656098584,8.51802759356464));
#44883=CARTESIAN_POINT('Ctrl Pts',(56.4424020712778,30.385690937642,8.50794672681606));
#44884=CARTESIAN_POINT('Ctrl Pts',(56.5480120447472,30.2581842271216,8.4964171367295));
#44885=CARTESIAN_POINT('Ctrl Pts',(56.559597816621,30.2437939891989,8.49512942679026));
#44886=CARTESIAN_POINT('Ctrl Pts',(56.6007131482481,30.1912483620644,8.49047927739289));
#44887=CARTESIAN_POINT('Ctrl Pts',(56.6290566620034,30.1521848114466,8.48711877522837));
#44888=CARTESIAN_POINT('Ctrl Pts',(56.6705522976385,30.0903980712548,8.48198277974947));
#44889=CARTESIAN_POINT('Ctrl Pts',(56.6847193968599,30.0683789471376,8.48018593036477));
#44890=CARTESIAN_POINT('Ctrl Pts',(56.7211006445427,30.0093095509574,8.47546443273589));
#44891=CARTESIAN_POINT('Ctrl Pts',(56.7425533873057,29.9718032287985,8.47256663411431));
#44892=CARTESIAN_POINT('Ctrl Pts',(56.7667184417699,29.9261773979232,8.46918426654362));
#44893=CARTESIAN_POINT('Ctrl Pts',(56.7706167883617,29.9187027917944,8.46863462902968));
#44894=CARTESIAN_POINT('Ctrl Pts',(56.776924496986,29.9064192296812,8.46773895018348));
#44895=CARTESIAN_POINT('Ctrl Pts',(56.7793619556296,29.9016249333387,8.46739124256643));
#44896=CARTESIAN_POINT('Ctrl Pts',(56.7837137702428,29.8929788619906,8.46676763488132));
#44897=CARTESIAN_POINT('Ctrl Pts',(56.7856350756323,29.889130721446,8.46649131286668));
#44898=CARTESIAN_POINT('Ctrl Pts',(56.7898264203119,29.8806675861137,8.46588630089161));
#44899=CARTESIAN_POINT('Ctrl Pts',(56.7920910610675,29.8760500227428,8.46555794397369));
#44900=CARTESIAN_POINT('Ctrl Pts',(56.7985410065383,29.8627690190155,8.46461837391806));
#44901=CARTESIAN_POINT('Ctrl Pts',(56.8026815926539,29.854083846374,8.46400983650715));
#44902=CARTESIAN_POINT('Ctrl Pts',(56.8315050402309,29.7924811138403,8.45973275047185));
#44903=CARTESIAN_POINT('Ctrl Pts',(56.8539192818499,29.7385267260891,8.45618988373333));
#44904=CARTESIAN_POINT('Ctrl Pts',(56.9062500355181,29.5950866044397,8.44709999805547));
#44905=CARTESIAN_POINT('Ctrl Pts',(56.932245405664,29.5043279932132,8.44166691345847));
#44906=CARTESIAN_POINT('Ctrl Pts',(56.9787132256952,29.2842368042079,8.42858758735995));
#44907=CARTESIAN_POINT('Ctrl Pts',(56.9930751777289,29.1540825538138,8.42091109011923));
#44908=CARTESIAN_POINT('Ctrl Pts',(56.9947974714085,29.0076996463334,8.41182619130378));
#44909=CARTESIAN_POINT('Ctrl Pts',(56.9947960021885,28.9919300558255,8.41084206442606));
#44910=CARTESIAN_POINT('Ctrl Pts',(56.9944897664339,28.9663057357634,8.40923338300949));
#44911=CARTESIAN_POINT('Ctrl Pts',(56.99429890841,28.9564501413433,8.40861235782462));
#44912=CARTESIAN_POINT('Ctrl Pts',(56.9938284126205,28.9388822819454,8.40750110094649));
#44913=CARTESIAN_POINT('Ctrl Pts',(56.9935770518839,28.931169411457,8.40701175694995));
#44914=CARTESIAN_POINT('Ctrl Pts',(56.9929517391726,28.9148851690452,8.4059754212361));
#44915=CARTESIAN_POINT('Ctrl Pts',(56.9925672310889,28.906314382412,8.40542811109744));
#44916=CARTESIAN_POINT('Ctrl Pts',(56.9913976589648,28.8835285059193,8.40396797809907));
#44917=CARTESIAN_POINT('Ctrl Pts',(56.9905156941617,28.8693190945943,8.40305216454925));
#44918=CARTESIAN_POINT('Ctrl Pts',(56.9855071615004,28.8005419816199,8.39859302286931));
#44919=CARTESIAN_POINT('Ctrl Pts',(56.9792887277719,28.7461548352643,8.39498539362176));
#44920=CARTESIAN_POINT('Ctrl Pts',(56.9393896668113,28.4907673758662,8.37764757653191));
#44921=CARTESIAN_POINT('Ctrl Pts',(56.8772836977574,28.2954905515171,8.36305632880771));
#44922=CARTESIAN_POINT('Ctrl Pts',(56.7721120674023,28.0836361336892,8.34709360829288));
#44923=CARTESIAN_POINT('Ctrl Pts',(56.7568000917467,28.0546124354514,8.3449076875678));
#44924=CARTESIAN_POINT('Ctrl Pts',(56.7366419769971,28.0185857366959,8.34220743457325));
#44925=CARTESIAN_POINT('Ctrl Pts',(56.7324587430085,28.0112199322495,8.34165606389915));
#44926=CARTESIAN_POINT('Ctrl Pts',(56.725760404761,27.9995985716569,8.34078753395666));
#44927=CARTESIAN_POINT('Ctrl Pts',(56.7232762421965,27.9953254323746,8.3404684786106));
#44928=CARTESIAN_POINT('Ctrl Pts',(56.7188086205444,27.9877057637038,8.3399001526055));
#44929=CARTESIAN_POINT('Ctrl Pts',(56.716831268837,27.9843558253007,8.33965050553661));
#44930=CARTESIAN_POINT('Ctrl Pts',(56.7120756572793,27.9763526602667,8.33905457393747));
#44931=CARTESIAN_POINT('Ctrl Pts',(56.7092882235913,27.9717049534576,8.33870888604583));
#44932=CARTESIAN_POINT('Ctrl Pts',(56.7008048678788,27.9576897996132,8.33766746427776));
#44933=CARTESIAN_POINT('Ctrl Pts',(56.6950505187952,27.9483577110346,8.33697538272542));
#44934=CARTESIAN_POINT('Ctrl Pts',(56.6815677575474,27.9268903077562,8.3353853345737));
#44935=CARTESIAN_POINT('Ctrl Pts',(56.6737843309387,27.9147900784078,8.33449059586083));
#44936=CARTESIAN_POINT('Ctrl Pts',(56.6467398710512,27.8737296251712,8.33145577675558));
#44937=CARTESIAN_POINT('Ctrl Pts',(56.6268518324997,27.845188087313,8.32934853542777));
#44938=CARTESIAN_POINT('Ctrl Pts',(56.5101896246053,27.6867651009654,8.31757769673423));
#44939=CARTESIAN_POINT('Ctrl Pts',(56.3986247380188,27.5685273320437,8.30845360514863));
#44940=CARTESIAN_POINT('Ctrl Pts',(56.222803197247,27.4225958348863,8.29489106082445));
#44941=CARTESIAN_POINT('Ctrl Pts',(56.1695344379213,27.3827061366246,8.29087672061366));
#44942=CARTESIAN_POINT('Ctrl Pts',(56.0980470617953,27.3345547603204,8.28554138469478));
#44943=CARTESIAN_POINT('Ctrl Pts',(56.0815560081281,27.3237984146603,8.28431416109304));
#44944=CARTESIAN_POINT('Ctrl Pts',(56.0566836759589,27.3080952175748,8.28246714045477));
#44945=CARTESIAN_POINT('Ctrl Pts',(56.0484207110797,27.3029625251493,8.28185416932386));
#44946=CARTESIAN_POINT('Ctrl Pts',(56.0335478042022,27.2938740276097,8.28075182676299));
#44947=CARTESIAN_POINT('Ctrl Pts',(56.0269518233965,27.2898956619678,8.28026328863778));
#44948=CARTESIAN_POINT('Ctrl Pts',(56.0128954408432,27.2815282054937,8.27922282194575));
#44949=CARTESIAN_POINT('Ctrl Pts',(56.0054292015416,27.2771492811587,8.27867053928193));
#44950=CARTESIAN_POINT('Ctrl Pts',(55.9853076387526,27.2655233952203,8.27718300540029));
#44951=CARTESIAN_POINT('Ctrl Pts',(55.9726011414008,27.2583665033544,8.27624456233005));
#44952=CARTESIAN_POINT('Ctrl Pts',(55.9079798444097,27.2228964849301,8.27147557734829));
#44953=CARTESIAN_POINT('Ctrl Pts',(55.8549075095272,27.1967650584404,8.26756938521929));
#44954=CARTESIAN_POINT('Ctrl Pts',(55.6876709633612,27.1234655668044,8.25528528327806));
#44955=CARTESIAN_POINT('Ctrl Pts',(55.5702376308585,27.0845116853745,8.24667470788412));
#44956=CARTESIAN_POINT('Ctrl Pts',(55.401437341854,27.0454264671311,8.23460684890185));
#44957=CARTESIAN_POINT('Ctrl Pts',(55.3524953532946,27.0360099284948,8.23114633076581));
#44958=CARTESIAN_POINT('Ctrl Pts',(55.2485069064231,27.0200152378205,8.22392942381763));
#44959=CARTESIAN_POINT('Ctrl Pts',(55.1934305756995,27.0138778595804,8.22018606778666));
#44960=CARTESIAN_POINT('Ctrl Pts',(55.1291559800636,27.0094151981833,8.21595987885241));
#44961=CARTESIAN_POINT('Ctrl Pts',(55.1201423807294,27.0088508503753,8.21537047148527));
#44962=CARTESIAN_POINT('Ctrl Pts',(55.1055739511626,27.0080379988359,8.21442341772966));
#44963=CARTESIAN_POINT('Ctrl Pts',(55.1000214900196,27.0077514772047,8.21406377793684));
#44964=CARTESIAN_POINT('Ctrl Pts',(55.0901590856073,27.0072838865674,8.21342739056677));
#44965=CARTESIAN_POINT('Ctrl Pts',(55.0858496812303,27.0070935789836,8.21315014147792));
#44966=CARTESIAN_POINT('Ctrl Pts',(55.0765388023001,27.0067126590164,8.21255290892033));
#44967=CARTESIAN_POINT('Ctrl Pts',(55.0715372215094,27.0065268902636,8.21223319503527));
#44968=CARTESIAN_POINT('Ctrl Pts',(55.0575609893412,27.0060604532007,8.21134275398049));
#44969=CARTESIAN_POINT('Ctrl Pts',(55.0485849304879,27.0058215487369,8.21077428342502));
#44970=CARTESIAN_POINT('Ctrl Pts',(54.9952126091148,27.0047615893928,8.20741273008998));
#44971=CARTESIAN_POINT('Ctrl Pts',(54.9507969406287,27.0053624482015,8.20469178018524));
#44972=CARTESIAN_POINT('Ctrl Pts',(54.8005753961197,27.0124164654871,8.19563782833387));
#44973=CARTESIAN_POINT('Ctrl Pts',(54.6952727551984,27.0258158428439,8.18953468951974));
#44974=CARTESIAN_POINT('Ctrl Pts',(54.4602159764818,27.0749914084892,8.17557762138048));
#44975=CARTESIAN_POINT('Ctrl Pts',(54.3320297671583,27.1156343574414,8.16770877327091));
#44976=CARTESIAN_POINT('Ctrl Pts',(54.1944626067768,27.1750659146981,8.15840843936318));
#44977=CARTESIAN_POINT('Ctrl Pts',(54.180099703904,27.1814735662994,8.15742690382859));
#44978=CARTESIAN_POINT('Ctrl Pts',(54.1568717847352,27.1921672381511,8.15582162321066));
#44979=CARTESIAN_POINT('Ctrl Pts',(54.1479599190364,27.1963503175325,8.15520138250034));
#44980=CARTESIAN_POINT('Ctrl Pts',(54.1321195658418,27.203929109405,8.15409099906686));
#44981=CARTESIAN_POINT('Ctrl Pts',(54.1251790819601,27.2072993973665,8.15360173873721));
#44982=CARTESIAN_POINT('Ctrl Pts',(54.118152524075,27.2107620041935,8.15310357690825));
#44983=CARTESIAN_POINT('Ctrl Pts',(54.1180466490105,27.2108141898865,8.15309607002942));
#44984=CARTESIAN_POINT('Ctrl Pts',(54.1177887596464,27.2109413316997,8.15307778325715));
#44985=CARTESIAN_POINT('Ctrl Pts',(54.1176367502749,27.2110162977933,8.1530670030174));
#44986=CARTESIAN_POINT('Ctrl Pts',(54.1173457965148,27.211159832859,8.15304636649674));
#44987=CARTESIAN_POINT('Ctrl Pts',(54.117206850563,27.211228398645,8.15303651032698));
#44988=CARTESIAN_POINT('Ctrl Pts',(54.1169408917992,27.2113596800952,8.15301764230519));
#44989=CARTESIAN_POINT('Ctrl Pts',(54.1168138775863,27.2114223931455,8.15300863053929));
#44990=CARTESIAN_POINT('Ctrl Pts',(54.1165707474469,27.2115424704492,8.15299137844165));
#44991=CARTESIAN_POINT('Ctrl Pts',(54.1164546304108,27.2115998324896,8.15298313818617));
#44992=CARTESIAN_POINT('Ctrl Pts',(54.116232349553,27.2117096665957,8.15296736249361));
#44993=CARTESIAN_POINT('Ctrl Pts',(54.1161261847943,27.211762136818,8.15295982711954));
#44994=CARTESIAN_POINT('Ctrl Pts',(54.1159229451708,27.2118626072496,8.15294540029001));
#44995=CARTESIAN_POINT('Ctrl Pts',(54.1158258697616,27.2119106058016,8.15293850890411));
#44996=CARTESIAN_POINT('Ctrl Pts',(54.1156400217996,27.2120025164262,8.15292531449426));
#44997=CARTESIAN_POINT('Ctrl Pts',(54.1155512484882,27.2120464272644,8.15291901150686));
#44998=CARTESIAN_POINT('Ctrl Pts',(54.1153812861664,27.212130513197,8.15290694313924));
#44999=CARTESIAN_POINT('Ctrl Pts',(54.1153000965344,27.2121706872541,8.15290117779046));
#45000=CARTESIAN_POINT('Ctrl Pts',(54.1151446458352,27.2122476201745,8.15289013835576));
#45001=CARTESIAN_POINT('Ctrl Pts',(54.1150703843588,27.2122843781163,8.15288486430396));
#45002=CARTESIAN_POINT('Ctrl Pts',(54.1149281918077,27.212354771609,8.15287476516567));
#45003=CARTESIAN_POINT('Ctrl Pts',(54.1148602604231,27.2123884063735,8.15286994010999));
#45004=CARTESIAN_POINT('Ctrl Pts',(54.1147301823403,27.2124528209722,8.15286070035654));
#45005=CARTESIAN_POINT('Ctrl Pts',(54.114668035342,27.2124836001691,8.15285628568162));
#45006=CARTESIAN_POINT('Ctrl Pts',(54.1145490285704,27.2125425477173,8.15284783148068));
#45007=CARTESIAN_POINT('Ctrl Pts',(54.1144921683139,27.2125707156508,8.15284379195728));
#45008=CARTESIAN_POINT('Ctrl Pts',(54.1143832798162,27.2126246642626,8.15283605582754));
#45009=CARTESIAN_POINT('Ctrl Pts',(54.1143312516281,27.212650444365,8.15283235925588));
#45010=CARTESIAN_POINT('Ctrl Pts',(54.1141982389485,27.212716359727,8.1528229083778));
#45011=CARTESIAN_POINT('Ctrl Pts',(54.1141172559033,27.2127564982966,8.15281715394772));
#45012=CARTESIAN_POINT('Ctrl Pts',(54.1139568574756,27.2128360120172,8.15280575571763));
#45013=CARTESIAN_POINT('Ctrl Pts',(54.1138774419861,27.2128753869593,8.15280011192473));
#45014=CARTESIAN_POINT('Ctrl Pts',(54.1137201416349,27.2129533910067,8.15278893238084));
#45015=CARTESIAN_POINT('Ctrl Pts',(54.1136422566119,27.2129920199411,8.15278339663249));
#45016=CARTESIAN_POINT('Ctrl Pts',(54.1134879809048,27.2130685492242,8.15277243064033));
#45017=CARTESIAN_POINT('Ctrl Pts',(54.1134115901486,27.2131064493683,8.15276700040491));
#45018=CARTESIAN_POINT('Ctrl Pts',(54.1051878579613,27.2171871896666,8.15218237959018));
#45019=CARTESIAN_POINT('Ctrl Pts',(54.0970683729949,27.221285644437,8.15160126197576));
#45020=CARTESIAN_POINT('Ctrl Pts',(54.0739685122751,27.2331446351095,8.14993663567994));
#45021=CARTESIAN_POINT('Ctrl Pts',(54.0590584667462,27.2410397392601,8.1488484488452));
#45022=CARTESIAN_POINT('Ctrl Pts',(54.0256560441113,27.2592730805417,8.1463788285868));
#45023=CARTESIAN_POINT('Ctrl Pts',(54.0072248494119,27.2697185788375,8.1449937227598));
#45024=CARTESIAN_POINT('Ctrl Pts',(53.9485953074711,27.3041908283477,8.14051426695418));
#45025=CARTESIAN_POINT('Ctrl Pts',(53.9090777232144,27.3293388741704,8.13738175681123));
#45026=CARTESIAN_POINT('Ctrl Pts',(53.7076371806353,27.4677268950455,8.1208183630309));
#45027=CARTESIAN_POINT('Ctrl Pts',(53.5623375767471,27.6031548623208,8.10665155905615));
#45028=CARTESIAN_POINT('Ctrl Pts',(53.4251585275416,27.7754925464801,8.09193658266342));
#45029=CARTESIAN_POINT('Ctrl Pts',(53.4113076380329,27.7935171566382,8.09043381708143));
#45030=CARTESIAN_POINT('Ctrl Pts',(53.3933093289834,27.8177865439424,8.08846221613078));
#45031=CARTESIAN_POINT('Ctrl Pts',(53.3888852563978,27.8238227789836,8.08797601528031));
#45032=CARTESIAN_POINT('Ctrl Pts',(53.3817529677131,27.833669875875,8.08718980179458));
#45033=CARTESIAN_POINT('Ctrl Pts',(53.3790240423468,27.8374655438449,8.08688840760071));
#45034=CARTESIAN_POINT('Ctrl Pts',(53.373744935414,27.8448629939448,8.08630429009437));
#45035=CARTESIAN_POINT('Ctrl Pts',(53.3711933406214,27.848463676389,8.08602147639216));
#45036=CARTESIAN_POINT('Ctrl Pts',(53.3650617392373,27.857177439294,8.08534060854149));
#45037=CARTESIAN_POINT('Ctrl Pts',(53.3614937026915,27.8622989681191,8.08494336001744));
#45038=CARTESIAN_POINT('Ctrl Pts',(53.3491172110995,27.8802430701113,8.08356142502039));
#45039=CARTESIAN_POINT('Ctrl Pts',(53.3404344990017,27.8931522473017,8.08258477761368));
#45040=CARTESIAN_POINT('Ctrl Pts',(53.2881647674047,27.9728632955881,8.07665212271868));
#45041=CARTESIAN_POINT('Ctrl Pts',(53.2484610732735,28.0421357450481,8.07191177482973));
#45042=CARTESIAN_POINT('Ctrl Pts',(53.1555421411716,28.2294626789315,8.05966272425286));
#45043=CARTESIAN_POINT('Ctrl Pts',(53.1094790196468,28.3506288573462,8.05227533838761));
#45044=CARTESIAN_POINT('Ctrl Pts',(53.0620083681325,28.5247786913044,8.04153445069465));
#45045=CARTESIAN_POINT('Ctrl Pts',(53.0504549522644,28.5746526538862,8.03844809372298));
#45046=CARTESIAN_POINT('Ctrl Pts',(53.0358931407055,28.650712418942,8.0336899774711));
#45047=CARTESIAN_POINT('Ctrl Pts',(53.0314640679572,28.6766058846017,8.03206141837956));
#45048=CARTESIAN_POINT('Ctrl Pts',(53.0260399462113,28.7125777836419,8.02978374256859));
#45049=CARTESIAN_POINT('Ctrl Pts',(53.0246082386157,28.7225883789649,8.02914827043418));
#45050=CARTESIAN_POINT('Ctrl Pts',(53.0222734521298,28.7398488241723,8.02804960786271));
#45051=CARTESIAN_POINT('Ctrl Pts',(53.0213339623722,28.7470936108333,8.02758756357256));
#45052=CARTESIAN_POINT('Ctrl Pts',(53.0195267044595,28.7616569670688,8.02665689313479));
#45053=CARTESIAN_POINT('Ctrl Pts',(53.0186596562856,28.7689755084668,8.0261882522436));
#45054=CARTESIAN_POINT('Ctrl Pts',(53.0169832861877,28.7838294399719,8.02523509241176));
#45055=CARTESIAN_POINT('Ctrl Pts',(53.0161763134885,28.7913649681525,8.02475050811267));
#45056=CARTESIAN_POINT('Ctrl Pts',(53.0144150978591,28.8087462250547,8.02363031446452));
#45057=CARTESIAN_POINT('Ctrl Pts',(53.0134911172677,28.8185947546147,8.02299377249657));
#45058=CARTESIAN_POINT('Ctrl Pts',(53.010721092675,28.8506846536523,8.02091358617041));
#45059=CARTESIAN_POINT('Ctrl Pts',(53.0091751042848,28.8729495691398,8.01946071785727));
#45060=CARTESIAN_POINT('Ctrl Pts',(53.0061451499444,28.930560992448,8.01567552951475));
#45061=CARTESIAN_POINT('Ctrl Pts',(53.0052274032376,28.9659278090522,8.01332666869485));
#45062=CARTESIAN_POINT('Ctrl Pts',(53.0052504224343,29.0012981915817,8.01095242425188));
#45063=CARTESIAN_POINT('Ctrl Pts',(53.0052504239928,29.0013005840736,8.01095226365531));
#45064=CARTESIAN_POINT('Ctrl Pts',(53.0053388406021,29.1369081142874,8.00184957505844));
#45065=CARTESIAN_POINT('Ctrl Pts',(53.0192545284315,29.2719898001661,7.99237942723991));
#45066=CARTESIAN_POINT('Ctrl Pts',(53.0466869993245,29.4044698800804,7.98296685046478));
#45067=CARTESIAN_POINT('',(53.0052501027731,29.0006399384729,7.85153510469012));
#45068=CARTESIAN_POINT('Ctrl Pts',(53.0466869980082,29.4044698737233,7.82538782795619));
#45069=CARTESIAN_POINT('Ctrl Pts',(53.0325529122127,29.3362119011294,7.82984329733494));
#45070=CARTESIAN_POINT('Ctrl Pts',(53.0220201571551,29.2673051406182,7.83429876671369));
#45071=CARTESIAN_POINT('Ctrl Pts',(53.0151170648001,29.1981597740513,7.83875423609244));
#45072=CARTESIAN_POINT('Ctrl Pts',(53.0120643951503,29.1675824688255,7.84072452353009));
#45073=CARTESIAN_POINT('Ctrl Pts',(53.0097208440697,29.1369585167129,7.84269481096774));
#45074=CARTESIAN_POINT('Ctrl Pts',(53.0080856139562,29.1063232861218,7.84466509840538));
#45075=CARTESIAN_POINT('Ctrl Pts',(53.0062072319163,29.0711327239763,7.846928359402));
#45076=CARTESIAN_POINT('Ctrl Pts',(53.0052613253156,29.035891947952,7.84919162039861));
#45077=CARTESIAN_POINT('Ctrl Pts',(53.0052501010842,29.0006350396436,7.85145488139523));
#45078=CARTESIAN_POINT('Ctrl Pts',(53.0052501373994,29.0007403748082,7.85317985144906));
#45079=CARTESIAN_POINT('Ctrl Pts',(53.0051782706844,28.8071139598332,7.86510701368834));
#45080=CARTESIAN_POINT('Ctrl Pts',(53.0332974065051,28.6144740104776,7.87586527852367));
#45081=CARTESIAN_POINT('Ctrl Pts',(53.1028854012033,28.3816000185706,7.8902825160751));
#45082=CARTESIAN_POINT('Ctrl Pts',(53.1187615718485,28.3348655761312,7.8932454082853));
#45083=CARTESIAN_POINT('Ctrl Pts',(53.144185645828,28.2682464831858,7.89760280475556));
#45084=CARTESIAN_POINT('Ctrl Pts',(53.1523563722456,28.2478543390825,7.89895512368827));
#45085=CARTESIAN_POINT('Ctrl Pts',(53.1676432792812,28.2114550641497,7.90140513167815));
#45086=CARTESIAN_POINT('Ctrl Pts',(53.1746367592018,28.1953986847102,7.90249874781297));
#45087=CARTESIAN_POINT('Ctrl Pts',(53.1856602556443,28.1709734176104,7.90418312755723));
#45088=CARTESIAN_POINT('Ctrl Pts',(53.1895389310317,28.1625368692697,7.90476874941434));
#45089=CARTESIAN_POINT('Ctrl Pts',(53.1966988743869,28.1472454250324,7.90583733585362));
#45090=CARTESIAN_POINT('Ctrl Pts',(53.1999606997407,28.140381579019,7.90631962649599));
#45091=CARTESIAN_POINT('Ctrl Pts',(53.2071495128054,28.1254745252446,7.90737291391453));
#45092=CARTESIAN_POINT('Ctrl Pts',(53.2110915602217,28.117438803687,7.90794442285225));
#45093=CARTESIAN_POINT('Ctrl Pts',(53.2220131414629,28.0955493770993,7.90951159337613));
#45094=CARTESIAN_POINT('Ctrl Pts',(53.2291002934953,28.0817503577574,7.91051097372083));
#45095=CARTESIAN_POINT('Ctrl Pts',(53.267065447613,28.0099049663438,7.91577573055826));
#45096=CARTESIAN_POINT('Ctrl Pts',(53.3006353222276,27.9533346262717,7.92013508337376));
#45097=CARTESIAN_POINT('Ctrl Pts',(53.4216680174323,27.7705921592164,7.93495338316444));
#45098=CARTESIAN_POINT('Ctrl Pts',(53.5208794188734,27.6528665181079,7.94578731747667));
#45099=CARTESIAN_POINT('Ctrl Pts',(53.6655955949209,27.5166090843662,7.95949451744284));
#45100=CARTESIAN_POINT('Ctrl Pts',(53.6996621998492,27.4866573860359,7.96259124876788));
#45101=CARTESIAN_POINT('Ctrl Pts',(53.748040437147,27.4469637482342,7.96678347572212));
#45102=CARTESIAN_POINT('Ctrl Pts',(53.7615001675755,27.4362089158825,7.96792891741035));
#45103=CARTESIAN_POINT('Ctrl Pts',(53.7820324435844,27.4202342616527,7.96964291392799));
#45104=CARTESIAN_POINT('Ctrl Pts',(53.7890025832364,27.41488485604,7.97021908548508));
#45105=CARTESIAN_POINT('Ctrl Pts',(53.8004147631619,27.4062455110561,7.97115293232619));
#45106=CARTESIAN_POINT('Ctrl Pts',(53.8048354498848,27.4029277375999,7.97151237250194));
#45107=CARTESIAN_POINT('Ctrl Pts',(53.8133507818529,27.3965920456828,7.97220024909773));
#45108=CARTESIAN_POINT('Ctrl Pts',(53.817443286168,27.3935713352731,7.97252886980725));
#45109=CARTESIAN_POINT('Ctrl Pts',(53.8215671025125,27.3905518121983,7.97285798786338));
#45110=CARTESIAN_POINT('Ctrl Pts',(53.8215868514777,27.3905373522542,7.97285956396411));
#45111=CARTESIAN_POINT('Ctrl Pts',(53.8216264999087,27.3905083232925,7.97286272808345));
#45112=CARTESIAN_POINT('Ctrl Pts',(53.8216463995561,27.3904937541503,7.97286431611587));
#45113=CARTESIAN_POINT('Ctrl Pts',(53.8216863529331,27.3904645041958,7.97286750438227));
#45114=CARTESIAN_POINT('Ctrl Pts',(53.8217064060929,27.3904498238094,7.97286910457007));
#45115=CARTESIAN_POINT('Ctrl Pts',(53.8217466692585,27.3904203493695,7.97287231736561));
#45116=CARTESIAN_POINT('Ctrl Pts',(53.821766879252,27.3904055553339,7.97287392997161));
#45117=CARTESIAN_POINT('Ctrl Pts',(53.8218074584304,27.3903758519061,7.97287716778841));
#45118=CARTESIAN_POINT('Ctrl Pts',(53.8218278282283,27.3903609420743,7.97287879304737));
#45119=CARTESIAN_POINT('Ctrl Pts',(53.8218687300298,27.3903310048753,7.97288205640828));
#45120=CARTESIAN_POINT('Ctrl Pts',(53.8218892623325,27.3903159772987,7.97288369453331));
#45121=CARTESIAN_POINT('Ctrl Pts',(53.8219304931214,27.3902858017273,7.97288698394135));
#45122=CARTESIAN_POINT('Ctrl Pts',(53.8219511907179,27.3902706543934,7.97288863515258));
#45123=CARTESIAN_POINT('Ctrl Pts',(53.8219927549243,27.3902402372659,7.9728919509563));
#45124=CARTESIAN_POINT('Ctrl Pts',(53.8220136217205,27.3902249673459,7.97289361556285));
#45125=CARTESIAN_POINT('Ctrl Pts',(53.8220555274688,27.3901943027767,7.97289695840539));
#45126=CARTESIAN_POINT('Ctrl Pts',(53.822076566187,27.3901789083088,7.97289863662187));
#45127=CARTESIAN_POINT('Ctrl Pts',(53.8221188190231,27.3901479923014,7.97290200694048));
#45128=CARTESIAN_POINT('Ctrl Pts',(53.8221400331938,27.3901324707336,7.97290369904594));
#45129=CARTESIAN_POINT('Ctrl Pts',(53.8255303786376,27.3876519922626,7.97317411455021));
#45130=CARTESIAN_POINT('Ctrl Pts',(53.8289071945918,27.3851976494757,7.9734420951267));
#45131=CARTESIAN_POINT('Ctrl Pts',(53.8366602707974,27.3795996576406,7.97405429305732));
#45132=CARTESIAN_POINT('Ctrl Pts',(53.8410415739903,27.3764631314709,7.97439802400921));
#45133=CARTESIAN_POINT('Ctrl Pts',(53.8539702548244,27.3672866381343,7.97540597571461));
#45134=CARTESIAN_POINT('Ctrl Pts',(53.8625526759578,27.3612960319134,7.97606695682257));
#45135=CARTESIAN_POINT('Ctrl Pts',(53.9603845055397,27.2941474745379,7.98351481198376));
#45136=CARTESIAN_POINT('Ctrl Pts',(54.0544340146758,27.2402713392987,7.98986678760313));
#45137=CARTESIAN_POINT('Ctrl Pts',(54.2264966772028,27.1595055463054,8.00093123807221));
#45138=CARTESIAN_POINT('Ctrl Pts',(54.302661490933,27.1293193840149,8.00565499964381));
#45139=CARTESIAN_POINT('Ctrl Pts',(54.4614270214716,27.0774439892774,8.01547184908633));
#45140=CARTESIAN_POINT('Ctrl Pts',(54.5439930987406,27.0562053290519,8.02056280009881));
#45141=CARTESIAN_POINT('Ctrl Pts',(54.6488427362445,27.0362838424559,8.02715552292962));
#45142=CARTESIAN_POINT('Ctrl Pts',(54.6700910034197,27.0326025898979,8.02849769562327));
#45143=CARTESIAN_POINT('Ctrl Pts',(54.7013608619136,27.0277059045726,8.03048363336539));
#45144=CARTESIAN_POINT('Ctrl Pts',(54.7113391168775,27.0262208273878,8.03111894207711));
#45145=CARTESIAN_POINT('Ctrl Pts',(54.7289981545191,27.0237293799725,8.03224627515015));
#45146=CARTESIAN_POINT('Ctrl Pts',(54.7366743948,27.0226919342857,8.03273731493095));
#45147=CARTESIAN_POINT('Ctrl Pts',(54.7527468917203,27.0206149846569,8.03376762320148));
#45148=CARTESIAN_POINT('Ctrl Pts',(54.76114409241,27.0195841370265,8.0343071522992));
#45149=CARTESIAN_POINT('Ctrl Pts',(54.7831508070464,27.017024573152,8.03572446486952));
#45150=CARTESIAN_POINT('Ctrl Pts',(54.7967697666477,27.0155825608502,8.03660493527909));
#45151=CARTESIAN_POINT('Ctrl Pts',(54.8537843792192,27.0101387676742,8.04030565199234));
#45152=CARTESIAN_POINT('Ctrl Pts',(54.8972875809921,27.0074196620286,8.04316529798201));
#45153=CARTESIAN_POINT('Ctrl Pts',(55.1332879461497,27.0004175880705,8.05888325087212));
#45154=CARTESIAN_POINT('Ctrl Pts',(55.3255348008295,27.0226031035623,8.07255937847067));
#45155=CARTESIAN_POINT('Ctrl Pts',(55.5643239127779,27.0859609528477,8.08949010822986));
#45156=CARTESIAN_POINT('Ctrl Pts',(55.6164908244172,27.1021203445245,8.09317488126119));
#45157=CARTESIAN_POINT('Ctrl Pts',(55.6768580204353,27.1235724148032,8.09737285986934));
#45158=CARTESIAN_POINT('Ctrl Pts',(55.6857597994288,27.126807332844,8.09799016420973));
#45159=CARTESIAN_POINT('Ctrl Pts',(55.6994294318784,27.1318854012932,8.09893506296532));
#45160=CARTESIAN_POINT('Ctrl Pts',(55.7042136625355,27.1336836273054,8.099265191668));
#45161=CARTESIAN_POINT('Ctrl Pts',(55.7130130637199,27.1370296702158,8.09987124912225));
#45162=CARTESIAN_POINT('Ctrl Pts',(55.7170301215142,27.1385720846138,8.10014747970763));
#45163=CARTESIAN_POINT('Ctrl Pts',(55.7260928516315,27.1420855575564,8.1007696911307));
#45164=CARTESIAN_POINT('Ctrl Pts',(55.7311354977661,27.1440641740094,8.10111521839786));
#45165=CARTESIAN_POINT('Ctrl Pts',(55.7460216969471,27.1499752576161,8.10213339595545));
#45166=CARTESIAN_POINT('Ctrl Pts',(55.7558422175344,27.1539657442208,8.10280270760767));
#45167=CARTESIAN_POINT('Ctrl Pts',(55.8427970332698,27.1901093500087,8.10871176970505));
#45168=CARTESIAN_POINT('Ctrl Pts',(55.9178817307676,27.2270060179964,8.1136943467432));
#45169=CARTESIAN_POINT('Ctrl Pts',(56.0983340129353,27.3302273871267,8.12588862447967));
#45170=CARTESIAN_POINT('Ctrl Pts',(56.2002232800636,27.4018940580011,8.1329906044136));
#45171=CARTESIAN_POINT('Ctrl Pts',(56.3333811355945,27.5155145216936,8.14336211221535));
#45172=CARTESIAN_POINT('Ctrl Pts',(56.3707083773103,27.5499102157675,8.14640577215395));
#45173=CARTESIAN_POINT('Ctrl Pts',(56.4303251666695,27.6092054542406,8.15154095243316));
#45174=CARTESIAN_POINT('Ctrl Pts',(56.4533738396536,27.6333091666162,8.15360023647118));
#45175=CARTESIAN_POINT('Ctrl Pts',(56.4838602010689,27.6668346823559,8.15643386960506));
#45176=CARTESIAN_POINT('Ctrl Pts',(56.4918337919665,27.675763318839,8.1571856827259));
#45177=CARTESIAN_POINT('Ctrl Pts',(56.5050592631595,27.6908439383564,8.15845107151565));
#45178=CARTESIAN_POINT('Ctrl Pts',(56.5103550274791,27.69695715066,8.1589628209023));
#45179=CARTESIAN_POINT('Ctrl Pts',(56.5207072038393,27.7090551732024,8.15997331675761));
#45180=CARTESIAN_POINT('Ctrl Pts',(56.5257658269011,27.7150379055222,8.16047195982389));
#45181=CARTESIAN_POINT('Ctrl Pts',(56.5367973606769,27.7282416692045,8.16157020430357));
#45182=CARTESIAN_POINT('Ctrl Pts',(56.54275486851,27.735475270906,8.16217041239061));
#45183=CARTESIAN_POINT('Ctrl Pts',(56.5633658866787,27.7608636140096,8.16427214928182));
#45184=CARTESIAN_POINT('Ctrl Pts',(56.5777512214011,27.7792326650985,8.16578424756278));
#45185=CARTESIAN_POINT('Ctrl Pts',(56.6905762575426,27.9286283006916,8.17801926972722));
#45186=CARTESIAN_POINT('Ctrl Pts',(56.7728311074475,28.0710572120392,8.18937950248035));
#45187=CARTESIAN_POINT('Ctrl Pts',(56.8443473802909,28.2398741427858,8.20215400905679));
#45188=CARTESIAN_POINT('Ctrl Pts',(56.8516972908301,28.2579584033221,8.20351310807925));
#45189=CARTESIAN_POINT('Ctrl Pts',(56.8884387975637,28.3523069390134,8.21054817692882));
#45190=CARTESIAN_POINT('Ctrl Pts',(56.9133914526277,28.4302252225377,8.21617450750814));
#45191=CARTESIAN_POINT('Ctrl Pts',(56.9373653468214,28.5247202143254,8.22262746872963));
#45192=CARTESIAN_POINT('Ctrl Pts',(56.9410558390742,28.5400243177338,8.22366113555754));
#45193=CARTESIAN_POINT('Ctrl Pts',(56.9459627559037,28.5614845005892,8.22509314792217));
#45194=CARTESIAN_POINT('Ctrl Pts',(56.9473317915747,28.5676045945369,8.2254995597009));
#45195=CARTESIAN_POINT('Ctrl Pts',(56.9496161736368,28.5780475607388,8.2261895558984));
#45196=CARTESIAN_POINT('Ctrl Pts',(56.9505460546672,28.5823671761166,8.22647395165991));
#45197=CARTESIAN_POINT('Ctrl Pts',(56.9523103968837,28.5906975952653,8.22702041769142));
#45198=CARTESIAN_POINT('Ctrl Pts',(56.95314686131,28.5947079038648,8.22728260543257));
#45199=CARTESIAN_POINT('Ctrl Pts',(56.9551296247389,28.6043626834639,8.22791175668868));
#45200=CARTESIAN_POINT('Ctrl Pts',(56.9562638509619,28.6100096371196,8.22827804499206));
#45201=CARTESIAN_POINT('Ctrl Pts',(56.9603353697647,28.6307452221363,8.22961710770363));
#45202=CARTESIAN_POINT('Ctrl Pts',(56.963122772361,28.6458632082343,8.23058186394867));
#45203=CARTESIAN_POINT('Ctrl Pts',(56.9878907333125,28.7894886951186,8.2396511677492));
#45204=CARTESIAN_POINT('Ctrl Pts',(56.9974007269941,28.9198465826145,8.24716799285208));
#45205=CARTESIAN_POINT('Ctrl Pts',(56.9905243007948,29.1929210651952,8.26303145078461));
#45206=CARTESIAN_POINT('Ctrl Pts',(56.9716240657333,29.3348087673227,8.27136104388139));
#45207=CARTESIAN_POINT('Ctrl Pts',(56.9334254809607,29.4911467164158,8.28134020669378));
#45208=CARTESIAN_POINT('Ctrl Pts',(56.9288612492393,29.5087764092044,8.28247669939506));
#45209=CARTESIAN_POINT('Ctrl Pts',(56.9215682140005,29.5354363485407,8.28421340616306));
#45210=CARTESIAN_POINT('Ctrl Pts',(56.9190155971305,29.5445141113622,8.28480796249878));
#45211=CARTESIAN_POINT('Ctrl Pts',(56.91426781817,29.5609503041304,8.28589043878393));
#45212=CARTESIAN_POINT('Ctrl Pts',(56.9120943375698,29.5683148466648,8.28637764973094));
#45213=CARTESIAN_POINT('Ctrl Pts',(56.9073213796683,29.5841500013966,8.28743004810564));
#45214=CARTESIAN_POINT('Ctrl Pts',(56.9047078843137,29.5926161833357,8.28799568191869));
#45215=CARTESIAN_POINT('Ctrl Pts',(56.8974827864586,29.6154796364638,8.28953141865264));
#45216=CARTESIAN_POINT('Ctrl Pts',(56.8927638492993,29.6298421213637,8.29050499746797));
#45217=CARTESIAN_POINT('Ctrl Pts',(56.8684477982419,29.7011079648638,8.29538110489173));
#45218=CARTESIAN_POINT('Ctrl Pts',(56.8464475328608,29.7571524316037,8.29936170931126));
#45219=CARTESIAN_POINT('Ctrl Pts',(56.7668789019433,29.9356622739177,8.31252798930379));
#45220=CARTESIAN_POINT('Ctrl Pts',(56.6993879853999,30.0532795014724,8.32200452630818));
#45221=CARTESIAN_POINT('Ctrl Pts',(56.5724518816859,30.2301303946447,8.33713275703242));
#45222=CARTESIAN_POINT('Ctrl Pts',(56.5202624073695,30.2940752388877,8.34281079875641));
#45223=CARTESIAN_POINT('Ctrl Pts',(56.4535239264509,30.3662158224888,8.34931651813064));
#45224=CARTESIAN_POINT('Ctrl Pts',(56.4426504254366,30.3776927327135,8.35035466028569));
#45225=CARTESIAN_POINT('Ctrl Pts',(56.4272668962547,30.3935480726096,8.35179177111658));
#45226=CARTESIAN_POINT('Ctrl Pts',(56.4228712180596,30.3980359520426,8.35219888079509));
#45227=CARTESIAN_POINT('Ctrl Pts',(56.4153463240153,30.4056464299816,8.35288970286832));
#45228=CARTESIAN_POINT('Ctrl Pts',(56.4122278151736,30.4087795081299,8.35317423128276));
#45229=CARTESIAN_POINT('Ctrl Pts',(56.406201086132,30.4147942707852,8.35372066888673));
#45230=CARTESIAN_POINT('Ctrl Pts',(56.4032943918977,30.4176773870263,8.35398269715249));
#45231=CARTESIAN_POINT('Ctrl Pts',(56.3962839556397,30.4245882705351,8.35461108436352));
#45232=CARTESIAN_POINT('Ctrl Pts',(56.3921716057262,30.4286073104517,8.35497677170313));
#45233=CARTESIAN_POINT('Ctrl Pts',(56.3770535850464,30.4432550280401,8.35631072036938));
#45234=CARTESIAN_POINT('Ctrl Pts',(56.3659427783482,30.453775089757,8.35727104465866));
#45235=CARTESIAN_POINT('Ctrl Pts',(56.2580272130034,30.5536233367732,8.36642076633832));
#45236=CARTESIAN_POINT('Ctrl Pts',(56.1527053856061,30.6332967113054,8.37400961384961));
#45237=CARTESIAN_POINT('Ctrl Pts',(55.9191949633797,30.7760202801605,8.38990375442104));
#45238=CARTESIAN_POINT('Ctrl Pts',(55.7905725054278,30.8368874114338,8.39819027300954));
#45239=CARTESIAN_POINT('Ctrl Pts',(55.6396310435328,30.8895031706067,8.40810494080142));
#45240=CARTESIAN_POINT('Ctrl Pts',(55.6225937989777,30.8951852237519,8.40922600044863));
#45241=CARTESIAN_POINT('Ctrl Pts',(55.5965468996002,30.9034829415232,8.41094388654605));
#45242=CARTESIAN_POINT('Ctrl Pts',(55.5875913838737,30.9062664747814,8.41153524363983));
#45243=CARTESIAN_POINT('Ctrl Pts',(55.5719799154879,30.9109983339104,8.41256748137844));
#45244=CARTESIAN_POINT('Ctrl Pts',(55.5653327611299,30.9129753064665,8.4130074239507));
#45245=CARTESIAN_POINT('Ctrl Pts',(55.5503815434838,30.9173373109663,8.41399799979415));
#45246=CARTESIAN_POINT('Ctrl Pts',(55.5420720624937,30.9197031235706,8.41454924458674));
#45247=CARTESIAN_POINT('Ctrl Pts',(55.5197657845366,30.9258976240372,8.41603105598138));
#45248=CARTESIAN_POINT('Ctrl Pts',(55.5057423516452,30.929627628444,8.41696477198374));
#45249=CARTESIAN_POINT('Ctrl Pts',(55.4420046896465,30.9458382898341,8.4212190800153));
#45250=CARTESIAN_POINT('Ctrl Pts',(55.3918652237134,30.9565519815638,8.42459526557367));
#45251=CARTESIAN_POINT('Ctrl Pts',(55.1793604333108,30.9934636179582,8.43903673866605));
#45252=CARTESIAN_POINT('Ctrl Pts',(55.0145033397704,31.00146012583,8.45063049761431));
#45253=CARTESIAN_POINT('Ctrl Pts',(54.7847139521278,30.984197854818,8.46655766027285));
#45254=CARTESIAN_POINT('Ctrl Pts',(54.7191361735904,30.9759824025713,8.47106545127165));
#45255=CARTESIAN_POINT('Ctrl Pts',(54.6401264777183,30.9620701769926,8.47636372730492));
#45256=CARTESIAN_POINT('Ctrl Pts',(54.6261979584369,30.9594643126329,8.47729262712057));
#45257=CARTESIAN_POINT('Ctrl Pts',(54.6064000915318,30.9555415681116,8.47860452028953));
#45258=CARTESIAN_POINT('Ctrl Pts',(54.6005074787988,30.954346294883,8.47899392175048));
#45259=CARTESIAN_POINT('Ctrl Pts',(54.5903384198048,30.9522356610469,8.47966397008109));
#45260=CARTESIAN_POINT('Ctrl Pts',(54.5860594425998,30.9513328529467,8.47994531507664));
#45261=CARTESIAN_POINT('Ctrl Pts',(54.5771273880849,30.9494176031344,8.48053130959683));
#45262=CARTESIAN_POINT('Ctrl Pts',(54.5724749437298,30.9484025674189,8.48083581107727));
#45263=CARTESIAN_POINT('Ctrl Pts',(54.5601376171116,30.9456645834027,8.48164146642693));
#45264=CARTESIAN_POINT('Ctrl Pts',(54.5524591345759,30.9439127464125,8.48214101142094));
#45265=CARTESIAN_POINT('Ctrl Pts',(54.5195031495712,30.9361882527642,8.48427776483224));
#45266=CARTESIAN_POINT('Ctrl Pts',(54.4943319806861,30.929767389537,8.48589131101878));
#45267=CARTESIAN_POINT('Ctrl Pts',(54.265668734328,30.8666563805137,8.50043977111997));
#45268=CARTESIAN_POINT('Ctrl Pts',(54.0722446236612,30.7784666200613,8.51208338386741));
#45269=CARTESIAN_POINT('Ctrl Pts',(53.8658311991624,30.6413475328652,8.52696109766131));
#45270=CARTESIAN_POINT('Ctrl Pts',(53.8359810413947,30.620314853492,8.52917668332887));
#45271=CARTESIAN_POINT('Ctrl Pts',(53.7858427539271,30.5828862533135,8.53302383471036));
#45272=CARTESIAN_POINT('Ctrl Pts',(53.7652677474955,30.566889554619,8.5346406625211));
#45273=CARTESIAN_POINT('Ctrl Pts',(53.7365561871637,30.543650109021,8.53695483452359));
#45274=CARTESIAN_POINT('Ctrl Pts',(53.7281559159123,30.536736329232,8.53763913457046));
#45275=CARTESIAN_POINT('Ctrl Pts',(53.7137745989997,30.524701207848,8.53882343559457));
#45276=CARTESIAN_POINT('Ctrl Pts',(53.7077664875431,30.5196124840884,8.53932211146326));
#45277=CARTESIAN_POINT('Ctrl Pts',(53.6963210498624,30.5098015166555,8.54027969099137));
#45278=CARTESIAN_POINT('Ctrl Pts',(53.6908788511034,30.5050851271656,8.5407383501809));
#45279=CARTESIAN_POINT('Ctrl Pts',(53.6781644939301,30.4939453139193,8.54181783822952));
#45280=CARTESIAN_POINT('Ctrl Pts',(53.6709134773524,30.4874981398074,8.54243964487541));
#45281=CARTESIAN_POINT('Ctrl Pts',(53.6460419103465,30.4650567727477,8.54459415563102));
#45282=CARTESIAN_POINT('Ctrl Pts',(53.6286612793629,30.4488008449952,8.54613778460997));
#45283=CARTESIAN_POINT('Ctrl Pts',(53.5033168289792,30.3272908985036,8.55755804734225));
#45284=CARTESIAN_POINT('Ctrl Pts',(53.4073247155229,30.2104259018816,8.56796294142006));
#45285=CARTESIAN_POINT('Ctrl Pts',(53.2789883139807,30.0121510594262,8.58442438378906));
#45286=CARTESIAN_POINT('Ctrl Pts',(53.2372074337793,29.9374939929077,8.5903835927923));
#45287=CARTESIAN_POINT('Ctrl Pts',(53.1892904238783,29.8372663513482,8.59791292371472));
#45288=CARTESIAN_POINT('Ctrl Pts',(53.178684409554,29.8139371964776,8.5996335702745));
#45289=CARTESIAN_POINT('Ctrl Pts',(53.1617626335976,29.7747274758743,8.60246547242562));
#45290=CARTESIAN_POINT('Ctrl Pts',(53.155196321472,29.7589589656347,8.60358847458665));
#45291=CARTESIAN_POINT('Ctrl Pts',(53.1464203146975,29.737096914073,8.60512178486127));
#45292=CARTESIAN_POINT('Ctrl Pts',(53.1440367758686,29.7310745680028,8.60554171208159));
#45293=CARTESIAN_POINT('Ctrl Pts',(53.1400621261174,29.7208873306222,8.6062477850384));
#45294=CARTESIAN_POINT('Ctrl Pts',(53.1384555823467,29.7167285543304,8.60653483325504));
#45295=CARTESIAN_POINT('Ctrl Pts',(53.135415809442,29.7087804813747,8.60708110364233));
#45296=CARTESIAN_POINT('Ctrl Pts',(53.1339801667318,29.7049921680535,8.60734047321248));
#45297=CARTESIAN_POINT('Ctrl Pts',(53.130591985456,29.695968717672,8.6079559510489));
#45298=CARTESIAN_POINT('Ctrl Pts',(53.1286498690825,29.6907296650083,8.6083114480895));
#45299=CARTESIAN_POINT('Ctrl Pts',(53.1218496389619,29.6721461567782,8.60956611953298));
#45300=CARTESIAN_POINT('Ctrl Pts',(53.1171119072584,29.6587576882261,8.61045854341411));
#45301=CARTESIAN_POINT('Ctrl Pts',(53.085548406168,29.5664381857209,8.6165408732498));
#45302=CARTESIAN_POINT('Ctrl Pts',(53.0635683757526,29.4859954439104,8.62148610651734));
#45303=CARTESIAN_POINT('Ctrl Pts',(53.0466869433582,29.4044696098012,8.62635914573793));
#45304=CARTESIAN_POINT('Origin',(55.,29.,3.45145488139523));
#45305=CARTESIAN_POINT('',(53.0466870746609,29.4044702439035,9.58304844318572));
#45306=CARTESIAN_POINT('',(53.0466869980009,29.4044698736881,9.42363003822484));
#45307=CARTESIAN_POINT('',(53.0466869980082,29.4044698737233,3.45145488139523));
#45308=CARTESIAN_POINT('Ctrl Pts',(53.0466870746609,29.4044702439035,9.58304844318572));
#45309=CARTESIAN_POINT('Ctrl Pts',(53.0629212292667,29.4828700384529,9.57839245605286));
#45310=CARTESIAN_POINT('Ctrl Pts',(53.0838774118282,29.5603023718,9.57376218584092));
#45311=CARTESIAN_POINT('Ctrl Pts',(53.1356701680259,29.7141753006802,9.56420549992052));
#45312=CARTESIAN_POINT('Ctrl Pts',(53.1666475684883,29.7903092405455,9.55928854534223));
#45313=CARTESIAN_POINT('Ctrl Pts',(53.2113957035532,29.883385594677,9.5529062262179));
#45314=CARTESIAN_POINT('Ctrl Pts',(53.2208681939823,29.9023111447698,9.55158860919816));
#45315=CARTESIAN_POINT('Ctrl Pts',(53.2352630803224,29.9299631278263,9.5496322677227));
#45316=CARTESIAN_POINT('Ctrl Pts',(53.2399531662748,29.9388093267766,9.54900163708479));
#45317=CARTESIAN_POINT('Ctrl Pts',(53.24838463308,29.9544270610249,9.54787960314639));
#45318=CARTESIAN_POINT('Ctrl Pts',(53.2520992072219,29.9612128922966,9.54738915261613));
#45319=CARTESIAN_POINT('Ctrl Pts',(53.2599765092736,29.9754065907911,9.54635703633499));
#45320=CARTESIAN_POINT('Ctrl Pts',(53.2641472788581,29.9828097946619,9.54581509173274));
#45321=CARTESIAN_POINT('Ctrl Pts',(53.2752467853263,30.0022205835238,9.54438448735879));
#45322=CARTESIAN_POINT('Ctrl Pts',(53.2822535229024,30.0141828109329,9.54349304772926));
#45323=CARTESIAN_POINT('Ctrl Pts',(53.3125670569246,30.0647200738163,9.53968431760354));
#45324=CARTESIAN_POINT('Ctrl Pts',(53.337051374791,30.1025697731689,9.53672470203159));
#45325=CARTESIAN_POINT('Ctrl Pts',(53.4793766827536,30.3070492585799,9.52012015679283));
#45326=CARTESIAN_POINT('Ctrl Pts',(53.6209374607404,30.4556209856089,9.5055500372503));
#45327=CARTESIAN_POINT('Ctrl Pts',(53.8049502178952,30.5973991208908,9.48975803476037));
#45328=CARTESIAN_POINT('Ctrl Pts',(53.8277266589832,30.6141881280966,9.48785309992596));
#45329=CARTESIAN_POINT('Ctrl Pts',(53.8658806446695,30.641078555526,9.4847525087568));
#45330=CARTESIAN_POINT('Ctrl Pts',(53.8810539581841,30.6514615801605,9.48354225619057));
#45331=CARTESIAN_POINT('Ctrl Pts',(53.9005940195775,30.6644397780509,9.48201470661506));
#45332=CARTESIAN_POINT('Ctrl Pts',(53.9048294970119,30.6672296948135,9.48168542930842));
#45333=CARTESIAN_POINT('Ctrl Pts',(53.9125030206562,30.6722423993857,9.48109223830474));
#45334=CARTESIAN_POINT('Ctrl Pts',(53.9159373393983,30.6744708032694,9.48082796475142));
#45335=CARTESIAN_POINT('Ctrl Pts',(53.9229247533851,30.6789741734083,9.48029277248145));
#45336=CARTESIAN_POINT('Ctrl Pts',(53.9264781750549,30.6812484212234,9.48002191153501));
#45337=CARTESIAN_POINT('Ctrl Pts',(53.9344251950867,30.6862991753266,9.47941904525199));
#45338=CARTESIAN_POINT('Ctrl Pts',(53.9388224347124,30.689069788366,9.47908742618165));
#45339=CARTESIAN_POINT('Ctrl Pts',(53.9515909899784,30.6970454559404,9.47812998829549));
#45340=CARTESIAN_POINT('Ctrl Pts',(53.959990264535,30.7022057723218,9.47750699795683));
#45341=CARTESIAN_POINT('Ctrl Pts',(54.0166935315869,30.7364665317156,9.4733444223246));
#45342=CARTESIAN_POINT('Ctrl Pts',(54.0661793172897,30.7635724605396,9.46992092134261));
#45343=CARTESIAN_POINT('Ctrl Pts',(54.228078004946,30.8435237755441,9.45916231017186));
#45344=CARTESIAN_POINT('Ctrl Pts',(54.3442983029437,30.8879888685677,9.45207861607605));
#45345=CARTESIAN_POINT('Ctrl Pts',(54.5303026463826,30.939887633603,9.44077206145705));
#45346=CARTESIAN_POINT('Ctrl Pts',(54.5976126791062,30.9549585551151,9.43668973088029));
#45347=CARTESIAN_POINT('Ctrl Pts',(54.7064041304362,30.9734602029374,9.42999577090137));
#45348=CARTESIAN_POINT('Ctrl Pts',(54.7474481387295,30.9791313482567,9.42744941846956));
#45349=CARTESIAN_POINT('Ctrl Pts',(54.8015270885474,30.9848939797551,9.42405381788397));
#45350=CARTESIAN_POINT('Ctrl Pts',(54.8144301621943,30.9861418454432,9.42324065041736));
#45351=CARTESIAN_POINT('Ctrl Pts',(54.8356131613484,30.9879822486269,9.42190039560307));
#45352=CARTESIAN_POINT('Ctrl Pts',(54.843886377314,30.9886490356598,9.42137562978404));
#45353=CARTESIAN_POINT('Ctrl Pts',(54.859944694503,30.9898424451795,9.42035440274547));
#45354=CARTESIAN_POINT('Ctrl Pts',(54.867729209144,30.9903750602085,9.41985813790678));
#45355=CARTESIAN_POINT('Ctrl Pts',(54.8857819108956,30.991503848869,9.41870438085794));
#45356=CARTESIAN_POINT('Ctrl Pts',(54.8960519117186,30.9920662991893,9.41804585208336));
#45357=CARTESIAN_POINT('Ctrl Pts',(54.9295570385912,30.9936414527312,9.41589013576712));
#45358=CARTESIAN_POINT('Ctrl Pts',(54.9528049011314,30.9943272048731,9.4143828805405));
#45359=CARTESIAN_POINT('Ctrl Pts',(55.1406846059619,30.9965823330495,9.40210430218785));
#45360=CARTESIAN_POINT('Ctrl Pts',(55.3048925877464,30.9781690635832,9.39068893716648));
#45361=CARTESIAN_POINT('Ctrl Pts',(55.5388543884596,30.9220930204886,9.37392638300965));
#45362=CARTESIAN_POINT('Ctrl Pts',(55.6117060589764,30.9001638817124,9.36864617136044));
#45363=CARTESIAN_POINT('Ctrl Pts',(55.7056143148866,30.865933709072,9.36188596900769));
#45364=CARTESIAN_POINT('Ctrl Pts',(55.7279482970938,30.8573345285957,9.36028199566582));
#45365=CARTESIAN_POINT('Ctrl Pts',(55.7651573987638,30.8422336916814,9.35762217847848));
#45366=CARTESIAN_POINT('Ctrl Pts',(55.7801172487516,30.8359487841865,9.35655624473106));
#45367=CARTESIAN_POINT('Ctrl Pts',(55.8008204191682,30.8269522442517,9.35508752981595));
#45368=CARTESIAN_POINT('Ctrl Pts',(55.8066295229105,30.8243948755541,9.35467613621507));
#45369=CARTESIAN_POINT('Ctrl Pts',(55.8164749123956,30.8200043762972,9.35398023363882));
#45370=CARTESIAN_POINT('Ctrl Pts',(55.8205174463477,30.8181854509298,9.35369487987156));
#45371=CARTESIAN_POINT('Ctrl Pts',(55.8282679723809,30.8146670121401,9.35314857123481));
#45372=CARTESIAN_POINT('Ctrl Pts',(55.8319768426479,30.8129695896632,9.35288748758152));
#45373=CARTESIAN_POINT('Ctrl Pts',(55.8408497350366,30.8088758095767,9.35226364557963));
#45374=CARTESIAN_POINT('Ctrl Pts',(55.8460087911326,30.8064686818755,9.35190153746928));
#45375=CARTESIAN_POINT('Ctrl Pts',(55.8646053839787,30.797694688492,9.35059825280139));
#45376=CARTESIAN_POINT('Ctrl Pts',(55.8779823247171,30.791199522991,9.34966453411634));
#45377=CARTESIAN_POINT('Ctrl Pts',(56.0161332342461,30.7222008432487,9.34004797304366));
#45378=CARTESIAN_POINT('Ctrl Pts',(56.1341114986657,30.6469077318902,9.33204302059598));
#45379=CARTESIAN_POINT('Ctrl Pts',(56.3484976829093,30.4760375574891,9.31611203851446));
#45380=CARTESIAN_POINT('Ctrl Pts',(56.4449508762514,30.3817536447246,9.30822576688206));
#45381=CARTESIAN_POINT('Ctrl Pts',(56.5427263751081,30.2646531941541,9.29876432214763));
#45382=CARTESIAN_POINT('Ctrl Pts',(56.5540890891429,30.2506635998045,9.29763939155595));
#45383=CARTESIAN_POINT('Ctrl Pts',(56.5710818667813,30.2291531735158,9.29591678305528));
#45384=CARTESIAN_POINT('Ctrl Pts',(56.5768511337334,30.221743120833,9.2953246214681));
#45385=CARTESIAN_POINT('Ctrl Pts',(56.5867902383234,30.208789648711,9.29429149451994));
#45386=CARTESIAN_POINT('Ctrl Pts',(56.5909839175347,30.2032646622589,9.29385147247178));
#45387=CARTESIAN_POINT('Ctrl Pts',(56.6003309557442,30.1908160593666,9.29286138837444));
#45388=CARTESIAN_POINT('Ctrl Pts',(56.6054683415163,30.1838806762978,9.29231071880553));
#45389=CARTESIAN_POINT('Ctrl Pts',(56.6190983177958,30.1652285625857,9.29083207970321));
#45390=CARTESIAN_POINT('Ctrl Pts',(56.6275085622282,30.1534525683509,9.28990098420736));
#45391=CARTESIAN_POINT('Ctrl Pts',(56.6648605689016,30.0999305291931,9.28567923959813));
#45392=CARTESIAN_POINT('Ctrl Pts',(56.6923272344461,30.0571828835495,9.28233404890007));
#45393=CARTESIAN_POINT('Ctrl Pts',(56.8118328617738,29.8545789071831,9.26658961948357));
#45394=CARTESIAN_POINT('Ctrl Pts',(56.8830435181873,29.6834994285822,9.25349149439364));
#45395=CARTESIAN_POINT('Ctrl Pts',(56.9434004817155,29.4529179469108,9.23716295247995));
#45396=CARTESIAN_POINT('Ctrl Pts',(56.9549436670145,29.4001705817781,9.23352106089846));
#45397=CARTESIAN_POINT('Ctrl Pts',(56.9659771044791,29.3377140769954,9.22936535192815));
#45398=CARTESIAN_POINT('Ctrl Pts',(56.9675541780455,29.3284011845437,9.22874975632469));
#45399=CARTESIAN_POINT('Ctrl Pts',(56.9698817329363,29.3140375549769,9.22780691257717));
#45400=CARTESIAN_POINT('Ctrl Pts',(56.9706790464509,29.3089947005647,9.22747714697915));
#45401=CARTESIAN_POINT('Ctrl Pts',(56.9721127335726,29.2996955924127,9.22687143008134));
#45402=CARTESIAN_POINT('Ctrl Pts',(56.9727546926228,29.2954403584541,9.22659517948702));
#45403=CARTESIAN_POINT('Ctrl Pts',(56.9741746188858,29.2858173423959,9.22597251457005));
#45404=CARTESIAN_POINT('Ctrl Pts',(56.9749444666062,29.2804484525763,9.22562655678444));
#45405=CARTESIAN_POINT('Ctrl Pts',(56.977158581962,29.2645459225875,9.22460592192089));
#45406=CARTESIAN_POINT('Ctrl Pts',(56.9785405690673,29.2540036055051,9.22393460748502));
#45407=CARTESIAN_POINT('Ctrl Pts',(56.9912663811667,29.1505121268705,9.21739194519921));
#45408=CARTESIAN_POINT('Ctrl Pts',(56.9961377890792,29.0568712389921,9.21184452678314));
#45409=CARTESIAN_POINT('Ctrl Pts',(56.9936514464864,28.922034796767,9.20396415077414));
#45410=CARTESIAN_POINT('Ctrl Pts',(56.9916161515464,28.8808788626741,9.20157371489591));
#45411=CARTESIAN_POINT('Ctrl Pts',(56.9766394036156,28.6949787911995,9.19074375865892));
#45412=CARTESIAN_POINT('Ctrl Pts',(56.949183164245,28.551871666362,9.18227746006094));
#45413=CARTESIAN_POINT('Ctrl Pts',(56.9010420998777,28.3955150138639,9.17213446920513));
#45414=CARTESIAN_POINT('Ctrl Pts',(56.8954106222268,28.3780822382142,9.17099128851613));
#45415=CARTESIAN_POINT('Ctrl Pts',(56.8865107930642,28.3517763246286,9.16924643044634));
#45416=CARTESIAN_POINT('Ctrl Pts',(56.8834180435864,28.34284448277,9.16865049335632));
#45417=CARTESIAN_POINT('Ctrl Pts',(56.8776975571026,28.3266958869117,9.1675665560186));
#45418=CARTESIAN_POINT('Ctrl Pts',(56.8750913852583,28.3194716472468,9.16707927411058));
#45419=CARTESIAN_POINT('Ctrl Pts',(56.8693946274083,28.3039615709289,9.16602790803968));
#45420=CARTESIAN_POINT('Ctrl Pts',(56.866290537898,28.2956809020408,9.16546338501665));
#45421=CARTESIAN_POINT('Ctrl Pts',(56.8577576501786,28.2733705366715,9.1639335761702));
#45422=CARTESIAN_POINT('Ctrl Pts',(56.8522251245152,28.2593813859716,9.16296485945009));
#45423=CARTESIAN_POINT('Ctrl Pts',(56.8240849595031,28.1905161748066,9.15814797679511));
#45424=CARTESIAN_POINT('Ctrl Pts',(56.7991962943826,28.1366104644012,9.15422397637789));
#45425=CARTESIAN_POINT('Ctrl Pts',(56.7095932397148,27.9632982234795,9.14108762670742));
#45426=CARTESIAN_POINT('Ctrl Pts',(56.6350982025969,27.8493890358803,9.13157789411601));
#45427=CARTESIAN_POINT('Ctrl Pts',(56.497444818211,27.6795628040207,9.1163843632431));
#45428=CARTESIAN_POINT('Ctrl Pts',(56.4412946946562,27.6184907503992,9.11067607143012));
#45429=CARTESIAN_POINT('Ctrl Pts',(56.3700705436731,27.5501084800544,9.1041395129003));
#45430=CARTESIAN_POINT('Ctrl Pts',(56.3585079060432,27.5392690113728,9.10309876626112));
#45431=CARTESIAN_POINT('Ctrl Pts',(56.3421785383655,27.5243225716828,9.10165868930248));
#45432=CARTESIAN_POINT('Ctrl Pts',(56.3375200650745,27.5200989291875,9.101251174327));
#45433=CARTESIAN_POINT('Ctrl Pts',(56.3295519149469,27.5129428999809,9.10055987224279));
#45434=CARTESIAN_POINT('Ctrl Pts',(56.326252339191,27.5099993800346,9.1002752663979));
#45435=CARTESIAN_POINT('Ctrl Pts',(56.3198799655207,27.5043525857226,9.09972884389562));
#45436=CARTESIAN_POINT('Ctrl Pts',(56.3168086168745,27.5016477789005,9.09946690723354));
#45437=CARTESIAN_POINT('Ctrl Pts',(56.3094061995396,27.4951691236515,9.09883895978292));
#45438=CARTESIAN_POINT('Ctrl Pts',(56.3050670808205,27.4914044682882,9.09847361852502));
#45439=CARTESIAN_POINT('Ctrl Pts',(56.2891436535107,27.4777092883983,9.09714265504694));
#45440=CARTESIAN_POINT('Ctrl Pts',(56.277461426206,27.4678927232152,9.09618492255271));
#45441=CARTESIAN_POINT('Ctrl Pts',(56.1630081960595,27.3739371336043,9.08696887568781));
#45442=CARTESIAN_POINT('Ctrl Pts',(56.0521734604722,27.3001148163087,9.07932152273101));
#45443=CARTESIAN_POINT('Ctrl Pts',(55.8108853689013,27.1721129183092,9.06345755135915));
#45444=CARTESIAN_POINT('Ctrl Pts',(55.6803915945405,27.1196365957924,9.05526242006114));
#45445=CARTESIAN_POINT('Ctrl Pts',(55.5278628728143,27.0762734427691,9.04543107533549));
#45446=CARTESIAN_POINT('Ctrl Pts',(55.5101762476722,27.0715075211143,9.04428803631034));
#45447=CARTESIAN_POINT('Ctrl Pts',(55.4832677859087,27.0646527071757,9.04254335086274));
#45448=CARTESIAN_POINT('Ctrl Pts',(55.4740922901799,27.0623846118992,9.04194744297643));
#45449=CARTESIAN_POINT('Ctrl Pts',(55.4574326851246,27.0583919337905,9.04086353658711));
#45450=CARTESIAN_POINT('Ctrl Pts',(55.4499540352015,27.0566451925302,9.04037625622628));
#45451=CARTESIAN_POINT('Ctrl Pts',(55.4338421475247,27.0529800296137,9.03932486855463));
#45452=CARTESIAN_POINT('Ctrl Pts',(55.4252058922145,27.0510757533583,9.03876032222565));
#45453=CARTESIAN_POINT('Ctrl Pts',(55.4018441987151,27.0460872203015,9.03723038907686));
#45454=CARTESIAN_POINT('Ctrl Pts',(55.3870962961026,27.0431120758194,9.03626157041945));
#45455=CARTESIAN_POINT('Ctrl Pts',(55.3139888127193,27.0292226143452,9.03144322658926));
#45456=CARTESIAN_POINT('Ctrl Pts',(55.2552010981877,27.0207517412582,9.02751781095116));
#45457=CARTESIAN_POINT('Ctrl Pts',(55.0377957239877,26.9992719234312,9.01280849003101));
#45458=CARTESIAN_POINT('Ctrl Pts',(54.8781700891338,27.0026298796944,9.001577538853));
#45459=CARTESIAN_POINT('Ctrl Pts',(54.6746889918854,27.0314073877667,8.98739629280573));
#45460=CARTESIAN_POINT('Ctrl Pts',(54.6289457058607,27.0395144981569,8.98422244072869));
#45461=CARTESIAN_POINT('Ctrl Pts',(54.5664066301552,27.0528660229284,8.97993653281451));
#45462=CARTESIAN_POINT('Ctrl Pts',(54.549337081132,27.0567457927715,8.97877230523381));
#45463=CARTESIAN_POINT('Ctrl Pts',(54.5199010625942,27.0638451045723,8.97677679019698));
#45464=CARTESIAN_POINT('Ctrl Pts',(54.5075105980079,27.0669596543449,8.97594057998621));
#45465=CARTESIAN_POINT('Ctrl Pts',(54.4895722407362,27.0716524400323,8.97473626008998));
#45466=CARTESIAN_POINT('Ctrl Pts',(54.4840002167434,27.0731359583144,8.97436306108693));
#45467=CARTESIAN_POINT('Ctrl Pts',(54.4742487945974,27.0757775493957,8.97371158889935));
#45468=CARTESIAN_POINT('Ctrl Pts',(54.4700666369413,27.0769251180672,8.97343272458887));
#45469=CARTESIAN_POINT('Ctrl Pts',(54.4611865952873,27.0793929373537,8.97284177624467));
#45470=CARTESIAN_POINT('Ctrl Pts',(54.4564898013933,27.0807167901991,8.97252990126463));
#45471=CARTESIAN_POINT('Ctrl Pts',(54.4437141380367,27.0843684364214,8.9716833291817));
#45472=CARTESIAN_POINT('Ctrl Pts',(54.4356449427866,27.0867301228209,8.97115054192122));
#45473=CARTESIAN_POINT('Ctrl Pts',(54.3978378163487,27.098055484479,8.9686621881177));
#45474=CARTESIAN_POINT('Ctrl Pts',(54.3682951677902,27.1076624275052,8.96674091714015));
#45475=CARTESIAN_POINT('Ctrl Pts',(54.1450040832168,27.1860868897679,8.95231171174125));
#45476=CARTESIAN_POINT('Ctrl Pts',(53.9627047528751,27.2838012642721,8.94094279944695));
#45477=CARTESIAN_POINT('Ctrl Pts',(53.7547391584642,27.4407168242663,8.92529714442832));
#45478=CARTESIAN_POINT('Ctrl Pts',(53.712322075242,27.4755580267179,8.9219483000231));
#45479=CARTESIAN_POINT('Ctrl Pts',(53.6607691719418,27.5215916038688,8.91764106516368));
#45480=CARTESIAN_POINT('Ctrl Pts',(53.6502429534061,27.5311955558391,8.91674850352265));
#45481=CARTESIAN_POINT('Ctrl Pts',(53.6335432045502,27.5467632533205,8.91531076752127));
#45482=CARTESIAN_POINT('Ctrl Pts',(53.6273035817171,27.5526556196751,8.91476861785809));
#45483=CARTESIAN_POINT('Ctrl Pts',(53.6155263387598,27.5639220817934,8.91373572470794));
#45484=CARTESIAN_POINT('Ctrl Pts',(53.6099814860972,27.5692884168674,8.91324532009406));
#45485=CARTESIAN_POINT('Ctrl Pts',(53.5974279708174,27.5815796324077,8.91212555587818));
#45486=CARTESIAN_POINT('Ctrl Pts',(53.5904392408955,27.5885244965228,8.91149533122864));
#45487=CARTESIAN_POINT('Ctrl Pts',(53.5724106732602,27.6067073380958,8.90985149323946));
#45488=CARTESIAN_POINT('Ctrl Pts',(53.5614521754252,27.6180246527265,8.90883438802049));
#45489=CARTESIAN_POINT('Ctrl Pts',(53.4603658985925,27.7249260258943,8.89928083086915));
#45490=CARTESIAN_POINT('Ctrl Pts',(53.3797701644002,27.8290472370523,8.89033949761056));
#45491=CARTESIAN_POINT('Ctrl Pts',(53.2591067995655,28.021482104707,8.87456353198744));
#45492=CARTESIAN_POINT('Ctrl Pts',(53.2141242439784,28.1062132515969,8.86784241256776));
#45493=CARTESIAN_POINT('Ctrl Pts',(53.1526417335254,28.2453693657681,8.85740620544516));
#45494=CARTESIAN_POINT('Ctrl Pts',(53.1320690747568,28.2978352851099,8.8536001271766));
#45495=CARTESIAN_POINT('Ctrl Pts',(53.1106392407729,28.3601292878444,8.84928286212643));
#45496=CARTESIAN_POINT('Ctrl Pts',(53.1076000202736,28.3691744043055,8.84866088495536));
#45497=CARTESIAN_POINT('Ctrl Pts',(53.103027987653,28.3831118231407,8.84771036809934));
#45498=CARTESIAN_POINT('Ctrl Pts',(53.1014489843403,28.3879886596338,8.84737924785006));
#45499=CARTESIAN_POINT('Ctrl Pts',(53.098579380892,28.3969695698789,8.84677225421259));
#45500=CARTESIAN_POINT('Ctrl Pts',(53.0972832621853,28.4010717182088,8.84649607207644));
#45501=CARTESIAN_POINT('Ctrl Pts',(53.0943906109038,28.4103309728315,8.84587507196094));
#45502=CARTESIAN_POINT('Ctrl Pts',(53.0928017385375,28.4154903777272,8.84553069958124));
#45503=CARTESIAN_POINT('Ctrl Pts',(53.0881802769191,28.4307167257565,8.84451910270566));
#45504=CARTESIAN_POINT('Ctrl Pts',(53.0852062528604,28.4408014510849,8.84385515297177));
#45505=CARTESIAN_POINT('Ctrl Pts',(53.0607663816614,28.5261572256575,8.83828286711351));
#45506=CARTESIAN_POINT('Ctrl Pts',(53.0436656390178,28.6026174969733,8.83359987630482));
#45507=CARTESIAN_POINT('Ctrl Pts',(53.0139813176481,28.7851986005292,8.82272297364465));
#45508=CARTESIAN_POINT('Ctrl Pts',(53.0053362195786,28.8917083089376,8.81660852304238));
#45509=CARTESIAN_POINT('Ctrl Pts',(53.0051727022678,29.0955686315939,8.80464977371496));
#45510=CARTESIAN_POINT('Ctrl Pts',(53.0121945389434,29.1926010975497,8.79884651696826));
#45511=CARTESIAN_POINT('Ctrl Pts',(53.0284983074822,29.3040534939942,8.79185370977796));
#45512=CARTESIAN_POINT('Ctrl Pts',(53.0309185144273,29.3193517386526,8.79088684825428));
#45513=CARTESIAN_POINT('Ctrl Pts',(53.0351559686856,29.3442542714803,8.7893008353633));
#45514=CARTESIAN_POINT('Ctrl Pts',(53.0368661209276,29.3538763035654,8.78868504842196));
#45515=CARTESIAN_POINT('Ctrl Pts',(53.0400513753408,29.3710638200922,8.78757960302407));
#45516=CARTESIAN_POINT('Ctrl Pts',(53.0414997617339,29.3786341029149,8.78709079687659));
#45517=CARTESIAN_POINT('Ctrl Pts',(53.0441951859792,29.3922928947487,8.78620533548143));
#45518=CARTESIAN_POINT('Ctrl Pts',(53.045426876134,29.3983843464669,8.78580917318068));
#45519=CARTESIAN_POINT('Ctrl Pts',(53.0466869980092,29.404469873728,8.78541210591381));
#45520=CARTESIAN_POINT('Ctrl Pts',(53.0466869433582,29.4044696098012,8.62635914573793));
#45521=CARTESIAN_POINT('Ctrl Pts',(53.0339617519014,29.3430155919505,8.63003243338377));
#45522=CARTESIAN_POINT('Ctrl Pts',(53.0241335957554,29.2809461466272,8.633664504864));
#45523=CARTESIAN_POINT('Ctrl Pts',(53.0092986084201,29.1463066780345,8.64154158808043));
#45524=CARTESIAN_POINT('Ctrl Pts',(53.0052933510497,29.0737709068806,8.64578545019623));
#45525=CARTESIAN_POINT('Ctrl Pts',(53.0052143251304,28.9403687723671,8.65375965806322));
#45526=CARTESIAN_POINT('Ctrl Pts',(53.0079592341221,28.8795911913357,8.65745684262587));
#45527=CARTESIAN_POINT('Ctrl Pts',(53.0148509017096,28.8039374181489,8.66218413492357));
#45528=CARTESIAN_POINT('Ctrl Pts',(53.0163985773011,28.7888534763602,8.66313283702782));
#45529=CARTESIAN_POINT('Ctrl Pts',(53.0191240084723,28.7649754066958,8.66464504693492));
#45530=CARTESIAN_POINT('Ctrl Pts',(53.0201887506642,28.756168775202,8.66520502324));
#45531=CARTESIAN_POINT('Ctrl Pts',(53.0222845615333,28.7397536633467,8.6662531115338));
#45532=CARTESIAN_POINT('Ctrl Pts',(53.0233008897726,28.7321434409339,8.66674075311983));
#45533=CARTESIAN_POINT('Ctrl Pts',(53.0256614638483,28.7152131021653,8.66782955572197));
#45534=CARTESIAN_POINT('Ctrl Pts',(53.0270278151354,28.7058963018412,8.66843140006313));
#45535=CARTESIAN_POINT('Ctrl Pts',(53.0312200749308,28.6786552807828,8.67019912156417));
#45536=CARTESIAN_POINT('Ctrl Pts',(53.0342245936739,28.6607599110723,8.67137057180523));
#45537=CARTESIAN_POINT('Ctrl Pts',(53.0622986407156,28.5064686953323,8.68156167208651));
#45538=CARTESIAN_POINT('Ctrl Pts',(53.101280203247,28.3730157249933,8.69103349600716));
#45539=CARTESIAN_POINT('Ctrl Pts',(53.204821199865,28.1199216006208,8.71005608366088));
#45540=CARTESIAN_POINT('Ctrl Pts',(53.2683938458869,28.000624895526,8.71954095136477));
#45541=CARTESIAN_POINT('Ctrl Pts',(53.3519792973415,27.8760401127119,8.72946809080181));
#45542=CARTESIAN_POINT('Ctrl Pts',(53.3605819111638,27.8635289586691,8.73046494493539));
#45543=CARTESIAN_POINT('Ctrl Pts',(53.3726297011737,27.8464288670951,8.73182602505888));
#45544=CARTESIAN_POINT('Ctrl Pts',(53.3759528151812,27.8417551245087,8.73219788392165));
#45545=CARTESIAN_POINT('Ctrl Pts',(53.3816804136443,27.833772746842,8.73283264538639));
#45546=CARTESIAN_POINT('Ctrl Pts',(53.3840749802726,27.8304570888838,8.73309620531474));
#45547=CARTESIAN_POINT('Ctrl Pts',(53.3890807897185,27.8235704737932,8.73364336498074));
#45548=CARTESIAN_POINT('Ctrl Pts',(53.3916937306331,27.820000815035,8.73392683550291));
#45549=CARTESIAN_POINT('Ctrl Pts',(53.3980560227791,27.8113693867685,8.73461197997416));
#45550=CARTESIAN_POINT('Ctrl Pts',(53.401817558563,27.8063165715681,8.73501282276074));
#45551=CARTESIAN_POINT('Ctrl Pts',(53.4151688815038,27.7885581818633,8.73642109211247));
#45552=CARTESIAN_POINT('Ctrl Pts',(53.4248870479576,27.775949274491,8.7374200654158));
#45553=CARTESIAN_POINT('Ctrl Pts',(53.4492181556541,27.745150384719,8.73986160133772));
#45554=CARTESIAN_POINT('Ctrl Pts',(53.4640015635813,27.7270974955134,8.74129396545186));
#45555=CARTESIAN_POINT('Ctrl Pts',(53.5262487159168,27.6537479185619,8.74713842522752));
#45556=CARTESIAN_POINT('Ctrl Pts',(53.5764113039279,27.6008093879875,8.75141712260328));
#45557=CARTESIAN_POINT('Ctrl Pts',(53.752562042392,27.4342157733545,8.76554339734793));
#45558=CARTESIAN_POINT('Ctrl Pts',(53.8901003336186,27.3338971240844,8.77525437258152));
#45559=CARTESIAN_POINT('Ctrl Pts',(54.0585846095429,27.2412272844805,8.7871177409156));
#45560=CARTESIAN_POINT('Ctrl Pts',(54.0786896069976,27.2306126776088,8.78853150610421));
#45561=CARTESIAN_POINT('Ctrl Pts',(54.108064486066,27.2157403525991,8.79059650927869));
#45562=CARTESIAN_POINT('Ctrl Pts',(54.1171929775767,27.2112062149685,8.79123813760003));
#45563=CARTESIAN_POINT('Ctrl Pts',(54.1333564992454,27.2033316251375,8.79237427943566));
#45564=CARTESIAN_POINT('Ctrl Pts',(54.1403771453484,27.1999620138441,8.79286777418812));
#45565=CARTESIAN_POINT('Ctrl Pts',(54.1549545495421,27.1930702122522,8.79389255546922));
#45566=CARTESIAN_POINT('Ctrl Pts',(54.1625140071921,27.1895541213319,8.79442403941102));
#45567=CARTESIAN_POINT('Ctrl Pts',(54.1820381294309,27.1806214161179,8.79579699336725));
#45568=CARTESIAN_POINT('Ctrl Pts',(54.1940344976324,27.1752754595303,8.79664084884711));
#45569=CARTESIAN_POINT('Ctrl Pts',(54.2455194370674,27.1529389162304,8.80026415186306));
#45570=CARTESIAN_POINT('Ctrl Pts',(54.2854963652778,27.137109865231,8.80308220907734));
#45571=CARTESIAN_POINT('Ctrl Pts',(54.394475753681,27.0979829455769,8.81078219123228));
#45572=CARTESIAN_POINT('Ctrl Pts',(54.4642894265538,27.0771529419011,8.81573565910689));
#45573=CARTESIAN_POINT('Ctrl Pts',(54.6312663400331,27.037133102232,8.82758363536409));
#45574=CARTESIAN_POINT('Ctrl Pts',(54.7290342899673,27.021266137794,8.83452508477089));
#45575=CARTESIAN_POINT('Ctrl Pts',(54.847581976215,27.0109801991336,8.8427598748806));
#45576=CARTESIAN_POINT('Ctrl Pts',(54.867618598136,27.0095462277785,8.84414514028256));
#45577=CARTESIAN_POINT('Ctrl Pts',(54.943370030991,27.0052738178297,8.84935067876955));
#45578=CARTESIAN_POINT('Ctrl Pts',(54.9991792297645,27.0044699833988,8.85312173641572));
#45579=CARTESIAN_POINT('Ctrl Pts',(55.063996596931,27.0062563270266,8.85737512596282));
#45580=CARTESIAN_POINT('Ctrl Pts',(55.0730378615593,27.0065670625668,8.85796554968094));
#45581=CARTESIAN_POINT('Ctrl Pts',(55.0876365129166,27.0071682545114,8.85891391234663));
#45582=CARTESIAN_POINT('Ctrl Pts',(55.0931952255836,27.0074204718616,8.85927385338326));
#45583=CARTESIAN_POINT('Ctrl Pts',(55.103061596589,27.0079095200346,8.85991056991172));
#45584=CARTESIAN_POINT('Ctrl Pts',(55.1073696146435,27.0081370679286,8.86018784891336));
#45585=CARTESIAN_POINT('Ctrl Pts',(55.1166709735545,27.008658626772,8.86078491476619));
#45586=CARTESIAN_POINT('Ctrl Pts',(55.1216639530849,27.0089574427859,8.86110443349912));
#45587=CARTESIAN_POINT('Ctrl Pts',(55.1356023392242,27.0098442442184,8.86199377617303));
#45588=CARTESIAN_POINT('Ctrl Pts',(55.1445451169611,27.0104737641912,8.86256135249215));
#45589=CARTESIAN_POINT('Ctrl Pts',(55.1975007508767,27.0145604845682,8.86590602106181));
#45590=CARTESIAN_POINT('Ctrl Pts',(55.2413968545781,27.0194180567326,8.86861182223439));
#45591=CARTESIAN_POINT('Ctrl Pts',(55.3888156308679,27.040706399693,8.87758118215502));
#45592=CARTESIAN_POINT('Ctrl Pts',(55.4911983146346,27.0638345989884,8.88361965625112));
#45593=CARTESIAN_POINT('Ctrl Pts',(55.7100035059867,27.131746371403,8.89693269806536));
#45594=CARTESIAN_POINT('Ctrl Pts',(55.8249932578367,27.1795996074377,8.90420940960151));
#45595=CARTESIAN_POINT('Ctrl Pts',(55.9562613016356,27.2492334900576,8.91335756276838));
#45596=CARTESIAN_POINT('Ctrl Pts',(55.9775350575996,27.2610220872304,8.91486749967388));
#45597=CARTESIAN_POINT('Ctrl Pts',(56.0070490099876,27.2780896076299,8.91700354039067));
#45598=CARTESIAN_POINT('Ctrl Pts',(56.0154745387334,27.2830449733191,8.91761812666999));
#45599=CARTESIAN_POINT('Ctrl Pts',(56.0300590172571,27.2917675500995,8.9186905103074));
#45600=CARTESIAN_POINT('Ctrl Pts',(56.0362346163038,27.2955066736166,8.91914728865245));
#45601=CARTESIAN_POINT('Ctrl Pts',(56.0490899206826,27.3033858252593,8.92010384400551));
#45602=CARTESIAN_POINT('Ctrl Pts',(56.0557657186988,27.3075319607317,8.92060383792477));
#45603=CARTESIAN_POINT('Ctrl Pts',(56.071554022037,27.31746735783,8.92179416727123));
#45604=CARTESIAN_POINT('Ctrl Pts',(56.0806442968801,27.3232913162408,8.92248576918895));
#45605=CARTESIAN_POINT('Ctrl Pts',(56.1110937195471,27.3431501301637,8.92482387854965));
#45606=CARTESIAN_POINT('Ctrl Pts',(56.1322295746422,27.3575211309882,8.9264827943959));
#45607=CARTESIAN_POINT('Ctrl Pts',(56.182127083131,27.3928690034287,8.93048807357716));
#45608=CARTESIAN_POINT('Ctrl Pts',(56.21061394839,27.4142168839691,8.93284786581775));
#45609=CARTESIAN_POINT('Ctrl Pts',(56.3202247492292,27.5010338299848,8.94222126387747));
#45610=CARTESIAN_POINT('Ctrl Pts',(56.3967290785025,27.5720516842204,8.94942910954438));
#45611=CARTESIAN_POINT('Ctrl Pts',(56.5496285809665,27.7380811708835,8.96515364908256));
#45612=CARTESIAN_POINT('Ctrl Pts',(56.6236004788266,27.8347898953716,8.97365926549698));
#45613=CARTESIAN_POINT('Ctrl Pts',(56.6967221996578,27.9509954889552,8.98275166740897));
#45614=CARTESIAN_POINT('Ctrl Pts',(56.7049697317664,27.96445428017,8.98378862452541));
#45615=CARTESIAN_POINT('Ctrl Pts',(56.7163669278282,27.9835582308935,8.98523645209028));
#45616=CARTESIAN_POINT('Ctrl Pts',(56.7196499961326,27.9891225620709,8.98565531387402));
#45617=CARTESIAN_POINT('Ctrl Pts',(56.72512889531,27.9985124507206,8.9863572544016));
#45618=CARTESIAN_POINT('Ctrl Pts',(56.7273391569256,28.0023294857427,8.98664124448828));
#45619=CARTESIAN_POINT('Ctrl Pts',(56.7318264575111,28.0101384928698,8.98721943628707));
#45620=CARTESIAN_POINT('Ctrl Pts',(56.734102389273,28.0141310498923,8.98751356769985));
#45621=CARTESIAN_POINT('Ctrl Pts',(56.7398715270099,28.0243333590517,8.98826148660413));
#45622=CARTESIAN_POINT('Ctrl Pts',(56.7433453342593,28.0305540892133,8.98871405527718));
#45623=CARTESIAN_POINT('Ctrl Pts',(56.757367348263,28.055983166626,8.99055053578103));
#45624=CARTESIAN_POINT('Ctrl Pts',(56.7676324748415,28.0753469269005,8.99191767831141));
#45625=CARTESIAN_POINT('Ctrl Pts',(56.7939237708745,28.1269805638565,8.99549157665237));
#45626=CARTESIAN_POINT('Ctrl Pts',(56.8093989144137,28.159523168094,8.99767154549399));
#45627=CARTESIAN_POINT('Ctrl Pts',(56.8969696595348,28.3573207785658,9.01059514996441));
#45628=CARTESIAN_POINT('Ctrl Pts',(56.947271299809,28.531307575048,9.02069645124172));
#45629=CARTESIAN_POINT('Ctrl Pts',(56.9814506393162,28.7636606783768,9.03479364372171));
#45630=CARTESIAN_POINT('Ctrl Pts',(56.9871715998522,28.8179254432515,9.03812037631632));
#45631=CARTESIAN_POINT('Ctrl Pts',(56.9916123178096,28.8871787201719,9.04244154257054));
#45632=CARTESIAN_POINT('Ctrl Pts',(56.9923973064914,28.9020141847028,9.0433715524119));
#45633=CARTESIAN_POINT('Ctrl Pts',(56.9933797676268,28.9255646313478,9.04485532526244));
#45634=CARTESIAN_POINT('Ctrl Pts',(56.993685959376,28.9342747111131,9.04540570637596));
#45635=CARTESIAN_POINT('Ctrl Pts',(56.9941329710121,28.949908038901,9.04639656327099));
#45636=CARTESIAN_POINT('Ctrl Pts',(56.9942948402786,28.9568305812597,9.04683637729215));
#45637=CARTESIAN_POINT('Ctrl Pts',(56.994589142589,28.9730243310096,9.0478677594611));
#45638=CARTESIAN_POINT('Ctrl Pts',(56.9946929819655,28.9822958370831,9.04846020644303));
#45639=CARTESIAN_POINT('Ctrl Pts',(56.9948059392661,29.0090165397491,9.05017342181876));
#45640=CARTESIAN_POINT('Ctrl Pts',(56.9946507447887,29.0264652174341,9.05129925217472));
#45641=CARTESIAN_POINT('Ctrl Pts',(56.9911452086702,29.1856796636067,9.06163961237966));
#45642=CARTESIAN_POINT('Ctrl Pts',(56.9729161528102,29.3266856651235,9.07132993736857));
#45643=CARTESIAN_POINT('Ctrl Pts',(56.9089868983004,29.5936511461629,9.09043190483563));
#45644=CARTESIAN_POINT('Ctrl Pts',(56.865255489369,29.719360944655,9.09976459903682));
#45645=CARTESIAN_POINT('Ctrl Pts',(56.8029299277564,29.8536416616001,9.10956131935182));
#45646=CARTESIAN_POINT('Ctrl Pts',(56.7963468054112,29.8674091302034,9.11056330836447));
#45647=CARTESIAN_POINT('Ctrl Pts',(56.7870686310291,29.8862540672901,9.1119301020083));
#45648=CARTESIAN_POINT('Ctrl Pts',(56.7845088629206,29.8913970405553,9.11230262370906));
#45649=CARTESIAN_POINT('Ctrl Pts',(56.7800874954173,29.9001848811438,9.11293822247558));
#45650=CARTESIAN_POINT('Ctrl Pts',(56.7782368489789,29.9038351737172,9.11320196058803));
#45651=CARTESIAN_POINT('Ctrl Pts',(56.7743634056875,29.9114173676052,9.11374916619371));
#45652=CARTESIAN_POINT('Ctrl Pts',(56.7723387570832,29.9153482637589,9.11403250606704));
#45653=CARTESIAN_POINT('Ctrl Pts',(56.7674033403298,29.9248527079061,9.11471680703336));
#45654=CARTESIAN_POINT('Ctrl Pts',(56.7644792250177,29.9304193494136,9.11511694200707));
#45655=CARTESIAN_POINT('Ctrl Pts',(56.7540933302514,29.9499659271914,9.11651999490905));
#45656=CARTESIAN_POINT('Ctrl Pts',(56.746491108611,29.9638711109603,9.11751454249604));
#45657=CARTESIAN_POINT('Ctrl Pts',(56.6981128591645,30.0499074444926,9.1236551203135));
#45658=CARTESIAN_POINT('Ctrl Pts',(56.6530365776821,30.1195383623674,9.12856885887016));
#45659=CARTESIAN_POINT('Ctrl Pts',(56.5231220956694,30.2951884972068,9.14134978664947));
#45660=CARTESIAN_POINT('Ctrl Pts',(56.4315876693103,30.3956970323677,9.14909484268164));
#45661=CARTESIAN_POINT('Ctrl Pts',(56.2862365603152,30.5258320256136,9.16076686370978));
#45662=CARTESIAN_POINT('Ctrl Pts',(56.2401572629954,30.5635142490026,9.16438669119289));
#45663=CARTESIAN_POINT('Ctrl Pts',(56.180397587677,30.6080782747756,9.16902625657335));
#45664=CARTESIAN_POINT('Ctrl Pts',(56.1682279547663,30.6169408242262,9.16996827828832));
#45665=CARTESIAN_POINT('Ctrl Pts',(56.1487502291927,30.6307908278767,9.17147220735112));
#45666=CARTESIAN_POINT('Ctrl Pts',(56.1415071056893,30.6358689852694,9.17203064908879));
#45667=CARTESIAN_POINT('Ctrl Pts',(56.1279130982254,30.6452655056541,9.17307734023843));
#45668=CARTESIAN_POINT('Ctrl Pts',(56.1215705669622,30.6495957086155,9.17356513022025));
#45669=CARTESIAN_POINT('Ctrl Pts',(56.1073691152046,30.6591716257776,9.17465616735537));
#45670=CARTESIAN_POINT('Ctrl Pts',(56.0994976492308,30.6643983163253,9.17526011130222));
#45671=CARTESIAN_POINT('Ctrl Pts',(56.0762703728932,30.6795846624958,9.17704012042851));
#45672=CARTESIAN_POINT('Ctrl Pts',(56.0608146035181,30.6893889114735,9.17822187720772));
#45673=CARTESIAN_POINT('Ctrl Pts',(55.9241024519535,30.7734954138644,9.18865452849517));
#45674=CARTESIAN_POINT('Ctrl Pts',(55.7953804149375,30.8348315440107,9.19838255002727));
#45675=CARTESIAN_POINT('Ctrl Pts',(55.5378401612045,30.9253229480719,9.21738241669839));
#45676=CARTESIAN_POINT('Ctrl Pts',(55.4104448065578,30.9564460318103,9.22657205271839));
#45677=CARTESIAN_POINT('Ctrl Pts',(55.2657186252561,30.9770322855557,9.23624702864736));
#45678=CARTESIAN_POINT('Ctrl Pts',(55.2505010913404,30.9790180098671,9.2372547553672));
#45679=CARTESIAN_POINT('Ctrl Pts',(55.2295457028681,30.9815068673438,9.23862794323933));
#45680=CARTESIAN_POINT('Ctrl Pts',(55.2238267926976,30.9821610085647,9.23900121590713));
#45681=CARTESIAN_POINT('Ctrl Pts',(55.2140339886487,30.9832382076427,9.23963776358058));
#45682=CARTESIAN_POINT('Ctrl Pts',(55.2099615162392,30.9836734859811,9.23990170385414));
#45683=CARTESIAN_POINT('Ctrl Pts',(55.2014920190159,30.9845523572671,9.24044896394319));
#45684=CARTESIAN_POINT('Ctrl Pts',(55.19709483377,30.9849938839615,9.24073215793868));
#45685=CARTESIAN_POINT('Ctrl Pts',(55.1864504205745,30.9860269837559,9.24141551310351));
#45686=CARTESIAN_POINT('Ctrl Pts',(55.1802017295913,30.9866037044988,9.24181485380407));
#45687=CARTESIAN_POINT('Ctrl Pts',(55.1582440985284,30.9885258216843,9.24321207107382));
#45688=CARTESIAN_POINT('Ctrl Pts',(55.142521551041,30.9897144976411,9.24420166955198));
#45689=CARTESIAN_POINT('Ctrl Pts',(55.0449583985146,30.99592815997,9.25028424800081));
#45690=CARTESIAN_POINT('Ctrl Pts',(54.9628775016304,30.9960900445842,9.25514963820476));
#45691=CARTESIAN_POINT('Ctrl Pts',(54.7358001410951,30.982520521511,9.26846233415437));
#45692=CARTESIAN_POINT('Ctrl Pts',(54.5919810933355,30.9579858950746,9.27675761395452));
#45693=CARTESIAN_POINT('Ctrl Pts',(54.4022424608979,30.9037865037627,9.28862532778164));
#45694=CARTESIAN_POINT('Ctrl Pts',(54.3529541697322,30.8876038052835,9.29179286536457));
#45695=CARTESIAN_POINT('Ctrl Pts',(54.2907024865597,30.8644400784415,9.29593047234084));
#45696=CARTESIAN_POINT('Ctrl Pts',(54.2771060716231,30.8592106172561,9.29684267137894));
#45697=CARTESIAN_POINT('Ctrl Pts',(54.2555275314168,30.8506385830807,9.2983045489736));
#45698=CARTESIAN_POINT('Ctrl Pts',(54.247507604182,30.8473921110868,9.29885101759913));
#45699=CARTESIAN_POINT('Ctrl Pts',(54.2330997268035,30.841450406801,9.29983854186114));
#45700=CARTESIAN_POINT('Ctrl Pts',(54.2267041926349,30.8387738365748,9.30027896418759));
#45701=CARTESIAN_POINT('Ctrl Pts',(54.2118789257908,30.8324783466594,9.30130477328933));
#45702=CARTESIAN_POINT('Ctrl Pts',(54.2034599984423,30.8288345304843,9.30189099391295));
#45703=CARTESIAN_POINT('Ctrl Pts',(54.1793351363773,30.8181948079571,9.303581630362));
#45704=CARTESIAN_POINT('Ctrl Pts',(54.1636944352306,30.8110538782385,9.30469094524407));
#45705=CARTESIAN_POINT('Ctrl Pts',(54.1285089680757,30.7944365914974,9.30721723835268));
#45706=CARTESIAN_POINT('Ctrl Pts',(54.1090230066409,30.7848415156968,9.30863815459307));
#45707=CARTESIAN_POINT('Ctrl Pts',(54.0465054187845,30.7527783601519,9.31326910091151));
#45708=CARTESIAN_POINT('Ctrl Pts',(54.0041387413426,30.7290585957074,9.31652024617999));
#45709=CARTESIAN_POINT('Ctrl Pts',(53.8661777342329,30.6450652506076,9.32748305733285));
#45710=CARTESIAN_POINT('Ctrl Pts',(53.7748464040783,30.578222816338,9.33537995111363));
#45711=CARTESIAN_POINT('Ctrl Pts',(53.6154587579674,30.439361385762,9.35009308193447));
#45712=CARTESIAN_POINT('Ctrl Pts',(53.5461232957958,30.3692927925865,9.35689324698141));
#45713=CARTESIAN_POINT('Ctrl Pts',(53.4753388251414,30.2862927084301,9.36405816488137));
#45714=CARTESIAN_POINT('Ctrl Pts',(53.4685035406163,30.2781467977636,9.36475251360451));
#45715=CARTESIAN_POINT('Ctrl Pts',(53.4582804068789,30.2657636738789,9.36579427166871));
#45716=CARTESIAN_POINT('Ctrl Pts',(53.4548442933306,30.2615668138262,9.36614498583346));
#45717=CARTESIAN_POINT('Ctrl Pts',(53.4487127132625,30.2540150859693,9.3667717602668));
#45718=CARTESIAN_POINT('Ctrl Pts',(53.4460109556245,30.2506654760099,9.36704826263214));
#45719=CARTESIAN_POINT('Ctrl Pts',(53.440127727406,30.2433230146068,9.36765107403969));
#45720=CARTESIAN_POINT('Ctrl Pts',(53.4369507419554,30.239326689692,9.36797706713424));
#45721=CARTESIAN_POINT('Ctrl Pts',(53.4279404882153,30.2279029462622,9.36890310710753));
#45722=CARTESIAN_POINT('Ctrl Pts',(53.4221444834489,30.2204461197527,9.36950059698377));
#45723=CARTESIAN_POINT('Ctrl Pts',(53.3835996994863,30.1701228996162,9.37348835233874));
#45724=CARTESIAN_POINT('Ctrl Pts',(53.3525452861601,30.1259802979351,9.37677154541507));
#45725=CARTESIAN_POINT('Ctrl Pts',(53.2575319217559,29.978559298931,9.38724728457753));
#45726=CARTESIAN_POINT('Ctrl Pts',(53.2012020971099,29.8706910060105,9.39418406983926));
#45727=CARTESIAN_POINT('Ctrl Pts',(53.1349386626491,29.7094834498775,9.40436892285359));
#45728=CARTESIAN_POINT('Ctrl Pts',(53.1167979495078,29.6598258502138,9.40748084197396));
#45729=CARTESIAN_POINT('Ctrl Pts',(53.0825149897801,29.5529933806987,9.41419402490627));
#45730=CARTESIAN_POINT('Ctrl Pts',(53.0669119579143,29.4957015797813,9.41780520397248));
#45731=CARTESIAN_POINT('Ctrl Pts',(53.0513919897812,29.4267125639665,9.42220626268059));
#45732=CARTESIAN_POINT('Ctrl Pts',(53.0489919156069,29.4156010501272,9.42291666214691));
#45733=CARTESIAN_POINT('Ctrl Pts',(53.0466869980009,29.4044698736881,9.42363003822484));
#45734=CARTESIAN_POINT('Origin',(55.,29.,3.45145488139523));
#45735=CARTESIAN_POINT('',(53.0466869980528,29.4044698739386,10.38234667127));
#45736=CARTESIAN_POINT('',(53.046686906026,29.4044694295118,10.2256126172116));
#45737=CARTESIAN_POINT('',(53.0466869980082,29.4044698737233,3.45145488139523));
#45738=CARTESIAN_POINT('',(53.0052500005621,28.9999526465424,9.60767889029237));
#45739=CARTESIAN_POINT('Ctrl Pts',(53.0466869980528,29.4044698739386,10.38234667127));
#45740=CARTESIAN_POINT('Ctrl Pts',(53.0495690730458,29.418388326014,10.3813700720195));
#45741=CARTESIAN_POINT('Ctrl Pts',(53.0525999295262,29.4322760519837,10.3803968981023));
#45742=CARTESIAN_POINT('Ctrl Pts',(53.0659164325032,29.4903088798927,10.3763384924675));
#45743=CARTESIAN_POINT('Ctrl Pts',(53.0775575452908,29.5341327205029,10.3732935163058));
#45744=CARTESIAN_POINT('Ctrl Pts',(53.0931574468468,29.5857064922055,10.3697627720438));
#45745=CARTESIAN_POINT('Ctrl Pts',(53.0956846717732,29.5938718333258,10.3692053724519));
#45746=CARTESIAN_POINT('Ctrl Pts',(53.0998983088677,29.6071823754082,10.3682996436764));
#45747=CARTESIAN_POINT('Ctrl Pts',(53.101553291598,29.6123373013907,10.3679495863005));
#45748=CARTESIAN_POINT('Ctrl Pts',(53.1045612374735,29.621577006171,10.367323506836));
#45749=CARTESIAN_POINT('Ctrl Pts',(53.1059064428019,29.625664186882,10.3670470470468));
#45750=CARTESIAN_POINT('Ctrl Pts',(53.1088791695915,29.6345988596246,10.366443769413));
#45751=CARTESIAN_POINT('Ctrl Pts',(53.1105121055804,29.6394444511355,10.3661172711826));
#45752=CARTESIAN_POINT('Ctrl Pts',(53.1152262281519,29.6532574511882,10.365188346825));
#45753=CARTESIAN_POINT('Ctrl Pts',(53.118352794664,29.6622093865426,10.3645885027962));
#45754=CARTESIAN_POINT('Ctrl Pts',(53.1399962193134,29.7227873677053,10.360541950609));
#45755=CARTESIAN_POINT('Ctrl Pts',(53.1605734442592,29.7736580474306,10.3572059697192));
#45756=CARTESIAN_POINT('Ctrl Pts',(53.2642710874475,30.0023986563568,10.3422153684849));
#45757=CARTESIAN_POINT('Ctrl Pts',(53.3712601990154,30.1682351125603,10.3312624043519));
#45758=CARTESIAN_POINT('Ctrl Pts',(53.5273378627706,30.3460750710649,10.3169054423481));
#45759=CARTESIAN_POINT('Ctrl Pts',(53.5548328177161,30.37555201321,10.3144282951032));
#45760=CARTESIAN_POINT('Ctrl Pts',(53.5925661032047,30.4136245646633,10.3110832037014));
#45761=CARTESIAN_POINT('Ctrl Pts',(53.6020260386991,30.4229804544224,10.3102489258938));
#45762=CARTESIAN_POINT('Ctrl Pts',(53.6175917323802,30.4380699145239,10.3088827889616));
#45763=CARTESIAN_POINT('Ctrl Pts',(53.6236413559673,30.4438609964227,10.3083534312968));
#45764=CARTESIAN_POINT('Ctrl Pts',(53.6353762496506,30.4549536104352,10.3073295451221));
#45765=CARTESIAN_POINT('Ctrl Pts',(53.6410564046646,30.4602603502263,10.3068352527054));
#45766=CARTESIAN_POINT('Ctrl Pts',(53.654319455554,30.4725070787383,10.3056840233319));
#45767=CARTESIAN_POINT('Ctrl Pts',(53.6619252136078,30.4794218749748,10.3050260421009));
#45768=CARTESIAN_POINT('Ctrl Pts',(53.6864219311068,30.5013496956282,10.3029135396763));
#45769=CARTESIAN_POINT('Ctrl Pts',(53.7035142137582,30.5161341591406,10.3014496459182));
#45770=CARTESIAN_POINT('Ctrl Pts',(53.7924942332987,30.5904949725454,10.2938769090778));
#45771=CARTESIAN_POINT('Ctrl Pts',(53.8682398251174,30.6452534830512,10.2875801836952));
#45772=CARTESIAN_POINT('Ctrl Pts',(54.0541636482885,30.760732251701,10.2725129889987));
#45773=CARTESIAN_POINT('Ctrl Pts',(54.1668045260358,30.8167466349176,10.2636617426247));
#45774=CARTESIAN_POINT('Ctrl Pts',(54.335977836697,30.8818098369856,10.2512263658725));
#45775=CARTESIAN_POINT('Ctrl Pts',(54.3888170236623,30.8996289869442,10.2474589358557));
#45776=CARTESIAN_POINT('Ctrl Pts',(54.4510216936421,30.9177414270883,10.2432091060772));
#45777=CARTESIAN_POINT('Ctrl Pts',(54.459722668644,30.9202108672135,10.2426188138007));
#45778=CARTESIAN_POINT('Ctrl Pts',(54.4738028851581,30.9241037170545,10.2416706202782));
#45779=CARTESIAN_POINT('Ctrl Pts',(54.4791716972671,30.9255639170195,10.2413107180681));
#45780=CARTESIAN_POINT('Ctrl Pts',(54.4887140546065,30.9281164007025,10.2406740438168));
#45781=CARTESIAN_POINT('Ctrl Pts',(54.4928851036639,30.929217627894,10.2403967685246));
#45782=CARTESIAN_POINT('Ctrl Pts',(54.501900445257,30.9315665710594,10.239799680712));
#45783=CARTESIAN_POINT('Ctrl Pts',(54.5067458645648,30.9328095985027,10.2394801365001));
#45784=CARTESIAN_POINT('Ctrl Pts',(54.5202895211314,30.9362297943436,10.2385906510481));
#45785=CARTESIAN_POINT('Ctrl Pts',(54.5289979668841,30.9383665938054,10.2380229585962));
#45786=CARTESIAN_POINT('Ctrl Pts',(54.5806990007094,30.950683521716,10.2346761086877));
#45787=CARTESIAN_POINT('Ctrl Pts',(54.624009301221,30.9594925835633,10.2319683507442));
#45788=CARTESIAN_POINT('Ctrl Pts',(54.7710568645391,30.9843452148307,10.2229881150481));
#45789=CARTESIAN_POINT('Ctrl Pts',(54.8757601674787,30.9936420442041,10.2169413334741));
#45790=CARTESIAN_POINT('Ctrl Pts',(55.1048237348402,30.9958566914059,10.2036296340241));
#45791=CARTESIAN_POINT('Ctrl Pts',(55.2287579617121,30.985471384532,10.1963627789262));
#45792=CARTESIAN_POINT('Ctrl Pts',(55.374854130337,30.959362972407,10.1872258538473));
#45793=CARTESIAN_POINT('Ctrl Pts',(55.3987107719586,30.954647926769,10.1857161296592));
#45794=CARTESIAN_POINT('Ctrl Pts',(55.4320256460817,30.9474282817201,10.1835804204124));
#45795=CARTESIAN_POINT('Ctrl Pts',(55.4415613268412,30.9452883232437,10.182965949786));
#45796=CARTESIAN_POINT('Ctrl Pts',(55.4581126833832,30.9414459674622,10.1818937107096));
#45797=CARTESIAN_POINT('Ctrl Pts',(55.4651356129703,30.9397753825082,10.1814369605777));
#45798=CARTESIAN_POINT('Ctrl Pts',(55.4797848789184,30.9362065477715,10.180480408078));
#45799=CARTESIAN_POINT('Ctrl Pts',(55.4874093612983,30.9343012788357,10.1799803885014));
#45800=CARTESIAN_POINT('Ctrl Pts',(55.5054825717024,30.9296713528955,10.1787898947011));
#45801=CARTESIAN_POINT('Ctrl Pts',(55.5159207413699,30.9269068326108,10.17809815305));
#45802=CARTESIAN_POINT('Ctrl Pts',(55.5509998253696,30.9173107707106,10.1757590734199));
#45803=CARTESIAN_POINT('Ctrl Pts',(55.5755308554245,30.9100904516269,10.174099313024));
#45804=CARTESIAN_POINT('Ctrl Pts',(55.6338835050969,30.8916891490242,10.1700916242326));
#45805=CARTESIAN_POINT('Ctrl Pts',(55.6675567524781,30.880070173855,10.167730245548));
#45806=CARTESIAN_POINT('Ctrl Pts',(55.7986014462323,30.8308887289958,10.1583470747256));
#45807=CARTESIAN_POINT('Ctrl Pts',(55.8932651326754,30.7866143241155,10.1511305955659));
#45808=CARTESIAN_POINT('Ctrl Pts',(56.0895559994211,30.6752954436137,10.135409264161));
#45809=CARTESIAN_POINT('Ctrl Pts',(56.1894194729557,30.6059369982914,10.1269159392035));
#45810=CARTESIAN_POINT('Ctrl Pts',(56.2944610502715,30.517777138703,10.1178342410082));
#45811=CARTESIAN_POINT('Ctrl Pts',(56.3064344986906,30.5074832639866,10.1167969320462));
#45812=CARTESIAN_POINT('Ctrl Pts',(56.3231341421418,30.4927777310115,10.1153487005424));
#45813=CARTESIAN_POINT('Ctrl Pts',(56.3279626954465,30.4884839248695,10.1149297808473));
#45814=CARTESIAN_POINT('Ctrl Pts',(56.3360522328033,30.4812195818173,10.1142277711554));
#45815=CARTESIAN_POINT('Ctrl Pts',(56.3393243534943,30.4782615789316,10.1139437694234));
#45816=CARTESIAN_POINT('Ctrl Pts',(56.3459853791995,30.4721997279641,10.1133655810159));
#45817=CARTESIAN_POINT('Ctrl Pts',(56.3493734109576,30.4690949863342,10.1130714644863));
#45818=CARTESIAN_POINT('Ctrl Pts',(56.357986034671,30.461147575945,10.1123236300263));
#45819=CARTESIAN_POINT('Ctrl Pts',(56.3631955231479,30.4562885285496,10.11187113037));
#45820=CARTESIAN_POINT('Ctrl Pts',(56.3843170379587,30.4363752001297,10.1100352935692));
#45821=CARTESIAN_POINT('Ctrl Pts',(56.4000072989275,30.4210865678213,10.1086687109356));
#45822=CARTESIAN_POINT('Ctrl Pts',(56.4408130376617,30.3799933704081,10.1050966360637));
#45823=CARTESIAN_POINT('Ctrl Pts',(56.4654879503862,30.3537611619265,10.1029178968978));
#45824=CARTESIAN_POINT('Ctrl Pts',(56.6091296023158,30.1925207405835,10.0900162602896));
#45825=CARTESIAN_POINT('Ctrl Pts',(56.7100926744953,30.042590259918,10.0799336850375));
#45826=CARTESIAN_POINT('Ctrl Pts',(56.8138254146022,29.8319112989469,10.065840992096));
#45827=CARTESIAN_POINT('Ctrl Pts',(56.8360224934992,29.7817030346368,10.0624946878773));
#45828=CARTESIAN_POINT('Ctrl Pts',(56.8615723158017,29.7167967780808,10.0581513665782));
#45829=CARTESIAN_POINT('Ctrl Pts',(56.8668689394584,29.7028865143727,10.0572196100878));
#45830=CARTESIAN_POINT('Ctrl Pts',(56.8750214607103,29.6807335398309,10.055733689976));
#45831=CARTESIAN_POINT('Ctrl Pts',(56.877979881727,29.6725289512857,10.055182925316));
#45832=CARTESIAN_POINT('Ctrl Pts',(56.8831901475673,29.6577768378664,10.0541917353995));
#45833=CARTESIAN_POINT('Ctrl Pts',(56.8854619006575,29.6512364543924,10.0537519746699));
#45834=CARTESIAN_POINT('Ctrl Pts',(56.8906935210182,29.6359177547879,10.0527211804419));
#45835=CARTESIAN_POINT('Ctrl Pts',(56.8936263588951,29.6271304405155,10.0521292714356));
#45836=CARTESIAN_POINT('Ctrl Pts',(56.9018943740286,29.6017710904626,10.0504191543564));
#45837=CARTESIAN_POINT('Ctrl Pts',(56.9070738374667,29.5851495552795,10.0492959126677));
#45838=CARTESIAN_POINT('Ctrl Pts',(56.9511171342135,29.4370091218193,10.0392614627375));
#45839=CARTESIAN_POINT('Ctrl Pts',(56.976531744876,29.3019007898177,10.0299075200651));
#45840=CARTESIAN_POINT('Ctrl Pts',(56.9993109129814,29.0279263631165,10.0107918941993));
#45841=CARTESIAN_POINT('Ctrl Pts',(56.9964655033797,28.889749982484,10.0010854107477));
#45842=CARTESIAN_POINT('Ctrl Pts',(56.9775354058949,28.7380715721173,9.99097350566615));
#45843=CARTESIAN_POINT('Ctrl Pts',(56.9755087813167,28.7232006685105,9.98998830541222));
#45844=CARTESIAN_POINT('Ctrl Pts',(56.9724793636188,28.7027032703608,9.98864020060802));
#45845=CARTESIAN_POINT('Ctrl Pts',(56.9716200049681,28.6970565344992,9.98826985272575));
#45846=CARTESIAN_POINT('Ctrl Pts',(56.9701046355262,28.6873788799004,9.98763699892714));
#45847=CARTESIAN_POINT('Ctrl Pts',(56.9694604841787,28.6833461801242,9.98737384414405));
#45848=CARTESIAN_POINT('Ctrl Pts',(56.968091967137,28.6749443357144,9.98682678110305));
#45849=CARTESIAN_POINT('Ctrl Pts',(56.9673654306842,28.670575595047,9.98654300572342));
#45850=CARTESIAN_POINT('Ctrl Pts',(56.965565918277,28.6599732484891,9.98585590639869));
#45851=CARTESIAN_POINT('Ctrl Pts',(56.964477818784,28.653742187183,9.98545342531314));
#45852=CARTESIAN_POINT('Ctrl Pts',(56.9605177328844,28.6316842176639,9.98403302468994));
#45853=CARTESIAN_POINT('Ctrl Pts',(56.9574838828276,28.6158864965843,9.98302375292391));
#45854=CARTESIAN_POINT('Ctrl Pts',(56.94951708552,28.5769512050477,9.98055225078294));
#45855=CARTESIAN_POINT('Ctrl Pts',(56.9443629224555,28.553860923034,9.9791005464766));
#45856=CARTESIAN_POINT('Ctrl Pts',(56.9212628061124,28.4583944737858,9.97313640610307));
#45857=CARTESIAN_POINT('Ctrl Pts',(56.8996754475119,28.386956590116,9.9687630983016));
#45858=CARTESIAN_POINT('Ctrl Pts',(56.8169881925049,28.1601009400205,9.95470215577796));
#45859=CARTESIAN_POINT('Ctrl Pts',(56.7403987723663,28.0111204047871,9.9451329520471));
#45860=CARTESIAN_POINT('Ctrl Pts',(56.6344471595296,27.8563041998709,9.93356235028809));
#45861=CARTESIAN_POINT('Ctrl Pts',(56.6224694444249,27.8393749731165,9.9322740523967));
#45862=CARTESIAN_POINT('Ctrl Pts',(56.6035775823074,27.8135373818747,9.93027017498601));
#45863=CARTESIAN_POINT('Ctrl Pts',(56.5968479685092,27.8044954354465,9.92956162505039));
#45864=CARTESIAN_POINT('Ctrl Pts',(56.5852913793253,27.7892396159635,9.92835344023985));
#45865=CARTESIAN_POINT('Ctrl Pts',(56.5805035572744,27.7829963157455,9.92785533460698));
#45866=CARTESIAN_POINT('Ctrl Pts',(56.5707451524356,27.7704261050039,9.92684491292012));
#45867=CARTESIAN_POINT('Ctrl Pts',(56.5657729782752,27.7641006211836,9.92633254000641));
#45868=CARTESIAN_POINT('Ctrl Pts',(56.5534357289488,27.7485994106841,9.92506712973168));
#45869=CARTESIAN_POINT('Ctrl Pts',(56.5460275511586,27.7394585289619,9.9243123865968));
#45870=CARTESIAN_POINT('Ctrl Pts',(56.5182567663241,27.705805492649,9.92150141248882));
#45871=CARTESIAN_POINT('Ctrl Pts',(56.4973894458384,27.6817179035125,9.91942493336286));
#45872=CARTESIAN_POINT('Ctrl Pts',(56.4438669293128,27.6228466933229,9.91418266389034));
#45873=CARTESIAN_POINT('Ctrl Pts',(56.4105253612589,27.588716700212,9.91098981920189));
#45874=CARTESIAN_POINT('Ctrl Pts',(56.2380275214923,27.4243635371041,9.89483003549955));
#45875=CARTESIAN_POINT('Ctrl Pts',(56.0819570479171,27.3133762427855,9.88119559215382));
#45876=CARTESIAN_POINT('Ctrl Pts',(55.8883226319175,27.2137605166992,9.86657798900654));
#45877=CARTESIAN_POINT('Ctrl Pts',(55.8638623968812,27.2018035356543,9.86477169064446));
#45878=CARTESIAN_POINT('Ctrl Pts',(55.831892603013,27.1869786276877,9.8624694342865));
#45879=CARTESIAN_POINT('Ctrl Pts',(55.8246011290096,27.1836506991593,9.86194823733075));
#45880=CARTESIAN_POINT('Ctrl Pts',(55.812917650065,27.1784030557935,9.86111952391067));
#45881=CARTESIAN_POINT('Ctrl Pts',(55.8085385331707,27.1764551076325,9.86081034542445));
#45882=CARTESIAN_POINT('Ctrl Pts',(55.8001606095793,27.1727644958179,9.8602216334051));
#45883=CARTESIAN_POINT('Ctrl Pts',(55.7961630883288,27.1710191564822,9.85994194679333));
#45884=CARTESIAN_POINT('Ctrl Pts',(55.7867067333492,27.1669273385498,9.85928314645982));
#45885=CARTESIAN_POINT('Ctrl Pts',(55.781243034054,27.1645920915607,9.85890470733511));
#45886=CARTESIAN_POINT('Ctrl Pts',(55.7630929143796,27.1569302562574,9.85765458160374));
#45887=CARTESIAN_POINT('Ctrl Pts',(55.750361492667,27.1517103768047,9.85678902507696));
#45888=CARTESIAN_POINT('Ctrl Pts',(55.6796925758607,27.1235867248475,9.85204157713664));
#45889=CARTESIAN_POINT('Ctrl Pts',(55.6207550883577,27.1032729646532,9.84829244817451));
#45890=CARTESIAN_POINT('Ctrl Pts',(55.4088153647025,27.0411654802553,9.8352291888377));
#45891=CARTESIAN_POINT('Ctrl Pts',(55.2519020388455,27.0148776444196,9.82626528922662));
#45892=CARTESIAN_POINT('Ctrl Pts',(55.0335836777962,27.0046301481973,9.81319400996679));
#45893=CARTESIAN_POINT('Ctrl Pts',(54.9735487066553,27.0045231150141,9.80954420042224));
#45894=CARTESIAN_POINT('Ctrl Pts',(54.8985131368656,27.0077760806353,9.80487012341394));
#45895=CARTESIAN_POINT('Ctrl Pts',(54.8834304084885,27.008601687515,9.8039249845544));
#45896=CARTESIAN_POINT('Ctrl Pts',(54.8595205925043,27.0101830348796,9.80241719114877));
#45897=CARTESIAN_POINT('Ctrl Pts',(54.8506864646157,27.010826432235,9.80185803288893));
#45898=CARTESIAN_POINT('Ctrl Pts',(54.8342023672404,27.0121374112109,9.80081069074307));
#45899=CARTESIAN_POINT('Ctrl Pts',(54.8265513742967,27.012790373792,9.80032297141463));
#45900=CARTESIAN_POINT('Ctrl Pts',(54.8095098011816,27.0143439272724,9.79923298471219));
#45901=CARTESIAN_POINT('Ctrl Pts',(54.8001215030099,27.0152669861094,9.79863002687059));
#45902=CARTESIAN_POINT('Ctrl Pts',(54.7726120058559,27.0181688890737,9.79685579525983));
#45903=CARTESIAN_POINT('Ctrl Pts',(54.7545113570441,27.020329537037,9.7956788857739));
#45904=CARTESIAN_POINT('Ctrl Pts',(54.5911811373924,27.0421004323816,9.78497009870276));
#45905=CARTESIAN_POINT('Ctrl Pts',(54.4485231394684,27.0774077268452,9.77492883083884));
#45906=CARTESIAN_POINT('Ctrl Pts',(54.1925431457231,27.1716166297644,9.7559338576299));
#45907=CARTESIAN_POINT('Ctrl Pts',(54.0784403644572,27.2263862987119,9.74707793014061));
#45908=CARTESIAN_POINT('Ctrl Pts',(53.9569549464975,27.2996099100484,9.73768681087294));
#45909=CARTESIAN_POINT('Ctrl Pts',(53.943728775343,27.3077941682116,9.73666522575495));
#45910=CARTESIAN_POINT('Ctrl Pts',(53.9252669192777,27.3195190363828,9.73524187051626));
#45911=CARTESIAN_POINT('Ctrl Pts',(53.919950662539,27.3229308615527,9.73483231405498));
#45912=CARTESIAN_POINT('Ctrl Pts',(53.9109706983788,27.3287543628982,9.73414116019926));
#45913=CARTESIAN_POINT('Ctrl Pts',(53.9072986079801,27.3311529523888,9.73385871865714));
#45914=CARTESIAN_POINT('Ctrl Pts',(53.9002745310404,27.3357741648256,9.73331885798567));
#45915=CARTESIAN_POINT('Ctrl Pts',(53.896921314201,27.3379948402088,9.733061309224));
#45916=CARTESIAN_POINT('Ctrl Pts',(53.8883594841403,27.3437022573785,9.73240409067887));
#45917=CARTESIAN_POINT('Ctrl Pts',(53.8831604992021,27.3472034666383,9.73200537564485));
#45918=CARTESIAN_POINT('Ctrl Pts',(53.8642100798863,27.3600957016342,9.73055305626359));
#45919=CARTESIAN_POINT('Ctrl Pts',(53.8505594347303,27.3696346176597,9.7295088476598));
#45920=CARTESIAN_POINT('Ctrl Pts',(53.8169046124162,27.393785063307,9.7269349869487));
#45921=CARTESIAN_POINT('Ctrl Pts',(53.7970496904925,27.4086006831486,9.72541702399541));
#45922=CARTESIAN_POINT('Ctrl Pts',(53.7137906291889,27.4731769958865,9.71902979454633));
#45923=CARTESIAN_POINT('Ctrl Pts',(53.6531531755986,27.5263892383107,9.71432081920447));
#45924=CARTESIAN_POINT('Ctrl Pts',(53.4838765212235,27.6941402765568,9.7004631684836));
#45925=CARTESIAN_POINT('Ctrl Pts',(53.3854280604051,27.8180307082878,9.69137989380192));
#45926=CARTESIAN_POINT('Ctrl Pts',(53.2900633231478,27.9725207817267,9.68019192523581));
#45927=CARTESIAN_POINT('Ctrl Pts',(53.2778948316235,27.9930488112211,9.67870919637831));
#45928=CARTESIAN_POINT('Ctrl Pts',(53.2614229027687,28.0220088688517,9.67662044695475));
#45929=CARTESIAN_POINT('Ctrl Pts',(53.2568064698014,28.0302612274474,9.67602558500137));
#45930=CARTESIAN_POINT('Ctrl Pts',(53.2484622638812,28.0454294980589,9.67493266161727));
#45931=CARTESIAN_POINT('Ctrl Pts',(53.2447163235432,28.0523352404296,9.67443525491053));
#45932=CARTESIAN_POINT('Ctrl Pts',(53.2372102271168,28.0663701264627,9.67342461426553));
#45933=CARTESIAN_POINT('Ctrl Pts',(53.2334522928931,28.07350028627,9.67291131395324));
#45934=CARTESIAN_POINT('Ctrl Pts',(53.2242833787699,28.0911556240099,9.67164053931098));
#45935=CARTESIAN_POINT('Ctrl Pts',(53.2189227128478,28.1017064477949,9.67088132686099));
#45936=CARTESIAN_POINT('Ctrl Pts',(53.1992573694939,28.1412797565151,9.66803406566511));
#45937=CARTESIAN_POINT('Ctrl Pts',(53.1855662725116,28.1705999007872,9.6659250824205));
#45938=CARTESIAN_POINT('Ctrl Pts',(53.1530701165786,28.2448516047975,9.66058251691468));
#45939=CARTESIAN_POINT('Ctrl Pts',(53.1351870010847,28.2901613252473,9.65732053421681));
#45940=CARTESIAN_POINT('Ctrl Pts',(53.087007981703,28.4266616106876,9.64749429688095));
#45941=CARTESIAN_POINT('Ctrl Pts',(53.0616228603348,28.5194308407119,9.6408105480962));
#45942=CARTESIAN_POINT('Ctrl Pts',(53.0208816117651,28.7258026560622,9.62614955016616));
#45943=CARTESIAN_POINT('Ctrl Pts',(53.0084205342428,28.8396541017884,9.61819241389745));
#45944=CARTESIAN_POINT('Ctrl Pts',(53.0055328640902,28.9647238913065,9.60996833674216));
#45945=CARTESIAN_POINT('Ctrl Pts',(53.0053714639023,28.9754933620863,9.60926446488619));
#45946=CARTESIAN_POINT('Ctrl Pts',(53.0052730197494,28.9897890285981,9.60833627449039));
#45947=CARTESIAN_POINT('Ctrl Pts',(53.0052580891371,28.9933142555978,9.60810788431084));
#45948=CARTESIAN_POINT('Ctrl Pts',(53.0052508595823,28.9978772359666,9.60781291889297));
#45949=CARTESIAN_POINT('Ctrl Pts',(53.0052500251962,28.9989149398816,9.60774588249731));
#45950=CARTESIAN_POINT('Ctrl Pts',(53.0052500005621,28.9999526465424,9.60767889029237));
#45951=CARTESIAN_POINT('Ctrl Pts',(53.0052500005549,28.9999529473371,9.60767887087368));
#45952=CARTESIAN_POINT('Ctrl Pts',(53.0052499758941,29.000998421014,9.60761137725482));
#45953=CARTESIAN_POINT('Ctrl Pts',(53.005250773152,29.0020438978185,9.60754392846873));
#45954=CARTESIAN_POINT('Ctrl Pts',(53.0052578036797,29.0065833662361,9.60725126225896));
#45955=CARTESIAN_POINT('Ctrl Pts',(53.0052723951246,29.0100773799544,9.60702650522149));
#45956=CARTESIAN_POINT('Ctrl Pts',(53.0053240150624,29.0176644004869,9.6065395837483));
#45957=CARTESIAN_POINT('Ctrl Pts',(53.0053644607703,29.0217573505928,9.60627761129943));
#45958=CARTESIAN_POINT('Ctrl Pts',(53.005503607383,29.0324938046946,9.60559220016993));
#45959=CARTESIAN_POINT('Ctrl Pts',(53.0056229039718,29.0391370582672,9.60516988931161));
#45960=CARTESIAN_POINT('Ctrl Pts',(53.0061825007537,29.063513836217,9.60362643214059));
#45961=CARTESIAN_POINT('Ctrl Pts',(53.0068261641602,29.0812424682206,9.60251590105475));
#45962=CARTESIAN_POINT('Ctrl Pts',(53.0084820983296,29.1145799638644,9.60044624452814));
#45963=CARTESIAN_POINT('Ctrl Pts',(53.0094415994123,29.1301898770908,9.59948484584387));
#45964=CARTESIAN_POINT('Ctrl Pts',(53.0169604534845,29.2327922197205,9.59320695819293));
#45965=CARTESIAN_POINT('Ctrl Pts',(53.0290309706326,29.3192034122154,9.58811224818012));
#45966=CARTESIAN_POINT('Ctrl Pts',(53.0466870746609,29.4044702439035,9.58304844318572));
#45967=CARTESIAN_POINT('',(53.0052509575277,28.9983381707197,9.45054880350992));
#45968=CARTESIAN_POINT('Ctrl Pts',(53.0466869980009,29.4044698736881,9.42363003822484));
#45969=CARTESIAN_POINT('Ctrl Pts',(53.0459416970957,29.4008705797895,9.42386071017391));
#45970=CARTESIAN_POINT('Ctrl Pts',(53.0452063454643,29.39726923002,9.42409169317728));
#45971=CARTESIAN_POINT('Ctrl Pts',(53.042735689669,29.3849963486351,9.42487947785384));
#45972=CARTESIAN_POINT('Ctrl Pts',(53.0410481227673,29.376315436298,9.42543776448021));
#45973=CARTESIAN_POINT('Ctrl Pts',(53.0380029722169,29.3600752802278,9.42648431520925));
#45974=CARTESIAN_POINT('Ctrl Pts',(53.0366312084331,29.3525188364851,9.42697212099367));
#45975=CARTESIAN_POINT('Ctrl Pts',(53.0340280434432,29.3376924565463,9.42793098056701));
#45976=CARTESIAN_POINT('Ctrl Pts',(53.0327932462526,29.3304232358528,9.42840191856188));
#45977=CARTESIAN_POINT('Ctrl Pts',(53.0301021431149,29.3140308080912,9.42946581604622));
#45978=CARTESIAN_POINT('Ctrl Pts',(53.0286688671776,29.3049040423193,9.43005948974283));
#45979=CARTESIAN_POINT('Ctrl Pts',(53.0252105952784,29.2818381886003,9.43156334767361));
#45980=CARTESIAN_POINT('Ctrl Pts',(53.0232697702393,29.2678871768863,9.43247613613497));
#45981=CARTESIAN_POINT('Ctrl Pts',(53.010597734152,29.1691466070122,9.43896009296105));
#45982=CARTESIAN_POINT('Ctrl Pts',(53.0051794209271,29.0837777997029,9.44469429247309));
#45983=CARTESIAN_POINT('Ctrl Pts',(53.0052506940152,28.9983360368706,9.45054848948101));
#45984=CARTESIAN_POINT('Ctrl Pts',(53.0052506922627,28.9983381391186,9.4505483454417));
#45985=CARTESIAN_POINT('Ctrl Pts',(53.0053360688677,28.8958596912809,9.45756983960953));
#45986=CARTESIAN_POINT('Ctrl Pts',(53.0133185283999,28.7935409683466,9.46474865672663));
#45987=CARTESIAN_POINT('Ctrl Pts',(53.0417524955803,28.6114204569449,9.47755645448682));
#45988=CARTESIAN_POINT('Ctrl Pts',(53.0593460938601,28.5313929905911,9.48319153730964));
#45989=CARTESIAN_POINT('Ctrl Pts',(53.0861323595426,28.4375176667941,9.48965343160242));
#45990=CARTESIAN_POINT('Ctrl Pts',(53.0906342468335,28.4224204141284,9.49068785799599));
#45991=CARTESIAN_POINT('Ctrl Pts',(53.0971783369115,28.4013877451173,9.49212073586949));
#45992=CARTESIAN_POINT('Ctrl Pts',(53.0990702685024,28.3954066890209,9.49252726625751));
#45993=CARTESIAN_POINT('Ctrl Pts',(53.1023429541446,28.3852278269214,9.49321740277765));
#45994=CARTESIAN_POINT('Ctrl Pts',(53.1037094909693,28.3810255293687,9.49350182104717));
#45995=CARTESIAN_POINT('Ctrl Pts',(53.1063696633716,28.3729366149144,9.49404828209716));
#45996=CARTESIAN_POINT('Ctrl Pts',(53.1076613134889,28.3690494179567,9.49431044262206));
#45997=CARTESIAN_POINT('Ctrl Pts',(53.1107974350566,28.3597075781107,9.49493946354938));
#45998=CARTESIAN_POINT('Ctrl Pts',(53.1126535812137,28.354256851091,9.4953056493554));
#45999=CARTESIAN_POINT('Ctrl Pts',(53.1195474751755,28.3342960250955,9.49664384706668));
#46000=CARTESIAN_POINT('Ctrl Pts',(53.1247293166695,28.319835771151,9.49760785453345));
#46001=CARTESIAN_POINT('Ctrl Pts',(53.1755413179797,28.1830384014123,9.50668876950381));
#46002=CARTESIAN_POINT('Ctrl Pts',(53.2329192510483,28.0653818655933,9.51421608376746));
#46003=CARTESIAN_POINT('Ctrl Pts',(53.343425568204,27.8859015597017,9.52645647427454));
#46004=CARTESIAN_POINT('Ctrl Pts',(53.3895315308279,27.8202353933873,9.53111945293398));
#46005=CARTESIAN_POINT('Ctrl Pts',(53.4672402839038,27.7226338684504,9.5385504370169));
#46006=CARTESIAN_POINT('Ctrl Pts',(53.4961801786764,27.6886868676587,9.54123842635654));
#46007=CARTESIAN_POINT('Ctrl Pts',(53.5465529826735,27.6334610827604,9.54581594942825));
#46008=CARTESIAN_POINT('Ctrl Pts',(53.567375608819,27.6116470010812,9.54768147987465));
#46009=CARTESIAN_POINT('Ctrl Pts',(53.5965462103473,27.5824426645817,9.55026419949747));
#46010=CARTESIAN_POINT('Ctrl Pts',(53.6044741536321,27.5746372591323,9.55096313130802));
#46011=CARTESIAN_POINT('Ctrl Pts',(53.6176322581613,27.56189754124,9.55211850213845));
#46012=CARTESIAN_POINT('Ctrl Pts',(53.6228246111244,27.5569243950305,9.55257325416506));
#46013=CARTESIAN_POINT('Ctrl Pts',(53.6337063205593,27.5466142994162,9.55352392727902));
#46014=CARTESIAN_POINT('Ctrl Pts',(53.6394003149998,27.5412824442345,9.55402005415353));
#46015=CARTESIAN_POINT('Ctrl Pts',(53.6526651782905,27.5290064656959,9.55517288012548));
#46016=CARTESIAN_POINT('Ctrl Pts',(53.6602586571839,27.5220872056808,9.55583061067058));
#46017=CARTESIAN_POINT('Ctrl Pts',(53.6851645613722,27.4997423573191,9.55798102065656));
#46018=CARTESIAN_POINT('Ctrl Pts',(53.70269204625,27.4845603860608,9.55948369911505));
#46019=CARTESIAN_POINT('Ctrl Pts',(53.8487892743152,27.3624059680822,9.57192759293028));
#46020=CARTESIAN_POINT('Ctrl Pts',(53.9900595205541,27.2717063888752,9.58353597148203));
#46021=CARTESIAN_POINT('Ctrl Pts',(54.207842460338,27.1677860628093,9.60034511316957));
#46022=CARTESIAN_POINT('Ctrl Pts',(54.276469392384,27.1396166148063,9.60548955985397));
#46023=CARTESIAN_POINT('Ctrl Pts',(54.3687790892687,27.1076091008016,9.61209451489979));
#46024=CARTESIAN_POINT('Ctrl Pts',(54.3911854622391,27.1002820961431,9.61367385542165));
#46025=CARTESIAN_POINT('Ctrl Pts',(54.4290507003729,27.0886387575816,9.61629713395748));
#46026=CARTESIAN_POINT('Ctrl Pts',(54.4444408744317,27.0841088238704,9.61735082704268));
#46027=CARTESIAN_POINT('Ctrl Pts',(54.4659670015113,27.078054048192,9.61880563409571));
#46028=CARTESIAN_POINT('Ctrl Pts',(54.4720576044124,27.0763720955708,9.61921515133751));
#46029=CARTESIAN_POINT('Ctrl Pts',(54.482429374154,27.0735608467089,9.61990882631535));
#46030=CARTESIAN_POINT('Ctrl Pts',(54.4867064679319,27.072416820097,9.62019381622719));
#46031=CARTESIAN_POINT('Ctrl Pts',(54.4949375083668,27.0702445408815,9.62074017174274));
#46032=CARTESIAN_POINT('Ctrl Pts',(54.4988908318044,27.0692141872465,9.62100166190868));
#46033=CARTESIAN_POINT('Ctrl Pts',(54.5083844573914,27.0667709884579,9.62162746434251));
#46034=CARTESIAN_POINT('Ctrl Pts',(54.5139277609839,27.0653697942057,9.62199111717304));
#46035=CARTESIAN_POINT('Ctrl Pts',(54.5340857271592,27.0603665263138,9.62330742317342));
#46036=CARTESIAN_POINT('Ctrl Pts',(54.5487354462649,27.0569059579732,9.62425241733721));
#46037=CARTESIAN_POINT('Ctrl Pts',(54.6972737366062,27.0235886971723,9.63372971889622));
#46038=CARTESIAN_POINT('Ctrl Pts',(54.8338841506935,27.0074485383128,9.64160856401191));
#46039=CARTESIAN_POINT('Ctrl Pts',(55.1076711734894,27.0034795333221,9.65751678658724));
#46040=CARTESIAN_POINT('Ctrl Pts',(55.2440791306989,27.0155339251103,9.66551404193645));
#46041=CARTESIAN_POINT('Ctrl Pts',(55.3959234597077,27.0448532392174,9.6751048628551));
#46042=CARTESIAN_POINT('Ctrl Pts',(55.413622082804,27.0485208221932,9.67623298081443));
#46043=CARTESIAN_POINT('Ctrl Pts',(55.4404474455923,27.0544609989755,9.67795947653587));
#46044=CARTESIAN_POINT('Ctrl Pts',(55.4496122926045,27.0565585323131,9.67855229915918));
#46045=CARTESIAN_POINT('Ctrl Pts',(55.4655133706311,27.0603162646877,9.67958615727658));
#46046=CARTESIAN_POINT('Ctrl Pts',(55.4722564565403,27.061946974783,9.68002624514899));
#46047=CARTESIAN_POINT('Ctrl Pts',(55.4873622339189,27.0656835874223,9.68101592894047));
#46048=CARTESIAN_POINT('Ctrl Pts',(55.4957200112584,27.0678086022267,9.68156612911156));
#46049=CARTESIAN_POINT('Ctrl Pts',(55.5180331267686,27.0736361455722,9.68304218227929));
#46050=CARTESIAN_POINT('Ctrl Pts',(55.5319622775878,27.077436051199,9.68397114219285));
#46051=CARTESIAN_POINT('Ctrl Pts',(55.5944062635061,27.0952014688741,9.68817038106894));
#46052=CARTESIAN_POINT('Ctrl Pts',(55.6424179645967,27.1108534578942,9.69149449666976));
#46053=CARTESIAN_POINT('Ctrl Pts',(55.8631616941933,27.1922049157091,9.70723759566076));
#46054=CARTESIAN_POINT('Ctrl Pts',(56.0268137616826,27.2798821530425,9.7203604592127));
#46055=CARTESIAN_POINT('Ctrl Pts',(56.219636844515,27.4206238315568,9.73671485530023));
#46056=CARTESIAN_POINT('Ctrl Pts',(56.2619445606678,27.454218586595,9.74035869072997));
#46057=CARTESIAN_POINT('Ctrl Pts',(56.3099935952219,27.4956617481897,9.74451631665368));
#46058=CARTESIAN_POINT('Ctrl Pts',(56.3171029937693,27.5018823452057,9.74513199006277));
#46059=CARTESIAN_POINT('Ctrl Pts',(56.3279865516533,27.5115426277974,9.74607492724682));
#46060=CARTESIAN_POINT('Ctrl Pts',(56.3317920290417,27.5149465925349,9.74640470924202));
#46061=CARTESIAN_POINT('Ctrl Pts',(56.3387808784571,27.5212465244928,9.74701044127508));
#46062=CARTESIAN_POINT('Ctrl Pts',(56.3419679355262,27.5241381695752,9.74728669072402));
#46063=CARTESIAN_POINT('Ctrl Pts',(56.3491504332117,27.530697415725,9.74790933427302));
#46064=CARTESIAN_POINT('Ctrl Pts',(56.3531402837717,27.5343710054415,9.74825527197328));
#46065=CARTESIAN_POINT('Ctrl Pts',(56.3649062378751,27.5452933170343,9.74927579282326));
#46066=CARTESIAN_POINT('Ctrl Pts',(56.3726395785295,27.5525881129492,9.7499470144441));
#46067=CARTESIAN_POINT('Ctrl Pts',(56.4499211104742,27.6266636044718,9.75666404576276));
#46068=CARTESIAN_POINT('Ctrl Pts',(56.5146087759355,27.6983512733615,9.76236613089779));
#46069=CARTESIAN_POINT('Ctrl Pts',(56.6395177159165,27.8587601040813,9.77423558020565));
#46070=CARTESIAN_POINT('Ctrl Pts',(56.6982893321938,27.9482111100355,9.78037242202436));
#46071=CARTESIAN_POINT('Ctrl Pts',(56.7753296469176,28.088902235911,9.78985568581314));
#46072=CARTESIAN_POINT('Ctrl Pts',(56.7991432882776,28.1368793303052,9.79306062131764));
#46073=CARTESIAN_POINT('Ctrl Pts',(56.8304832998937,28.2069687799051,9.79774412149385));
#46074=CARTESIAN_POINT('Ctrl Pts',(56.8395976856202,28.2283472824962,9.7991727267698));
#46075=CARTESIAN_POINT('Ctrl Pts',(56.8552230825568,28.2668490799455,9.80174889416493));
#46076=CARTESIAN_POINT('Ctrl Pts',(56.8618757290859,28.2839122313541,9.80289172880693));
#46077=CARTESIAN_POINT('Ctrl Pts',(56.8716038384508,28.3099159792574,9.80463616493265));
#46078=CARTESIAN_POINT('Ctrl Pts',(56.8748523528716,28.318791123227,9.80523203040897));
#46079=CARTESIAN_POINT('Ctrl Pts',(56.8806260680405,28.3349194517617,9.80631589150973));
#46080=CARTESIAN_POINT('Ctrl Pts',(56.883172696741,28.3421648116684,9.80680316927669));
#46081=CARTESIAN_POINT('Ctrl Pts',(56.888561886439,28.3577852507839,9.8078545871825));
#46082=CARTESIAN_POINT('Ctrl Pts',(56.8913907052689,28.3661648645643,9.80841916656646));
#46083=CARTESIAN_POINT('Ctrl Pts',(56.8988815608539,28.3888512491494,9.80994927715174));
#46084=CARTESIAN_POINT('Ctrl Pts',(56.9034375194463,28.403192185941,9.81091824153763));
#46085=CARTESIAN_POINT('Ctrl Pts',(56.9251742786741,28.4743955588294,9.81573868131982));
#46086=CARTESIAN_POINT('Ctrl Pts',(56.9399698718405,28.5319490216354,9.81966612755386));
#46087=CARTESIAN_POINT('Ctrl Pts',(56.9800688781851,28.7229101178879,9.83280433425878));
#46088=CARTESIAN_POINT('Ctrl Pts',(56.9943286854381,28.8582369062114,9.84231208604171));
#46089=CARTESIAN_POINT('Ctrl Pts',(56.9949923949745,29.0767891165306,9.85750172841403));
#46090=CARTESIAN_POINT('Ctrl Pts',(56.9900824657855,29.1595801791502,9.86320822322789));
#46091=CARTESIAN_POINT('Ctrl Pts',(56.9781154026179,29.2575618268934,9.86974294992048));
#46092=CARTESIAN_POINT('Ctrl Pts',(56.9760069651293,29.2732675468439,9.87078354183027));
#46093=CARTESIAN_POINT('Ctrl Pts',(56.9728007347376,29.2951683548048,9.87222344242186));
#46094=CARTESIAN_POINT('Ctrl Pts',(56.971860524448,29.3013854199484,9.87263093316545));
#46095=CARTESIAN_POINT('Ctrl Pts',(56.9702090978858,29.3119667021194,9.87332220639564));
#46096=CARTESIAN_POINT('Ctrl Pts',(56.9695127430637,29.3163331613723,9.87360680745689));
#46097=CARTESIAN_POINT('Ctrl Pts',(56.968143889916,29.3247367248853,9.87415323042804));
#46098=CARTESIAN_POINT('Ctrl Pts',(56.9674734822896,29.328774100442,9.87441517228775));
#46099=CARTESIAN_POINT('Ctrl Pts',(56.965832164826,29.3384737290061,9.87504314515319));
#46100=CARTESIAN_POINT('Ctrl Pts',(56.9648492040429,29.3441339460175,9.87540850650723));
#46101=CARTESIAN_POINT('Ctrl Pts',(56.9611657809141,29.3648139595006,9.87673964521521));
#46102=CARTESIAN_POINT('Ctrl Pts',(56.9583173570028,29.3798073295202,9.87769753006313));
#46103=CARTESIAN_POINT('Ctrl Pts',(56.9290256875976,29.5248901405142,9.88690930303182));
#46104=CARTESIAN_POINT('Ctrl Pts',(56.8898266658836,29.6520851490981,9.89455289946474));
#46105=CARTESIAN_POINT('Ctrl Pts',(56.7836444059424,29.904122816633,9.91043733821508));
#46106=CARTESIAN_POINT('Ctrl Pts',(56.7154587988827,30.0276280791224,9.9186572198982));
#46107=CARTESIAN_POINT('Ctrl Pts',(56.6244826906004,30.1577612851378,9.92850396082088));
#46108=CARTESIAN_POINT('Ctrl Pts',(56.6139102949083,30.1724541491756,9.92963371510011));
#46109=CARTESIAN_POINT('Ctrl Pts',(56.597541739919,30.1945611952276,9.93136220630375));
#46110=CARTESIAN_POINT('Ctrl Pts',(56.5918904706328,30.2020818543581,9.93195536811335));
#46111=CARTESIAN_POINT('Ctrl Pts',(56.581530993039,30.2156669861914,9.93303637448017));
#46112=CARTESIAN_POINT('Ctrl Pts',(56.5768405427671,30.2217448192102,9.93352351947392));
#46113=CARTESIAN_POINT('Ctrl Pts',(56.5666506743015,30.2347923085853,9.93457698730869));
#46114=CARTESIAN_POINT('Ctrl Pts',(56.5611395956579,30.2417526079383,9.93514376425288));
#46115=CARTESIAN_POINT('Ctrl Pts',(56.5460709382021,30.260524924223,9.93668560544819));
#46116=CARTESIAN_POINT('Ctrl Pts',(56.53642471704,30.2722647123701,9.9376641921941));
#46117=CARTESIAN_POINT('Ctrl Pts',(56.4872186143846,30.3307744816435,9.94261528462617));
#46118=CARTESIAN_POINT('Ctrl Pts',(56.4456570318063,30.3758104342456,9.94666881979499));
#46119=CARTESIAN_POINT('Ctrl Pts',(56.2900758247581,30.529553162102,9.96141419288964));
#46120=CARTESIAN_POINT('Ctrl Pts',(56.1653495569065,30.6265848223277,9.97253177881446));
#46121=CARTESIAN_POINT('Ctrl Pts',(55.9910987118607,30.7317254031406,9.98657241061256));
#46122=CARTESIAN_POINT('Ctrl Pts',(55.9508422835098,30.7541519424434,9.98971988688185));
#46123=CARTESIAN_POINT('Ctrl Pts',(55.8943499612955,30.7831065022833,9.99397378403834));
#46124=CARTESIAN_POINT('Ctrl Pts',(55.8787530821983,30.790844414494,9.99513161158623));
#46125=CARTESIAN_POINT('Ctrl Pts',(55.8515867512439,30.8038817635485,9.99711725392325));
#46126=CARTESIAN_POINT('Ctrl Pts',(55.8400644126504,30.8092764339178,9.9979499292518));
#46127=CARTESIAN_POINT('Ctrl Pts',(55.8232546074597,30.8169514436016,9.99915012083318));
#46128=CARTESIAN_POINT('Ctrl Pts',(55.8180079112515,30.8193195860626,9.99952267888443));
#46129=CARTESIAN_POINT('Ctrl Pts',(55.8087917209322,30.8234314658229,10.0001734270476));
#46130=CARTESIAN_POINT('Ctrl Pts',(55.8048266971107,30.8251850173134,10.000452204058));
#46131=CARTESIAN_POINT('Ctrl Pts',(55.7963818471959,30.8288869236203,10.0010433993271));
#46132=CARTESIAN_POINT('Ctrl Pts',(55.7919005704293,30.8308317546181,10.0013556058933));
#46133=CARTESIAN_POINT('Ctrl Pts',(55.7796653729336,30.8360883852332,10.0022040244171));
#46134=CARTESIAN_POINT('Ctrl Pts',(55.7718974222734,30.8393675618542,10.0027383124441));
#46135=CARTESIAN_POINT('Ctrl Pts',(55.7351861414385,30.8545914029928,10.0052439169423));
#46136=CARTESIAN_POINT('Ctrl Pts',(55.7059832527734,30.8659034902259,10.0071803615581));
#46137=CARTESIAN_POINT('Ctrl Pts',(55.4833665999367,30.9461612293699,10.0216042786443));
#46138=CARTESIAN_POINT('Ctrl Pts',(55.2806014413385,30.9855654544182,10.0329598561837));
#46139=CARTESIAN_POINT('Ctrl Pts',(55.0205587099119,30.9953980999633,10.0485880663818));
#46140=CARTESIAN_POINT('Ctrl Pts',(54.9656885783205,30.9952087979307,10.0519356417687));
#46141=CARTESIAN_POINT('Ctrl Pts',(54.8966663524097,30.9921226627856,10.0562414441393));
#46142=CARTESIAN_POINT('Ctrl Pts',(54.8824408601993,30.9913338189283,10.0571338969357));
#46143=CARTESIAN_POINT('Ctrl Pts',(54.8596623148908,30.989825756979,10.0585714988692));
#46144=CARTESIAN_POINT('Ctrl Pts',(54.8511031645073,30.9892035938218,10.0591136243213));
#46145=CARTESIAN_POINT('Ctrl Pts',(54.8348559724147,30.9879171404027,10.0601464981653));
#46146=CARTESIAN_POINT('Ctrl Pts',(54.827167231888,30.987263429567,10.0606369078677));
#46147=CARTESIAN_POINT('Ctrl Pts',(54.8096697139541,30.9856734454236,10.0617567211384));
#46148=CARTESIAN_POINT('Ctrl Pts',(54.7998637524608,30.984709078516,10.0623869900399));
#46149=CARTESIAN_POINT('Ctrl Pts',(54.7743974470396,30.9820139473264,10.064031020264));
#46150=CARTESIAN_POINT('Ctrl Pts',(54.7587499928447,30.9801702476956,10.0650482748138));
#46151=CARTESIAN_POINT('Ctrl Pts',(54.6129358232106,30.9612353966709,10.0745961132229));
#46152=CARTESIAN_POINT('Ctrl Pts',(54.4847565821058,30.9315215476126,10.0835309761045));
#46153=CARTESIAN_POINT('Ctrl Pts',(54.2698834093651,30.8587895409991,10.0992867036722));
#46154=CARTESIAN_POINT('Ctrl Pts',(54.1816413926526,30.8216636711942,10.1059939321268));
#46155=CARTESIAN_POINT('Ctrl Pts',(54.0459512514499,30.7527181313321,10.116436364918));
#46156=CARTESIAN_POINT('Ctrl Pts',(53.9966097122881,30.7249461087004,10.1202609216073));
#46157=CARTESIAN_POINT('Ctrl Pts',(53.9403943409392,30.6900753396555,10.1245963202701));
#46158=CARTESIAN_POINT('Ctrl Pts',(53.9323131197786,30.6849817627873,10.125218988419));
#46159=CARTESIAN_POINT('Ctrl Pts',(53.9199500020293,30.6770646567884,10.1261703355741));
#46160=CARTESIAN_POINT('Ctrl Pts',(53.9156420163624,30.6742824211915,10.1265016020197));
#46161=CARTESIAN_POINT('Ctrl Pts',(53.9077399701651,30.6691357333901,10.1271087340785));
#46162=CARTESIAN_POINT('Ctrl Pts',(53.9041428402204,30.666776276315,10.1273849094593));
#46163=CARTESIAN_POINT('Ctrl Pts',(53.8960511044921,30.66143116393,10.128005732962));
#46164=CARTESIAN_POINT('Ctrl Pts',(53.8915609702659,30.6584389031172,10.1283499366483));
#46165=CARTESIAN_POINT('Ctrl Pts',(53.8783681618668,30.6495695971501,10.1293605747934));
#46166=CARTESIAN_POINT('Ctrl Pts',(53.8696995317367,30.6436419010416,10.1300237437421));
#46167=CARTESIAN_POINT('Ctrl Pts',(53.7978441631585,30.5936691512846,10.1355169785491));
#46168=CARTESIAN_POINT('Ctrl Pts',(53.7372026165893,30.5460613348966,10.1401289402219));
#46169=CARTESIAN_POINT('Ctrl Pts',(53.570576160553,30.3988853932701,10.1532093808646));
#46170=CARTESIAN_POINT('Ctrl Pts',(53.4725259012915,30.2911067530876,10.1614653410175));
#46171=CARTESIAN_POINT('Ctrl Pts',(53.3494357415144,30.1219412049327,10.1739544003478));
#46172=CARTESIAN_POINT('Ctrl Pts',(53.3143326301787,30.0684749480322,10.1778380972421));
#46173=CARTESIAN_POINT('Ctrl Pts',(53.2742761830909,30.0005636627152,10.1827471833781));
#46174=CARTESIAN_POINT('Ctrl Pts',(53.2668380374022,29.9876233734652,10.1836814787001));
#46175=CARTESIAN_POINT('Ctrl Pts',(53.2552802890311,29.966983411356,10.1851705192136));
#46176=CARTESIAN_POINT('Ctrl Pts',(53.2510647288182,29.9593378971974,10.1857218405727));
#46177=CARTESIAN_POINT('Ctrl Pts',(53.2432298588933,29.9449049683259,10.1867622493972));
#46178=CARTESIAN_POINT('Ctrl Pts',(53.2395993433071,29.9381237941058,10.1872509290967));
#46179=CARTESIAN_POINT('Ctrl Pts',(53.231521273635,29.9228233385789,10.1883533012213));
#46180=CARTESIAN_POINT('Ctrl Pts',(53.2270959077578,29.9142926195885,10.1889677577493));
#46181=CARTESIAN_POINT('Ctrl Pts',(53.215943098064,29.8924080415755,10.1905438131376));
#46182=CARTESIAN_POINT('Ctrl Pts',(53.2093039429204,29.8790100984037,10.1915084448982));
#46183=CARTESIAN_POINT('Ctrl Pts',(53.1675495408933,29.792312296337,10.1977501970633));
#46184=CARTESIAN_POINT('Ctrl Pts',(53.1367958100224,29.7170080939009,10.2031747726119));
#46185=CARTESIAN_POINT('Ctrl Pts',(53.0845700925143,29.5628491908539,10.2142760587746));
#46186=CARTESIAN_POINT('Ctrl Pts',(53.0631910746295,29.4841733732124,10.219939613526));
#46187=CARTESIAN_POINT('Ctrl Pts',(53.046686906026,29.4044694295118,10.2256126172116));
#46188=CARTESIAN_POINT('Origin',(55.,29.,3.45145488139523));
#46189=CARTESIAN_POINT('',(53.0466869981205,29.4044698742655,11.1853016190124));
#46190=CARTESIAN_POINT('',(53.0466869605703,29.4044696929239,11.0269053946991));
#46191=CARTESIAN_POINT('',(53.0466869980082,29.4044698737233,3.45145488139523));
#46192=CARTESIAN_POINT('Ctrl Pts',(53.0466869981205,29.4044698742655,11.1853016190124));
#46193=CARTESIAN_POINT('Ctrl Pts',(53.0479173957098,29.4104118535368,11.184903118068));
#46194=CARTESIAN_POINT('Ctrl Pts',(53.0491749170844,29.4163482693752,11.1845037845888));
#46195=CARTESIAN_POINT('Ctrl Pts',(53.0612457493572,29.4720758323217,11.1807436998875));
#46196=CARTESIAN_POINT('Ctrl Pts',(53.073935115407,29.5214374187202,11.1773269476064));
#46197=CARTESIAN_POINT('Ctrl Pts',(53.1370384659788,29.7329601762889,11.1623207508052));
#46198=CARTESIAN_POINT('Ctrl Pts',(53.2061450379722,29.8887813661741,11.1502458245123));
#46199=CARTESIAN_POINT('Ctrl Pts',(53.3086358224714,30.0578736706919,11.1368086806637));
#46200=CARTESIAN_POINT('Ctrl Pts',(53.3236321127687,30.0814806293452,11.1349264384882));
#46201=CARTESIAN_POINT('Ctrl Pts',(53.3492149677126,30.1199413102985,11.1318587351635));
#46202=CARTESIAN_POINT('Ctrl Pts',(53.3595173270891,30.1349785978192,11.1306590437985));
#46203=CARTESIAN_POINT('Ctrl Pts',(53.3738541828781,30.1553014647984,11.129039535674));
#46204=CARTESIAN_POINT('Ctrl Pts',(53.3777107475931,30.1607106778413,11.1286086657285));
#46205=CARTESIAN_POINT('Ctrl Pts',(53.3842203626667,30.1697452309607,11.1278894683531));
#46206=CARTESIAN_POINT('Ctrl Pts',(53.3868587385396,30.1733810180536,11.1276001636494));
#46207=CARTESIAN_POINT('Ctrl Pts',(53.3918817450293,30.1802539579623,11.1270535557052));
#46208=CARTESIAN_POINT('Ctrl Pts',(53.3942639111198,30.1834928562604,11.1267960825059));
#46209=CARTESIAN_POINT('Ctrl Pts',(53.4005282873806,30.1919564468405,11.1261235224744));
#46210=CARTESIAN_POINT('Ctrl Pts',(53.4044263450956,30.197169430461,11.1257095181733));
#46211=CARTESIAN_POINT('Ctrl Pts',(53.4180393422656,30.2151898803768,11.1242788679372));
#46212=CARTESIAN_POINT('Ctrl Pts',(53.4278838233706,30.2278993173337,11.1232707362546));
#46213=CARTESIAN_POINT('Ctrl Pts',(53.5019203996787,30.3211318586019,11.115870373929));
#46214=CARTESIAN_POINT('Ctrl Pts',(53.5721167289946,30.3967056303169,11.1098390345751));
#46215=CARTESIAN_POINT('Ctrl Pts',(53.711862243571,30.5255526901074,11.0987812377998));
#46216=CARTESIAN_POINT('Ctrl Pts',(53.7796759668888,30.5803223307149,11.0937552727402));
#46217=CARTESIAN_POINT('Ctrl Pts',(53.8971812832609,30.6631390302291,11.0852756192782));
#46218=CARTESIAN_POINT('Ctrl Pts',(53.9448812926906,30.693801743741,11.0818905250617));
#46219=CARTESIAN_POINT('Ctrl Pts',(54.0146825961297,30.7345780404748,11.0769653965981));
#46220=CARTESIAN_POINT('Ctrl Pts',(54.0357645831624,30.7463852244605,11.075481551706));
#46221=CARTESIAN_POINT('Ctrl Pts',(54.0735719803378,30.7666663503262,11.0728233446672));
#46222=CARTESIAN_POINT('Ctrl Pts',(54.0902123710778,30.7752930186779,11.0716543365598));
#46223=CARTESIAN_POINT('Ctrl Pts',(54.1154543093734,30.787930781863,11.0698813405863));
#46224=CARTESIAN_POINT('Ctrl Pts',(54.1239672621804,30.7921172385842,11.0692834401493));
#46225=CARTESIAN_POINT('Ctrl Pts',(54.1392941516113,30.7995193165221,11.0682069072867));
#46226=CARTESIAN_POINT('Ctrl Pts',(54.1460970978525,30.8027573766767,11.0677290595288));
#46227=CARTESIAN_POINT('Ctrl Pts',(54.1607322937888,30.8096219976689,11.0667009392318));
#46228=CARTESIAN_POINT('Ctrl Pts',(54.1685700407108,30.8132364093234,11.0661502621887));
#46229=CARTESIAN_POINT('Ctrl Pts',(54.1896112181133,30.8227745343384,11.0646715818871));
#46230=CARTESIAN_POINT('Ctrl Pts',(54.2028558693172,30.8286055336138,11.0637404523625));
#46231=CARTESIAN_POINT('Ctrl Pts',(54.2628790592461,30.8542549024386,11.0595182625735));
#46232=CARTESIAN_POINT('Ctrl Pts',(54.3103373569291,30.8724244171051,11.0561726463161));
#46233=CARTESIAN_POINT('Ctrl Pts',(54.5330619060581,30.9480784776424,11.0404281760269));
#46234=CARTESIAN_POINT('Ctrl Pts',(54.7150649256158,30.9828852408997,11.0273305334125));
#46235=CARTESIAN_POINT('Ctrl Pts',(54.9531032915996,30.9949287553075,11.0110024958234));
#46236=CARTESIAN_POINT('Ctrl Pts',(55.0070957009292,30.9954675712134,11.0073606422615));
#46237=CARTESIAN_POINT('Ctrl Pts',(55.0704890120499,30.9935265415539,11.0032049707928));
#46238=CARTESIAN_POINT('Ctrl Pts',(55.0799277550418,30.9931704229922,11.0025893767182));
#46239=CARTESIAN_POINT('Ctrl Pts',(55.0944641096882,30.9925185468703,11.0016465348096));
#46240=CARTESIAN_POINT('Ctrl Pts',(55.0995635591539,30.9922702444036,11.0013167695369));
#46241=CARTESIAN_POINT('Ctrl Pts',(55.1089595725383,30.9917765671847,11.000711052944));
#46242=CARTESIAN_POINT('Ctrl Pts',(55.1132562776703,30.9915368684109,11.0004348023314));
#46243=CARTESIAN_POINT('Ctrl Pts',(55.1229665896756,30.9909636352675,10.9998121370069));
#46244=CARTESIAN_POINT('Ctrl Pts',(55.1283796244238,30.9906219261404,10.9994661788346));
#46245=CARTESIAN_POINT('Ctrl Pts',(55.1443994302832,30.9895450255104,10.9984455417617));
#46246=CARTESIAN_POINT('Ctrl Pts',(55.1550019892645,30.9887470927683,10.9977742255248));
#46247=CARTESIAN_POINT('Ctrl Pts',(55.2588827455396,30.9800933644161,10.9912334696443));
#46248=CARTESIAN_POINT('Ctrl Pts',(55.3515180749092,30.9657644204252,10.9856877460274));
#46249=CARTESIAN_POINT('Ctrl Pts',(55.4830098840597,30.9358275740894,10.9778074504149));
#46250=CARTESIAN_POINT('Ctrl Pts',(55.5229119951667,30.9254324365484,10.9754154090299));
#46251=CARTESIAN_POINT('Ctrl Pts',(55.7030022551476,30.8725043358041,10.9645155078979));
#46252=CARTESIAN_POINT('Ctrl Pts',(55.8385435394685,30.815852949008,10.9559798898452));
#46253=CARTESIAN_POINT('Ctrl Pts',(55.9820615388183,30.736344700073,10.9457991949431));
#46254=CARTESIAN_POINT('Ctrl Pts',(55.9973542254578,30.7276059451016,10.9446994248852));
#46255=CARTESIAN_POINT('Ctrl Pts',(56.0205471010052,30.7139421766547,10.9430075271734));
#46256=CARTESIAN_POINT('Ctrl Pts',(56.0285321184148,30.7091623231774,10.9424206139127));
#46257=CARTESIAN_POINT('Ctrl Pts',(56.0424023387193,30.7007271737196,10.9413932595839));
#46258=CARTESIAN_POINT('Ctrl Pts',(56.0483025343716,30.6970967413966,10.9409537276399));
#46259=CARTESIAN_POINT('Ctrl Pts',(56.0615612288514,30.688843048078,10.9399602872031));
#46260=CARTESIAN_POINT('Ctrl Pts',(56.0689086300643,30.6842023097892,10.9394057444101));
#46261=CARTESIAN_POINT('Ctrl Pts',(56.0886369614801,30.6715604777657,10.937905735818));
#46262=CARTESIAN_POINT('Ctrl Pts',(56.1009597175034,30.6634700315696,10.9369569847941));
#46263=CARTESIAN_POINT('Ctrl Pts',(56.1577384577369,30.6252849613021,10.9325293727329));
#46264=CARTESIAN_POINT('Ctrl Pts',(56.2010540858673,30.5935425080134,10.9289892165654));
#46265=CARTESIAN_POINT('Ctrl Pts',(56.370142381797,30.4588183006083,10.9144885636206));
#46266=CARTESIAN_POINT('Ctrl Pts',(56.4843870804772,30.3423943466993,10.9030265472225));
#46267=CARTESIAN_POINT('Ctrl Pts',(56.6228996924192,30.1616701758897,10.8872942103337));
#46268=CARTESIAN_POINT('Ctrl Pts',(56.6600146073323,30.1079865511835,10.8828447958437));
#46269=CARTESIAN_POINT('Ctrl Pts',(56.7018652099514,30.040615501885,10.8776075479342));
#46270=CARTESIAN_POINT('Ctrl Pts',(56.7091683818849,30.0285763388076,10.8766845751651));
#46271=CARTESIAN_POINT('Ctrl Pts',(56.7193997067,30.0113002413017,10.8753795228245));
#46272=CARTESIAN_POINT('Ctrl Pts',(56.7224324712386,30.0061261917491,10.8749911236577));
#46273=CARTESIAN_POINT('Ctrl Pts',(56.7276350274129,29.9971578997408,10.874322237993));
#46274=CARTESIAN_POINT('Ctrl Pts',(56.7298157534512,29.993370084897,10.8740410600041));
#46275=CARTESIAN_POINT('Ctrl Pts',(56.7343495700943,29.9854348623235,10.8734548234153));
#46276=CARTESIAN_POINT('Ctrl Pts',(56.7367002511536,29.9812861651738,10.8731499163506));
#46277=CARTESIAN_POINT('Ctrl Pts',(56.7429082084445,29.9702376124107,10.8723420143372));
#46278=CARTESIAN_POINT('Ctrl Pts',(56.7467394328504,29.9633231058578,10.871840644242));
#46279=CARTESIAN_POINT('Ctrl Pts',(56.763105813286,29.9333667534069,10.8696859537068));
#46280=CARTESIAN_POINT('Ctrl Pts',(56.7752275405135,29.9101005103275,10.8680567871382));
#46281=CARTESIAN_POINT('Ctrl Pts',(56.8806455135975,29.6976372627188,10.8535149778111));
#46282=CARTESIAN_POINT('Ctrl Pts',(56.9438476582421,29.4949812605348,10.8418855281712));
#46283=CARTESIAN_POINT('Ctrl Pts',(56.9793533405505,29.2500399628906,10.827025941114));
#46284=CARTESIAN_POINT('Ctrl Pts',(56.9835965967408,29.21378479698,10.8248111297885));
#46285=CARTESIAN_POINT('Ctrl Pts',(56.9891602693871,29.1514851699476,10.8209652043284));
#46286=CARTESIAN_POINT('Ctrl Pts',(56.9909690288687,29.1254932779681,10.8193488151818));
#46287=CARTESIAN_POINT('Ctrl Pts',(56.992810643918,29.0886094747079,10.8170351632214));
#46288=CARTESIAN_POINT('Ctrl Pts',(56.9932642323921,29.0777405552135,10.8163509364347));
#46289=CARTESIAN_POINT('Ctrl Pts',(56.993892821994,29.0589997160505,10.8151667218523));
#46290=CARTESIAN_POINT('Ctrl Pts',(56.9941101610349,29.0511293934325,10.8146680586413));
#46291=CARTESIAN_POINT('Ctrl Pts',(56.9944370761235,29.0360579777306,10.8137104752412));
#46292=CARTESIAN_POINT('Ctrl Pts',(56.9945542585883,29.0288571602491,10.81325179936));
#46293=CARTESIAN_POINT('Ctrl Pts',(56.9947377917281,29.0119527398768,10.8121722290512));
#46294=CARTESIAN_POINT('Ctrl Pts',(56.9947723333937,29.002249041973,10.8115503564651));
#46295=CARTESIAN_POINT('Ctrl Pts',(56.994647120394,28.96874299574,10.8093953987938));
#46296=CARTESIAN_POINT('Ctrl Pts',(56.9941321359902,28.944944767473,10.8078513828529));
#46297=CARTESIAN_POINT('Ctrl Pts',(56.9872369048706,28.7706181310325,10.7964382816055));
#46298=CARTESIAN_POINT('Ctrl Pts',(56.96424702481,28.6212599827965,10.786041848419));
#46299=CARTESIAN_POINT('Ctrl Pts',(56.8939010301089,28.3629038921197,10.7673795819106));
#46300=CARTESIAN_POINT('Ctrl Pts',(56.8532208825915,28.2527847747689,10.7592059604423));
#46301=CARTESIAN_POINT('Ctrl Pts',(56.7976056360496,28.1352417241513,10.75063518569));
#46302=CARTESIAN_POINT('Ctrl Pts',(56.7919938366106,28.1236718602279,10.749793457039));
#46303=CARTESIAN_POINT('Ctrl Pts',(56.7836972318426,28.1069797484381,10.748582696393));
#46304=CARTESIAN_POINT('Ctrl Pts',(56.7811015522182,28.1018139127747,10.7482085004851));
#46305=CARTESIAN_POINT('Ctrl Pts',(56.7765185975514,28.0927910608531,10.747555900586));
#46306=CARTESIAN_POINT('Ctrl Pts',(56.7745411482423,28.0889291458236,10.7472768988925));
#46307=CARTESIAN_POINT('Ctrl Pts',(56.7703166265176,28.0807446836479,10.7466863268141));
#46308=CARTESIAN_POINT('Ctrl Pts',(56.7680663143756,28.0764239046193,10.7463749614147));
#46309=CARTESIAN_POINT('Ctrl Pts',(56.7619064716202,28.0647015374453,10.745531224554));
#46310=CARTESIAN_POINT('Ctrl Pts',(56.7579660929301,28.0573161448546,10.7450007413924));
#46311=CARTESIAN_POINT('Ctrl Pts',(56.7393686967835,28.0229814886399,10.7425386128614));
#46312=CARTESIAN_POINT('Ctrl Pts',(56.7241368926758,27.996346250165,10.7406403968461));
#46313=CARTESIAN_POINT('Ctrl Pts',(56.6019263594041,27.7936412023188,10.7262030553403));
#46314=CARTESIAN_POINT('Ctrl Pts',(56.4688612769897,27.6347391440333,10.7148138465871));
#46315=CARTESIAN_POINT('Ctrl Pts',(56.2724894900143,27.4628556887063,10.699141639253));
#46316=CARTESIAN_POINT('Ctrl Pts',(56.229703036479,27.4284174349074,10.6957908767106));
#46317=CARTESIAN_POINT('Ctrl Pts',(56.1740920263018,27.3873194408094,10.6914814773104));
#46318=CARTESIAN_POINT('Ctrl Pts',(56.1625404088881,27.3789724082071,10.6905887518947));
#46319=CARTESIAN_POINT('Ctrl Pts',(56.1438904645085,27.3657981058144,10.6891508145615));
#46320=CARTESIAN_POINT('Ctrl Pts',(56.1368485600079,27.3608915308453,10.6886086288669));
#46321=CARTESIAN_POINT('Ctrl Pts',(56.1234159129372,27.3516602927348,10.6875757076763));
#46322=CARTESIAN_POINT('Ctrl Pts',(56.1170312973135,27.3473269585053,10.6870853113305));
#46323=CARTESIAN_POINT('Ctrl Pts',(56.1024384251102,27.337545749628,10.6859656226645));
#46324=CARTESIAN_POINT('Ctrl Pts',(56.0942146795669,27.3321214537507,10.6853354657309));
#46325=CARTESIAN_POINT('Ctrl Pts',(56.0727399293934,27.318184117613,10.6836919206335));
#46326=CARTESIAN_POINT('Ctrl Pts',(56.0594278867333,27.3097668362873,10.682675042638));
#46327=CARTESIAN_POINT('Ctrl Pts',(55.9340270504829,27.2325386027843,10.6731119944592));
#46328=CARTESIAN_POINT('Ctrl Pts',(55.8155106487474,27.1748268703832,10.6641599451784));
#46329=CARTESIAN_POINT('Ctrl Pts',(55.6020376745032,27.0958412660723,10.6483501118685));
#46330=CARTESIAN_POINT('Ctrl Pts',(55.5095802179762,27.0690420951221,10.6416056283205));
#46331=CARTESIAN_POINT('Ctrl Pts',(55.3608951535313,27.0373729641743,10.6311797646546));
#46332=CARTESIAN_POINT('Ctrl Pts',(55.3057699006022,27.0280324025505,10.6274046216544));
#46333=CARTESIAN_POINT('Ctrl Pts',(55.2408713594164,27.0198234276597,10.6231177368504));
#46334=CARTESIAN_POINT('Ctrl Pts',(55.231413963883,27.0186959205171,10.6224969289618));
#46335=CARTESIAN_POINT('Ctrl Pts',(55.2168582063221,27.0170662345597,10.6215478175747));
#46336=CARTESIAN_POINT('Ctrl Pts',(55.2117655336011,27.0165159037767,10.6212169451255));
#46337=CARTESIAN_POINT('Ctrl Pts',(55.2023915699497,27.0155394373256,10.6206101861181));
#46338=CARTESIAN_POINT('Ctrl Pts',(55.1981110352372,27.0151075367222,10.6203339925379));
#46339=CARTESIAN_POINT('Ctrl Pts',(55.1884515891324,27.0141644697298,10.6197126927414));
#46340=CARTESIAN_POINT('Ctrl Pts',(55.1830719868308,27.0136613068226,10.6193680341015));
#46341=CARTESIAN_POINT('Ctrl Pts',(55.1671972038752,27.0122415529256,10.6183548081336));
#46342=CARTESIAN_POINT('Ctrl Pts',(55.1566965381588,27.0113862227185,10.6176895313233));
#46343=CARTESIAN_POINT('Ctrl Pts',(55.0665914375948,27.0047648811474,10.612019428782));
#46344=CARTESIAN_POINT('Ctrl Pts',(54.9867039625937,27.0036974297328,10.6072490160118));
#46345=CARTESIAN_POINT('Ctrl Pts',(54.7797659816205,27.0133601742127,10.5950765589432));
#46346=CARTESIAN_POINT('Ctrl Pts',(54.6534355426449,27.0314638439355,10.5878102759338));
#46347=CARTESIAN_POINT('Ctrl Pts',(54.4798802030211,27.0735706225143,10.5772330332545));
#46348=CARTESIAN_POINT('Ctrl Pts',(54.4305564535005,27.0875700711281,10.5741597757567));
#46349=CARTESIAN_POINT('Ctrl Pts',(54.3603872276319,27.1104414125342,10.5696534696104));
#46350=CARTESIAN_POINT('Ctrl Pts',(54.3390662326753,27.1177931439971,10.568266066649));
#46351=CARTESIAN_POINT('Ctrl Pts',(54.3010706376584,27.1316196606291,10.5657579652111));
#46352=CARTESIAN_POINT('Ctrl Pts',(54.2843496323999,27.1379602944284,10.564641634116));
#46353=CARTESIAN_POINT('Ctrl Pts',(54.2590079767507,27.1479616538364,10.5629295174205));
#46354=CARTESIAN_POINT('Ctrl Pts',(54.250323833365,27.1514598044487,10.5623391440559));
#46355=CARTESIAN_POINT('Ctrl Pts',(54.235252037774,27.1576547047003,10.5613079910349));
#46356=CARTESIAN_POINT('Ctrl Pts',(54.2288531736067,27.1603238863828,10.5608681430407));
#46357=CARTESIAN_POINT('Ctrl Pts',(54.2145019829606,27.1663982815804,10.5598769531324));
#46358=CARTESIAN_POINT('Ctrl Pts',(54.2065576699362,27.1698219590532,10.5593249947485));
#46359=CARTESIAN_POINT('Ctrl Pts',(54.1853019587432,27.1791467171951,10.5578392495165));
#46360=CARTESIAN_POINT('Ctrl Pts',(54.1720326874393,27.1851419651319,10.5569022841117));
#46361=CARTESIAN_POINT('Ctrl Pts',(54.1118692052364,27.2131218269267,10.5526098664729));
#46362=CARTESIAN_POINT('Ctrl Pts',(54.0657802010192,27.2367806514338,10.5491975868977));
#46363=CARTESIAN_POINT('Ctrl Pts',(53.8609279150984,27.3522249210113,10.5334474576494));
#46364=CARTESIAN_POINT('Ctrl Pts',(53.7143722319871,27.4638389675572,10.5204262365663));
#46365=CARTESIAN_POINT('Ctrl Pts',(53.5471728835833,27.6320730994778,10.5041781176262));
#46366=CARTESIAN_POINT('Ctrl Pts',(53.5107516800801,27.6718165755646,10.5005423337591));
#46367=CARTESIAN_POINT('Ctrl Pts',(53.4698898958908,27.7202032301406,10.4963926498353));
#46368=CARTESIAN_POINT('Ctrl Pts',(53.4638494511345,27.727459940722,10.4957773001635));
#46369=CARTESIAN_POINT('Ctrl Pts',(53.4546228365756,27.7387058065863,10.4948347522434));
#46370=CARTESIAN_POINT('Ctrl Pts',(53.4514001721478,27.7426646453096,10.4945050389598));
#46371=CARTESIAN_POINT('Ctrl Pts',(53.4454886793395,27.7499837455226,10.4938993710734));
#46372=CARTESIAN_POINT('Ctrl Pts',(53.4427955392515,27.7533403228703,10.4936231175417));
#46373=CARTESIAN_POINT('Ctrl Pts',(53.4367320774332,27.7609477847521,10.4930003870121));
#46374=CARTESIAN_POINT('Ctrl Pts',(53.4333682252884,27.7652037115515,10.4926543669801));
#46375=CARTESIAN_POINT('Ctrl Pts',(53.4234601155921,27.7778450608105,10.4916333764883));
#46376=CARTESIAN_POINT('Ctrl Pts',(53.4169653986011,27.7862693194231,10.4909617721521));
#46377=CARTESIAN_POINT('Ctrl Pts',(53.3506008822971,27.8737892988014,10.4840699691063));
#46378=CARTESIAN_POINT('Ctrl Pts',(53.2966346134733,27.9572057746131,10.4782138183344));
#46379=CARTESIAN_POINT('Ctrl Pts',(53.1881314881602,28.1559911507267,10.4650028524586));
#46380=CARTESIAN_POINT('Ctrl Pts',(53.1379975507274,28.2732510592699,10.4577085693707));
#46381=CARTESIAN_POINT('Ctrl Pts',(53.0811457175145,28.4517010914942,10.4465002439396));
#46382=CARTESIAN_POINT('Ctrl Pts',(53.0655119645662,28.5097057585235,10.4428451306343));
#46383=CARTESIAN_POINT('Ctrl Pts',(53.0493482015937,28.5826275201633,10.4381928876952));
#46384=CARTESIAN_POINT('Ctrl Pts',(53.046335308905,28.5969659042384,10.437275502051));
#46385=CARTESIAN_POINT('Ctrl Pts',(53.0417912933126,28.6198402932392,10.4358072478891));
#46386=CARTESIAN_POINT('Ctrl Pts',(53.0401573745232,28.6283555178188,10.4352596389853));
#46387=CARTESIAN_POINT('Ctrl Pts',(53.0371772654387,28.6444528542036,10.4342223585928));
#46388=CARTESIAN_POINT('Ctrl Pts',(53.0358193602937,28.6520326565767,10.4337330673491));
#46389=CARTESIAN_POINT('Ctrl Pts',(53.0328496574708,28.6691809486894,10.4326240746163));
#46390=CARTESIAN_POINT('Ctrl Pts',(53.0312637300384,28.6787536635291,10.432003570335));
#46391=CARTESIAN_POINT('Ctrl Pts',(53.0273637659834,28.7034082541043,10.4304016148792));
#46392=CARTESIAN_POINT('Ctrl Pts',(53.0251528556004,28.7185055765894,10.42941695894));
#46393=CARTESIAN_POINT('Ctrl Pts',(53.0111433060758,28.8224770909891,10.4226091811801));
#46394=CARTESIAN_POINT('Ctrl Pts',(53.0051764273415,28.9120211813228,10.4166051860083));
#46395=CARTESIAN_POINT('Ctrl Pts',(53.0053199386138,29.0852451139712,10.40474182193));
#46396=CARTESIAN_POINT('Ctrl Pts',(53.0106437099445,29.1687467095709,10.3989125419693));
#46397=CARTESIAN_POINT('Ctrl Pts',(53.0266490509963,29.2945956694281,10.3900729023009));
#46398=CARTESIAN_POINT('Ctrl Pts',(53.0335050515345,29.3373401353415,10.3870619400876));
#46399=CARTESIAN_POINT('Ctrl Pts',(53.0433414089626,29.388052704001,10.3834990366669));
#46400=CARTESIAN_POINT('Ctrl Pts',(53.0449883625416,29.3962666255798,10.3829222587101));
#46401=CARTESIAN_POINT('Ctrl Pts',(53.0466869980528,29.4044698739386,10.38234667127));
#46402=CARTESIAN_POINT('Ctrl Pts',(53.046686906026,29.4044694295118,10.2256126172116));
#46403=CARTESIAN_POINT('Ctrl Pts',(53.0350407226984,29.3482262607362,10.2296157780208));
#46404=CARTESIAN_POINT('Ctrl Pts',(53.0258218492307,29.2914710729161,10.2336223948554));
#46405=CARTESIAN_POINT('Ctrl Pts',(53.0139553736562,29.1911698338599,10.2405792198535));
#46406=CARTESIAN_POINT('Ctrl Pts',(53.0102590915804,29.1478200512932,10.2435455173555));
#46407=CARTESIAN_POINT('Ctrl Pts',(53.0071062847788,29.0876518767495,10.2475787081908));
#46408=CARTESIAN_POINT('Ctrl Pts',(53.0064404082734,29.0709112546044,10.2486918633672));
#46409=CARTESIAN_POINT('Ctrl Pts',(53.0056502091502,29.0418203681737,10.2506084139827));
#46410=CARTESIAN_POINT('Ctrl Pts',(53.005429534729,29.0294738671999,10.2514162463307));
#46411=CARTESIAN_POINT('Ctrl Pts',(53.0052746918278,29.0114389476523,10.2525873706492));
#46412=CARTESIAN_POINT('Ctrl Pts',(53.0052501855137,29.0057518792958,10.252955376216));
#46413=CARTESIAN_POINT('Ctrl Pts',(53.0052498607057,28.9957378010465,10.2536010117082));
#46414=CARTESIAN_POINT('Ctrl Pts',(53.0052637986602,28.991410880354,10.2538791984862));
#46415=CARTESIAN_POINT('Ctrl Pts',(53.0053237018397,28.9821596742046,10.2544722838053));
#46416=CARTESIAN_POINT('Ctrl Pts',(53.0053738218267,28.9772355041171,10.254786951314));
#46417=CARTESIAN_POINT('Ctrl Pts',(53.0055616906364,28.963702257855,10.2556490924921));
#46418=CARTESIAN_POINT('Ctrl Pts',(53.0057369467571,28.9550936890837,10.2561945361551));
#46419=CARTESIAN_POINT('Ctrl Pts',(53.0069977259391,28.9081143910642,10.2591562739429));
#46420=CARTESIAN_POINT('Ctrl Pts',(53.0091349875553,28.8697771872304,10.2615189698474));
#46421=CARTESIAN_POINT('Ctrl Pts',(53.019586270932,28.7464774220151,10.269010849271));
#46422=CARTESIAN_POINT('Ctrl Pts',(53.032246465273,28.661975556857,10.273983407082));
#46423=CARTESIAN_POINT('Ctrl Pts',(53.0821684856085,28.4310316076204,10.28771179323));
#46424=CARTESIAN_POINT('Ctrl Pts',(53.1306857634178,28.2876370783362,10.2964324430252));
#46425=CARTESIAN_POINT('Ctrl Pts',(53.2050263701861,28.1295615073894,10.3071923573722));
#46426=CARTESIAN_POINT('Ctrl Pts',(53.2155344597733,28.108217424236,10.3086698410969));
#46427=CARTESIAN_POINT('Ctrl Pts',(53.2308614757275,28.0784412317783,10.3107683386989));
#46428=CARTESIAN_POINT('Ctrl Pts',(53.2353643392029,28.0698480442936,10.3113783947861));
#46429=CARTESIAN_POINT('Ctrl Pts',(53.24331848095,28.0549341500002,10.3124451134721));
#46430=CARTESIAN_POINT('Ctrl Pts',(53.2467416628636,28.0485986013929,10.3129007841581));
#46431=CARTESIAN_POINT('Ctrl Pts',(53.2539794183607,28.0353748457618,10.3138572351222));
#46432=CARTESIAN_POINT('Ctrl Pts',(53.2578006142291,28.0284904236114,10.3143582440335));
#46433=CARTESIAN_POINT('Ctrl Pts',(53.2669992972825,28.0121465065167,10.3155550931965));
#46434=CARTESIAN_POINT('Ctrl Pts',(53.2724135783117,28.0027081128945,10.3162522372658));
#46435=CARTESIAN_POINT('Ctrl Pts',(53.2910612276461,27.9708083454527,10.3186291357621));
#46436=CARTESIAN_POINT('Ctrl Pts',(53.3046571312825,27.9485630590077,10.3203218656568));
#46437=CARTESIAN_POINT('Ctrl Pts',(53.3383407352497,27.8958033127008,10.3244239187341));
#46438=CARTESIAN_POINT('Ctrl Pts',(53.3588377833842,27.8655626339511,10.3268475452018));
#46439=CARTESIAN_POINT('Ctrl Pts',(53.5036790097016,27.6640152125446,10.343501870294));
#46440=CARTESIAN_POINT('Ctrl Pts',(53.6537460258476,27.5129196402236,10.3587083204905));
#46441=CARTESIAN_POINT('Ctrl Pts',(53.8454512160862,27.3731311190602,10.3746090677654));
#46442=CARTESIAN_POINT('Ctrl Pts',(53.8664633857991,27.3584214479719,10.3763086787094));
#46443=CARTESIAN_POINT('Ctrl Pts',(53.8942609989628,27.33974994105,10.3784955172523));
#46444=CARTESIAN_POINT('Ctrl Pts',(53.9007932989818,27.3354178812729,10.379005061237));
#46445=CARTESIAN_POINT('Ctrl Pts',(53.9113279967889,27.3285205872392,10.379819626343));
#46446=CARTESIAN_POINT('Ctrl Pts',(53.9153142458423,27.3259310128522,10.3801262139349));
#46447=CARTESIAN_POINT('Ctrl Pts',(53.9229882947404,27.320984662802,10.3807132385846));
#46448=CARTESIAN_POINT('Ctrl Pts',(53.9266746154415,27.3186257599857,10.3809938084781));
#46449=CARTESIAN_POINT('Ctrl Pts',(53.9354605608555,27.3130442401722,10.3816592212217));
#46450=CARTESIAN_POINT('Ctrl Pts',(53.940567145963,27.3098325576558,10.3820433502638));
#46451=CARTESIAN_POINT('Ctrl Pts',(53.9578162253593,27.2990929927712,10.3833323320043));
#46452=CARTESIAN_POINT('Ctrl Pts',(53.9700253293506,27.2916721998946,10.38423052009));
#46453=CARTESIAN_POINT('Ctrl Pts',(54.0400560904264,27.2501306681416,10.3893085001337));
#46454=CARTESIAN_POINT('Ctrl Pts',(54.0994973549946,27.2188116755968,10.3933344535615));
#46455=CARTESIAN_POINT('Ctrl Pts',(54.3160514350864,27.1183301816542,10.4074116833743));
#46456=CARTESIAN_POINT('Ctrl Pts',(54.4803524552498,27.066496715233,10.4171007556858));
#46457=CARTESIAN_POINT('Ctrl Pts',(54.6928507255704,27.0285418110605,10.4301569637365));
#46458=CARTESIAN_POINT('Ctrl Pts',(54.7366828672855,27.0222103981964,10.4328723853485));
#46459=CARTESIAN_POINT('Ctrl Pts',(54.7943780152452,27.0158284099807,10.4364923205691));
#46460=CARTESIAN_POINT('Ctrl Pts',(54.8080840464261,27.0144558551782,10.4373555950078));
#46461=CARTESIAN_POINT('Ctrl Pts',(54.8302467709426,27.0124680440881,10.4387573358217));
#46462=CARTESIAN_POINT('Ctrl Pts',(54.8386952488474,27.011764549097,10.4392930453349));
#46463=CARTESIAN_POINT('Ctrl Pts',(54.8548662731484,27.0105217543932,10.4403211487774));
#46464=CARTESIAN_POINT('Ctrl Pts',(54.862587992884,27.0099735112418,10.4408132543663));
#46465=CARTESIAN_POINT('Ctrl Pts',(54.8803433233945,27.008816712521,10.4419476078609));
#46466=CARTESIAN_POINT('Ctrl Pts',(54.8903786684757,27.0082390298562,10.4425908042254));
#46467=CARTESIAN_POINT('Ctrl Pts',(54.9217625901733,27.0066703211804,10.4446089515019));
#46468=CARTESIAN_POINT('Ctrl Pts',(54.9431224280297,27.0059465443453,10.4459921359856));
#46469=CARTESIAN_POINT('Ctrl Pts',(55.0481797974832,27.0040759980108,10.4528449994996));
#46470=CARTESIAN_POINT('Ctrl Pts',(55.1318704857231,27.0078551995579,10.4584644013651));
#46471=CARTESIAN_POINT('Ctrl Pts',(55.3237270353406,27.0286618493743,10.4716876386143));
#46472=CARTESIAN_POINT('Ctrl Pts',(55.4312306644319,27.0493562326891,10.4793561429385));
#46473=CARTESIAN_POINT('Ctrl Pts',(55.6158140029894,27.1008992570814,10.492649588523));
#46474=CARTESIAN_POINT('Ctrl Pts',(55.6936999077347,27.1279438821387,10.4982959963964));
#46475=CARTESIAN_POINT('Ctrl Pts',(55.7794478044841,27.1638081887538,10.5044001791477));
#46476=CARTESIAN_POINT('Ctrl Pts',(55.7891651861763,27.167963546166,10.5050902103229));
#46477=CARTESIAN_POINT('Ctrl Pts',(55.8038066109382,27.1743626418544,10.5061267839308));
#46478=CARTESIAN_POINT('Ctrl Pts',(55.8087551239265,27.1765494296717,10.5064765837486));
#46479=CARTESIAN_POINT('Ctrl Pts',(55.8176231437749,27.1805114812061,10.5071023909059));
#46480=CARTESIAN_POINT('Ctrl Pts',(55.8215458428407,27.1822793106631,10.5073788342229));
#46481=CARTESIAN_POINT('Ctrl Pts',(55.8301207040129,27.1861771428477,10.5079822959901));
#46482=CARTESIAN_POINT('Ctrl Pts',(55.8347703955529,27.1883123535018,10.5083089933811));
#46483=CARTESIAN_POINT('Ctrl Pts',(55.8480268890261,27.194461812322,10.5092390569006));
#46484=CARTESIAN_POINT('Ctrl Pts',(55.8566134478797,27.198519730605,10.5098398309845));
#46485=CARTESIAN_POINT('Ctrl Pts',(55.9149166143125,27.2265843210733,10.5139100252239));
#46486=CARTESIAN_POINT('Ctrl Pts',(55.9636518427676,27.2525870798069,10.5172672302328));
#46487=CARTESIAN_POINT('Ctrl Pts',(56.1853549714155,27.3829783601173,10.5326151036141));
#46488=CARTESIAN_POINT('Ctrl Pts',(56.3428973653652,27.5112215840867,10.5438708305135));
#46489=CARTESIAN_POINT('Ctrl Pts',(56.5023590486919,27.6872898844324,10.5583419401807));
#46490=CARTESIAN_POINT('Ctrl Pts',(56.5255062890806,27.7142625142157,10.5605323358436));
#46491=CARTESIAN_POINT('Ctrl Pts',(56.5559173241261,27.7516772772596,10.5635439997119));
#46492=CARTESIAN_POINT('Ctrl Pts',(56.5638207852027,27.7615926035183,10.5643396524925));
#46493=CARTESIAN_POINT('Ctrl Pts',(56.5761954366325,27.7774246478945,10.5656065473039));
#46494=CARTESIAN_POINT('Ctrl Pts',(56.5807291739131,27.7832922198068,10.5660753161907));
#46495=CARTESIAN_POINT('Ctrl Pts',(56.5899321204793,27.7953409521138,10.5670364379988));
#46496=CARTESIAN_POINT('Ctrl Pts',(56.5945982446578,27.80152429947,10.5675289000155));
#46497=CARTESIAN_POINT('Ctrl Pts',(56.605259469547,27.8158245813264,10.5686661201026));
#46498=CARTESIAN_POINT('Ctrl Pts',(56.6112291910843,27.8239600880884,10.5693118429407));
#46499=CARTESIAN_POINT('Ctrl Pts',(56.6297701179323,27.8496337361131,10.5713459192947));
#46500=CARTESIAN_POINT('Ctrl Pts',(56.6421182859114,27.8673302982771,10.5727426933415));
#46501=CARTESIAN_POINT('Ctrl Pts',(56.7018391537842,27.9559479068702,10.5797137639257));
#46502=CARTESIAN_POINT('Ctrl Pts',(56.7449107445599,28.029647271972,10.5854437215525));
#46503=CARTESIAN_POINT('Ctrl Pts',(56.8348137828815,28.2089372016656,10.5991979691759));
#46504=CARTESIAN_POINT('Ctrl Pts',(56.8774616090698,28.3162913452631,10.607301680632));
#46505=CARTESIAN_POINT('Ctrl Pts',(56.9158326236954,28.4441718255519,10.6165402510007));
#46506=CARTESIAN_POINT('Ctrl Pts',(56.9208302197223,28.4616962821369,10.6177971678152));
#46507=CARTESIAN_POINT('Ctrl Pts',(56.9290439595196,28.4920705440284,10.6199576824002));
#46508=CARTESIAN_POINT('Ctrl Pts',(56.9323735170887,28.5048883633434,10.6208639131236));
#46509=CARTESIAN_POINT('Ctrl Pts',(56.9464615495164,28.5614312406258,10.6248349599033));
#46510=CARTESIAN_POINT('Ctrl Pts',(56.9558662656171,28.6054838785606,10.6278593601577));
#46511=CARTESIAN_POINT('Ctrl Pts',(56.9652700431564,28.6582193667054,10.6313694031988));
#46512=CARTESIAN_POINT('Ctrl Pts',(56.9667138358292,28.6666277786656,10.6319257428232));
#46513=CARTESIAN_POINT('Ctrl Pts',(56.9689848385807,28.6803822183651,10.6328300997086));
#46514=CARTESIAN_POINT('Ctrl Pts',(56.9698443094873,28.6857227037458,10.6331798366538));
#46515=CARTESIAN_POINT('Ctrl Pts',(56.9713484150483,28.6953173760913,10.6338055774295));
#46516=CARTESIAN_POINT('Ctrl Pts',(56.9720010162079,28.6995701946013,10.6340820168166));
#46517=CARTESIAN_POINT('Ctrl Pts',(56.9733996605177,28.7088857128001,10.6346855238921));
#46518=CARTESIAN_POINT('Ctrl Pts',(56.9741399838849,28.7139491762335,10.6350122701672));
#46519=CARTESIAN_POINT('Ctrl Pts',(56.9761990774471,28.7284212315035,10.6359426132004));
#46520=CARTESIAN_POINT('Ctrl Pts',(56.9774701498546,28.7378366233103,10.6365436154714));
#46521=CARTESIAN_POINT('Ctrl Pts',(56.9856803637684,28.8021137369989,10.640619644003));
#46522=CARTESIAN_POINT('Ctrl Pts',(56.9904035269121,28.8572397402892,10.6439820863451));
#46523=CARTESIAN_POINT('Ctrl Pts',(57.0017560467262,29.1157834878625,10.6594236973491));
#46524=CARTESIAN_POINT('Ctrl Pts',(56.9795276978379,29.3192372298545,10.6707591252862));
#46525=CARTESIAN_POINT('Ctrl Pts',(56.918028907439,29.5489721143186,10.6852625930721));
#46526=CARTESIAN_POINT('Ctrl Pts',(56.9083011262369,29.5818864735817,10.6873792934897));
#46527=CARTESIAN_POINT('Ctrl Pts',(56.8938765195091,29.6264309378896,10.690304705856));
#46528=CARTESIAN_POINT('Ctrl Pts',(56.8899116326901,29.6382930365026,10.6910896869985));
#46529=CARTESIAN_POINT('Ctrl Pts',(56.8834297425095,29.6570954697695,10.6923437677455));
#46530=CARTESIAN_POINT('Ctrl Pts',(56.8809852655695,29.664060599425,10.6928104838228));
#46531=CARTESIAN_POINT('Ctrl Pts',(56.8758917249126,29.6783199993225,10.6937704809354));
#46532=CARTESIAN_POINT('Ctrl Pts',(56.8732386446973,29.685612691185,10.6942638876669));
#46533=CARTESIAN_POINT('Ctrl Pts',(56.8670035068345,29.7024452336274,10.6954084717785));
#46534=CARTESIAN_POINT('Ctrl Pts',(56.8633907912754,29.7119734218592,10.6960606557505));
#46535=CARTESIAN_POINT('Ctrl Pts',(56.8517075832032,29.7420886343454,10.6981358304062));
#46536=CARTESIAN_POINT('Ctrl Pts',(56.8433679274945,29.7625687732652,10.6995677339656));
#46537=CARTESIAN_POINT('Ctrl Pts',(56.7995789965492,29.8651853943119,10.7068499338198));
#46538=CARTESIAN_POINT('Ctrl Pts',(56.7589778640264,29.9449991381945,10.7128721331996));
#46539=CARTESIAN_POINT('Ctrl Pts',(56.6604405534051,30.1102064157275,10.7260907744026));
#46540=CARTESIAN_POINT('Ctrl Pts',(56.6009558802444,30.1943867739529,10.73331019486));
#46541=CARTESIAN_POINT('Ctrl Pts',(56.482979896208,30.3365999390005,10.7461255235278));
#46542=CARTESIAN_POINT('Ctrl Pts',(56.426878599694,30.3963342512788,10.7517364140023));
#46543=CARTESIAN_POINT('Ctrl Pts',(56.3595680370643,30.4596964989118,10.7578074190578));
#46544=CARTESIAN_POINT('Ctrl Pts',(56.3518199140318,30.4668749258188,10.7584970388792));
#46545=CARTESIAN_POINT('Ctrl Pts',(56.340018235709,30.4776359310917,10.7595331183805));
#46546=CARTESIAN_POINT('Ctrl Pts',(56.3360066686391,30.4812639872418,10.7598828309417));
#46547=CARTESIAN_POINT('Ctrl Pts',(56.3287775352729,30.4877487477433,10.7605085459773));
#46548=CARTESIAN_POINT('Ctrl Pts',(56.3255654519433,30.4906113874324,10.7607849838447));
#46549=CARTESIAN_POINT('Ctrl Pts',(56.3185125646593,30.4968561615193,10.7613885085125));
#46550=CARTESIAN_POINT('Ctrl Pts',(56.3146680045797,30.5002339119567,10.761715273762));
#46551=CARTESIAN_POINT('Ctrl Pts',(56.3036481380033,30.5098408460756,10.7626457252992));
#46552=CARTESIAN_POINT('Ctrl Pts',(56.2964411490592,30.5160337079596,10.7632468161508));
#46553=CARTESIAN_POINT('Ctrl Pts',(56.2469657134213,30.5579364054363,10.767325113329));
#46554=CARTESIAN_POINT('Ctrl Pts',(56.2032673768529,30.5919290710427,10.7706895921694));
#46555=CARTESIAN_POINT('Ctrl Pts',(55.9920541777211,30.7425566662864,10.7861683262419));
#46556=CARTESIAN_POINT('Ctrl Pts',(55.8087050722569,30.8348516582826,10.7975353488147));
#46557=CARTESIAN_POINT('Ctrl Pts',(55.5823396905267,30.9081543563048,10.8120519231057));
#46558=CARTESIAN_POINT('Ctrl Pts',(55.5498891720246,30.9177576109,10.8141396307958));
#46559=CARTESIAN_POINT('Ctrl Pts',(55.5051991105093,30.9297554558347,10.8170310409521));
#46560=CARTESIAN_POINT('Ctrl Pts',(55.4931570295078,30.9328679193741,10.8178117335872));
#46561=CARTESIAN_POINT('Ctrl Pts',(55.4739360547926,30.9376445675464,10.8190606697128));
#46562=CARTESIAN_POINT('Ctrl Pts',(55.4667755562385,30.9393819716401,10.8195265653349));
#46563=CARTESIAN_POINT('Ctrl Pts',(55.4520482564599,30.9428690776637,10.8204861451413));
#46564=CARTESIAN_POINT('Ctrl Pts',(55.4444805428587,30.9446143379468,10.8209799618274));
#46565=CARTESIAN_POINT('Ctrl Pts',(55.4269195650122,30.9485563725602,10.8221276503424));
#46566=CARTESIAN_POINT('Ctrl Pts',(55.416919275081,30.9507205242393,10.8227825463726));
#46567=CARTESIAN_POINT('Ctrl Pts',(55.3850337483867,30.9573644527695,10.8248751301049));
#46568=CARTESIAN_POINT('Ctrl Pts',(55.3630903336494,30.9615534484491,10.8263219435899));
#46569=CARTESIAN_POINT('Ctrl Pts',(55.2511602236223,30.9809784316085,10.8337386835625));
#46570=CARTESIAN_POINT('Ctrl Pts',(55.1602860144448,30.9903922589665,10.8398878143379));
#46571=CARTESIAN_POINT('Ctrl Pts',(54.9828251411902,30.9965431117853,10.852100186989));
#46572=CARTESIAN_POINT('Ctrl Pts',(54.8964526215905,30.9939298406651,10.8581365283839));
#46573=CARTESIAN_POINT('Ctrl Pts',(54.7147616270727,30.9765932393952,10.8708354484242));
#46574=CARTESIAN_POINT('Ctrl Pts',(54.6197723353993,30.9605389720721,10.8774746793239));
#46575=CARTESIAN_POINT('Ctrl Pts',(54.5159771247606,30.9351647013695,10.8844928999035));
#46576=CARTESIAN_POINT('Ctrl Pts',(54.5056710087397,30.9325577418094,10.8851870471155));
#46577=CARTESIAN_POINT('Ctrl Pts',(54.4901390399321,30.928496506684,10.8862285632749));
#46578=CARTESIAN_POINT('Ctrl Pts',(54.4848976621158,30.9271031519031,10.8865792348255));
#46579=CARTESIAN_POINT('Ctrl Pts',(54.4755075754509,30.9245658674375,10.8872059640997));
#46580=CARTESIAN_POINT('Ctrl Pts',(54.4713568417557,30.9234298775484,10.8874824636349));
#46581=CARTESIAN_POINT('Ctrl Pts',(54.4622894716872,30.9209167130579,10.8880853050008));
#46582=CARTESIAN_POINT('Ctrl Pts',(54.4573744419035,30.9195340934358,10.8884113306473));
#46583=CARTESIAN_POINT('Ctrl Pts',(54.44338098808,30.915539630377,10.8893375564395));
#46584=CARTESIAN_POINT('Ctrl Pts',(54.434315589454,30.9128821071736,10.8899351979694));
#46585=CARTESIAN_POINT('Ctrl Pts',(54.3735576568381,30.8946012034681,10.8939266984291));
#46586=CARTESIAN_POINT('Ctrl Pts',(54.322494071468,30.8769471445177,10.8972132540807));
#46587=CARTESIAN_POINT('Ctrl Pts',(54.1001235644696,30.7898070794933,10.9114780764638));
#46588=CARTESIAN_POINT('Ctrl Pts',(53.9382465763814,30.6987862041523,10.9218209064492));
#46589=CARTESIAN_POINT('Ctrl Pts',(53.751098866752,30.5562184408159,10.9359849281507));
#46590=CARTESIAN_POINT('Ctrl Pts',(53.7121657212748,30.5241561940714,10.9390668628493));
#46591=CARTESIAN_POINT('Ctrl Pts',(53.6637070203923,30.4810661323083,10.9431070734989));
#46592=CARTESIAN_POINT('Ctrl Pts',(53.6530275125162,30.4713602265913,10.9440108630092));
#46593=CARTESIAN_POINT('Ctrl Pts',(53.636137072563,30.4556716042274,10.9454624019386));
#46594=CARTESIAN_POINT('Ctrl Pts',(53.6298578667981,30.4497628893232,10.9460070213086));
#46595=CARTESIAN_POINT('Ctrl Pts',(53.6185956571647,30.439026662849,10.946993011114));
#46596=CARTESIAN_POINT('Ctrl Pts',(53.6135991311149,30.4342134860504,10.9474337618296));
#46597=CARTESIAN_POINT('Ctrl Pts',(53.6085281671203,30.4292773419323,10.9478845028505));
#46598=CARTESIAN_POINT('Ctrl Pts',(53.6084284778147,30.4291802827151,10.9478933652562));
#46599=CARTESIAN_POINT('Ctrl Pts',(53.6082328022992,30.4289897297946,10.9479107635255));
#46600=CARTESIAN_POINT('Ctrl Pts',(53.6081368154871,30.4288962369787,10.9479192993444));
#46601=CARTESIAN_POINT('Ctrl Pts',(53.6079483179992,30.4287126001484,10.9479360643327));
#46602=CARTESIAN_POINT('Ctrl Pts',(53.6078558066219,30.4286224567841,10.9479442934756));
#46603=CARTESIAN_POINT('Ctrl Pts',(53.607674050519,30.4284453186715,10.9479604634835));
#46604=CARTESIAN_POINT('Ctrl Pts',(53.6075848052084,30.4283583245622,10.9479684043198));
#46605=CARTESIAN_POINT('Ctrl Pts',(53.6007183386965,30.4216638086814,10.9485794501217));
#46606=CARTESIAN_POINT('Ctrl Pts',(53.5939883225987,30.4150082369068,10.9491846421686));
#46607=CARTESIAN_POINT('Ctrl Pts',(53.574324941759,30.3952835767955,10.9509716727746));
#46608=CARTESIAN_POINT('Ctrl Pts',(53.5615248933915,30.382083558152,10.9521592662796));
#46609=CARTESIAN_POINT('Ctrl Pts',(53.5326175947253,30.3514363484568,10.9548985449528));
#46610=CARTESIAN_POINT('Ctrl Pts',(53.5166359954398,30.3338749859522,10.9564552656265));
#46611=CARTESIAN_POINT('Ctrl Pts',(53.4645205901585,30.2745129239468,10.9616762091697));
#46612=CARTESIAN_POINT('Ctrl Pts',(53.4298126716526,30.2314995227753,10.96539414302));
#46613=CARTESIAN_POINT('Ctrl Pts',(53.3547992983306,30.1302016185715,10.9739958229886));
#46614=CARTESIAN_POINT('Ctrl Pts',(53.3157236029943,30.0710989654623,10.9789079403431));
#46615=CARTESIAN_POINT('Ctrl Pts',(53.2181185175537,29.9048761294885,10.9923366594161));
#46616=CARTESIAN_POINT('Ctrl Pts',(53.1661326736707,29.7942533014942,11.000876740139));
#46617=CARTESIAN_POINT('Ctrl Pts',(53.119202302704,29.6647377972203,11.0099993780796));
#46618=CARTESIAN_POINT('Ctrl Pts',(53.1140050060943,29.649845548715,11.0110355530373));
#46619=CARTESIAN_POINT('Ctrl Pts',(53.1069290566603,29.6287699732057,11.0124824830614));
#46620=CARTESIAN_POINT('Ctrl Pts',(53.1049031225325,29.6226372166187,11.0129012165313));
#46621=CARTESIAN_POINT('Ctrl Pts',(53.1015439296516,29.6123002224271,11.0136030041663));
#46622=CARTESIAN_POINT('Ctrl Pts',(53.1001947750544,29.6081012431901,11.0138869688013));
#46623=CARTESIAN_POINT('Ctrl Pts',(53.0974680764198,29.599517278291,11.0144651692206));
#46624=CARTESIAN_POINT('Ctrl Pts',(53.0960917445688,29.5951319543999,11.0147593343632));
#46625=CARTESIAN_POINT('Ctrl Pts',(53.0926198461209,29.5839343358586,11.015507443055));
#46626=CARTESIAN_POINT('Ctrl Pts',(53.0905455888152,29.5771154263083,11.0159601665655));
#46627=CARTESIAN_POINT('Ctrl Pts',(53.0822370125922,29.5492666030976,11.017798088019));
#46628=CARTESIAN_POINT('Ctrl Pts',(53.0763129438462,29.5281447535067,11.0191664835478));
#46629=CARTESIAN_POINT('Ctrl Pts',(53.0618155657209,29.4729708204912,11.0226850761764));
#46630=CARTESIAN_POINT('Ctrl Pts',(53.0537968846057,29.4388057818093,11.0248091069509));
#46631=CARTESIAN_POINT('Ctrl Pts',(53.0466869605703,29.4044696929237,11.0269053946991));
#46632=CARTESIAN_POINT('Origin',(55.,29.,3.45145488139523));
#46633=CARTESIAN_POINT('',(53.0466870113635,29.4044699382201,11.9837090255998));
#46634=CARTESIAN_POINT('',(53.0466869751866,29.4044697635106,11.8238528479472));
#46635=CARTESIAN_POINT('',(53.0466869980082,29.4044698737233,3.45145488139523));
#46636=CARTESIAN_POINT('',(53.0052503739419,28.9987785905819,11.2108651376668));
#46637=CARTESIAN_POINT('Ctrl Pts',(53.0466870113634,29.4044699382199,11.9837090255998));
#46638=CARTESIAN_POINT('Ctrl Pts',(53.0538097894638,29.4388680817256,11.9816662505898));
#46639=CARTESIAN_POINT('Ctrl Pts',(53.061844969036,29.4730963065561,11.9796169044452));
#46640=CARTESIAN_POINT('Ctrl Pts',(53.09498543007,29.5991713655257,11.9719638822383));
#46641=CARTESIAN_POINT('Ctrl Pts',(53.1257370561887,29.6893633633536,11.9662738775896));
#46642=CARTESIAN_POINT('Ctrl Pts',(53.1688157940404,29.7912206098217,11.9594075582874));
#46643=CARTESIAN_POINT('Ctrl Pts',(53.1749907810353,29.8053613968169,11.9584442761393));
#46644=CARTESIAN_POINT('Ctrl Pts',(53.1853364467838,29.8283229538182,11.9568629656974));
#46645=CARTESIAN_POINT('Ctrl Pts',(53.1894089606461,29.8371874401807,11.9562482680825));
#46646=CARTESIAN_POINT('Ctrl Pts',(53.1968144769038,29.8529999476218,11.955144024865));
#46647=CARTESIAN_POINT('Ctrl Pts',(53.2001230496378,29.8599592444974,11.9546553242181));
#46648=CARTESIAN_POINT('Ctrl Pts',(53.2072261186174,29.874679369694,11.9536157925928));
#46649=CARTESIAN_POINT('Ctrl Pts',(53.2110308638909,29.8824350490196,11.9530646153756));
#46650=CARTESIAN_POINT('Ctrl Pts',(53.2213592625894,29.9031473406664,11.951583177748));
#46651=CARTESIAN_POINT('Ctrl Pts',(53.2279739758153,29.9160577181682,11.950649770706));
#46652=CARTESIAN_POINT('Ctrl Pts',(53.2617914738048,29.9803244939344,11.9459520974273));
#46653=CARTESIAN_POINT('Ctrl Pts',(53.2910862348425,30.0305423812689,11.9421148823816));
#46654=CARTESIAN_POINT('Ctrl Pts',(53.3839858434895,30.1749147579098,11.9305729581624));
#46655=CARTESIAN_POINT('Ctrl Pts',(53.4534814039693,30.2649906761116,11.9226806801986));
#46656=CARTESIAN_POINT('Ctrl Pts',(53.5575751184224,30.3784306675668,11.9119501063205));
#46657=CARTESIAN_POINT('Ctrl Pts',(53.5857963253953,30.4073694310569,11.9091351249319));
#46658=CARTESIAN_POINT('Ctrl Pts',(53.6221757422883,30.4424738257972,11.9056366151245));
#46659=CARTESIAN_POINT('Ctrl Pts',(53.6295276653558,30.4494605917484,11.9049359775062));
#46660=CARTESIAN_POINT('Ctrl Pts',(53.6509347266875,30.4694959161019,11.9029148558657));
#46661=CARTESIAN_POINT('Ctrl Pts',(53.6651254282159,30.4823984858458,11.9015983446014));
#46662=CARTESIAN_POINT('Ctrl Pts',(53.7148983943834,30.5263590369731,11.8970660815459));
#46663=CARTESIAN_POINT('Ctrl Pts',(53.7513989316061,30.5563592810732,11.8938896479144));
#46664=CARTESIAN_POINT('Ctrl Pts',(53.7958037704429,30.5902873217469,11.8902269799941));
#46665=CARTESIAN_POINT('Ctrl Pts',(53.8027085526086,30.5954922505024,11.8896630115996));
#46666=CARTESIAN_POINT('Ctrl Pts',(53.8140156356351,30.6039009596227,11.8887487864025));
#46667=CARTESIAN_POINT('Ctrl Pts',(53.8183975077816,30.6071318405387,11.888396748283));
#46668=CARTESIAN_POINT('Ctrl Pts',(53.8262676947547,30.6128851688339,11.8877685668948));
#46669=CARTESIAN_POINT('Ctrl Pts',(53.829750986991,30.6154142938848,11.8874919726828));
#46670=CARTESIAN_POINT('Ctrl Pts',(53.8373704220097,30.6209089818593,11.8868900745541));
#46671=CARTESIAN_POINT('Ctrl Pts',(53.8415097304841,30.6238699947694,11.886565079314));
#46672=CARTESIAN_POINT('Ctrl Pts',(53.8533018009081,30.63223729691,11.8856447294673));
#46673=CARTESIAN_POINT('Ctrl Pts',(53.8609815053392,30.6376056393879,11.8850518826844));
#46674=CARTESIAN_POINT('Ctrl Pts',(53.9117166687611,30.672541456117,11.8811760558672));
#46675=CARTESIAN_POINT('Ctrl Pts',(53.9558854363231,30.7004650390624,11.8779933688827));
#46676=CARTESIAN_POINT('Ctrl Pts',(54.1445262919131,30.8095985842591,11.8649588488438));
#46677=CARTESIAN_POINT('Ctrl Pts',(54.2977321777928,30.8743822915618,11.8556353385642));
#46678=CARTESIAN_POINT('Ctrl Pts',(54.5232934893647,30.9381684704359,11.8416916431834));
#46679=CARTESIAN_POINT('Ctrl Pts',(54.5903082454484,30.9534321814295,11.8375318522071));
#46680=CARTESIAN_POINT('Ctrl Pts',(54.6734479399201,30.9679019476223,11.8322842268581));
#46681=CARTESIAN_POINT('Ctrl Pts',(54.6889548439021,30.9704124472356,11.8313019109951));
#46682=CARTESIAN_POINT('Ctrl Pts',(54.7133853949728,30.9740720717457,11.8297480557055));
#46683=CARTESIAN_POINT('Ctrl Pts',(54.7222901401247,30.9753444524265,11.8291803874578));
#46684=CARTESIAN_POINT('Ctrl Pts',(54.7387313690129,30.977580336771,11.828129751617));
#46685=CARTESIAN_POINT('Ctrl Pts',(54.7462653684731,30.9785610983962,11.8276473347592));
#46686=CARTESIAN_POINT('Ctrl Pts',(54.7629685407394,30.9806385143998,11.8265755560198));
#46687=CARTESIAN_POINT('Ctrl Pts',(54.7721400530382,30.9817145801723,11.8259855610913));
#46688=CARTESIAN_POINT('Ctrl Pts',(54.7984837710797,30.9846201147672,11.8242864432542));
#46689=CARTESIAN_POINT('Ctrl Pts',(54.8156723594207,30.9862902810139,11.8231723867311));
#46690=CARTESIAN_POINT('Ctrl Pts',(54.9585046570007,30.9982989767491,11.8138675277587));
#46691=CARTESIAN_POINT('Ctrl Pts',(55.0848245668128,30.9969263900102,11.8053069640964));
#46692=CARTESIAN_POINT('Ctrl Pts',(55.3452942197386,30.9693319960172,11.7871381271022));
#46693=CARTESIAN_POINT('Ctrl Pts',(55.4786256416514,30.9412411329144,11.7775475019371));
#46694=CARTESIAN_POINT('Ctrl Pts',(55.6320341887414,30.8921399300865,11.7667580337657));
#46695=CARTESIAN_POINT('Ctrl Pts',(55.6558534778024,30.8840162119009,11.7650910430821));
#46696=CARTESIAN_POINT('Ctrl Pts',(55.6868304025286,30.8727925989438,11.7629396610332));
#46697=CARTESIAN_POINT('Ctrl Pts',(55.6941314372249,30.8700988404741,11.7624338134846));
#46698=CARTESIAN_POINT('Ctrl Pts',(55.7058548877583,30.8656952904802,11.7616237373361));
#46699=CARTESIAN_POINT('Ctrl Pts',(55.7102872107107,30.8640123709163,11.761317972123));
#46700=CARTESIAN_POINT('Ctrl Pts',(55.7188041916714,30.860743747667,11.7607314524022));
#46701=CARTESIAN_POINT('Ctrl Pts',(55.7228896508877,30.8591603786117,11.7604505716039));
#46702=CARTESIAN_POINT('Ctrl Pts',(55.7326159392391,30.8553539307358,11.7597829188126));
#46703=CARTESIAN_POINT('Ctrl Pts',(55.738251968181,30.8531185489593,11.7593968739072));
#46704=CARTESIAN_POINT('Ctrl Pts',(55.7573013836866,30.8454624016728,11.7580946172874));
#46705=CARTESIAN_POINT('Ctrl Pts',(55.7706663294563,30.839921275164,11.7571852581777));
#46706=CARTESIAN_POINT('Ctrl Pts',(55.8472771708882,30.8071770414912,11.7519909041624));
#46707=CARTESIAN_POINT('Ctrl Pts',(55.9091477563348,30.7768567233536,11.7478675446533));
#46708=CARTESIAN_POINT('Ctrl Pts',(56.1428155803405,30.6469367531515,11.7321182818738));
#46709=CARTESIAN_POINT('Ctrl Pts',(56.3009187131702,30.5251358285314,11.7209488020052));
#46710=CARTESIAN_POINT('Ctrl Pts',(56.4544611727968,30.3653222830452,11.7072813000356));
#46711=CARTESIAN_POINT('Ctrl Pts',(56.470189554697,30.3483711819584,11.7058437532572));
#46712=CARTESIAN_POINT('Ctrl Pts',(56.4924671750096,30.3235084425439,11.7037503031641));
#46713=CARTESIAN_POINT('Ctrl Pts',(56.4992559379192,30.3158132437027,11.7031043907966));
#46714=CARTESIAN_POINT('Ctrl Pts',(56.5110990150491,30.3021782329434,11.7019632571737));
#46715=CARTESIAN_POINT('Ctrl Pts',(56.5161784730587,30.2962604748537,11.7014690835676));
#46716=CARTESIAN_POINT('Ctrl Pts',(56.5265979565976,30.2839763572886,11.7004454322746));
#46717=CARTESIAN_POINT('Ctrl Pts',(56.5319331579411,30.2776061221461,11.6999157721246));
#46718=CARTESIAN_POINT('Ctrl Pts',(56.5455165401668,30.2611801358291,11.6985529110487));
#46719=CARTESIAN_POINT('Ctrl Pts',(56.5537063569369,30.251076837829,11.6977173914426));
#46720=CARTESIAN_POINT('Ctrl Pts',(56.5878062896415,30.2081584707105,11.6941790443864));
#46721=CARTESIAN_POINT('Ctrl Pts',(56.612778533835,30.1746151168608,11.691439826361));
#46722=CARTESIAN_POINT('Ctrl Pts',(56.6766227509312,30.0829803829853,11.684019867879));
#46723=CARTESIAN_POINT('Ctrl Pts',(56.7135244987207,30.0235929263517,11.6792739305129));
#46724=CARTESIAN_POINT('Ctrl Pts',(56.8059840648276,29.8557325788596,11.6660710123327));
#46725=CARTESIAN_POINT('Ctrl Pts',(56.8548432237346,29.7439167276699,11.6574899931631));
#46726=CARTESIAN_POINT('Ctrl Pts',(56.8972043280262,29.6162830842908,11.648255654697));
#46727=CARTESIAN_POINT('Ctrl Pts',(56.9010926088437,29.6041820964544,11.6473857163542));
#46728=CARTESIAN_POINT('Ctrl Pts',(56.9184008720312,29.5484938820193,11.6434100451176));
#46729=CARTESIAN_POINT('Ctrl Pts',(56.9304404092784,29.5044878526238,11.6403457743088));
#46730=CARTESIAN_POINT('Ctrl Pts',(56.9429364623159,29.4517729252662,11.6367956308598));
#46731=CARTESIAN_POINT('Ctrl Pts',(56.9448577638329,29.4434288638555,11.6362372452116));
#46732=CARTESIAN_POINT('Ctrl Pts',(56.9479071435624,29.4297844608363,11.6353302405198));
#46733=CARTESIAN_POINT('Ctrl Pts',(56.9490674329746,29.4244915383214,11.6349798853519));
#46734=CARTESIAN_POINT('Ctrl Pts',(56.951110448509,29.4149868635746,11.6343534909203));
#46735=CARTESIAN_POINT('Ctrl Pts',(56.9520011235146,29.4107769395934,11.6340770119628));
#46736=CARTESIAN_POINT('Ctrl Pts',(56.9539196163733,29.4015617052602,11.6334739464279));
#46737=CARTESIAN_POINT('Ctrl Pts',(56.9549418270598,29.3965553234961,11.6331476777984));
#46738=CARTESIAN_POINT('Ctrl Pts',(56.9578026098338,29.3822644165273,11.6322200652341));
#46739=CARTESIAN_POINT('Ctrl Pts',(56.9595943841911,29.3729705095743,11.6316212919688));
#46740=CARTESIAN_POINT('Ctrl Pts',(56.9712436677294,29.3101433574549,11.6276016649165));
#46741=CARTESIAN_POINT('Ctrl Pts',(56.9789734774285,29.2562335592232,11.6242898566734));
#46742=CARTESIAN_POINT('Ctrl Pts',(57.0037781264875,29.0126322177332,11.609669940758));
#46743=CARTESIAN_POINT('Ctrl Pts',(56.995845593778,28.8214082726878,11.5990294180597));
#46744=CARTESIAN_POINT('Ctrl Pts',(56.9525953196037,28.5895599521107,11.584776824973));
#46745=CARTESIAN_POINT('Ctrl Pts',(56.9427469146776,28.5452215248382,11.5819937612321));
#46746=CARTESIAN_POINT('Ctrl Pts',(56.9279192842535,28.4878007913889,11.578296086202));
#46747=CARTESIAN_POINT('Ctrl Pts',(56.9243031840296,28.4743784284856,11.5774250121243));
#46748=CARTESIAN_POINT('Ctrl Pts',(56.9182488684211,28.4528060805927,11.5760136872611));
#46749=CARTESIAN_POINT('Ctrl Pts',(56.9158982487471,28.4446318306983,11.5754762636879));
#46750=CARTESIAN_POINT('Ctrl Pts',(56.9113105863261,28.4290541021622,11.5744469307145));
#46751=CARTESIAN_POINT('Ctrl Pts',(56.9090826192967,28.4216480953487,11.5739553233128));
#46752=CARTESIAN_POINT('Ctrl Pts',(56.9038763566283,28.4046998196502,11.5728250746603));
#46753=CARTESIAN_POINT('Ctrl Pts',(56.900869306746,28.3951666686216,11.5721855083454));
#46754=CARTESIAN_POINT('Ctrl Pts',(56.8912996301227,28.3656046258594,11.5701901133847));
#46755=CARTESIAN_POINT('Ctrl Pts',(56.884491304176,28.3456573910055,11.5688263144881));
#46756=CARTESIAN_POINT('Ctrl Pts',(56.8498311674311,28.2491400272354,11.5621400556822));
#46757=CARTESIAN_POINT('Ctrl Pts',(56.8176251675408,28.1742265167114,11.5566760275323));
#46758=CARTESIAN_POINT('Ctrl Pts',(56.7187263105764,27.9781974219045,11.5416490434608));
#46759=CARTESIAN_POINT('Ctrl Pts',(56.6438879186226,27.8616988453802,11.5318954278903));
#46760=CARTESIAN_POINT('Ctrl Pts',(56.5494951613292,27.7437112196883,11.5215201700771));
#46761=CARTESIAN_POINT('Ctrl Pts',(56.5412700791149,27.7336338170292,11.520629962992));
#46762=CARTESIAN_POINT('Ctrl Pts',(56.5039730460282,27.688839045318,11.5166570048513));
#46763=CARTESIAN_POINT('Ctrl Pts',(56.4738201013662,27.6550342048124,11.5136151319945));
#46764=CARTESIAN_POINT('Ctrl Pts',(56.4366384099086,27.6161030907107,11.5100875089959));
#46765=CARTESIAN_POINT('Ctrl Pts',(56.4306969766072,27.6099616035171,11.5095302686884));
#46766=CARTESIAN_POINT('Ctrl Pts',(56.4209273631805,27.5999920377761,11.5086247460369));
#46767=CARTESIAN_POINT('Ctrl Pts',(56.4171228123291,27.5961411031845,11.5082747367804));
#46768=CARTESIAN_POINT('Ctrl Pts',(56.4102660808543,27.5892570546196,11.5076487081754));
#46769=CARTESIAN_POINT('Ctrl Pts',(56.407219732517,27.5862182975295,11.5073722514483));
#46770=CARTESIAN_POINT('Ctrl Pts',(56.4005312713572,27.5795895410592,11.5067689393829));
#46771=CARTESIAN_POINT('Ctrl Pts',(56.3968851829895,27.5760036864981,11.5064424039287));
#46772=CARTESIAN_POINT('Ctrl Pts',(56.3864374739455,27.5658073169048,11.5055132668322));
#46773=CARTESIAN_POINT('Ctrl Pts',(56.379602331889,27.5592311303847,11.5049132491439));
#46774=CARTESIAN_POINT('Ctrl Pts',(56.3328778016414,27.5149142069323,11.5008623015948));
#46775=CARTESIAN_POINT('Ctrl Pts',(56.2914876971954,27.4787821444609,11.4975223748204));
#46776=CARTESIAN_POINT('Ctrl Pts',(56.0947852974662,27.3208921594911,11.4824678473761));
#46777=CARTESIAN_POINT('Ctrl Pts',(55.9234448269947,27.220894492859,11.4714608277996));
#46778=CARTESIAN_POINT('Ctrl Pts',(55.7035812332166,27.133035519094,11.4570844675676));
#46779=CARTESIAN_POINT('Ctrl Pts',(55.6665350575063,27.1194911271889,11.4546592651777));
#46780=CARTESIAN_POINT('Ctrl Pts',(55.6165902578969,27.102892155519,11.4513743377371));
#46781=CARTESIAN_POINT('Ctrl Pts',(55.6040261598805,27.0988545282641,11.4505467352006));
#46782=CARTESIAN_POINT('Ctrl Pts',(55.583447633618,27.0924659476589,11.4491887867839));
#46783=CARTESIAN_POINT('Ctrl Pts',(55.5754567397167,27.0900400948422,11.4486608849259));
#46784=CARTESIAN_POINT('Ctrl Pts',(55.5599903610336,27.0854507268678,11.4476378810787));
#46785=CARTESIAN_POINT('Ctrl Pts',(55.5525169732418,27.0832806373436,11.4471430027919));
#46786=CARTESIAN_POINT('Ctrl Pts',(55.5350880668318,27.0783301103488,11.4459874895153));
#46787=CARTESIAN_POINT('Ctrl Pts',(55.5251233255616,27.0755832337051,11.4453257859688));
#46788=CARTESIAN_POINT('Ctrl Pts',(55.4930009525672,27.0669964609852,11.4431890826612));
#46789=CARTESIAN_POINT('Ctrl Pts',(55.4707645475696,27.0614610425126,11.4417044058973));
#46790=CARTESIAN_POINT('Ctrl Pts',(55.3549361880035,27.0347376999368,11.4339390822388));
#46791=CARTESIAN_POINT('Ctrl Pts',(55.2600126176054,27.0199433374644,11.427459521726));
#46792=CARTESIAN_POINT('Ctrl Pts',(55.0488567160701,27.0024807283037,11.4128570621028));
#46793=CARTESIAN_POINT('Ctrl Pts',(54.9327002420843,27.0030173186758,11.4046961807989));
#46794=CARTESIAN_POINT('Ctrl Pts',(54.8040248069984,27.014855753693,11.3958023955393));
#46795=CARTESIAN_POINT('Ctrl Pts',(54.7908116447361,27.0162045976485,11.3948910869031));
#46796=CARTESIAN_POINT('Ctrl Pts',(54.728436001254,27.0232022500196,11.3906009278552));
#46797=CARTESIAN_POINT('Ctrl Pts',(54.6794768891601,27.0305477455254,11.3872681312033));
#46798=CARTESIAN_POINT('Ctrl Pts',(54.6222310056602,27.0413282946609,11.3834492880775));
#46799=CARTESIAN_POINT('Ctrl Pts',(54.6136350219797,27.0430057811014,11.3828779550546));
#46800=CARTESIAN_POINT('Ctrl Pts',(54.5996808671677,27.0458244295359,11.3819542134975));
#46801=CARTESIAN_POINT('Ctrl Pts',(54.5943159666013,27.0469311238259,11.3815999632858));
#46802=CARTESIAN_POINT('Ctrl Pts',(54.5847411719375,27.0489474078351,11.3809694158557));
#46803=CARTESIAN_POINT('Ctrl Pts',(54.5805296097572,27.0498485431788,11.3806926529407));
#46804=CARTESIAN_POINT('Ctrl Pts',(54.5713728979939,27.0518388133912,11.3800922115206));
#46805=CARTESIAN_POINT('Ctrl Pts',(54.566428971824,27.0529331376466,11.3797688298633));
#46806=CARTESIAN_POINT('Ctrl Pts',(54.552465748608,27.0560796791825,11.3788576532064));
#46807=CARTESIAN_POINT('Ctrl Pts',(54.5434563430241,27.058175853239,11.3782722876881));
#46808=CARTESIAN_POINT('Ctrl Pts',(54.4861988745874,27.071918197102,11.3745664627704));
#46809=CARTESIAN_POINT('Ctrl Pts',(54.4383807057545,27.0853000993161,11.371536445795));
#46810=CARTESIAN_POINT('Ctrl Pts',(54.2538069756808,27.1444645128716,11.3599196234041));
#46811=CARTESIAN_POINT('Ctrl Pts',(54.1216758668048,27.2032339470628,11.3517473629666));
#46812=CARTESIAN_POINT('Ctrl Pts',(53.9184069212259,27.3214718333907,11.3379180168667));
#46813=CARTESIAN_POINT('Ctrl Pts',(53.8430145038438,27.3725228420936,11.3324697879212));
#46814=CARTESIAN_POINT('Ctrl Pts',(53.759280764476,27.4379888114136,11.3258699931241));
#46815=CARTESIAN_POINT('Ctrl Pts',(53.7472980900504,27.4475821828451,11.3249116515866));
#46816=CARTESIAN_POINT('Ctrl Pts',(53.7279019400991,27.4634816046326,11.3233368335462));
#46817=CARTESIAN_POINT('Ctrl Pts',(53.72042165207,27.4697054206964,11.3227236413917));
#46818=CARTESIAN_POINT('Ctrl Pts',(53.7071019055503,27.4809537794479,11.3216210558356));
#46819=CARTESIAN_POINT('Ctrl Pts',(53.7012454126589,27.4859579193552,11.32113249723));
#46820=CARTESIAN_POINT('Ctrl Pts',(53.6891281575991,27.496433669793,11.3201136985883));
#46821=CARTESIAN_POINT('Ctrl Pts',(53.6828723379975,27.501910745286,11.3195832391479));
#46822=CARTESIAN_POINT('Ctrl Pts',(53.6663449730392,27.5165642779621,11.3181697250393));
#46823=CARTESIAN_POINT('Ctrl Pts',(53.6561340625161,27.5258081540246,11.3172838759529));
#46824=CARTESIAN_POINT('Ctrl Pts',(53.633856039885,27.5464001191484,11.3153228820191));
#46825=CARTESIAN_POINT('Ctrl Pts',(53.6218330016006,27.5577941788005,11.3142458320497));
#46826=CARTESIAN_POINT('Ctrl Pts',(53.5862915794664,27.5923265642092,11.3110046863194));
#46827=CARTESIAN_POINT('Ctrl Pts',(53.5632048138538,27.6158990693339,11.3088223648409));
#46828=CARTESIAN_POINT('Ctrl Pts',(53.4782440662304,27.7070644653922,11.3004923645913));
#46829=CARTESIAN_POINT('Ctrl Pts',(53.4204734174192,27.778314324193,11.2941948282522));
#46830=CARTESIAN_POINT('Ctrl Pts',(53.2872586678309,27.9679254346141,11.2780882970514));
#46831=CARTESIAN_POINT('Ctrl Pts',(53.219007671074,28.0907515932836,11.2682127299869));
#46832=CARTESIAN_POINT('Ctrl Pts',(53.1583928870555,28.233364184433,11.2579642444861));
#46833=CARTESIAN_POINT('Ctrl Pts',(53.1527473294175,28.2470691704283,11.2569914392865));
#46834=CARTESIAN_POINT('Ctrl Pts',(53.1451478451073,28.2661175994676,11.255657211214));
#46835=CARTESIAN_POINT('Ctrl Pts',(53.143063392378,28.2714079800785,11.255288543607));
#46836=CARTESIAN_POINT('Ctrl Pts',(53.1395232481445,28.280506817126,11.2546578098463));
#46837=CARTESIAN_POINT('Ctrl Pts',(53.1380565726748,28.2843109204666,11.2543951042004));
#46838=CARTESIAN_POINT('Ctrl Pts',(53.1350190227311,28.2922619264598,11.2538481361846));
#46839=CARTESIAN_POINT('Ctrl Pts',(53.1334503014349,28.2964096010042,11.2535640108065));
#46840=CARTESIAN_POINT('Ctrl Pts',(53.1296671302251,28.3065139484548,11.2528746865588));
#46841=CARTESIAN_POINT('Ctrl Pts',(53.1274672647498,28.312476105509,11.2524703438871));
#46842=CARTESIAN_POINT('Ctrl Pts',(53.119734640586,28.3337457938983,11.2510360570699));
#46843=CARTESIAN_POINT('Ctrl Pts',(53.1143606139754,28.3491108890693,11.2500149862326));
#46844=CARTESIAN_POINT('Ctrl Pts',(53.1015199791031,28.3873185120338,11.2475090360808));
#46845=CARTESIAN_POINT('Ctrl Pts',(53.0942767583475,28.4102339221479,11.2460350666133));
#46846=CARTESIAN_POINT('Ctrl Pts',(53.065700507284,28.5066715184883,11.2399310645363));
#46847=CARTESIAN_POINT('Ctrl Pts',(53.0481931860629,28.5812644162781,11.2354470003281));
#46848=CARTESIAN_POINT('Ctrl Pts',(53.0152780457432,28.7696556976421,11.2243161395955));
#46849=CARTESIAN_POINT('Ctrl Pts',(53.0053205872547,28.8841094408609,11.2177155023488));
#46850=CARTESIAN_POINT('Ctrl Pts',(53.0052503739419,28.9987785905819,11.2108651376668));
#46851=CARTESIAN_POINT('Ctrl Pts',(53.0052503724545,28.9987810220628,11.2108649924095));
#46852=CARTESIAN_POINT('Ctrl Pts',(53.0052251363528,29.0400776714371,11.2083979187618));
#46853=CARTESIAN_POINT('Ctrl Pts',(53.0064823250465,29.0813635842419,11.2059024965257));
#46854=CARTESIAN_POINT('Ctrl Pts',(53.0105224873157,29.1469853474418,11.201870489345));
#46855=CARTESIAN_POINT('Ctrl Pts',(53.012473669472,29.171360649133,11.2003583762426));
#46856=CARTESIAN_POINT('Ctrl Pts',(53.0158391803227,29.2055006727038,11.1982175515189));
#46857=CARTESIAN_POINT('Ctrl Pts',(53.0168786565615,29.2153007583507,11.1976003577433));
#46858=CARTESIAN_POINT('Ctrl Pts',(53.0188444825034,29.2326104578244,11.1965053329133));
#46859=CARTESIAN_POINT('Ctrl Pts',(53.0197410262588,29.2401233099652,11.1960284332538));
#46860=CARTESIAN_POINT('Ctrl Pts',(53.0215964810996,29.2549540111086,11.195083704607));
#46861=CARTESIAN_POINT('Ctrl Pts',(53.0225533064496,29.2622720022626,11.194615947827));
#46862=CARTESIAN_POINT('Ctrl Pts',(53.0245401617277,29.2768385653728,11.1936816227368));
#46863=CARTESIAN_POINT('Ctrl Pts',(53.0255695316201,29.2840871118157,11.1932150819902));
#46864=CARTESIAN_POINT('Ctrl Pts',(53.0284194031172,29.3033910996125,11.1919682465461));
#46865=CARTESIAN_POINT('Ctrl Pts',(53.0303105441874,29.3154356449729,11.1911857467973));
#46866=CARTESIAN_POINT('Ctrl Pts',(53.0365993420809,29.3532244479218,11.1887160336788));
#46867=CARTESIAN_POINT('Ctrl Pts',(53.0413920055579,29.3788986797824,11.1870165602275));
#46868=CARTESIAN_POINT('Ctrl Pts',(53.0466869981205,29.4044698742655,11.1853016190124));
#46869=CARTESIAN_POINT('',(53.0052506385882,29.0015961351009,11.0506343150513));
#46870=CARTESIAN_POINT('Ctrl Pts',(53.0466869605703,29.4044696929237,11.0269053946991));
#46871=CARTESIAN_POINT('Ctrl Pts',(53.0192628668241,29.2720300049911,11.0349911058038));
#46872=CARTESIAN_POINT('Ctrl Pts',(53.0053590218994,29.1370467887781,11.0426855070452));
#46873=CARTESIAN_POINT('Ctrl Pts',(53.0052506385882,29.0015961350858,11.0506343150522));
#46874=CARTESIAN_POINT('Ctrl Pts',(53.0052506370171,29.0015941704433,11.0506344303456));
#46875=CARTESIAN_POINT('Ctrl Pts',(53.0051767730351,28.9091698430059,11.056058275815));
#46876=CARTESIAN_POINT('Ctrl Pts',(53.0115263315731,28.8168599802161,11.06157678144));
#46877=CARTESIAN_POINT('Ctrl Pts',(53.0261316534095,28.7118025760173,11.0681441965659));
#46878=CARTESIAN_POINT('Ctrl Pts',(53.0281506133318,28.6982981820567,11.0689937331365));
#46879=CARTESIAN_POINT('Ctrl Pts',(53.0317395704682,28.6758695805716,11.070414087241));
#46880=CARTESIAN_POINT('Ctrl Pts',(53.0332320371722,28.6669333049153,11.0709824962544));
#46881=CARTESIAN_POINT('Ctrl Pts',(53.0360411853563,28.6507909005072,11.072013923958));
#46882=CARTESIAN_POINT('Ctrl Pts',(53.0373367891327,28.6435812305822,11.0724762756496));
#46883=CARTESIAN_POINT('Ctrl Pts',(53.040057152452,28.6289079205794,11.073420780494));
#46884=CARTESIAN_POINT('Ctrl Pts',(53.0414849043694,28.6214449648288,11.0739030208879));
#46885=CARTESIAN_POINT('Ctrl Pts',(53.044692251646,28.6051839115285,11.0749579151741));
#46886=CARTESIAN_POINT('Ctrl Pts',(53.0464886581377,28.5963893368791,11.0755310923333));
#46887=CARTESIAN_POINT('Ctrl Pts',(53.0515746267285,28.5723199014462,11.0771072172899));
#46888=CARTESIAN_POINT('Ctrl Pts',(53.0549843462386,28.5570713538066,11.0781139543558));
#46889=CARTESIAN_POINT('Ctrl Pts',(53.074062017748,28.4762264202601,11.083496500005));
#46890=CARTESIAN_POINT('Ctrl Pts',(53.0928683404346,28.411422938835,11.0879714208204));
#46891=CARTESIAN_POINT('Ctrl Pts',(53.1330197167672,28.2953891285185,11.0962808707681));
#46892=CARTESIAN_POINT('Ctrl Pts',(53.1532902066643,28.2438557597506,11.1000825100931));
#46893=CARTESIAN_POINT('Ctrl Pts',(53.2200644579192,28.0928603256301,11.1115177851662));
#46894=CARTESIAN_POINT('Ctrl Pts',(53.2726604718383,27.9963211116007,11.1192364239334));
#46895=CARTESIAN_POINT('Ctrl Pts',(53.3625609857995,27.8595033831485,11.1304516136219));
#46896=CARTESIAN_POINT('Ctrl Pts',(53.3940123305174,27.8156251438108,11.1340928339998));
#46897=CARTESIAN_POINT('Ctrl Pts',(53.4330166166528,27.7656257287041,11.138247880553));
#46898=CARTESIAN_POINT('Ctrl Pts',(53.4388788154513,27.7582200593934,11.1388634488277));
#46899=CARTESIAN_POINT('Ctrl Pts',(53.447990559914,27.7468757744544,11.1398062595493));
#46900=CARTESIAN_POINT('Ctrl Pts',(53.4512029024119,27.7429076491068,11.1401360191826));
#46901=CARTESIAN_POINT('Ctrl Pts',(53.4571510481737,27.7356174653597,11.1407417302603));
#46902=CARTESIAN_POINT('Ctrl Pts',(53.4598823552929,27.7322919408812,11.1410179809589));
#46903=CARTESIAN_POINT('Ctrl Pts',(53.4660804561657,27.7247949916834,11.1416406525282));
#46904=CARTESIAN_POINT('Ctrl Pts',(53.4695535089778,27.7206288576123,11.1419866168159));
#46905=CARTESIAN_POINT('Ctrl Pts',(53.4798850920328,27.7083377838782,11.1430072895517));
#46906=CARTESIAN_POINT('Ctrl Pts',(53.4867917667126,27.7002533060767,11.1436786349842));
#46907=CARTESIAN_POINT('Ctrl Pts',(53.5579917743521,27.6182483527136,11.1504930088693));
#46908=CARTESIAN_POINT('Ctrl Pts',(53.6275925076459,27.5490939764906,11.1562810465238));
#46909=CARTESIAN_POINT('Ctrl Pts',(53.7905273469978,27.4094671138518,11.1688027241763));
#46910=CARTESIAN_POINT('Ctrl Pts',(53.8855282881106,27.3415154380705,11.1754916727222));
#46911=CARTESIAN_POINT('Ctrl Pts',(54.0260812719248,27.2585393833329,11.1851957646198));
#46912=CARTESIAN_POINT('Ctrl Pts',(54.0670607519601,27.2362464219997,11.1880021767607));
#46913=CARTESIAN_POINT('Ctrl Pts',(54.1276809976627,27.205972860229,11.1921478067746));
#46914=CARTESIAN_POINT('Ctrl Pts',(54.1467283362051,27.1968357707435,11.1934495042572));
#46915=CARTESIAN_POINT('Ctrl Pts',(54.1811849419512,27.1809749923955,11.1958050348111));
#46916=CARTESIAN_POINT('Ctrl Pts',(54.1965410531613,27.174140265133,11.1968550746472));
#46917=CARTESIAN_POINT('Ctrl Pts',(54.220336124091,27.1639078145889,11.1984834000007));
#46918=CARTESIAN_POINT('Ctrl Pts',(54.2287152625281,27.1603722870987,11.1990570261803));
#46919=CARTESIAN_POINT('Ctrl Pts',(54.2371954977776,27.1568622241155,11.1996378800133));
#46920=CARTESIAN_POINT('Ctrl Pts',(54.2372728223297,27.1568302243292,11.1996431763852));
#46921=CARTESIAN_POINT('Ctrl Pts',(54.237428968657,27.1567656166584,11.1996538717335));
#46922=CARTESIAN_POINT('Ctrl Pts',(54.2375077905893,27.1567330089311,11.1996592707218));
#46923=CARTESIAN_POINT('Ctrl Pts',(54.2376669701355,27.1566671701401,11.1996701739403));
#46924=CARTESIAN_POINT('Ctrl Pts',(54.2377473279252,27.156633939236,11.1996756781836));
#46925=CARTESIAN_POINT('Ctrl Pts',(54.2379096189275,27.1565668383592,11.1996867946377));
#46926=CARTESIAN_POINT('Ctrl Pts',(54.2379915522124,27.1565329685995,11.1996924068545));
#46927=CARTESIAN_POINT('Ctrl Pts',(54.2381570354275,27.1564645737052,11.1997037420826));
#46928=CARTESIAN_POINT('Ctrl Pts',(54.2382405852373,27.1564300488745,11.1997094650868));
#46929=CARTESIAN_POINT('Ctrl Pts',(54.2383784502063,27.1563730906598,11.1997189086266));
#46930=CARTESIAN_POINT('Ctrl Pts',(54.2384327641477,27.1563506539394,11.1997226290615));
#46931=CARTESIAN_POINT('Ctrl Pts',(54.2385464369865,27.1563037023418,11.1997304155308));
#46932=CARTESIAN_POINT('Ctrl Pts',(54.2386057961258,27.1562791879107,11.1997344815843));
#46933=CARTESIAN_POINT('Ctrl Pts',(54.2387300408201,27.1562278837454,11.1997429922784));
#46934=CARTESIAN_POINT('Ctrl Pts',(54.2387949264862,27.1562010946189,11.1997474369296));
#46935=CARTESIAN_POINT('Ctrl Pts',(54.2389307532673,27.156145024665,11.1997567410669));
#46936=CARTESIAN_POINT('Ctrl Pts',(54.239001694661,27.1561157445053,11.1997616005757));
#46937=CARTESIAN_POINT('Ctrl Pts',(54.2391502150572,27.1560544546284,11.1997717743174));
#46938=CARTESIAN_POINT('Ctrl Pts',(54.2392277944371,27.1560224456935,11.1997770885805));
#46939=CARTESIAN_POINT('Ctrl Pts',(54.2393902319972,27.1559554366164,11.1997882157666));
#46940=CARTESIAN_POINT('Ctrl Pts',(54.2394750905147,27.1559204374598,11.1997940287178));
#46941=CARTESIAN_POINT('Ctrl Pts',(54.2396527919452,27.1558471604044,11.1998062016306));
#46942=CARTESIAN_POINT('Ctrl Pts',(54.2397456354921,27.1558088835938,11.1998125616418));
#46943=CARTESIAN_POINT('Ctrl Pts',(54.2399400852995,27.1557287345289,11.1998258820107));
#46944=CARTESIAN_POINT('Ctrl Pts',(54.2400416920212,27.1556868637048,11.1998328424074));
#46945=CARTESIAN_POINT('Ctrl Pts',(54.2402545256621,27.1555991782713,11.199847422311));
#46946=CARTESIAN_POINT('Ctrl Pts',(54.2403657532592,27.1555533653291,11.1998550418734));
#46947=CARTESIAN_POINT('Ctrl Pts',(54.2405987740959,27.1554574122718,11.1998710049035));
#46948=CARTESIAN_POINT('Ctrl Pts',(54.2407205682898,27.1554072741037,11.1998793484474));
#46949=CARTESIAN_POINT('Ctrl Pts',(54.2409757658472,27.1553022482591,11.1998968309617));
#46950=CARTESIAN_POINT('Ctrl Pts',(54.2411091700964,27.1552473630328,11.1999059700057));
#46951=CARTESIAN_POINT('Ctrl Pts',(54.2413887383561,27.1551323784122,11.1999251223841));
#46952=CARTESIAN_POINT('Ctrl Pts',(54.2415349035882,27.1550722819034,11.1999351358179));
#46953=CARTESIAN_POINT('Ctrl Pts',(54.2418412649093,27.1549463625951,11.1999561241052));
#46954=CARTESIAN_POINT('Ctrl Pts',(54.2420014623424,27.1548805433249,11.19996709907));
#46955=CARTESIAN_POINT('Ctrl Pts',(54.2422949223019,27.154760016019,11.1999872039255));
#46956=CARTESIAN_POINT('Ctrl Pts',(54.242428186415,27.154705299819,11.1999963338896));
#46957=CARTESIAN_POINT('Ctrl Pts',(54.2427699477376,27.1545650211291,11.2000197482638));
#46958=CARTESIAN_POINT('Ctrl Pts',(54.2429784488883,27.1544794814349,11.2000340330585));
#46959=CARTESIAN_POINT('Ctrl Pts',(54.2435129074148,27.1542603202635,11.2000706502894));
#46960=CARTESIAN_POINT('Ctrl Pts',(54.2438388826662,27.1541267510385,11.2000929842324));
#46961=CARTESIAN_POINT('Ctrl Pts',(54.2513582620289,27.1510479914536,11.2006081797998));
#46962=CARTESIAN_POINT('Ctrl Pts',(54.2585687020462,27.1481448195484,11.2011024427319));
#46963=CARTESIAN_POINT('Ctrl Pts',(54.2751881568124,27.1415658758767,11.2022423040393));
#46964=CARTESIAN_POINT('Ctrl Pts',(54.2846084311702,27.1379193092652,11.2028888625588));
#46965=CARTESIAN_POINT('Ctrl Pts',(54.3148458457613,27.126477794034,11.2049659008887));
#46966=CARTESIAN_POINT('Ctrl Pts',(54.3357651494386,27.1189594186327,11.2064054551363));
#46967=CARTESIAN_POINT('Ctrl Pts',(54.5213715369854,27.0557348590577,11.2192052769545));
#46968=CARTESIAN_POINT('Ctrl Pts',(54.6925313301588,27.0214422622765,11.2312956838045));
#46969=CARTESIAN_POINT('Ctrl Pts',(54.9657041672717,27.0030389612919,11.2503567917627));
#46970=CARTESIAN_POINT('Ctrl Pts',(55.0658647217664,27.0038296361361,11.2572723810671));
#46971=CARTESIAN_POINT('Ctrl Pts',(55.1764623906592,27.0130404073134,11.2645641521427));
#46972=CARTESIAN_POINT('Ctrl Pts',(55.1873642100168,27.0140387556618,11.2652790987927));
#46973=CARTESIAN_POINT('Ctrl Pts',(55.2036468969991,27.0156651394719,11.266340670464));
#46974=CARTESIAN_POINT('Ctrl Pts',(55.2090341084174,27.0162254058106,11.2666908717954));
#46975=CARTESIAN_POINT('Ctrl Pts',(55.2182861419752,27.0172257183547,11.2672904708707));
#46976=CARTESIAN_POINT('Ctrl Pts',(55.2221520181459,27.0176551325566,11.2675404522504));
#46977=CARTESIAN_POINT('Ctrl Pts',(55.2309297652658,27.0186561484762,11.2681067791808));
#46978=CARTESIAN_POINT('Ctrl Pts',(55.2358407766467,27.0192347075428,11.268422732906));
#46979=CARTESIAN_POINT('Ctrl Pts',(55.2491678441229,27.0208550175699,11.2692778264275));
#46980=CARTESIAN_POINT('Ctrl Pts',(55.2575796038254,27.0219321978807,11.2698150357994));
#46981=CARTESIAN_POINT('Ctrl Pts',(55.2986067582139,27.0274521429859,11.2724240676346));
#46982=CARTESIAN_POINT('Ctrl Pts',(55.3311176842266,27.0326483754199,11.2744571672946));
#46983=CARTESIAN_POINT('Ctrl Pts',(55.5636799573556,27.0757479214197,11.2888485689236));
#46984=CARTESIAN_POINT('Ctrl Pts',(55.7570269342608,27.1432795891194,11.3001195995548));
#46985=CARTESIAN_POINT('Ctrl Pts',(55.9851235877938,27.2646174476047,11.315637204581));
#46986=CARTESIAN_POINT('Ctrl Pts',(56.0323460457051,27.2922875191933,11.3189765773551));
#46987=CARTESIAN_POINT('Ctrl Pts',(56.0903450285641,27.3295575613019,11.3232731226583));
#46988=CARTESIAN_POINT('Ctrl Pts',(56.1022383607847,27.3373813420324,11.3241648735549));
#46989=CARTESIAN_POINT('Ctrl Pts',(56.1211632839835,27.3501230177068,11.3256016126305));
#46990=CARTESIAN_POINT('Ctrl Pts',(56.1282487965111,27.3549602389235,11.3261435836601));
#46991=CARTESIAN_POINT('Ctrl Pts',(56.1416480140955,27.3642350637088,11.3271763375125));
#46992=CARTESIAN_POINT('Ctrl Pts',(56.1479676173911,27.3686639029365,11.3276667828341));
#46993=CARTESIAN_POINT('Ctrl Pts',(56.1623010398905,27.3788334353158,11.328786920785));
#46994=CARTESIAN_POINT('Ctrl Pts',(56.170298273157,27.3845970521586,11.3294174806135));
#46995=CARTESIAN_POINT('Ctrl Pts',(56.190977627709,27.3997348472565,11.3310627694155));
#46996=CARTESIAN_POINT('Ctrl Pts',(56.2035916861997,27.4092004217546,11.3320810004226));
#46997=CARTESIAN_POINT('Ctrl Pts',(56.3198912977781,27.4986466006772,11.3416082309948));
#46998=CARTESIAN_POINT('Ctrl Pts',(56.4155582209887,27.5884907417956,11.3505192794644));
#46999=CARTESIAN_POINT('Ctrl Pts',(56.5642008691953,27.7585033218186,11.3662031736123));
#47000=CARTESIAN_POINT('Ctrl Pts',(56.6215010430894,27.8343357128936,11.3728620074662));
#47001=CARTESIAN_POINT('Ctrl Pts',(56.7045000295729,27.962206410939,11.383326558291));
#47002=CARTESIAN_POINT('Ctrl Pts',(56.733717580542,28.0117892052258,11.3872159803154));
#47003=CARTESIAN_POINT('Ctrl Pts',(56.7652595442498,28.0710337795722,11.3916149595212));
#47004=CARTESIAN_POINT('Ctrl Pts',(56.7697045602931,28.0795298617922,11.3922400129659));
#47005=CARTESIAN_POINT('Ctrl Pts',(56.7764362293486,28.0926256213812,11.3931942263326));
#47006=CARTESIAN_POINT('Ctrl Pts',(56.7787665945079,28.0972024902508,11.3935259974834));
#47007=CARTESIAN_POINT('Ctrl Pts',(56.7830162067056,28.105629119362,11.3941336094542));
#47008=CARTESIAN_POINT('Ctrl Pts',(56.7849406731348,28.1094760757955,11.3944097635522));
#47009=CARTESIAN_POINT('Ctrl Pts',(56.7892470684695,28.1181544889911,11.3950299857938));
#47010=CARTESIAN_POINT('Ctrl Pts',(56.7916218764551,28.1229893781989,11.3953736134827));
#47011=CARTESIAN_POINT('Ctrl Pts',(56.7985497886887,28.1372395489647,11.39638097881));
#47012=CARTESIAN_POINT('Ctrl Pts',(56.8030485498886,28.1466812575976,11.3970414824349));
#47013=CARTESIAN_POINT('Ctrl Pts',(56.8379331835604,28.2214026429685,11.40221752678));
#47014=CARTESIAN_POINT('Ctrl Pts',(56.8648420246144,28.2882564661799,11.4065429188741));
#47015=CARTESIAN_POINT('Ctrl Pts',(56.9444395663345,28.521775064005,11.4210962456151));
#47016=CARTESIAN_POINT('Ctrl Pts',(56.9788354861453,28.6938036829274,11.4309528728006));
#47017=CARTESIAN_POINT('Ctrl Pts',(56.9932374945223,28.9111594352699,11.4441485162267));
#47018=CARTESIAN_POINT('Ctrl Pts',(56.9946923734695,28.9542804791905,11.4467975103225));
#47019=CARTESIAN_POINT('Ctrl Pts',(56.99476537855,29.0105619864894,11.4503105398052));
#47020=CARTESIAN_POINT('Ctrl Pts',(56.9946524120196,29.0237110350117,11.4511352144567));
#47021=CARTESIAN_POINT('Ctrl Pts',(56.994255339853,29.0451969973119,11.4524895721761));
#47022=CARTESIAN_POINT('Ctrl Pts',(56.9940489264057,29.0535350800062,11.4530168362547));
#47023=CARTESIAN_POINT('Ctrl Pts',(56.9935487268386,29.06965385284,11.4540394640852));
#47024=CARTESIAN_POINT('Ctrl Pts',(56.9932616646249,29.0774346113075,11.4545346096159));
#47025=CARTESIAN_POINT('Ctrl Pts',(56.9924940056851,29.0953882406103,11.4556807000366));
#47026=CARTESIAN_POINT('Ctrl Pts',(56.9919810434053,29.1055594407311,11.456332639337));
#47027=CARTESIAN_POINT('Ctrl Pts',(56.990074019455,29.13837510108,11.4584448037075));
#47028=CARTESIAN_POINT('Ctrl Pts',(56.9883715616364,29.1609991750557,11.4599145400454));
#47029=CARTESIAN_POINT('Ctrl Pts',(56.9706370009248,29.352873172703,11.4724992754705));
#47030=CARTESIAN_POINT('Ctrl Pts',(56.9334156968592,29.5194328918238,11.4843076048697));
#47031=CARTESIAN_POINT('Ctrl Pts',(56.8407904073717,29.7752031435464,11.5032528194016));
#47032=CARTESIAN_POINT('Ctrl Pts',(56.7987082313077,29.8683908740254,11.5103225661561));
#47033=CARTESIAN_POINT('Ctrl Pts',(56.744085483942,29.9681573558627,11.5178044196688));
#47034=CARTESIAN_POINT('Ctrl Pts',(56.7384105845374,29.9783105314687,11.5185646924057));
#47035=CARTESIAN_POINT('Ctrl Pts',(56.7298966243721,29.9932351392568,11.5196798975187));
#47036=CARTESIAN_POINT('Ctrl Pts',(56.7271260534956,29.998045074131,11.5200389434309));
#47037=CARTESIAN_POINT('Ctrl Pts',(56.7221867913369,30.0065378698789,11.5206721704081));
#47038=CARTESIAN_POINT('Ctrl Pts',(56.7200263062706,30.0102253880732,11.520946863337));
#47039=CARTESIAN_POINT('Ctrl Pts',(56.7153146800594,30.018208263435,11.5215409702845));
#47040=CARTESIAN_POINT('Ctrl Pts',(56.712759251383,30.0225009865374,11.5218601041405));
#47041=CARTESIAN_POINT('Ctrl Pts',(56.7057089265652,30.0342438431595,11.5227322917705));
#47042=CARTESIAN_POINT('Ctrl Pts',(56.7011813069444,30.0416743429283,11.5232832841574));
#47043=CARTESIAN_POINT('Ctrl Pts',(56.6779296990015,30.0792777475948,11.5260683514539));
#47044=CARTESIAN_POINT('Ctrl Pts',(56.6584497701847,30.1089784716266,11.5282571768284));
#47045=CARTESIAN_POINT('Ctrl Pts',(56.5235827966939,30.3030988308923,11.5426002473784));
#47046=CARTESIAN_POINT('Ctrl Pts',(56.384718077233,30.4498083940027,11.5537364029792));
#47047=CARTESIAN_POINT('Ctrl Pts',(56.1832905434293,30.606804112294,11.5690775599648));
#47048=CARTESIAN_POINT('Ctrl Pts',(56.1389675135638,30.6385201148349,11.5724032847463));
#47049=CARTESIAN_POINT('Ctrl Pts',(56.0815140352899,30.6761733422431,11.5766844254249));
#47050=CARTESIAN_POINT('Ctrl Pts',(56.0695405298957,30.6838386859315,11.5775750040077));
#47051=CARTESIAN_POINT('Ctrl Pts',(56.0502154314054,30.6959211780004,11.5790103019502));
#47052=CARTESIAN_POINT('Ctrl Pts',(56.0429153689251,30.7004201315897,11.5795520150633));
#47053=CARTESIAN_POINT('Ctrl Pts',(56.028990297087,30.7088786079672,11.5805845690374));
#47054=CARTESIAN_POINT('Ctrl Pts',(56.0223708568591,30.7128470324534,11.5810750743839));
#47055=CARTESIAN_POINT('Ctrl Pts',(56.0072381223122,30.7218002934895,11.5821957572079));
#47056=CARTESIAN_POINT('Ctrl Pts',(55.998710595643,30.7267605584172,11.5828268050143));
#47057=CARTESIAN_POINT('Ctrl Pts',(55.9764346339918,30.7394977617485,11.584474205524));
#47058=CARTESIAN_POINT('Ctrl Pts',(55.9626302119269,30.7471748936516,11.5854940750603));
#47059=CARTESIAN_POINT('Ctrl Pts',(55.8487434066712,30.8087520015826,11.5939014310232));
#47060=CARTESIAN_POINT('Ctrl Pts',(55.7443292361195,30.8541616358887,11.6015864159689));
#47061=CARTESIAN_POINT('Ctrl Pts',(55.5191178840482,30.9300052446717,11.6180157406892));
#47062=CARTESIAN_POINT('Ctrl Pts',(55.3981702014958,30.9585362527315,11.6267587365386));
#47063=CARTESIAN_POINT('Ctrl Pts',(55.229270909195,30.9820765757837,11.6383863038472));
#47064=CARTESIAN_POINT('Ctrl Pts',(55.1829704066307,30.9868858300555,11.6415124074608));
#47065=CARTESIAN_POINT('Ctrl Pts',(55.1274674476777,30.9906939280707,11.6451551823163));
#47066=CARTESIAN_POINT('Ctrl Pts',(55.1183903006699,30.9912543809673,11.6457475911816));
#47067=CARTESIAN_POINT('Ctrl Pts',(55.1042870712974,30.9920283806608,11.646662504895));
#47068=CARTESIAN_POINT('Ctrl Pts',(55.0992636172063,30.9922850193292,11.6469873035451));
#47069=CARTESIAN_POINT('Ctrl Pts',(55.0899335041494,30.9927263002338,11.6475884722788));
#47070=CARTESIAN_POINT('Ctrl Pts',(55.0856272482452,30.9929159836027,11.647865106625));
#47071=CARTESIAN_POINT('Ctrl Pts',(55.0758010861741,30.993316901565,11.6484944737691));
#47072=CARTESIAN_POINT('Ctrl Pts',(55.0702808997442,30.9935191676066,11.64884670693));
#47073=CARTESIAN_POINT('Ctrl Pts',(55.0558537119054,30.993987795505,11.64976395579));
#47074=CARTESIAN_POINT('Ctrl Pts',(55.0469455263116,30.9942174129774,11.6503270090435));
#47075=CARTESIAN_POINT('Ctrl Pts',(54.985534342647,30.9953886148407,11.6541876066196));
#47076=CARTESIAN_POINT('Ctrl Pts',(54.9330085987675,30.9943164685395,11.6573841402503));
#47077=CARTESIAN_POINT('Ctrl Pts',(54.762663358078,30.9841002088027,11.6675820582695));
#47078=CARTESIAN_POINT('Ctrl Pts',(54.6456000893342,30.9665671405793,11.674338794889));
#47079=CARTESIAN_POINT('Ctrl Pts',(54.4310573289674,30.914642796971,11.6872228406813));
#47080=CARTESIAN_POINT('Ctrl Pts',(54.3333655511008,30.8828562472095,11.6932959173462));
#47081=CARTESIAN_POINT('Ctrl Pts',(54.216655678899,30.8346554927968,11.7010785500937));
#47082=CARTESIAN_POINT('Ctrl Pts',(54.1949169279538,30.8252206102214,11.702551157675));
#47083=CARTESIAN_POINT('Ctrl Pts',(54.1638179458321,30.8110596021933,11.704693600754));
#47084=CARTESIAN_POINT('Ctrl Pts',(54.1543182873272,30.8066432255937,11.7053529237307));
#47085=CARTESIAN_POINT('Ctrl Pts',(54.1378033478903,30.7988066601301,11.7065078914939));
#47086=CARTESIAN_POINT('Ctrl Pts',(54.1307724733942,30.7954197201834,11.707002386718));
#47087=CARTESIAN_POINT('Ctrl Pts',(54.116308301459,30.7883471085804,11.7080255454397));
#47088=CARTESIAN_POINT('Ctrl Pts',(54.108877772405,30.7846561492121,11.708554384587));
#47089=CARTESIAN_POINT('Ctrl Pts',(54.08991049671,30.7750865643953,11.7099126974463));
#47090=CARTESIAN_POINT('Ctrl Pts',(54.0784077102076,30.7691418409684,11.7107444599615));
#47091=CARTESIAN_POINT('Ctrl Pts',(54.0338060328609,30.7455383491732,11.7140014929461));
#47092=CARTESIAN_POINT('Ctrl Pts',(54.0011518347511,30.727060201742,11.716455327511));
#47093=CARTESIAN_POINT('Ctrl Pts',(53.8455808004784,30.6331385214987,11.7284941146177));
#47094=CARTESIAN_POINT('Ctrl Pts',(53.7305862545401,30.5454453602615,11.7385170621569));
#47095=CARTESIAN_POINT('Ctrl Pts',(53.554418469581,30.3780742330368,11.7554478092301));
#47096=CARTESIAN_POINT('Ctrl Pts',(53.4879209909797,30.3047664452506,11.7623080824137));
#47097=CARTESIAN_POINT('Ctrl Pts',(53.4165316190242,30.2132403889172,11.7700068399111));
#47098=CARTESIAN_POINT('Ctrl Pts',(53.4061121366401,30.1995190210127,11.7711397341577));
#47099=CARTESIAN_POINT('Ctrl Pts',(53.3920085517055,30.1804377568026,11.7726842012654));
#47100=CARTESIAN_POINT('Ctrl Pts',(53.3881712780076,30.1751927370725,11.77310557299));
#47101=CARTESIAN_POINT('Ctrl Pts',(53.3817423034834,30.166314496629,11.7738133735093));
#47102=CARTESIAN_POINT('Ctrl Pts',(53.379137060122,30.162691192376,11.7741007146021));
#47103=CARTESIAN_POINT('Ctrl Pts',(53.3741925220906,30.1557655402927,11.7746470061117));
#47104=CARTESIAN_POINT('Ctrl Pts',(53.3718510931912,30.1524647835488,11.774906106986));
#47105=CARTESIAN_POINT('Ctrl Pts',(53.3663105937225,30.144603650465,11.7755202545913));
#47106=CARTESIAN_POINT('Ctrl Pts',(53.3631205283975,30.1400369248669,11.7758746962761));
#47107=CARTESIAN_POINT('Ctrl Pts',(53.3519231939686,30.1238635289034,11.7771219969975));
#47108=CARTESIAN_POINT('Ctrl Pts',(53.3440196850044,30.1121850623111,11.7780082085665));
#47109=CARTESIAN_POINT('Ctrl Pts',(53.2550712399639,29.9777015268172,11.7880615295092));
#47110=CARTESIAN_POINT('Ctrl Pts',(53.1877167505972,29.8463564868758,11.7964675023511));
#47111=CARTESIAN_POINT('Ctrl Pts',(53.0978000261856,29.6098134243791,11.8111852845085));
#47112=CARTESIAN_POINT('Ctrl Pts',(53.0681362896592,29.5080553194961,11.8173932560157));
#47113=CARTESIAN_POINT('Ctrl Pts',(53.0466869751866,29.4044697635106,11.8238528479472));
#47114=CARTESIAN_POINT('Origin',(55.,29.,3.45145488139523));
#47115=CARTESIAN_POINT('',(53.0466869981368,29.4044698743445,12.7818778464297));
#47116=CARTESIAN_POINT('',(53.0466869618782,29.40446969924,12.6249522205985));
#47117=CARTESIAN_POINT('',(53.0466869980082,29.4044698737233,3.45145488139523));
#47118=CARTESIAN_POINT('Ctrl Pts',(53.0466869981368,29.4044698743445,12.7818778464297));
#47119=CARTESIAN_POINT('Ctrl Pts',(53.0469807175671,29.4058883384094,12.7817808958998));
#47120=CARTESIAN_POINT('Ctrl Pts',(53.0472759905022,29.4073065231312,12.7816840045254));
#47121=CARTESIAN_POINT('Ctrl Pts',(53.0508269250449,29.4242689082659,12.7805256115402));
#47122=CARTESIAN_POINT('Ctrl Pts',(53.0542666696385,29.4397745153647,12.7794716157396));
#47123=CARTESIAN_POINT('Ctrl Pts',(53.059784672939,29.4633150901057,12.7778805836053));
#47124=CARTESIAN_POINT('Ctrl Pts',(53.0617284056302,29.4713805469485,12.7773371087376));
#47125=CARTESIAN_POINT('Ctrl Pts',(53.0654257556411,29.4863129439443,12.7763342637471));
#47126=CARTESIAN_POINT('Ctrl Pts',(53.0671657510172,29.4931830856705,12.7758741902327));
#47127=CARTESIAN_POINT('Ctrl Pts',(53.0700923085679,29.5044847953235,12.7751196865686));
#47128=CARTESIAN_POINT('Ctrl Pts',(53.0712575919899,29.5089217334113,12.7748240717453));
#47129=CARTESIAN_POINT('Ctrl Pts',(53.0735748342935,29.5176225947702,12.7742455933827));
#47130=CARTESIAN_POINT('Ctrl Pts',(53.0747256630267,29.5218867671066,12.7739626707361));
#47131=CARTESIAN_POINT('Ctrl Pts',(53.0776027074517,29.5324080602647,12.7732659549003));
#47132=CARTESIAN_POINT('Ctrl Pts',(53.0793453377625,29.538660713488,12.7728530959449));
#47133=CARTESIAN_POINT('Ctrl Pts',(53.0854797427908,29.5602630103817,12.7714304733238));
#47134=CARTESIAN_POINT('Ctrl Pts',(53.0900253867448,29.5755688233227,12.7704290973774));
#47135=CARTESIAN_POINT('Ctrl Pts',(53.1287771273081,29.7005336338774,12.7622950028036));
#47136=CARTESIAN_POINT('Ctrl Pts',(53.1722180030145,29.8071198302848,12.7556138070175));
#47137=CARTESIAN_POINT('Ctrl Pts',(53.2583711081099,29.9753174010266,12.7446364069224));
#47138=CARTESIAN_POINT('Ctrl Pts',(53.2957887879018,30.0393165683998,12.7403464341676));
#47139=CARTESIAN_POINT('Ctrl Pts',(53.3833185954148,30.171540967188,12.7309981990839));
#47140=CARTESIAN_POINT('Ctrl Pts',(53.434383462705,30.2389549345588,12.7259248507387));
#47141=CARTESIAN_POINT('Ctrl Pts',(53.5006892289883,30.3158209917544,12.7196246731006));
#47142=CARTESIAN_POINT('Ctrl Pts',(53.5119789453286,30.3285747940256,12.7185611613115));
#47143=CARTESIAN_POINT('Ctrl Pts',(53.5285580851662,30.3468275382929,12.717011682796));
#47144=CARTESIAN_POINT('Ctrl Pts',(53.533718112029,30.3524433995764,12.716531110956));
#47145=CARTESIAN_POINT('Ctrl Pts',(53.5442094291191,30.3637308989587,12.7155573053078));
#47146=CARTESIAN_POINT('Ctrl Pts',(53.5495419627123,30.3694011940714,12.7150640235623));
#47147=CARTESIAN_POINT('Ctrl Pts',(53.560660914068,30.3810866087176,12.7140388568684));
#47148=CARTESIAN_POINT('Ctrl Pts',(53.5664521615184,30.387096902307,12.7135067696218));
#47149=CARTESIAN_POINT('Ctrl Pts',(53.5814824381475,30.402501012635,12.7121304824753));
#47150=CARTESIAN_POINT('Ctrl Pts',(53.5907770110707,30.4118398342138,12.7112838749136));
#47151=CARTESIAN_POINT('Ctrl Pts',(53.6281408870226,30.448645022466,12.7078975961662));
#47152=CARTESIAN_POINT('Ctrl Pts',(53.6569245260463,30.4753703738079,12.705326399433));
#47153=CARTESIAN_POINT('Ctrl Pts',(53.7897970430816,30.5916293569452,12.693613143375));
#47154=CARTESIAN_POINT('Ctrl Pts',(53.902160051911,30.6711109754286,12.6840856601796));
#47155=CARTESIAN_POINT('Ctrl Pts',(54.1115938632293,30.7889620011166,12.6673376095533));
#47156=CARTESIAN_POINT('Ctrl Pts',(54.2052082189494,30.8324739062092,12.6601692430189));
#47157=CARTESIAN_POINT('Ctrl Pts',(54.3180257856908,30.8746305574751,12.6521776693993));
#47158=CARTESIAN_POINT('Ctrl Pts',(54.3343566065144,30.8804912861943,12.6510362977437));
#47159=CARTESIAN_POINT('Ctrl Pts',(54.3570447364804,30.8883008856725,12.6494738504019));
#47160=CARTESIAN_POINT('Ctrl Pts',(54.3633378864325,30.8904319775887,12.6490429180195));
#47161=CARTESIAN_POINT('Ctrl Pts',(54.3739038021108,30.8939512386906,12.6483236455304));
#47162=CARTESIAN_POINT('Ctrl Pts',(54.3781707756586,30.8953564731948,12.6480343277204));
#47163=CARTESIAN_POINT('Ctrl Pts',(54.3862653810412,30.8979919766568,12.6474877167445));
#47164=CARTESIAN_POINT('Ctrl Pts',(54.3900920346013,30.8992251052471,12.6472302534951));
#47165=CARTESIAN_POINT('Ctrl Pts',(54.4001229472724,30.9024240959168,12.6465577592845));
#47166=CARTESIAN_POINT('Ctrl Pts',(54.4063332068295,30.9043711982228,12.6461438104408));
#47167=CARTESIAN_POINT('Ctrl Pts',(54.4279100276121,30.9110203716658,12.6447135488102));
#47168=CARTESIAN_POINT('Ctrl Pts',(54.4433242650814,30.915567268953,12.6437057441309));
#47169=CARTESIAN_POINT('Ctrl Pts',(54.5631483565472,30.9493444376689,12.6359671451629));
#47170=CARTESIAN_POINT('Ctrl Pts',(54.6697433670408,30.9702080482977,12.6296372771496));
#47171=CARTESIAN_POINT('Ctrl Pts',(54.8892131666344,30.9948400571664,12.6168002770721));
#47172=CARTESIAN_POINT('Ctrl Pts',(55.0017613389849,30.9979128181507,12.6103129097961));
#47173=CARTESIAN_POINT('Ctrl Pts',(55.1520442615367,30.9893126425146,12.6012908456711));
#47174=CARTESIAN_POINT('Ctrl Pts',(55.1900500859954,30.9860420315021,12.5989796643989));
#47175=CARTESIAN_POINT('Ctrl Pts',(55.2547043451046,30.9786053721479,12.5949814732795));
#47176=CARTESIAN_POINT('Ctrl Pts',(55.2814053186271,30.9749846737277,12.5933108433031));
#47177=CARTESIAN_POINT('Ctrl Pts',(55.3189152194206,30.969122181462,12.5909329380871));
#47178=CARTESIAN_POINT('Ctrl Pts',(55.3297921431914,30.9673297174679,12.5902397214954));
#47179=CARTESIAN_POINT('Ctrl Pts',(55.348437426219,30.9640980964444,12.5890448382132));
#47180=CARTESIAN_POINT('Ctrl Pts',(55.3562131967178,30.9627027609968,12.5885445604634));
#47181=CARTESIAN_POINT('Ctrl Pts',(55.3710329026332,30.959952448083,12.5875872479403));
#47182=CARTESIAN_POINT('Ctrl Pts',(55.378078233747,30.9586055908613,12.5871304769543));
#47183=CARTESIAN_POINT('Ctrl Pts',(55.396289149536,30.9550222872038,12.5859454255917));
#47184=CARTESIAN_POINT('Ctrl Pts',(55.4074430001156,30.9527282008281,12.5852153311277));
#47185=CARTESIAN_POINT('Ctrl Pts',(55.4392753333226,30.9458964319583,12.583119171732));
#47186=CARTESIAN_POINT('Ctrl Pts',(55.4599015373,30.9411249989401,12.5817457573221));
#47187=CARTESIAN_POINT('Ctrl Pts',(55.6375786384987,30.8970323775887,12.5697795394161));
#47188=CARTESIAN_POINT('Ctrl Pts',(55.7893503483131,30.8390607756676,12.5585644909368));
#47189=CARTESIAN_POINT('Ctrl Pts',(56.0272010954461,30.7132953853573,12.5398157953161));
#47190=CARTESIAN_POINT('Ctrl Pts',(56.1178000634325,30.6556120318695,12.5323675653387));
#47191=CARTESIAN_POINT('Ctrl Pts',(56.2135251244105,30.5832080491782,12.5244576851107));
#47192=CARTESIAN_POINT('Ctrl Pts',(56.2236458039212,30.5753989721196,12.5236209921141));
#47193=CARTESIAN_POINT('Ctrl Pts',(56.2382230593088,30.5639259829635,12.5224161085554));
#47194=CARTESIAN_POINT('Ctrl Pts',(56.2427396715284,30.5603393655242,12.5220428221697));
#47195=CARTESIAN_POINT('Ctrl Pts',(56.250625287318,30.5540214804236,12.5213912512246));
#47196=CARTESIAN_POINT('Ctrl Pts',(56.2540010231757,30.5512987482055,12.5211123749626));
#47197=CARTESIAN_POINT('Ctrl Pts',(56.2611556148693,30.5454895283538,12.5205214600203));
#47198=CARTESIAN_POINT('Ctrl Pts',(56.2649320364964,30.5424001787604,12.5202096300353));
#47199=CARTESIAN_POINT('Ctrl Pts',(56.2751824261471,30.5339517505051,12.519363308362));
#47200=CARTESIAN_POINT('Ctrl Pts',(56.2816340094107,30.5285654924379,12.5188307246091));
#47201=CARTESIAN_POINT('Ctrl Pts',(56.3117415347404,30.5031048775729,12.5163446995061));
#47202=CARTESIAN_POINT('Ctrl Pts',(56.3349625019758,30.4825199803991,12.514425476324));
#47203=CARTESIAN_POINT('Ctrl Pts',(56.508349319307,30.3214371952223,12.4999955531089));
#47204=CARTESIAN_POINT('Ctrl Pts',(56.6364681248181,30.1590111191995,12.4886248397088));
#47205=CARTESIAN_POINT('Ctrl Pts',(56.7644602352575,29.9320509535065,12.4729768284465));
#47206=CARTESIAN_POINT('Ctrl Pts',(56.7894299815248,29.8831638721457,12.4696278131885));
#47207=CARTESIAN_POINT('Ctrl Pts',(56.8183040055526,29.8203664709771,12.4653203855262));
#47208=CARTESIAN_POINT('Ctrl Pts',(56.8241176511922,29.8073570346285,12.464427809293));
#47209=CARTESIAN_POINT('Ctrl Pts',(56.8332086375814,29.7864142087479,12.4629900553531));
#47210=CARTESIAN_POINT('Ctrl Pts',(56.8365750857559,29.7785198567145,12.4624479024795));
#47211=CARTESIAN_POINT('Ctrl Pts',(56.8428714222693,29.7634867560393,12.4614150068315));
#47212=CARTESIAN_POINT('Ctrl Pts',(56.8458110418532,29.7563522332293,12.4609246029548));
#47213=CARTESIAN_POINT('Ctrl Pts',(56.8524096261533,29.7400697341147,12.459804845473));
#47214=CARTESIAN_POINT('Ctrl Pts',(56.8560423360711,29.7309114005182,12.459174626859));
#47215=CARTESIAN_POINT('Ctrl Pts',(56.8653066195212,29.7070409698004,12.4575308149755));
#47216=CARTESIAN_POINT('Ctrl Pts',(56.8708319382767,29.6922886342081,12.4565137300095));
#47217=CARTESIAN_POINT('Ctrl Pts',(56.9208045725075,29.5538952469641,12.4469593702906));
#47218=CARTESIAN_POINT('Ctrl Pts',(56.9531007330669,29.426234631655,12.4380171297419));
#47219=CARTESIAN_POINT('Ctrl Pts',(56.9867412635985,29.2023107019161,12.4222896991071));
#47220=CARTESIAN_POINT('Ctrl Pts',(56.9941264447753,29.1073812093336,12.4156190822399));
#47221=CARTESIAN_POINT('Ctrl Pts',(56.9950631103932,28.9553076072849,12.4051829705105));
#47222=CARTESIAN_POINT('Ctrl Pts',(56.9929725583891,28.8983343042015,12.4013311509275));
#47223=CARTESIAN_POINT('Ctrl Pts',(56.9876847042695,28.8319862647204,12.3969690147217));
#47224=CARTESIAN_POINT('Ctrl Pts',(56.9868559761586,28.822454407065,12.396345335888));
#47225=CARTESIAN_POINT('Ctrl Pts',(56.9854774396395,28.8078197948792,12.3953927740173));
#47226=CARTESIAN_POINT('Ctrl Pts',(56.9849764817205,28.8027127398921,12.3950612934741));
#47227=CARTESIAN_POINT('Ctrl Pts',(56.984019347162,28.7933280431443,12.3944539578454));
#47228=CARTESIAN_POINT('Ctrl Pts',(56.9835690428404,28.7890499570381,12.3941777915038));
#47229=CARTESIAN_POINT('Ctrl Pts',(56.9825231289395,28.7794128800063,12.3935572233162));
#47230=CARTESIAN_POINT('Ctrl Pts',(56.9819196297804,28.7740548362671,12.3932132642148));
#47231=CARTESIAN_POINT('Ctrl Pts',(56.9803117541251,28.7602819679727,12.3923317068439));
#47232=CARTESIAN_POINT('Ctrl Pts',(56.9792754541041,28.7518708780475,12.3917958292416));
#47233=CARTESIAN_POINT('Ctrl Pts',(56.972525621047,28.6998214539949,12.3884937290925));
#47234=CARTESIAN_POINT('Ctrl Pts',(56.9654223242158,28.6563719727547,12.3857982192397));
#47235=CARTESIAN_POINT('Ctrl Pts',(56.9521007887792,28.5889778749672,12.3816634594334));
#47236=CARTESIAN_POINT('Ctrl Pts',(56.9468658581084,28.5648562515874,12.3801929312834));
#47237=CARTESIAN_POINT('Ctrl Pts',(56.9313726420217,28.4993561800107,12.37621084027));
#47238=CARTESIAN_POINT('Ctrl Pts',(56.9202334216269,28.4581989903333,12.3737206098934));
#47239=CARTESIAN_POINT('Ctrl Pts',(56.8833808671552,28.3375154408049,12.3663770209431));
#47240=CARTESIAN_POINT('Ctrl Pts',(56.8539810328816,28.2592144146441,12.3615546783459));
#47241=CARTESIAN_POINT('Ctrl Pts',(56.7858590401036,28.1074836800017,12.3517677098077));
#47242=CARTESIAN_POINT('Ctrl Pts',(56.7472965761595,28.034168608491,12.3468141078856));
#47243=CARTESIAN_POINT('Ctrl Pts',(56.6932543802115,27.9453111121851,12.3403874789645));
#47244=CARTESIAN_POINT('Ctrl Pts',(56.681924158206,27.9273350389749,12.3390646514332));
#47245=CARTESIAN_POINT('Ctrl Pts',(56.6648269473191,27.9011463368598,12.337102026232));
#47246=CARTESIAN_POINT('Ctrl Pts',(56.6592814534784,27.8927903586988,12.3364703986549));
#47247=CARTESIAN_POINT('Ctrl Pts',(56.6493458815801,27.8780616755569,12.3353472379894));
#47248=CARTESIAN_POINT('Ctrl Pts',(56.6449812567447,27.8716719877798,12.3348566644428));
#47249=CARTESIAN_POINT('Ctrl Pts',(56.6357506204271,27.8583259936068,12.3338249461486));
#47250=CARTESIAN_POINT('Ctrl Pts',(56.6308771687532,27.8513750455905,12.3332835264904));
#47251=CARTESIAN_POINT('Ctrl Pts',(56.6179498966411,27.833185160458,12.3318558106746));
#47252=CARTESIAN_POINT('Ctrl Pts',(56.609823443596,27.8219986407486,12.3309667549569));
#47253=CARTESIAN_POINT('Ctrl Pts',(56.5749104778022,27.7749749638184,12.3271817531637));
#47254=CARTESIAN_POINT('Ctrl Pts',(56.5470403225838,27.7399622759849,12.3242441343239));
#47255=CARTESIAN_POINT('Ctrl Pts',(56.3939753250386,27.5604098677388,12.3085229482105));
#47256=CARTESIAN_POINT('Ctrl Pts',(56.2496602941024,27.4335029933563,12.2949413010943));
#47257=CARTESIAN_POINT('Ctrl Pts',(56.0439061910508,27.2993364814037,12.2781087408986));
#47258=CARTESIAN_POINT('Ctrl Pts',(55.9970590764081,27.2714541074201,12.2744306170181));
#47259=CARTESIAN_POINT('Ctrl Pts',(55.9407979191054,27.2410183450529,12.2702391888441));
#47260=CARTESIAN_POINT('Ctrl Pts',(55.9324390631535,27.2365730553797,12.2696221471703));
#47261=CARTESIAN_POINT('Ctrl Pts',(55.9195199596595,27.2298201449515,12.2686775641504));
#47262=CARTESIAN_POINT('Ctrl Pts',(55.9149820975493,27.2274703280323,12.2683474911085));
#47263=CARTESIAN_POINT('Ctrl Pts',(55.9066064345219,27.2231739387031,12.267741485731));
#47264=CARTESIAN_POINT('Ctrl Pts',(55.902771380429,27.2212223538216,12.2674652519518));
#47265=CARTESIAN_POINT('Ctrl Pts',(55.8940933592255,27.2168415715172,12.2668429706206));
#47266=CARTESIAN_POINT('Ctrl Pts',(55.889246799769,27.2144196890535,12.2664973770948));
#47267=CARTESIAN_POINT('Ctrl Pts',(55.8748848028341,27.2073158096509,12.2654788221483));
#47268=CARTESIAN_POINT('Ctrl Pts',(55.8653416528803,27.2026898264538,12.2648092030439));
#47269=CARTESIAN_POINT('Ctrl Pts',(55.7783528166889,27.1613760024374,12.2587663115671));
#47270=CARTESIAN_POINT('Ctrl Pts',(55.6986447001155,27.1296335501159,12.2536637070502));
#47271=CARTESIAN_POINT('Ctrl Pts',(55.5331329645086,27.0757859887222,12.2434632996674));
#47272=CARTESIAN_POINT('Ctrl Pts',(55.4474104211088,27.054067156049,12.2383800131883));
#47273=CARTESIAN_POINT('Ctrl Pts',(55.2891787274565,27.0249895912462,12.2289766640238));
#47274=CARTESIAN_POINT('Ctrl Pts',(55.2171702024508,27.0157806819274,12.2246904993772));
#47275=CARTESIAN_POINT('Ctrl Pts',(55.1020526795171,27.0074007087402,12.2176971814632));
#47276=CARTESIAN_POINT('Ctrl Pts',(55.0591942192437,27.0056674499854,12.2150632937176));
#47277=CARTESIAN_POINT('Ctrl Pts',(55.0031933620288,27.0052093931292,12.2115675280871));
#47278=CARTESIAN_POINT('Ctrl Pts',(54.9900708043404,27.0052315520567,12.2107445187354));
#47279=CARTESIAN_POINT('Ctrl Pts',(54.9686154417186,27.005479496088,12.209392202544));
#47280=CARTESIAN_POINT('Ctrl Pts',(54.9602820096874,27.0056280414954,12.2088653004958));
#47281=CARTESIAN_POINT('Ctrl Pts',(54.9441637224632,27.0060164164032,12.2078428821351));
#47282=CARTESIAN_POINT('Ctrl Pts',(54.9363788480573,27.0062496225048,12.2073475809117));
#47283=CARTESIAN_POINT('Ctrl Pts',(54.9184037419414,27.0068934747523,12.2062004111372));
#47284=CARTESIAN_POINT('Ctrl Pts',(54.9082149646363,27.0073366889396,12.2055475422439));
#47285=CARTESIAN_POINT('Ctrl Pts',(54.8752929394498,27.0090218362612,12.2034292715091));
#47286=CARTESIAN_POINT('Ctrl Pts',(54.8525780991494,27.0105748036605,12.2019542813809));
#47287=CARTESIAN_POINT('Ctrl Pts',(54.6612150089133,27.0269531557886,12.1894095930878));
#47288=CARTESIAN_POINT('Ctrl Pts',(54.4950886623826,27.0628032986198,12.1776532116537));
#47289=CARTESIAN_POINT('Ctrl Pts',(54.2666424042816,27.1435111129261,12.1607783175178));
#47290=CARTESIAN_POINT('Ctrl Pts',(54.1991456005843,27.1716132918691,12.1557104095432));
#47291=CARTESIAN_POINT('Ctrl Pts',(54.1122935776851,27.2135087903003,12.1491932020922));
#47292=CARTESIAN_POINT('Ctrl Pts',(54.0914271279094,27.2240301324643,12.147627948555));
#47293=CARTESIAN_POINT('Ctrl Pts',(54.0566478650104,27.2423401120278,12.1450255987048));
#47294=CARTESIAN_POINT('Ctrl Pts',(54.0426352136535,27.2499330765607,12.1439789364462));
#47295=CARTESIAN_POINT('Ctrl Pts',(54.0232101475868,27.2607619883571,12.1425321261216));
#47296=CARTESIAN_POINT('Ctrl Pts',(54.0177202268807,27.2638566514157,12.1421236938401));
#47297=CARTESIAN_POINT('Ctrl Pts',(54.0084012250866,27.269168117333,12.1414313050845));
#47298=CARTESIAN_POINT('Ctrl Pts',(54.0045647103038,27.2713717224522,12.1411465237209));
#47299=CARTESIAN_POINT('Ctrl Pts',(53.9971963651563,27.2756365945551,12.1406001338026));
#47300=CARTESIAN_POINT('Ctrl Pts',(53.9936635181788,27.2776959704575,12.1403384031488));
#47301=CARTESIAN_POINT('Ctrl Pts',(53.9851937603913,27.2826681406235,12.1397114446968));
#47302=CARTESIAN_POINT('Ctrl Pts',(53.9802629891993,27.2855913993721,12.1393468817709));
#47303=CARTESIAN_POINT('Ctrl Pts',(53.9623353057765,27.2963247205819,12.1380226829196));
#47304=CARTESIAN_POINT('Ctrl Pts',(53.9494145678477,27.3042618841627,12.1370708298266));
#47305=CARTESIAN_POINT('Ctrl Pts',(53.8233671803382,27.3836861356027,12.1277971116481));
#47306=CARTESIAN_POINT('Ctrl Pts',(53.7175985178434,27.466249022772,12.1200962504797));
#47307=CARTESIAN_POINT('Ctrl Pts',(53.6158559968772,27.5636081977957,12.111916902352));
#47308=CARTESIAN_POINT('Ctrl Pts',(53.610851254808,27.5684477675121,12.1115124383648));
#47309=CARTESIAN_POINT('Ctrl Pts',(53.5115931108928,27.6654407336976,12.1034463747051));
#47310=CARTESIAN_POINT('Ctrl Pts',(53.4266910328677,27.7666727975071,12.0957150572584));
#47311=CARTESIAN_POINT('Ctrl Pts',(53.3418616630034,27.8909670392705,12.086389355817));
#47312=CARTESIAN_POINT('Ctrl Pts',(53.3315439851451,27.9065507134296,12.0852234561522));
#47313=CARTESIAN_POINT('Ctrl Pts',(53.3162995543261,27.9302938980027,12.0834509320837));
#47314=CARTESIAN_POINT('Ctrl Pts',(53.3112096252535,27.9383477968127,12.0828503326364));
#47315=CARTESIAN_POINT('Ctrl Pts',(53.3021185782943,27.9529635618515,12.0817614257736));
#47316=CARTESIAN_POINT('Ctrl Pts',(53.2980972926105,27.9595127118127,12.0812738681964));
#47317=CARTESIAN_POINT('Ctrl Pts',(53.2895590352827,27.9736002255042,12.0802258131476));
#47318=CARTESIAN_POINT('Ctrl Pts',(53.2850538469439,27.9811455064953,12.0796649014469));
#47319=CARTESIAN_POINT('Ctrl Pts',(53.2730945654491,28.0014789534306,12.0781543297065));
#47320=CARTESIAN_POINT('Ctrl Pts',(53.2657328271436,28.0143205318152,12.0772013830375));
#47321=CARTESIAN_POINT('Ctrl Pts',(53.2311111292295,28.0763022459907,12.0726059440563));
#47322=CARTESIAN_POINT('Ctrl Pts',(53.2057952194443,28.1264935291507,12.0688958513932));
#47323=CARTESIAN_POINT('Ctrl Pts',(53.1160457451258,28.324844784901,12.0542681238157));
#47324=CARTESIAN_POINT('Ctrl Pts',(53.0675850115898,28.4795406667179,12.0428693902826));
#47325=CARTESIAN_POINT('Ctrl Pts',(53.0267901116386,28.7008247081689,12.0273344514217));
#47326=CARTESIAN_POINT('Ctrl Pts',(53.0182625760941,28.7638189554259,12.0230047605399));
#47327=CARTESIAN_POINT('Ctrl Pts',(53.0115515312456,28.8409612466387,12.0178929337683));
#47328=CARTESIAN_POINT('Ctrl Pts',(53.0104918948063,28.8548167946697,12.0169822758678));
#47329=CARTESIAN_POINT('Ctrl Pts',(53.009184388195,28.8746351419822,12.0156914535194));
#47330=CARTESIAN_POINT('Ctrl Pts',(53.0088183780508,28.8805893704338,12.0153051515565));
#47331=CARTESIAN_POINT('Ctrl Pts',(53.0082307806828,28.8909037237693,12.0146386937589));
#47332=CARTESIAN_POINT('Ctrl Pts',(53.007996787886,28.8952630679949,12.0143578603055));
#47333=CARTESIAN_POINT('Ctrl Pts',(53.0075666182819,28.9038008397764,12.0138095334786));
#47334=CARTESIAN_POINT('Ctrl Pts',(53.007369272093,28.9079791219841,12.0135419721796));
#47335=CARTESIAN_POINT('Ctrl Pts',(53.0068614750438,28.9194991921929,12.0128063536769));
#47336=CARTESIAN_POINT('Ctrl Pts',(53.006578443521,28.9268422123311,12.0123397937604));
#47337=CARTESIAN_POINT('Ctrl Pts',(53.0056202914725,28.9558672745944,12.0105042251296));
#47338=CARTESIAN_POINT('Ctrl Pts',(53.0052582589013,28.9775590614289,12.0091514244171));
#47339=CARTESIAN_POINT('Ctrl Pts',(53.0051991626429,29.1354634294638,11.999414201243));
#47340=CARTESIAN_POINT('Ctrl Pts',(53.0190996273219,29.2712417536779,11.9916209411359));
#47341=CARTESIAN_POINT('Ctrl Pts',(53.0466870113634,29.4044699382199,11.9837090255998));
#47342=CARTESIAN_POINT('Ctrl Pts',(53.0466869751866,29.4044697635106,11.8238528479472));
#47343=CARTESIAN_POINT('Ctrl Pts',(53.0419512156118,29.3815992755424,11.8252790508395));
#47344=CARTESIAN_POINT('Ctrl Pts',(53.037615893422,29.3586396669258,11.8267169431701));
#47345=CARTESIAN_POINT('Ctrl Pts',(53.0307704408819,29.3185315798298,11.8292425819739));
#47346=CARTESIAN_POINT('Ctrl Pts',(53.0280795442047,29.30142513244,11.830324114331));
#47347=CARTESIAN_POINT('Ctrl Pts',(53.0242942861441,29.2751362439084,11.8319937253997));
#47348=CARTESIAN_POINT('Ctrl Pts',(53.0230404475711,29.2659773372315,11.8325768036252));
#47349=CARTESIAN_POINT('Ctrl Pts',(53.0209591771938,29.2499457901447,11.8335999813272));
#47350=CARTESIAN_POINT('Ctrl Pts',(53.0201037655562,29.2430768915739,11.8340391966616));
#47351=CARTESIAN_POINT('Ctrl Pts',(53.0182496217826,29.2275287387491,11.8350353117973));
#47352=CARTESIAN_POINT('Ctrl Pts',(53.0172721282171,29.2188471407096,11.8355928665027));
#47353=CARTESIAN_POINT('Ctrl Pts',(53.0147764264254,29.1952907738518,11.8371095265229));
#47354=CARTESIAN_POINT('Ctrl Pts',(53.0133684061827,29.1804051379565,11.8380720434669));
#47355=CARTESIAN_POINT('Ctrl Pts',(53.0075080436848,29.1100167962154,11.8426437734471));
#47356=CARTESIAN_POINT('Ctrl Pts',(53.0052139371755,29.0543640789963,11.8463191563776));
#47357=CARTESIAN_POINT('Ctrl Pts',(53.0053217315665,28.8899112222531,11.8573648722136));
#47358=CARTESIAN_POINT('Ctrl Pts',(53.0142912576156,28.781329208358,11.8649080511666));
#47359=CARTESIAN_POINT('Ctrl Pts',(53.0505905309261,28.5621830167179,11.8803896986878));
#47360=CARTESIAN_POINT('Ctrl Pts',(53.0786206905866,28.4521064091951,11.8883022770975));
#47361=CARTESIAN_POINT('Ctrl Pts',(53.1211067553984,28.3298928969766,11.8968733832638));
#47362=CARTESIAN_POINT('Ctrl Pts',(53.1265401053883,28.3148493479945,11.8979243464688));
#47363=CARTESIAN_POINT('Ctrl Pts',(53.1344338257212,28.2937899722925,11.8993882463013));
#47364=CARTESIAN_POINT('Ctrl Pts',(53.1367433787841,28.2877187913659,11.8998094073322));
#47365=CARTESIAN_POINT('Ctrl Pts',(53.1405295564135,28.2779104094156,11.9004882930398));
#47366=CARTESIAN_POINT('Ctrl Pts',(53.1419878661865,28.2741662596018,11.9007470821577));
#47367=CARTESIAN_POINT('Ctrl Pts',(53.1451016006014,28.2662427531927,11.9012939350696));
#47368=CARTESIAN_POINT('Ctrl Pts',(53.1467598594749,28.2620645342128,11.9015818228112));
#47369=CARTESIAN_POINT('Ctrl Pts',(53.1509091233061,28.2517120757535,11.9022940238727));
#47370=CARTESIAN_POINT('Ctrl Pts',(53.1534169676304,28.2455445702882,11.9027173421247));
#47371=CARTESIAN_POINT('Ctrl Pts',(53.1629450897412,28.2224443337686,11.9042996105202));
#47372=CARTESIAN_POINT('Ctrl Pts',(53.1701680246017,28.2055954712677,11.9054470909592));
#47373=CARTESIAN_POINT('Ctrl Pts',(53.1890811128194,28.1631043211552,11.9083299580833));
#47374=CARTESIAN_POINT('Ctrl Pts',(53.2010845336275,28.1376051376242,11.9100497229659));
#47375=CARTESIAN_POINT('Ctrl Pts',(53.303190217923,27.9321157218,11.9238918679677));
#47376=CARTESIAN_POINT('Ctrl Pts',(53.4195222732825,27.7664501705442,11.9350644621512));
#47377=CARTESIAN_POINT('Ctrl Pts',(53.591511541332,27.5866913990487,11.9500752093234));
#47378=CARTESIAN_POINT('Ctrl Pts',(53.6255399602801,27.5535768267661,11.9529813306361));
#47379=CARTESIAN_POINT('Ctrl Pts',(53.6711831189628,27.5122255619556,11.9568202564802));
#47380=CARTESIAN_POINT('Ctrl Pts',(53.6817513418575,27.5028535338857,11.9577051740104));
#47381=CARTESIAN_POINT('Ctrl Pts',(53.6988785196684,27.4879868909286,11.9591335130573));
#47382=CARTESIAN_POINT('Ctrl Pts',(53.7053749676326,27.4824207531465,11.9596739807484));
#47383=CARTESIAN_POINT('Ctrl Pts',(53.7178032855557,27.4719100875166,11.9607055790849));
#47384=CARTESIAN_POINT('Ctrl Pts',(53.7237284702546,27.4669578692044,11.9611963838534));
#47385=CARTESIAN_POINT('Ctrl Pts',(53.7373167027513,27.4557343156967,11.9623197442445));
#47386=CARTESIAN_POINT('Ctrl Pts',(53.7449979445959,27.4494854247736,11.9629531855563));
#47387=CARTESIAN_POINT('Ctrl Pts',(53.7687893592911,27.4304231024851,11.9649105506074));
#47388=CARTESIAN_POINT('Ctrl Pts',(53.7850511834993,27.4178019719537,11.9662420142328));
#47389=CARTESIAN_POINT('Ctrl Pts',(53.8637276223799,27.3586677674977,11.9726555461709));
#47390=CARTESIAN_POINT('Ctrl Pts',(53.9286267770662,27.3155881631054,11.9778663714132));
#47391=CARTESIAN_POINT('Ctrl Pts',(54.0713039527384,27.2324670177253,11.9891448209487));
#47392=CARTESIAN_POINT('Ctrl Pts',(54.1495377513363,27.1935223697184,11.9952286001361));
#47393=CARTESIAN_POINT('Ctrl Pts',(54.325178939865,27.1200333978468,12.0084967750014));
#47394=CARTESIAN_POINT('Ctrl Pts',(54.4232447037284,27.0876675370054,12.0156629276098));
#47395=CARTESIAN_POINT('Ctrl Pts',(54.5389890551211,27.05918707542,12.0235598166266));
#47396=CARTESIAN_POINT('Ctrl Pts',(54.5546428189481,27.0555353127704,12.0246160802028));
#47397=CARTESIAN_POINT('Ctrl Pts',(54.5766955352554,27.0506710754432,12.0260860621106));
#47398=CARTESIAN_POINT('Ctrl Pts',(54.5830584099579,27.0493002180431,12.0265080937872));
#47399=CARTESIAN_POINT('Ctrl Pts',(54.5933623770618,27.0471329870347,12.027188004103));
#47400=CARTESIAN_POINT('Ctrl Pts',(54.5972993029406,27.0463173553511,12.0274469532736));
#47401=CARTESIAN_POINT('Ctrl Pts',(54.6056402678626,27.044615601903,12.0279937803656));
#47402=CARTESIAN_POINT('Ctrl Pts',(54.6100448875586,27.0437324432224,12.0282814839686));
#47403=CARTESIAN_POINT('Ctrl Pts',(54.6209706816359,27.0415801078761,12.028992600216));
#47404=CARTESIAN_POINT('Ctrl Pts',(54.6274953522048,27.040328601931,12.0294150244595));
#47405=CARTESIAN_POINT('Ctrl Pts',(54.6519458204627,27.0357652517017,12.0309900444762));
#47406=CARTESIAN_POINT('Ctrl Pts',(54.669911126967,27.032666462086,12.0321313059987));
#47407=CARTESIAN_POINT('Ctrl Pts',(54.7155410940459,27.0254385489766,12.0349952878808));
#47408=CARTESIAN_POINT('Ctrl Pts',(54.7432554469232,27.0216440702078,12.0367026451986));
#47409=CARTESIAN_POINT('Ctrl Pts',(54.8705082851564,27.0069407617222,12.0444324790711));
#47410=CARTESIAN_POINT('Ctrl Pts',(54.9707066919013,27.002952628509,12.0502184319241));
#47411=CARTESIAN_POINT('Ctrl Pts',(55.2020989685393,27.0111691653767,12.0636654421015));
#47412=CARTESIAN_POINT('Ctrl Pts',(55.3326122572786,27.0287933533485,12.071330909542));
#47413=CARTESIAN_POINT('Ctrl Pts',(55.4841150389246,27.0647345553516,12.0809165538984));
#47414=CARTESIAN_POINT('Ctrl Pts',(55.5076864227765,27.070784063731,12.0824272693655));
#47415=CARTESIAN_POINT('Ctrl Pts',(55.5405813134076,27.0798710103584,12.0845653123574));
#47416=CARTESIAN_POINT('Ctrl Pts',(55.5500026743539,27.0825484240716,12.085181116696));
#47417=CARTESIAN_POINT('Ctrl Pts',(55.5663382016336,27.0873210425458,12.086255025847));
#47418=CARTESIAN_POINT('Ctrl Pts',(55.573261467544,27.0893846434909,12.0867121043316));
#47419=CARTESIAN_POINT('Ctrl Pts',(55.587688354362,27.0937703035204,12.0876687001785));
#47420=CARTESIAN_POINT('Ctrl Pts',(55.5951897623571,27.0960991618526,12.088168431345));
#47421=CARTESIAN_POINT('Ctrl Pts',(55.6129472503702,27.1017272847668,12.0893570565879));
#47422=CARTESIAN_POINT('Ctrl Pts',(55.6231906580103,27.1050654287251,12.0900472074169));
#47423=CARTESIAN_POINT('Ctrl Pts',(55.6575150540122,27.1165595517097,12.0923752391267));
#47424=CARTESIAN_POINT('Ctrl Pts',(55.6814662270759,27.1250926285658,12.0940253832694));
#47425=CARTESIAN_POINT('Ctrl Pts',(55.7383164421377,27.1465798601157,12.0980056521678));
#47426=CARTESIAN_POINT('Ctrl Pts',(55.7710460736974,27.1599551409798,12.1003489849417));
#47427=CARTESIAN_POINT('Ctrl Pts',(55.8976860216487,27.2156799144859,12.1096214791105));
#47428=CARTESIAN_POINT('Ctrl Pts',(55.9886052921856,27.2644039644018,12.1167402977709));
#47429=CARTESIAN_POINT('Ctrl Pts',(56.1791081919703,27.3863368829186,12.1324957911777));
#47430=CARTESIAN_POINT('Ctrl Pts',(56.2765030712926,27.4622256391759,12.1411262917899));
#47431=CARTESIAN_POINT('Ctrl Pts',(56.3777562598497,27.5574108790346,12.1503290114144));
#47432=CARTESIAN_POINT('Ctrl Pts',(56.3891053221239,27.5683358898091,12.1513638446633));
#47433=CARTESIAN_POINT('Ctrl Pts',(56.4049214252137,27.5839261949023,12.1528092350562));
#47434=CARTESIAN_POINT('Ctrl Pts',(56.4094967138372,27.5884801634515,12.1532277484406));
#47435=CARTESIAN_POINT('Ctrl Pts',(56.4171601308041,27.5961822870067,12.1539292738617));
#47436=CARTESIAN_POINT('Ctrl Pts',(56.4202600458961,27.5993185904848,12.1542131948735));
#47437=CARTESIAN_POINT('Ctrl Pts',(56.4265703415529,27.6057454477852,12.1547914102444));
#47438=CARTESIAN_POINT('Ctrl Pts',(56.4297797855824,27.6090368583078,12.1550856333739));
#47439=CARTESIAN_POINT('Ctrl Pts',(56.4379389268974,27.6174624550732,12.1558340682869));
#47440=CARTESIAN_POINT('Ctrl Pts',(56.4428725726163,27.6226121956811,12.1562870579342));
#47441=CARTESIAN_POINT('Ctrl Pts',(56.462891721976,27.6437337888924,12.1581274586418));
#47442=CARTESIAN_POINT('Ctrl Pts',(56.4777411421276,27.6599285704001,12.159498010232));
#47443=CARTESIAN_POINT('Ctrl Pts',(56.5163113070324,27.7034142026811,12.1630830153467));
#47444=CARTESIAN_POINT('Ctrl Pts',(56.5395635825951,27.7311111189526,12.1652704749985));
#47445=CARTESIAN_POINT('Ctrl Pts',(56.6755312922512,27.9023130084241,12.1783302321244));
#47446=CARTESIAN_POINT('Ctrl Pts',(56.7688718930371,28.0600947716442,12.1885476842108));
#47447=CARTESIAN_POINT('Ctrl Pts',(56.8598050429194,28.2768692697035,12.2026782303178));
#47448=CARTESIAN_POINT('Ctrl Pts',(56.8782197384901,28.3261433816623,12.2058888243322));
#47449=CARTESIAN_POINT('Ctrl Pts',(56.8992433578435,28.3899865112696,12.2100754965742));
#47450=CARTESIAN_POINT('Ctrl Pts',(56.9036680884007,28.4039382749811,12.2109919623107));
#47451=CARTESIAN_POINT('Ctrl Pts',(56.9104678913919,28.426227291768,12.2124590853075));
#47452=CARTESIAN_POINT('Ctrl Pts',(56.9129428983815,28.4345336893609,12.2130064917863));
#47453=CARTESIAN_POINT('Ctrl Pts',(56.9172994802477,28.4495108520588,12.2139948045407));
#47454=CARTESIAN_POINT('Ctrl Pts',(56.9192005806321,28.4561758296227,12.2144350706508));
#47455=CARTESIAN_POINT('Ctrl Pts',(56.9235815537708,28.471843986474,12.2154711951535));
#47456=CARTESIAN_POINT('Ctrl Pts',(56.9260329978837,28.4808548807646,12.2160679590589));
#47457=CARTESIAN_POINT('Ctrl Pts',(56.9329647357412,28.5070592552695,12.2178061159177));
#47458=CARTESIAN_POINT('Ctrl Pts',(56.9372786033813,28.5242954418574,12.2189528017679));
#47459=CARTESIAN_POINT('Ctrl Pts',(56.9741730293097,28.6805417574891,12.2293808984508));
#47460=CARTESIAN_POINT('Ctrl Pts',(56.99196488151,28.8225912117635,12.2391445851376));
#47461=CARTESIAN_POINT('Ctrl Pts',(56.9967301029314,29.0964381919624,12.2582071533406));
#47462=CARTESIAN_POINT('Ctrl Pts',(56.9860720076567,29.2274971143795,12.2674223188148));
#47463=CARTESIAN_POINT('Ctrl Pts',(56.9598826317511,29.3716483979431,12.277118753755));
#47464=CARTESIAN_POINT('Ctrl Pts',(56.9569691736887,29.3866964562119,12.2781252115103));
#47465=CARTESIAN_POINT('Ctrl Pts',(56.95272378902,29.4073456389041,12.2794969838196));
#47466=CARTESIAN_POINT('Ctrl Pts',(56.9515407254034,29.4129763489545,12.2798700889732));
#47467=CARTESIAN_POINT('Ctrl Pts',(56.949473969176,29.422605696224,12.2805064249537));
#47468=CARTESIAN_POINT('Ctrl Pts',(56.9486023039066,29.426606836467,12.2807703201062));
#47469=CARTESIAN_POINT('Ctrl Pts',(56.9467642156186,29.4349208961341,12.2813175678194));
#47470=CARTESIAN_POINT('Ctrl Pts',(56.945795773709,29.4392333144551,12.2816007941594));
#47471=CARTESIAN_POINT('Ctrl Pts',(56.9434170715261,29.4496632751095,12.2822843594));
#47472=CARTESIAN_POINT('Ctrl Pts',(56.9419922333662,29.4557775147664,12.2826838765769));
#47473=CARTESIAN_POINT('Ctrl Pts',(56.9368837210311,29.4772401396713,12.2840823888012));
#47474=CARTESIAN_POINT('Ctrl Pts',(56.9330466530229,29.4925518992694,12.2850730853336));
#47475=CARTESIAN_POINT('Ctrl Pts',(56.9081058231038,29.5872938172732,12.2911684978436));
#47476=CARTESIAN_POINT('Ctrl Pts',(56.8822892840167,29.6654111490091,12.2960445877808));
#47477=CARTESIAN_POINT('Ctrl Pts',(56.8015962854423,29.8668632091009,12.3087435340589));
#47478=CARTESIAN_POINT('Ctrl Pts',(56.7389150577306,29.9865976090572,12.3164428204456));
#47479=CARTESIAN_POINT('Ctrl Pts',(56.6311141609693,30.1498677420976,12.3281376082845));
#47480=CARTESIAN_POINT('Ctrl Pts',(56.5952884820006,30.1990758151192,12.3318364687067));
#47481=CARTESIAN_POINT('Ctrl Pts',(56.547795852996,30.2584059508841,12.3365656426763));
#47482=CARTESIAN_POINT('Ctrl Pts',(56.5381843928376,30.2701363287175,12.3375144693885));
#47483=CARTESIAN_POINT('Ctrl Pts',(56.5227399730999,30.2885531559872,12.3390268337446));
#47484=CARTESIAN_POINT('Ctrl Pts',(56.5169944191003,30.2953123908205,12.3395868386569));
#47485=CARTESIAN_POINT('Ctrl Pts',(56.5061925278264,30.3078496014009,12.3406349531305));
#47486=CARTESIAN_POINT('Ctrl Pts',(56.5011475305854,30.3136371643264,12.341122592085));
#47487=CARTESIAN_POINT('Ctrl Pts',(56.4898413192851,30.3264573361728,12.3422113536783));
#47488=CARTESIAN_POINT('Ctrl Pts',(56.4835635006655,30.3334749925806,12.3428131593945));
#47489=CARTESIAN_POINT('Ctrl Pts',(56.4650446992758,30.3538835792914,12.3445806552348));
#47490=CARTESIAN_POINT('Ctrl Pts',(56.4526706912477,30.3671519828045,12.3457519162749));
#47491=CARTESIAN_POINT('Ctrl Pts',(56.4242266887403,30.3968297444831,12.3484232444066));
#47492=CARTESIAN_POINT('Ctrl Pts',(56.4080510403679,30.4131338195804,12.3499277312928));
#47493=CARTESIAN_POINT('Ctrl Pts',(56.353891399217,30.4658702123953,12.3549187738795));
#47494=CARTESIAN_POINT('Ctrl Pts',(56.3147493991992,30.501076493275,12.3584539259184));
#47495=CARTESIAN_POINT('Ctrl Pts',(56.1794946706626,30.6133793199982,12.3704263803881));
#47496=CARTESIAN_POINT('Ctrl Pts',(56.0776448662427,30.6831155136171,12.3790754108769));
#47497=CARTESIAN_POINT('Ctrl Pts',(55.898656786947,30.7827267944133,12.3932814793841));
#47498=CARTESIAN_POINT('Ctrl Pts',(55.8249058789421,30.8180297654826,12.3988794317685));
#47499=CARTESIAN_POINT('Ctrl Pts',(55.739385175626,30.8526869808828,12.4049397574574));
#47500=CARTESIAN_POINT('Ctrl Pts',(55.7295485465239,30.8565824562932,12.4056305384745));
#47501=CARTESIAN_POINT('Ctrl Pts',(55.7146332005614,30.8623523420861,12.4066680127006));
#47502=CARTESIAN_POINT('Ctrl Pts',(55.7095772648969,30.8642845716856,12.4070179715116));
#47503=CARTESIAN_POINT('Ctrl Pts',(55.7004879783124,30.8677158961167,12.4076439466111));
#47504=CARTESIAN_POINT('Ctrl Pts',(55.6964576013655,30.8692225354257,12.4079203999416));
#47505=CARTESIAN_POINT('Ctrl Pts',(55.6876258132563,30.8724915116391,12.4085237474727));
#47506=CARTESIAN_POINT('Ctrl Pts',(55.6828224951334,30.8742484258394,12.4088503215082));
#47507=CARTESIAN_POINT('Ctrl Pts',(55.6690897125291,30.8792116785985,12.409779679836));
#47508=CARTESIAN_POINT('Ctrl Pts',(55.6601439145152,30.8823728634177,12.4103798782418));
#47509=CARTESIAN_POINT('Ctrl Pts',(55.5992040329686,30.9034193749124,12.4144354161375));
#47510=CARTESIAN_POINT('Ctrl Pts',(55.5465071744757,30.9192138732791,12.4177794640655));
#47511=CARTESIAN_POINT('Ctrl Pts',(55.3009911366779,30.9818653087853,12.4329019155806));
#47512=CARTESIAN_POINT('Ctrl Pts',(55.1025220139745,31.0019699918356,12.4439664273347));
#47513=CARTESIAN_POINT('Ctrl Pts',(54.8658582572031,30.99060737848,12.4583638784567));
#47514=CARTESIAN_POINT('Ctrl Pts',(54.8274412590852,30.9876455727915,12.4607341798565));
#47515=CARTESIAN_POINT('Ctrl Pts',(54.7761289782824,30.9821908134408,12.4639554113397));
#47516=CARTESIAN_POINT('Ctrl Pts',(54.7631361902104,30.9806802311339,12.4647758093165));
#47517=CARTESIAN_POINT('Ctrl Pts',(54.7418994474283,30.9779992371245,12.4661249240122));
#47518=CARTESIAN_POINT('Ctrl Pts',(54.7336461694053,30.9769047804184,12.4666512581355));
#47519=CARTESIAN_POINT('Ctrl Pts',(54.7176821979909,30.9746860351847,12.4676733511091));
#47520=CARTESIAN_POINT('Ctrl Pts',(54.7099707539901,30.9735681676936,12.4681688997993));
#47521=CARTESIAN_POINT('Ctrl Pts',(54.6919822097886,30.9708528033732,12.4693292217248));
#47522=CARTESIAN_POINT('Ctrl Pts',(54.6817107357628,30.9692200662155,12.4699950907774));
#47523=CARTESIAN_POINT('Ctrl Pts',(54.6484996092183,30.9636742527576,12.4721590983502));
#47524=CARTESIAN_POINT('Ctrl Pts',(54.6256162328235,30.959440178979,12.4736672634306));
#47525=CARTESIAN_POINT('Ctrl Pts',(54.5058477989047,30.9351050527657,12.4816540133819));
#47526=CARTESIAN_POINT('Ctrl Pts',(54.4104971514521,30.9082188780357,12.4883446342128));
#47527=CARTESIAN_POINT('Ctrl Pts',(54.2188552461025,30.8384426630757,12.5024181705178));
#47528=CARTESIAN_POINT('Ctrl Pts',(54.1231601719404,30.7947728583041,12.5097970797009));
#47529=CARTESIAN_POINT('Ctrl Pts',(53.9711076309196,30.7103090387457,12.521806593635));
#47530=CARTESIAN_POINT('Ctrl Pts',(53.9126331261713,30.6737418787728,12.5264988281467));
#47531=CARTESIAN_POINT('Ctrl Pts',(53.8476891926842,30.6282857120999,12.5317028428716));
#47532=CARTESIAN_POINT('Ctrl Pts',(53.8392609786101,30.6222883504641,12.5323780232504));
#47533=CARTESIAN_POINT('Ctrl Pts',(53.8265351566805,30.613082940841,12.5333967410772));
#47534=CARTESIAN_POINT('Ctrl Pts',(53.8222033548238,30.6099227859656,12.5337433750676));
#47535=CARTESIAN_POINT('Ctrl Pts',(53.8145248190347,30.6042735280494,12.5343575044096));
#47536=CARTESIAN_POINT('Ctrl Pts',(53.811173117761,30.6017913729685,12.5346254616606));
#47537=CARTESIAN_POINT('Ctrl Pts',(53.8078084765724,30.5992832565342,12.5348943391444));
#47538=CARTESIAN_POINT('Ctrl Pts',(53.8077878272654,30.5992678632258,12.5348959892817));
#47539=CARTESIAN_POINT('Ctrl Pts',(53.807746700905,30.5992372037786,12.534899275783));
#47540=CARTESIAN_POINT('Ctrl Pts',(53.8077262236916,30.5992219375308,12.5349009121598));
#47541=CARTESIAN_POINT('Ctrl Pts',(53.8076854378746,30.599191529519,12.5349041714315));
#47542=CARTESIAN_POINT('Ctrl Pts',(53.8076651294104,30.599176387869,12.5349057943153));
#47543=CARTESIAN_POINT('Ctrl Pts',(53.8076246787578,30.5991462273426,12.5349090267877));
#47544=CARTESIAN_POINT('Ctrl Pts',(53.8076045363477,30.5991312083105,12.5349106363941));
#47545=CARTESIAN_POINT('Ctrl Pts',(53.8075644135963,30.5991012899123,12.534913842648));
#47546=CARTESIAN_POINT('Ctrl Pts',(53.8075444337523,30.5990863909264,12.5349154392559));
#47547=CARTESIAN_POINT('Ctrl Pts',(53.8075046343914,30.59905671135,12.5349186196521));
#47548=CARTESIAN_POINT('Ctrl Pts',(53.8074848145996,30.5990419305637,12.5349202034626));
#47549=CARTESIAN_POINT('Ctrl Pts',(53.8074453315781,30.5990124846063,12.534923358565));
#47550=CARTESIAN_POINT('Ctrl Pts',(53.8074256685349,30.5989978195833,12.5349249298422));
#47551=CARTESIAN_POINT('Ctrl Pts',(53.8073864977531,30.5989686042417,12.5349280599789));
#47552=CARTESIAN_POINT('Ctrl Pts',(53.8073669893436,30.5989540534315,12.5349296188921));
#47553=CARTESIAN_POINT('Ctrl Pts',(53.8032720508302,30.5958996297157,12.5352568438614));
#47554=CARTESIAN_POINT('Ctrl Pts',(53.7992082037635,30.5928441467766,12.5355814269861));
#47555=CARTESIAN_POINT('Ctrl Pts',(53.7907535307393,30.5864365898141,12.536256483283));
#47556=CARTESIAN_POINT('Ctrl Pts',(53.7863648497103,30.5830817416007,12.5366067655989));
#47557=CARTESIAN_POINT('Ctrl Pts',(53.7750381924555,30.5743484979265,12.5375106331926));
#47558=CARTESIAN_POINT('Ctrl Pts',(53.7681215993419,30.5689423938447,12.5380624123228));
#47559=CARTESIAN_POINT('Ctrl Pts',(53.7477544398615,30.5528054211746,12.5396874870066));
#47560=CARTESIAN_POINT('Ctrl Pts',(53.7344064362684,30.5419457164503,12.5407528524038));
#47561=CARTESIAN_POINT('Ctrl Pts',(53.6864631204206,30.5018978144699,12.5445876006126));
#47562=CARTESIAN_POINT('Ctrl Pts',(53.6527213766615,30.4717054839354,12.547302310406));
#47563=CARTESIAN_POINT('Ctrl Pts',(53.5095985960259,30.3345866168695,12.5590364742024));
#47564=CARTESIAN_POINT('Ctrl Pts',(53.4116969465367,30.2164349910421,12.5676929370378));
#47565=CARTESIAN_POINT('Ctrl Pts',(53.2920782945655,30.0326800778617,12.5807543067708));
#47566=CARTESIAN_POINT('Ctrl Pts',(53.2586986786024,29.9753425252075,12.5847747144192));
#47567=CARTESIAN_POINT('Ctrl Pts',(53.2210968400383,29.9026476104092,12.5898651574802));
#47568=CARTESIAN_POINT('Ctrl Pts',(53.2141174477524,29.8887590501956,12.5908372996373));
#47569=CARTESIAN_POINT('Ctrl Pts',(53.2033728835073,29.8667403337599,12.5923785544426));
#47570=CARTESIAN_POINT('Ctrl Pts',(53.1994988633785,29.8586637611448,12.5929439001637));
#47571=CARTESIAN_POINT('Ctrl Pts',(53.1924391459161,29.8436877789592,12.5939923305448));
#47572=CARTESIAN_POINT('Ctrl Pts',(53.1892382103987,29.8367957028458,12.5944748807675));
#47573=CARTESIAN_POINT('Ctrl Pts',(53.1822171173267,29.8214493417256,12.5955495608239));
#47574=CARTESIAN_POINT('Ctrl Pts',(53.1784164193892,29.8129863981877,12.5961423415963));
#47575=CARTESIAN_POINT('Ctrl Pts',(53.1676277042094,29.7885078691729,12.597857479758));
#47576=CARTESIAN_POINT('Ctrl Pts',(53.1607910554668,29.7724269003875,12.5989849167366));
#47577=CARTESIAN_POINT('Ctrl Pts',(53.1075557881091,29.6424932672407,12.6081024705636));
#47578=CARTESIAN_POINT('Ctrl Pts',(53.071588248345,29.5247259449193,12.6164396592281));
#47579=CARTESIAN_POINT('Ctrl Pts',(53.0466869618782,29.40446969924,12.6249522205985));
#47580=CARTESIAN_POINT('Origin',(55.,29.,3.45145488139523));
#47581=CARTESIAN_POINT('',(53.0466869980082,29.4044698737233,13.5836009930267));
#47582=CARTESIAN_POINT('',(53.04668699692,29.404469868468,13.4272582639285));
#47583=CARTESIAN_POINT('',(53.0466869980082,29.4044698737233,3.45145488139523));
#47584=CARTESIAN_POINT('',(53.0052507998914,29.001786383575,12.8095451186048));
#47585=CARTESIAN_POINT('Ctrl Pts',(53.0052507998914,29.001786383575,12.8095451186048));
#47586=CARTESIAN_POINT('Ctrl Pts',(53.0051890516009,28.9328357086924,12.8139430725437));
#47587=CARTESIAN_POINT('Ctrl Pts',(53.0087066016235,28.8638003853531,12.8183410264827));
#47588=CARTESIAN_POINT('Ctrl Pts',(53.0158030880324,28.7950849516546,12.8227389804216));
#47589=CARTESIAN_POINT('Ctrl Pts',(53.0228954791111,28.7264091731285,12.8271343963337));
#47590=CARTESIAN_POINT('Ctrl Pts',(53.0335626602207,28.6580534147751,12.8315298122457));
#47591=CARTESIAN_POINT('Ctrl Pts',(53.0477522628778,28.5904193175927,12.8359252281577));
#47592=CARTESIAN_POINT('Ctrl Pts',(53.0619387315161,28.5228001585686,12.8403196732662));
#47593=CARTESIAN_POINT('Ctrl Pts',(53.0796459745629,28.4559028336968,12.8447141183747));
#47594=CARTESIAN_POINT('Ctrl Pts',(53.1007704663719,28.3901190762986,12.8491085634832));
#47595=CARTESIAN_POINT('Ctrl Pts',(53.1223815493405,28.3228200258898,12.8536042322405));
#47596=CARTESIAN_POINT('Ctrl Pts',(53.1475691441378,28.256687014512,12.8580999009978));
#47597=CARTESIAN_POINT('Ctrl Pts',(53.1761690580459,28.1921211367596,12.8625955697552));
#47598=CARTESIAN_POINT('Ctrl Pts',(53.2041597928622,28.1289305142925,12.8669954806225));
#47599=CARTESIAN_POINT('Ctrl Pts',(53.2354186133925,28.067241345108,12.8713953914898));
#47600=CARTESIAN_POINT('Ctrl Pts',(53.269744656693,28.0074054153596,12.8757953023572));
#47601=CARTESIAN_POINT('Ctrl Pts',(53.3051912872886,27.9456161179573,12.8803388500595));
#47602=CARTESIAN_POINT('Ctrl Pts',(53.3439085797145,27.8858036579552,12.8848823977619));
#47603=CARTESIAN_POINT('Ctrl Pts',(53.3856280207344,27.828321428436,12.8894259454642));
#47604=CARTESIAN_POINT('Ctrl Pts',(53.4273474617544,27.7708391989169,12.8939694931665));
#47605=CARTESIAN_POINT('Ctrl Pts',(53.4720686272115,27.715687600944,12.8985130408689));
#47606=CARTESIAN_POINT('Ctrl Pts',(53.5194807316863,27.6631790476463,12.9030565885712));
#47607=CARTESIAN_POINT('Ctrl Pts',(53.5659798138644,27.6116816597558,12.9075126404662));
#47608=CARTESIAN_POINT('Ctrl Pts',(53.6152600337689,27.5625123993747,12.9119686923612));
#47609=CARTESIAN_POINT('Ctrl Pts',(53.6670591499095,27.515986437845,12.9164247442562));
#47610=CARTESIAN_POINT('Ctrl Pts',(53.7187809653277,27.4695299078173,12.9208741463074));
#47611=CARTESIAN_POINT('Ctrl Pts',(53.7730138550993,27.4257091713566,12.9253235483587));
#47612=CARTESIAN_POINT('Ctrl Pts',(53.8294571511627,27.3848043457414,12.9297729504099));
#47613=CARTESIAN_POINT('Ctrl Pts',(53.8858345639926,27.3439472661363,12.9342171589126));
#47614=CARTESIAN_POINT('Ctrl Pts',(53.9444168644604,27.3059996228174,12.9386613674154));
#47615=CARTESIAN_POINT('Ctrl Pts',(54.0048699297654,27.2712016584301,12.9431055759181));
#47616=CARTESIAN_POINT('Ctrl Pts',(54.0652853203789,27.2364253803305,12.9475470147651));
#47617=CARTESIAN_POINT('Ctrl Pts',(54.1275687400213,27.2047951304345,12.951988453612));
#47618=CARTESIAN_POINT('Ctrl Pts',(54.1913579525975,27.1765073069319,12.956429892459));
#47619=CARTESIAN_POINT('Ctrl Pts',(54.2551290295052,27.1482275258328,12.9608700685773));
#47620=CARTESIAN_POINT('Ctrl Pts',(54.3204046026038,27.1232884826883,12.9653102446956));
#47621=CARTESIAN_POINT('Ctrl Pts',(54.386800359913,27.1018393735257,12.969750420814));
#47622=CARTESIAN_POINT('Ctrl Pts',(54.4531997412496,27.0803890936233,12.9741908392869));
#47623=CARTESIAN_POINT('Ctrl Pts',(54.5207189620964,27.0624292738929,12.9786312577599));
#47624=CARTESIAN_POINT('Ctrl Pts',(54.5889580729728,27.0480594023573,12.9830716762329));
#47625=CARTESIAN_POINT('Ctrl Pts',(54.6572691170193,27.0336743830509,12.9875167755022));
#47626=CARTESIAN_POINT('Ctrl Pts',(54.7263010862091,27.0228869657343,12.9919618747714));
#47627=CARTESIAN_POINT('Ctrl Pts',(54.7956442995689,27.0157454018697,12.9964069740407));
#47628=CARTESIAN_POINT('Ctrl Pts',(54.8650282663177,27.0085996408686,13.0008546857193));
#47629=CARTESIAN_POINT('Ctrl Pts',(54.9347233528058,27.0051040226376,13.0053023973979));
#47630=CARTESIAN_POINT('Ctrl Pts',(55.0043180075572,27.0052546735709,13.0097501090766));
#47631=CARTESIAN_POINT('Ctrl Pts',(55.0740323330363,27.0054055835544,13.0142054687692));
#47632=CARTESIAN_POINT('Ctrl Pts',(55.1436453939375,27.0092152509383,13.0186608284618));
#47633=CARTESIAN_POINT('Ctrl Pts',(55.2127497158283,27.0166278410457,13.0231161881544));
#47634=CARTESIAN_POINT('Ctrl Pts',(55.2470960604591,27.0203120588699,13.0253305984151));
#47635=CARTESIAN_POINT('Ctrl Pts',(55.2813168731432,27.0248855094267,13.0275450086759));
#47636=CARTESIAN_POINT('Ctrl Pts',(55.3153632560029,27.0303366837799,13.0297594189366));
#47637=CARTESIAN_POINT('Ctrl Pts',(55.3838747019394,27.0413060674741,13.0342154708316));
#47638=CARTESIAN_POINT('Ctrl Pts',(55.4519473094091,27.0558757741474,13.0386715227266));
#47639=CARTESIAN_POINT('Ctrl Pts',(55.5191739402604,27.0739974085546,13.0431275746216));
#47640=CARTESIAN_POINT('Ctrl Pts',(55.5863002476406,27.0920919997314,13.0475769766729));
#47641=CARTESIAN_POINT('Ctrl Pts',(55.6525826157851,27.1137278715667,13.0520263787241));
#47642=CARTESIAN_POINT('Ctrl Pts',(55.7176223913188,27.1388053121777,13.0564757807753));
#47643=CARTESIAN_POINT('Ctrl Pts',(55.7825862494096,27.1638534812368,13.060919989278));
#47644=CARTESIAN_POINT('Ctrl Pts',(55.8463099415538,27.1923350651303,13.0653641977808));
#47645=CARTESIAN_POINT('Ctrl Pts',(55.9084100494376,27.2241005815135,13.0698084062836));
#47646=CARTESIAN_POINT('Ctrl Pts',(55.9704714561837,27.2558463014476,13.0742498451305));
#47647=CARTESIAN_POINT('Ctrl Pts',(56.030910851616,27.2908716715472,13.0786912839774));
#47648=CARTESIAN_POINT('Ctrl Pts',(56.0893662903561,27.3289797583704,13.0831327228244));
#47649=CARTESIAN_POINT('Ctrl Pts',(56.1478051098524,27.3670770108283,13.0875728989427));
#47650=CARTESIAN_POINT('Ctrl Pts',(56.2042606830138,27.4082549730815,13.092013075061));
#47651=CARTESIAN_POINT('Ctrl Pts',(56.2583986406965,27.4522724969836,13.0964532511794));
#47652=CARTESIAN_POINT('Ctrl Pts',(56.3125395533489,27.4962924234598,13.1008936696524));
#47653=CARTESIAN_POINT('Ctrl Pts',(56.3643622214861,27.5431519088996,13.1053340881254));
#47654=CARTESIAN_POINT('Ctrl Pts',(56.4135654592249,27.592569626949,13.1097745065984));
#47655=CARTESIAN_POINT('Ctrl Pts',(56.4628205637716,27.6420394378974,13.1142196058676));
#47656=CARTESIAN_POINT('Ctrl Pts',(56.5094503812403,27.6940725164669,13.1186647051369));
#47657=CARTESIAN_POINT('Ctrl Pts',(56.5531914064352,27.7483514800569,13.1231098044062));
#47658=CARTESIAN_POINT('Ctrl Pts',(56.5969581384719,27.8026623436931,13.1275575160848));
#47659=CARTESIAN_POINT('Ctrl Pts',(56.6378324125062,27.8592213230825,13.1320052277634));
#47660=CARTESIAN_POINT('Ctrl Pts',(56.6755934288613,27.9176810896704,13.1364529394421));
#47661=CARTESIAN_POINT('Ctrl Pts',(56.713419376759,27.9762413801108,13.1409082991347));
#47662=CARTESIAN_POINT('Ctrl Pts',(56.7481211381305,28.0367085577472,13.1453636588273));
#47663=CARTESIAN_POINT('Ctrl Pts',(56.7795237191017,28.0987104263032,13.1498190185199));
#47664=CARTESIAN_POINT('Ctrl Pts',(56.7951314819567,28.1295266978026,13.1520334287806));
#47665=CARTESIAN_POINT('Ctrl Pts',(56.8099249942695,28.1607217689548,13.1542478390414));
#47666=CARTESIAN_POINT('Ctrl Pts',(56.8238872899822,28.1922483575124,13.1564622493021));
#47667=CARTESIAN_POINT('Ctrl Pts',(56.8519835806166,28.2556892280575,13.1609183011971));
#47668=CARTESIAN_POINT('Ctrl Pts',(56.8768209254941,28.3207220085586,13.1653743530921));
#47669=CARTESIAN_POINT('Ctrl Pts',(56.8982182734294,28.3869788348524,13.1698304049871));
#47670=CARTESIAN_POINT('Ctrl Pts',(56.91958368973,28.4531367849315,13.1742798070383));
#47671=CARTESIAN_POINT('Ctrl Pts',(56.9375191492765,28.5205146935349,13.1787292090895));
#47672=CARTESIAN_POINT('Ctrl Pts',(56.951891265693,28.5887238769252,13.1831786111407));
#47673=CARTESIAN_POINT('Ctrl Pts',(56.9662466063086,28.6568534433929,13.1876228196435));
#47674=CARTESIAN_POINT('Ctrl Pts',(56.9770467646036,28.7258118811823,13.1920670281462));
#47675=CARTESIAN_POINT('Ctrl Pts',(56.9842083969008,28.7951961910305,13.196511236649));
#47676=CARTESIAN_POINT('Ctrl Pts',(56.9913655660283,28.8645372601852,13.2009526754959));
#47677=CARTESIAN_POINT('Ctrl Pts',(56.994888657593,28.934303189525,13.2053941143429));
#47678=CARTESIAN_POINT('Ctrl Pts',(56.994745820978,29.0040831594111,13.2098355531898));
#47679=CARTESIAN_POINT('Ctrl Pts',(56.9946030249724,29.0738432904193,13.2142757293081));
#47680=CARTESIAN_POINT('Ctrl Pts',(56.9907963709682,29.143616965266,13.2187159054265));
#47681=CARTESIAN_POINT('Ctrl Pts',(56.9833461092831,29.2129924254327,13.2231560815448));
#47682=CARTESIAN_POINT('Ctrl Pts',(56.9758954409461,29.2823716722658,13.2275965000178));
#47683=CARTESIAN_POINT('Ctrl Pts',(56.9648008247325,29.3513521753054,13.2320369184908));
#47684=CARTESIAN_POINT('Ctrl Pts',(56.9501342784475,29.4195281379407,13.2364773369638));
#47685=CARTESIAN_POINT('Ctrl Pts',(56.9354522716568,29.4877759671792,13.240922436233));
#47686=CARTESIAN_POINT('Ctrl Pts',(56.9171909229189,29.5552170843471,13.2453675355023));
#47687=CARTESIAN_POINT('Ctrl Pts',(56.8954730083251,29.6214576712948,13.2498126347716));
#47688=CARTESIAN_POINT('Ctrl Pts',(56.873742329993,29.6877371882009,13.2542603464502));
#47689=CARTESIAN_POINT('Ctrl Pts',(56.8485512189845,29.7528143143941,13.2587080581288));
#47690=CARTESIAN_POINT('Ctrl Pts',(56.8200708197311,29.8163147515899,13.2631557698074));
#47691=CARTESIAN_POINT('Ctrl Pts',(56.7915414473187,29.8799243802681,13.2676111295001));
#47692=CARTESIAN_POINT('Ctrl Pts',(56.7597117201564,29.9419514733999,13.2720664891927));
#47693=CARTESIAN_POINT('Ctrl Pts',(56.7247985790647,30.0020466177561,13.2765218488853));
#47694=CARTESIAN_POINT('Ctrl Pts',(56.7074459917984,30.0319152060329,13.278736259146));
#47695=CARTESIAN_POINT('Ctrl Pts',(56.6893323791755,30.0613069992499,13.2809506694068));
#47696=CARTESIAN_POINT('Ctrl Pts',(56.6704881664024,30.0901820253561,13.2831650796675));
#47697=CARTESIAN_POINT('Ctrl Pts',(56.6325680070147,30.1482871638118,13.2876211315625));
#47698=CARTESIAN_POINT('Ctrl Pts',(56.5915383406987,30.2045252534154,13.2920771834575));
#47699=CARTESIAN_POINT('Ctrl Pts',(56.5476091767831,30.2585441583181,13.2965332353525));
#47700=CARTESIAN_POINT('Ctrl Pts',(56.5037455691235,30.3124824498689,13.3009826374037));
#47701=CARTESIAN_POINT('Ctrl Pts',(56.4569913582548,30.3642077535697,13.305432039455));
#47702=CARTESIAN_POINT('Ctrl Pts',(56.407599966251,30.4133965818235,13.3098814415062));
#47703=CARTESIAN_POINT('Ctrl Pts',(56.3582662261708,30.4625279945953,13.3143256500089));
#47704=CARTESIAN_POINT('Ctrl Pts',(56.3063017637939,30.5091284689646,13.3187698585117));
#47705=CARTESIAN_POINT('Ctrl Pts',(56.2519992527036,30.5529087010284,13.3232140670144));
#47706=CARTESIAN_POINT('Ctrl Pts',(56.1977305832446,30.5966616490046,13.3276555058614));
#47707=CARTESIAN_POINT('Ctrl Pts',(56.141127135589,30.6375975352699,13.3320969447083));
#47708=CARTESIAN_POINT('Ctrl Pts',(56.0825161761122,30.6754659921811,13.3365383835553));
#47709=CARTESIAN_POINT('Ctrl Pts',(56.0239218800946,30.7133236828552,13.3409785596736));
#47710=CARTESIAN_POINT('Ctrl Pts',(55.9633216159151,30.7481154102871,13.3454187357919));
#47711=CARTESIAN_POINT('Ctrl Pts',(55.9010718012957,30.7796339992846,13.3498589119103));
#47712=CARTESIAN_POINT('Ctrl Pts',(55.838818588944,30.8111543086363,13.3542993303832));
#47713=CARTESIAN_POINT('Ctrl Pts',(55.7749160847834,30.839400906139,13.3587397488562));
#47714=CARTESIAN_POINT('Ctrl Pts',(55.7097438877997,30.8642132861427,13.3631801673292));
#47715=CARTESIAN_POINT('Ctrl Pts',(55.6445029905841,30.889051821721,13.3676252665984));
#47716=CARTESIAN_POINT('Ctrl Pts',(55.5779901871625,30.9104487402747,13.3720703658677));
#47717=CARTESIAN_POINT('Ctrl Pts',(55.510602661537,30.9282926345685,13.376515465137));
#47718=CARTESIAN_POINT('Ctrl Pts',(55.443175531891,30.9461470158175,13.3809631768156));
#47719=CARTESIAN_POINT('Ctrl Pts',(55.374873135569,30.9604441163661,13.3854108884943));
#47720=CARTESIAN_POINT('Ctrl Pts',(55.3061026145814,30.9711237281932,13.3898586001729));
#47721=CARTESIAN_POINT('Ctrl Pts',(55.2372138399965,30.9818217040302,13.3943139598655));
#47722=CARTESIAN_POINT('Ctrl Pts',(55.1678558203644,30.9888897254161,13.3987693195581));
#47723=CARTESIAN_POINT('Ctrl Pts',(55.0984397550739,30.9923195469405,13.4032246792507));
#47724=CARTESIAN_POINT('Ctrl Pts',(55.0639384672216,30.9940242425206,13.4054390895115));
#47725=CARTESIAN_POINT('Ctrl Pts',(55.029422824276,30.9948310032179,13.4076534997722));
#47726=CARTESIAN_POINT('Ctrl Pts',(54.9949429193088,30.9947435896463,13.409867910033));
#47727=CARTESIAN_POINT('Ctrl Pts',(54.9255590979858,30.9945676875479,13.414323961928));
#47728=CARTESIAN_POINT('Ctrl Pts',(54.8560485862619,30.9907670296928,13.418780013823));
#47729=CARTESIAN_POINT('Ctrl Pts',(54.7868210938184,30.9833260741641,13.423236065718));
#47730=CARTESIAN_POINT('Ctrl Pts',(54.7176969107666,30.9758962229028,13.4276854677692));
#47731=CARTESIAN_POINT('Ctrl Pts',(54.6488553910336,30.9648369083776,13.4321348698204));
#47732=CARTESIAN_POINT('Ctrl Pts',(54.5807058473582,30.9501846005085,13.4365842718716));
#47733=CARTESIAN_POINT('Ctrl Pts',(54.5126358509912,30.9355493954927,13.4410284803744));
#47734=CARTESIAN_POINT('Ctrl Pts',(54.4452567022659,30.9173296293411,13.4454726888771));
#47735=CARTESIAN_POINT('Ctrl Pts',(54.3789704083292,30.8956133067609,13.4499168973799));
#47736=CARTESIAN_POINT('Ctrl Pts',(54.312725424385,30.8739105179156,13.4543583362268));
#47737=CARTESIAN_POINT('Ctrl Pts',(54.2475724077383,30.8487156475518,13.4587997750738));
#47738=CARTESIAN_POINT('Ctrl Pts',(54.1838995371631,30.8201669146145,13.4632412139207));
#47739=CARTESIAN_POINT('Ctrl Pts',(54.1202447691797,30.791626298259,13.467681390039));
#47740=CARTESIAN_POINT('Ctrl Pts',(54.0580697578255,30.7597339123429,13.4721215661574));
#47741=CARTESIAN_POINT('Ctrl Pts',(53.9977423209735,30.7246759427012,13.4765617422757));
#47742=CARTESIAN_POINT('Ctrl Pts',(53.9374115913163,30.6896160595179,13.4810021607487));
#47743=CARTESIAN_POINT('Ctrl Pts',(53.8789290579547,30.6513904973879,13.4854425792217));
#47744=CARTESIAN_POINT('Ctrl Pts',(53.8226360110713,30.6102302941113,13.4898829976947));
#47745=CARTESIAN_POINT('Ctrl Pts',(53.7662836237708,30.5690267024633,13.4943280969639));
#47746=CARTESIAN_POINT('Ctrl Pts',(53.7121257248894,30.5248825847199,13.4987731962332));
#47747=CARTESIAN_POINT('Ctrl Pts',(53.6604719929179,30.478070458653,13.5032182955025));
#47748=CARTESIAN_POINT('Ctrl Pts',(53.608787903763,30.4312308208413,13.5076660071811));
#47749=CARTESIAN_POINT('Ctrl Pts',(53.5596112555166,30.3817204007798,13.5121137188597));
#47750=CARTESIAN_POINT('Ctrl Pts',(53.5132142006241,30.3298479421626,13.5165614305384));
#47751=CARTESIAN_POINT('Ctrl Pts',(53.4667373641832,30.2778862868264,13.521016790231));
#47752=CARTESIAN_POINT('Ctrl Pts',(53.4230499677281,30.223554866777,13.5254721499236));
#47753=CARTESIAN_POINT('Ctrl Pts',(53.3823827849961,30.167194117627,13.5299275096162));
#47754=CARTESIAN_POINT('Ctrl Pts',(53.3621703144147,30.1391816046469,13.532141919877));
#47755=CARTESIAN_POINT('Ctrl Pts',(53.3427032393411,30.1106682137782,13.5343563301377));
#47756=CARTESIAN_POINT('Ctrl Pts',(53.3240056759864,30.0816980116345,13.5365707403984));
#47757=CARTESIAN_POINT('Ctrl Pts',(53.2855729774195,30.0221499825526,13.5411224437642));
#47758=CARTESIAN_POINT('Ctrl Pts',(53.2502489871136,29.9604451874632,13.54567414713));
#47759=CARTESIAN_POINT('Ctrl Pts',(53.2182765830912,29.8969332350508,13.5502258504958));
#47760=CARTESIAN_POINT('Ctrl Pts',(53.1863531525859,29.8335185666491,13.5547705818203));
#47761=CARTESIAN_POINT('Ctrl Pts',(53.1577713218888,29.768302644132,13.5593153131447));
#47762=CARTESIAN_POINT('Ctrl Pts',(53.1327301960058,29.701663054173,13.5638600444692));
#47763=CARTESIAN_POINT('Ctrl Pts',(53.1077286374661,29.6351287610584,13.568397594689));
#47764=CARTESIAN_POINT('Ctrl Pts',(53.0862568201633,29.5671757024611,13.5729351449088));
#47765=CARTESIAN_POINT('Ctrl Pts',(53.0684666775928,29.4982033590118,13.5774726951287));
#47766=CARTESIAN_POINT('Ctrl Pts',(53.0604577088734,29.4671526049776,13.5795154610947));
#47767=CARTESIAN_POINT('Ctrl Pts',(53.0531942706169,29.4358955521725,13.5815582270607));
#47768=CARTESIAN_POINT('Ctrl Pts',(53.0466869980082,29.4044698737233,13.5836009930267));
#47769=CARTESIAN_POINT('Ctrl Pts',(53.0052508197207,29.0018083902244,12.809862253678));
#47770=CARTESIAN_POINT('Ctrl Pts',(53.0053734539764,29.1370804004845,12.8004754443569));
#47771=CARTESIAN_POINT('Ctrl Pts',(53.019255454431,29.2719942701512,12.7909324149165));
#47772=CARTESIAN_POINT('Ctrl Pts',(53.0466869981368,29.4044698743445,12.7818778464297));
#47773=CARTESIAN_POINT('',(53.0052496133582,28.9993761608918,12.6531293428976));
#47774=CARTESIAN_POINT('Ctrl Pts',(53.0466869618782,29.40446969924,12.6249522205985));
#47775=CARTESIAN_POINT('Ctrl Pts',(53.0420700593701,29.3821732061242,12.6265305192134));
#47776=CARTESIAN_POINT('Ctrl Pts',(53.0378335579175,29.3597910973607,12.6281140142711));
#47777=CARTESIAN_POINT('Ctrl Pts',(53.0148268141735,29.2257048289013,12.6375857831214));
#47778=CARTESIAN_POINT('Ctrl Pts',(53.0052148113952,29.1126451148838,12.6455257903824));
#47779=CARTESIAN_POINT('Ctrl Pts',(53.0052500967933,28.9993785847915,12.6531300191543));
#47780=CARTESIAN_POINT('Ctrl Pts',(53.0052500975323,28.9993762171256,12.6531301781092));
#47781=CARTESIAN_POINT('Ctrl Pts',(53.005258509644,28.9724757367139,12.6549361597253));
#47782=CARTESIAN_POINT('Ctrl Pts',(53.0058110777771,28.9455763451103,12.6567216238253));
#47783=CARTESIAN_POINT('Ctrl Pts',(53.0071539488144,28.9126576596725,12.6588751396755));
#47784=CARTESIAN_POINT('Ctrl Pts',(53.0074276493387,28.9066217491526,12.6592687057323));
#47785=CARTESIAN_POINT('Ctrl Pts',(53.0079488580194,28.8961765363347,12.6599474213631));
#47786=CARTESIAN_POINT('Ctrl Pts',(53.0081835894833,28.8917666799494,12.6602332408541));
#47787=CARTESIAN_POINT('Ctrl Pts',(53.0086619027922,28.8833098917081,12.6607799162569));
#47788=CARTESIAN_POINT('Ctrl Pts',(53.0089031819618,28.8792628435459,12.6610408976375));
#47789=CARTESIAN_POINT('Ctrl Pts',(53.0094096150325,28.8711830188659,12.6615606382477));
#47790=CARTESIAN_POINT('Ctrl Pts',(53.0096746881991,28.8671502756342,12.6618194020265));
#47791=CARTESIAN_POINT('Ctrl Pts',(53.0103328114064,28.8575821816223,12.6624318724954));
#47792=CARTESIAN_POINT('Ctrl Pts',(53.0107367097063,28.8520475752137,12.6627849819217));
#47793=CARTESIAN_POINT('Ctrl Pts',(53.0120197303878,28.8354224180735,12.6638423466634));
#47794=CARTESIAN_POINT('Ctrl Pts',(53.0129685598533,28.824337249783,12.664542917958));
#47795=CARTESIAN_POINT('Ctrl Pts',(53.0170786580199,28.780626063589,12.6672898950697));
#47796=CARTESIAN_POINT('Ctrl Pts',(53.0209513186601,28.7480703284126,12.6693016686706));
#47797=CARTESIAN_POINT('Ctrl Pts',(53.0462820404368,28.5722040552806,12.6800546980204));
#47798=CARTESIAN_POINT('Ctrl Pts',(53.082505936071,28.431451549809,12.6882737896722));
#47799=CARTESIAN_POINT('Ctrl Pts',(53.1666153451381,28.2085192389684,12.7022277418259));
#47800=CARTESIAN_POINT('Ctrl Pts',(53.2056524155551,28.1236126314987,12.7077818172185));
#47801=CARTESIAN_POINT('Ctrl Pts',(53.2613415874518,28.0219380941724,12.7149350482694));
#47802=CARTESIAN_POINT('Ctrl Pts',(53.2725321979323,28.002306111188,12.716340401782));
#47803=CARTESIAN_POINT('Ctrl Pts',(53.2892947868855,27.9740268563558,12.7184022950935));
#47804=CARTESIAN_POINT('Ctrl Pts',(53.294604209995,27.9652254299716,12.7190494100881));
#47805=CARTESIAN_POINT('Ctrl Pts',(53.3040479025908,27.9498407401896,12.7201902466597));
#47806=CARTESIAN_POINT('Ctrl Pts',(53.3081531055625,27.9432398234786,12.7206829029397));
#47807=CARTESIAN_POINT('Ctrl Pts',(53.3162167258366,27.9304414349278,12.7216443796122));
#47808=CARTESIAN_POINT('Ctrl Pts',(53.3201710430309,27.9242415180766,12.7221130437136));
#47809=CARTESIAN_POINT('Ctrl Pts',(53.3308642827153,27.9076784693703,12.7233729533457));
#47810=CARTESIAN_POINT('Ctrl Pts',(53.3376653196701,27.8973560102034,12.7241664895252));
#47811=CARTESIAN_POINT('Ctrl Pts',(53.3631498778221,27.8594478222072,12.727112100226));
#47812=CARTESIAN_POINT('Ctrl Pts',(53.3824268371305,27.8322695364704,12.7292862501438));
#47813=CARTESIAN_POINT('Ctrl Pts',(53.5326205455334,27.6313729350644,12.7458437135092));
#47814=CARTESIAN_POINT('Ctrl Pts',(53.6904841149691,27.4796474602261,12.7613830213825));
#47815=CARTESIAN_POINT('Ctrl Pts',(53.8936803471424,27.3398987856025,12.778164471115));
#47816=CARTESIAN_POINT('Ctrl Pts',(53.9180869401973,27.3238903594304,12.780131195552));
#47817=CARTESIAN_POINT('Ctrl Pts',(53.9536389455595,27.3016718947633,12.782917500711));
#47818=CARTESIAN_POINT('Ctrl Pts',(53.9645053554937,27.2950247306425,12.7837588542112));
#47819=CARTESIAN_POINT('Ctrl Pts',(53.981534268291,27.2848307231675,12.7850605566893));
#47820=CARTESIAN_POINT('Ctrl Pts',(53.9876531183372,27.2812120870877,12.7855249482218));
#47821=CARTESIAN_POINT('Ctrl Pts',(53.9991334821608,27.2745052723796,12.7863898430106));
#47822=CARTESIAN_POINT('Ctrl Pts',(54.0044902533456,27.2714091900203,12.7867908175676));
#47823=CARTESIAN_POINT('Ctrl Pts',(54.0136406767586,27.2661771139352,12.7874712508678));
#47824=CARTESIAN_POINT('Ctrl Pts',(54.0174270501321,27.2640285387459,12.7877515011323));
#47825=CARTESIAN_POINT('Ctrl Pts',(54.0247644428291,27.2598966372955,12.7882920144446));
#47826=CARTESIAN_POINT('Ctrl Pts',(54.0283145220785,27.2579117595308,12.7885523804664));
#47827=CARTESIAN_POINT('Ctrl Pts',(54.0368098159874,27.2531960201805,12.7891727445255));
#47828=CARTESIAN_POINT('Ctrl Pts',(54.0417606419014,27.2504752619845,12.7895321085822));
#47829=CARTESIAN_POINT('Ctrl Pts',(54.0595239779061,27.2408113294044,12.7908139930658));
#47830=CARTESIAN_POINT('Ctrl Pts',(54.0724012935901,27.2339873738655,12.7917293754081));
#47831=CARTESIAN_POINT('Ctrl Pts',(54.2109526135514,27.1624998425249,12.8014428298402));
#47832=CARTESIAN_POINT('Ctrl Pts',(54.3431035534356,27.1112169097634,12.809542835432));
#47833=CARTESIAN_POINT('Ctrl Pts',(54.6091972642971,27.0393042639946,12.825562867554));
#47834=CARTESIAN_POINT('Ctrl Pts',(54.7419984089862,27.0174554376566,12.8334384882912));
#47835=CARTESIAN_POINT('Ctrl Pts',(54.8933239499874,27.0080286570439,12.8428492364542));
#47836=CARTESIAN_POINT('Ctrl Pts',(54.9106827996876,27.0071748649683,12.8439346452484));
#47837=CARTESIAN_POINT('Ctrl Pts',(54.9373017051486,27.0062141066126,12.8456089950573));
#47838=CARTESIAN_POINT('Ctrl Pts',(54.9465553220098,27.0059446029238,12.8461928904665));
#47839=CARTESIAN_POINT('Ctrl Pts',(54.9627318041459,27.0055861577793,12.8472169549449));
#47840=CARTESIAN_POINT('Ctrl Pts',(54.9696539316157,27.0054688253542,12.8476562345475));
#47841=CARTESIAN_POINT('Ctrl Pts',(54.9853022799942,27.0052850604732,12.8486517628217));
#47842=CARTESIAN_POINT('Ctrl Pts',(54.9940285630985,27.0052398512805,12.8492086619283));
#47843=CARTESIAN_POINT('Ctrl Pts',(55.0176607716491,27.0052724873913,12.8507216949258));
#47844=CARTESIAN_POINT('Ctrl Pts',(55.0325657496042,27.0054601521964,12.8516812127403));
#47845=CARTESIAN_POINT('Ctrl Pts',(55.1025835820192,27.0071267623856,12.856214204079));
#47846=CARTESIAN_POINT('Ctrl Pts',(55.1576172690809,27.010723006665,12.8598524806449));
#47847=CARTESIAN_POINT('Ctrl Pts',(55.391093871695,27.0357288709439,12.8756180582932));
#47848=CARTESIAN_POINT('Ctrl Pts',(55.566348323001,27.0789199314493,12.8883765795719));
#47849=CARTESIAN_POINT('Ctrl Pts',(55.7832258921363,27.1646650176396,12.9043494143566));
#47850=CARTESIAN_POINT('Ctrl Pts',(55.8322349945113,27.1863618540079,12.9079636054641));
#47851=CARTESIAN_POINT('Ctrl Pts',(55.8887757539769,27.2141685095905,12.9120919796301));
#47852=CARTESIAN_POINT('Ctrl Pts',(55.8972067387195,27.2183893440583,12.9127064544593));
#47853=CARTESIAN_POINT('Ctrl Pts',(55.9101533827926,27.2249860816154,12.9136479498189));
#47854=CARTESIAN_POINT('Ctrl Pts',(55.9146902485402,27.2273197295348,12.9139774767896));
#47855=CARTESIAN_POINT('Ctrl Pts',(55.9230376726558,27.2316540103501,12.9145829700766));
#47856=CARTESIAN_POINT('Ctrl Pts',(55.9268506933373,27.2336495599271,12.9148592340194));
#47857=CARTESIAN_POINT('Ctrl Pts',(55.935458577342,27.2381900561372,12.9154821982093));
#47858=CARTESIAN_POINT('Ctrl Pts',(55.9402495222327,27.2407422400837,12.9158284399616));
#47859=CARTESIAN_POINT('Ctrl Pts',(55.954411980335,27.2483611022329,12.9168506984003));
#47860=CARTESIAN_POINT('Ctrl Pts',(55.9637535634786,27.2534834277916,12.9175233365335));
#47861=CARTESIAN_POINT('Ctrl Pts',(56.054349375983,27.3041086046727,12.9240349945454));
#47862=CARTESIAN_POINT('Ctrl Pts',(56.1323752267257,27.355180490015,12.9295537695112));
#47863=CARTESIAN_POINT('Ctrl Pts',(56.2944189346148,27.4782637066949,12.9414463241599));
#47864=CARTESIAN_POINT('Ctrl Pts',(56.3765925310782,27.5521759292839,12.9477758710708));
#47865=CARTESIAN_POINT('Ctrl Pts',(56.4888459720409,27.6713851064656,12.9574575690478));
#47866=CARTESIAN_POINT('Ctrl Pts',(56.5238804198786,27.7117190892901,12.9606546419061));
#47867=CARTESIAN_POINT('Ctrl Pts',(56.5717503339568,27.7715185701758,12.965327575746));
#47868=CARTESIAN_POINT('Ctrl Pts',(56.5859304580374,27.7898800669154,12.9667537405785));
#47869=CARTESIAN_POINT('Ctrl Pts',(56.6107108074562,27.8231513605512,12.9693258810721));
#47870=CARTESIAN_POINT('Ctrl Pts',(56.621432380324,27.8379677169106,12.9704671510169));
#47871=CARTESIAN_POINT('Ctrl Pts',(56.6373801969232,27.8606568225585,12.9722096803928));
#47872=CARTESIAN_POINT('Ctrl Pts',(56.6427569098827,27.8684229962685,12.9728052231761));
#47873=CARTESIAN_POINT('Ctrl Pts',(56.6524045956514,27.8825718856845,12.9738887424962));
#47874=CARTESIAN_POINT('Ctrl Pts',(56.6566942758634,27.8889416702826,12.9743760033577));
#47875=CARTESIAN_POINT('Ctrl Pts',(56.6658470247894,27.9027035299753,12.9754276608575));
#47876=CARTESIAN_POINT('Ctrl Pts',(56.6706978898526,27.91010348664,12.9759924984914));
#47877=CARTESIAN_POINT('Ctrl Pts',(56.6836740925846,27.9301887791068,12.9775239866285));
#47878=CARTESIAN_POINT('Ctrl Pts',(56.6917050952847,27.942934085098,12.9784940807524));
#47879=CARTESIAN_POINT('Ctrl Pts',(56.730807861266,28.0065777533603,12.9833307541744));
#47880=CARTESIAN_POINT('Ctrl Pts',(56.759727867836,28.058756025133,12.9872739281187));
#47881=CARTESIAN_POINT('Ctrl Pts',(56.8466202679737,28.2335742339024,13.0004206178233));
#47882=CARTESIAN_POINT('Ctrl Pts',(56.8944306704516,28.3608290766274,13.009919336971));
#47883=CARTESIAN_POINT('Ctrl Pts',(56.95003357156,28.5719329934062,13.025091233151));
#47884=CARTESIAN_POINT('Ctrl Pts',(56.9661105339601,28.6531794661694,13.0307895191124));
#47885=CARTESIAN_POINT('Ctrl Pts',(56.9791976622831,28.7508917520852,13.0373158786409));
#47886=CARTESIAN_POINT('Ctrl Pts',(56.9811128620717,28.7666115451036,13.0383557647059));
#47887=CARTESIAN_POINT('Ctrl Pts',(56.9835265916393,28.788601476027,13.0397948615663));
#47888=CARTESIAN_POINT('Ctrl Pts',(56.9841829229186,28.7948532070713,13.0402022425832));
#47889=CARTESIAN_POINT('Ctrl Pts',(56.9852505327707,28.8055072443768,13.0408933858884));
#47890=CARTESIAN_POINT('Ctrl Pts',(56.9856767446721,28.8099079776097,13.0411779660155));
#47891=CARTESIAN_POINT('Ctrl Pts',(56.9864693445362,28.8183854125024,13.041724393136));
#47892=CARTESIAN_POINT('Ctrl Pts',(56.9868378195759,28.8224618502742,13.0419863598279));
#47893=CARTESIAN_POINT('Ctrl Pts',(56.9876934405249,28.8322639896143,13.0426144517984));
#47894=CARTESIAN_POINT('Ctrl Pts',(56.9881684008509,28.8379907580309,13.0429799068639));
#47895=CARTESIAN_POINT('Ctrl Pts',(56.9898151031853,28.8589445216109,13.0443118553914));
#47896=CARTESIAN_POINT('Ctrl Pts',(56.9908367509594,28.8741832405085,13.0452704435188));
#47897=CARTESIAN_POINT('Ctrl Pts',(56.9990238046862,29.0216592298222,13.0544629434021));
#47898=CARTESIAN_POINT('Ctrl Pts',(56.993179481434,29.1543077908929,13.0620895835918));
#47899=CARTESIAN_POINT('Ctrl Pts',(56.9539738731566,29.4254964389924,13.078003732705));
#47900=CARTESIAN_POINT('Ctrl Pts',(56.9188740128804,29.563006623236,13.0862714786937));
#47901=CARTESIAN_POINT('Ctrl Pts',(56.8633221346202,29.7123021543208,13.0961539328045));
#47902=CARTESIAN_POINT('Ctrl Pts',(56.8568988089205,29.7288830619931,13.0972640425058));
#47903=CARTESIAN_POINT('Ctrl Pts',(56.8467642940753,29.7540400944956,13.0989685654779));
#47904=CARTESIAN_POINT('Ctrl Pts',(56.8432129795499,29.7626799651483,13.0995576412356));
#47905=CARTESIAN_POINT('Ctrl Pts',(56.8369211555333,29.7776864865177,13.1005873661059));
#47906=CARTESIAN_POINT('Ctrl Pts',(56.8342078830856,29.7840644377953,13.1010270920073));
#47907=CARTESIAN_POINT('Ctrl Pts',(56.8280277934161,29.7983840155855,13.1020191073718));
#47908=CARTESIAN_POINT('Ctrl Pts',(56.8245423738731,29.8063174138656,13.1025720199074));
#47909=CARTESIAN_POINT('Ctrl Pts',(56.8150347676198,29.827581000764,13.1040630300306));
#47910=CARTESIAN_POINT('Ctrl Pts',(56.8089175558138,29.8408678718873,13.1050043453805));
#47911=CARTESIAN_POINT('Ctrl Pts',(56.7801801493911,29.9015217495957,13.1093466980461));
#47912=CARTESIAN_POINT('Ctrl Pts',(56.7558437163744,29.9480479051199,13.1128061941598));
#47913=CARTESIAN_POINT('Ctrl Pts',(56.638753371119,30.1518927778984,13.128560038587));
#47914=CARTESIAN_POINT('Ctrl Pts',(56.5264955286858,30.2969822525403,13.1415268472822));
#47915=CARTESIAN_POINT('Ctrl Pts',(56.3702829227037,30.4500551217581,13.1565085240204));
#47916=CARTESIAN_POINT('Ctrl Pts',(56.3437703476986,30.4746581664952,13.1589607422659));
#47917=CARTESIAN_POINT('Ctrl Pts',(56.3000957447577,30.5130305330613,13.1628393331244));
#47918=CARTESIAN_POINT('Ctrl Pts',(56.2833501191642,30.5272599343804,13.1642903520899));
#47919=CARTESIAN_POINT('Ctrl Pts',(56.2608617180058,30.5457380609807,13.1661880040148));
#47920=CARTESIAN_POINT('Ctrl Pts',(56.2553271069651,30.5502362024321,13.1666510345344));
#47921=CARTESIAN_POINT('Ctrl Pts',(56.2461853697867,30.5575848999437,13.1674091235518));
#47922=CARTESIAN_POINT('Ctrl Pts',(56.242592359016,30.5604527954277,13.1677053884831));
#47923=CARTESIAN_POINT('Ctrl Pts',(56.235533522762,30.5660472284429,13.1682840760909));
#47924=CARTESIAN_POINT('Ctrl Pts',(56.2320685283388,30.5687747287695,13.1685665637616));
#47925=CARTESIAN_POINT('Ctrl Pts',(56.2235091673775,30.5754664536779,13.1692605834954));
#47926=CARTESIAN_POINT('Ctrl Pts',(56.2184044923577,30.5794175271527,13.1696711977433));
#47927=CARTESIAN_POINT('Ctrl Pts',(56.2007786930571,30.5929237794877,13.1710780737985));
#47928=CARTESIAN_POINT('Ctrl Pts',(56.1881632600141,30.6023556848185,13.172066193636));
#47929=CARTESIAN_POINT('Ctrl Pts',(56.0758778956707,30.6842502598361,13.1807093355327));
#47930=CARTESIAN_POINT('Ctrl Pts',(55.9697900866757,30.7474918441199,13.1878423757985));
#47931=CARTESIAN_POINT('Ctrl Pts',(55.7655791709926,30.844863256513,13.2009794451731));
#47932=CARTESIAN_POINT('Ctrl Pts',(55.6693393437374,30.8819178322031,13.2069567120401));
#47933=CARTESIAN_POINT('Ctrl Pts',(55.5368054123103,30.9214882141226,13.2152711386408));
#47934=CARTESIAN_POINT('Ctrl Pts',(55.5026740937519,30.9306982029106,13.2174183599116));
#47935=CARTESIAN_POINT('Ctrl Pts',(55.4436063777527,30.9449645767648,13.2211570884229));
#47936=CARTESIAN_POINT('Ctrl Pts',(55.4187843442119,30.9504597934128,13.2227349734993));
#47937=CARTESIAN_POINT('Ctrl Pts',(55.3833038700587,30.9576061315152,13.2250029049775));
#47938=CARTESIAN_POINT('Ctrl Pts',(55.3727259374319,30.9596476701852,13.2256806177267));
#47939=CARTESIAN_POINT('Ctrl Pts',(55.3544081283186,30.9630293260337,13.2268571351839));
#47940=CARTESIAN_POINT('Ctrl Pts',(55.346675843672,30.964409609232,13.2273546615312));
#47941=CARTESIAN_POINT('Ctrl Pts',(55.3318163495819,30.9669716989779,13.2283125837807));
#47942=CARTESIAN_POINT('Ctrl Pts',(55.3246904637155,30.9681605257084,13.2287727498787));
#47943=CARTESIAN_POINT('Ctrl Pts',(55.3078884230617,30.9708699146411,13.2298597078878));
#47944=CARTESIAN_POINT('Ctrl Pts',(55.2982072844609,30.9723579572064,13.2304875116423));
#47945=CARTESIAN_POINT('Ctrl Pts',(55.2644349807819,30.9772946102586,13.2326830646434));
#47946=CARTESIAN_POINT('Ctrl Pts',(55.2402927672055,30.9803734835933,13.2342622963263));
#47947=CARTESIAN_POINT('Ctrl Pts',(55.0855628378242,30.9972353825786,13.2444499901521));
#47948=CARTESIAN_POINT('Ctrl Pts',(54.9539612599652,30.9985343547,13.2534475445453));
#47949=CARTESIAN_POINT('Ctrl Pts',(54.7233996596851,30.9780193477641,13.2695567074557));
#47950=CARTESIAN_POINT('Ctrl Pts',(54.624398071639,30.9616302087489,13.2765791256516));
#47951=CARTESIAN_POINT('Ctrl Pts',(54.4998630576276,30.9312362421884,13.2852907805544));
#47952=CARTESIAN_POINT('Ctrl Pts',(54.4728230626734,30.9240309306456,13.2871741358083));
#47953=CARTESIAN_POINT('Ctrl Pts',(54.428425701111,30.9111940939926,13.2902434533576));
#47954=CARTESIAN_POINT('Ctrl Pts',(54.4109786290441,30.9058892740607,13.2914436637295));
#47955=CARTESIAN_POINT('Ctrl Pts',(54.3872762970908,30.8983259392221,13.2930637527363));
#47956=CARTESIAN_POINT('Ctrl Pts',(54.380956583815,30.8962744947742,13.2934946945814));
#47957=CARTESIAN_POINT('Ctrl Pts',(54.3703812385538,30.8927831251972,13.294213978301));
#47958=CARTESIAN_POINT('Ctrl Pts',(54.3661200539562,30.8913603461469,13.2945032979451));
#47959=CARTESIAN_POINT('Ctrl Pts',(54.3580545723318,30.8886370200833,13.2950499089708));
#47960=CARTESIAN_POINT('Ctrl Pts',(54.3542493509525,30.8873393509604,13.2953073704552));
#47961=CARTESIAN_POINT('Ctrl Pts',(54.3442946947251,30.8839109506206,13.2959798537793));
#47962=CARTESIAN_POINT('Ctrl Pts',(54.3381516571582,30.8817615925326,13.2963937935686));
#47963=CARTESIAN_POINT('Ctrl Pts',(54.3168780481539,30.8742012082629,13.2978239928542));
#47964=CARTESIAN_POINT('Ctrl Pts',(54.3018019589459,30.8686372852733,13.2988317452235));
#47965=CARTESIAN_POINT('Ctrl Pts',(54.1860727634522,30.8243305020476,13.3065347285346));
#47966=CARTESIAN_POINT('Ctrl Pts',(54.0886308192715,30.7776590132154,13.3128333253503));
#47967=CARTESIAN_POINT('Ctrl Pts',(53.8979549179244,30.666509646274,13.3256631051083));
#47968=CARTESIAN_POINT('Ctrl Pts',(53.8054813490004,30.6015246241497,13.3321739387852));
#47969=CARTESIAN_POINT('Ctrl Pts',(53.6897006446243,30.5045278471628,13.3412259813916));
#47970=CARTESIAN_POINT('Ctrl Pts',(53.6611149841582,30.4791467457248,13.3435419171897));
#47971=CARTESIAN_POINT('Ctrl Pts',(53.6136199231396,30.4344706888291,13.3475476030747));
#47972=CARTESIAN_POINT('Ctrl Pts',(53.5943406426183,30.4155838151899,13.3492208891125));
#47973=CARTESIAN_POINT('Ctrl Pts',(53.5677297540622,30.388434795049,13.3516019358723));
#47974=CARTESIAN_POINT('Ctrl Pts',(53.5600739781826,30.3804934919873,13.352295586868));
#47975=CARTESIAN_POINT('Ctrl Pts',(53.5470480865,30.3667555487657,13.353490986667));
#47976=CARTESIAN_POINT('Ctrl Pts',(53.5416457713439,30.3609896891154,13.353991343401));
#47977=CARTESIAN_POINT('Ctrl Pts',(53.5314056771144,30.3499295200854,13.3549486475392));
#47978=CARTESIAN_POINT('Ctrl Pts',(53.5265619050445,30.3446409084019,13.3554053302285));
#47979=CARTESIAN_POINT('Ctrl Pts',(53.5141061253413,30.3308931044141,13.356589806811));
#47980=CARTESIAN_POINT('Ctrl Pts',(53.5065378815352,30.3223947799361,13.3573194112538));
#47981=CARTESIAN_POINT('Ctrl Pts',(53.4851177927023,30.2979238985391,13.3594132423356));
#47982=CARTESIAN_POINT('Ctrl Pts',(53.4714469490872,30.2817956398368,13.3607847949351));
#47983=CARTESIAN_POINT('Ctrl Pts',(53.3550465780414,30.1399609332491,13.3727778801633));
#47984=CARTESIAN_POINT('Ctrl Pts',(53.2677810735677,30.0023872863944,13.384025521532));
#47985=CARTESIAN_POINT('Ctrl Pts',(53.1649050598222,29.7857873114781,13.4007345969455));
#47986=CARTESIAN_POINT('Ctrl Pts',(53.1357586664016,29.7138913589845,13.4061221151343));
#47987=CARTESIAN_POINT('Ctrl Pts',(53.103096413825,29.6175519029457,13.4130046660651));
#47988=CARTESIAN_POINT('Ctrl Pts',(53.0957414126947,29.5944854164993,13.4146277919164));
#47989=CARTESIAN_POINT('Ctrl Pts',(53.0841203307741,29.5556082578695,13.4173159677041));
#47990=CARTESIAN_POINT('Ctrl Pts',(53.0796258550381,29.5398690839979,13.4183913715069));
#47991=CARTESIAN_POINT('Ctrl Pts',(53.0736521685307,29.5179306490023,13.419870833062));
#47992=CARTESIAN_POINT('Ctrl Pts',(53.072008303696,29.5117774385784,13.4202836667103));
#47993=CARTESIAN_POINT('Ctrl Pts',(53.0692692431778,29.5013242407116,13.4209812808956));
#47994=CARTESIAN_POINT('Ctrl Pts',(53.0681588808038,29.4970283103165,13.4212669159244));
#47995=CARTESIAN_POINT('Ctrl Pts',(53.0660565420174,29.4887809941834,13.4218131973759));
#47996=CARTESIAN_POINT('Ctrl Pts',(53.06506232812,29.4848302441166,13.4220739757925));
#47997=CARTESIAN_POINT('Ctrl Pts',(53.0627123030393,29.4753694767777,13.4226963422761));
#47998=CARTESIAN_POINT('Ctrl Pts',(53.0613678764538,29.4698566288474,13.4230572870091));
#47999=CARTESIAN_POINT('Ctrl Pts',(53.0566159294787,29.4500035193902,13.4243512311863));
#48000=CARTESIAN_POINT('Ctrl Pts',(53.0533437522474,29.4356309171549,13.4252769140447));
#48001=CARTESIAN_POINT('Ctrl Pts',(53.0490256293916,29.4156430622009,13.4265506113638));
#48002=CARTESIAN_POINT('Ctrl Pts',(53.0478442633022,29.4100586740838,13.4269049972294));
#48003=CARTESIAN_POINT('Ctrl Pts',(53.04668699692,29.404469868468,13.4272582639285));
#48004=CARTESIAN_POINT('Origin',(55.,29.,3.45145488139523));
#48005=CARTESIAN_POINT('',(53.0466870452705,29.4044701019679,14.3843322575863));
#48006=CARTESIAN_POINT('',(53.0466869970967,29.4044698693216,14.2242573078582));
#48007=CARTESIAN_POINT('',(53.0466869980082,29.4044698737233,3.45145488139523));
#48008=CARTESIAN_POINT('',(53.0052501563995,28.9992103260818,13.6096063772323));
#48009=CARTESIAN_POINT('Ctrl Pts',(53.0466870452705,29.4044701019679,14.3843322575863));
#48010=CARTESIAN_POINT('Ctrl Pts',(53.0651942708541,29.4938472977425,14.3789669817368));
#48011=CARTESIAN_POINT('Ctrl Pts',(53.089821908192,29.5818877886488,14.3735004590224));
#48012=CARTESIAN_POINT('Ctrl Pts',(53.1256881001794,29.6828107362223,14.3668534278733));
#48013=CARTESIAN_POINT('Ctrl Pts',(53.1311373838443,29.6975873416164,14.3658705425979));
#48014=CARTESIAN_POINT('Ctrl Pts',(53.1402787406042,29.7214994452985,14.3642634905551));
#48015=CARTESIAN_POINT('Ctrl Pts',(53.1438645997717,29.7306750185046,14.3636428411623));
#48016=CARTESIAN_POINT('Ctrl Pts',(53.1503800876598,29.7469894802121,14.3625320028294));
#48017=CARTESIAN_POINT('Ctrl Pts',(53.1532834702555,29.7541386873287,14.3620426990456));
#48018=CARTESIAN_POINT('Ctrl Pts',(53.1595037545394,29.769204002796,14.3610061832558));
#48019=CARTESIAN_POINT('Ctrl Pts',(53.1628304062841,29.7771158907305,14.3604586512175));
#48020=CARTESIAN_POINT('Ctrl Pts',(53.1718166940001,29.7981080659995,14.3589972964518));
#48021=CARTESIAN_POINT('Ctrl Pts',(53.1775655484712,29.811149393054,14.3580804741788));
#48022=CARTESIAN_POINT('Ctrl Pts',(53.2061400163677,29.8741333785546,14.3536080789534));
#48023=CARTESIAN_POINT('Ctrl Pts',(53.2308796009079,29.923176502266,14.3499877399848));
#48024=CARTESIAN_POINT('Ctrl Pts',(53.3579669551592,30.1511945817571,14.332476096662));
#48025=CARTESIAN_POINT('Ctrl Pts',(53.4856042391137,30.314573690023,14.3177007073119));
#48026=CARTESIAN_POINT('Ctrl Pts',(53.6583134307999,30.4764287406221,14.3017586179392));
#48027=CARTESIAN_POINT('Ctrl Pts',(53.6811305092218,30.4968460794232,14.2997221901765));
#48028=CARTESIAN_POINT('Ctrl Pts',(53.7107698363668,30.5221639560008,14.297173626867));
#48029=CARTESIAN_POINT('Ctrl Pts',(53.717163959834,30.5275566188298,14.2966293847403));
#48030=CARTESIAN_POINT('Ctrl Pts',(53.7273345525257,30.5360253709058,14.2957727179552));
#48031=CARTESIAN_POINT('Ctrl Pts',(53.7310886056742,30.5391280505007,14.2954584358674));
#48032=CARTESIAN_POINT('Ctrl Pts',(53.738208769231,30.5449690224707,14.2948660328008));
#48033=CARTESIAN_POINT('Ctrl Pts',(53.741572414137,30.5477100509863,14.2945877242164));
#48034=CARTESIAN_POINT('Ctrl Pts',(53.7494405794122,30.5540791969193,14.2939402678272));
#48035=CARTESIAN_POINT('Ctrl Pts',(53.7539519628697,30.5576987211543,14.2935717310558));
#48036=CARTESIAN_POINT('Ctrl Pts',(53.7685545380172,30.5693104666846,14.2923872734525));
#48037=CARTESIAN_POINT('Ctrl Pts',(53.7787076100021,30.5772248365823,14.2915766322095));
#48038=CARTESIAN_POINT('Ctrl Pts',(53.8029823476145,30.5957721463632,14.2896669795025));
#48039=CARTESIAN_POINT('Ctrl Pts',(53.8171703356499,30.6063169157242,14.288573298804));
#48040=CARTESIAN_POINT('Ctrl Pts',(53.8696930583156,30.6442794398413,14.2845985610984));
#48041=CARTESIAN_POINT('Ctrl Pts',(53.9088580425179,30.6705264095227,14.2817765646807));
#48042=CARTESIAN_POINT('Ctrl Pts',(54.0859502996677,30.7803190623223,14.2694604641199));
#48043=CARTESIAN_POINT('Ctrl Pts',(54.2327738565179,30.8483477444895,14.2603476341313));
#48044=CARTESIAN_POINT('Ctrl Pts',(54.4400526960422,30.9153828242194,14.2472893587488));
#48045=CARTESIAN_POINT('Ctrl Pts',(54.4946295599682,30.9305004995872,14.2438403196924));
#48046=CARTESIAN_POINT('Ctrl Pts',(54.5642270961294,30.9466252096432,14.2393927256583));
#48047=CARTESIAN_POINT('Ctrl Pts',(54.5787188679156,30.9498127909308,14.2384640493554));
#48048=CARTESIAN_POINT('Ctrl Pts',(54.6018560005165,30.9546320094794,14.2369766658718));
#48049=CARTESIAN_POINT('Ctrl Pts',(54.6104791058872,30.9563686784118,14.2364212942788));
#48050=CARTESIAN_POINT('Ctrl Pts',(54.6266562736075,30.9595155201606,14.2353773536211));
#48051=CARTESIAN_POINT('Ctrl Pts',(54.6342075693632,30.9609391899764,14.2348892218689));
#48052=CARTESIAN_POINT('Ctrl Pts',(54.6511280164718,30.9640281194881,14.2337934991875));
#48053=CARTESIAN_POINT('Ctrl Pts',(54.6605011880695,30.9656700299328,14.2331851834562));
#48054=CARTESIAN_POINT('Ctrl Pts',(54.6882609692822,30.9703282723082,14.2313794558799));
#48055=CARTESIAN_POINT('Ctrl Pts',(54.70667808594,30.9731540588176,14.2301761004223));
#48056=CARTESIAN_POINT('Ctrl Pts',(54.8539410364848,30.9936417322771,14.220508702191));
#48057=CARTESIAN_POINT('Ctrl Pts',(54.9841705405366,30.9989193876083,14.2116517668491));
#48058=CARTESIAN_POINT('Ctrl Pts',(55.2573569930519,30.9832860576243,14.1926440728428));
#48059=CARTESIAN_POINT('Ctrl Pts',(55.3994516440834,30.9596173436848,14.1825093673263));
#48060=CARTESIAN_POINT('Ctrl Pts',(55.5517191505958,30.9169880287433,14.1720568930949));
#48061=CARTESIAN_POINT('Ctrl Pts',(55.5656169527115,30.9129335103937,14.1711070739291));
#48062=CARTESIAN_POINT('Ctrl Pts',(55.5848606013737,30.9070913397125,14.169798921699));
#48063=CARTESIAN_POINT('Ctrl Pts',(55.5902444712192,30.9054319109035,14.1694337027521));
#48064=CARTESIAN_POINT('Ctrl Pts',(55.5994991604183,30.9025364198383,14.168807313624));
#48065=CARTESIAN_POINT('Ctrl Pts',(55.6033733308077,30.9013113097393,14.1685455230875));
#48066=CARTESIAN_POINT('Ctrl Pts',(55.6114793866004,30.8987206995965,14.1679987041204));
#48067=CARTESIAN_POINT('Ctrl Pts',(55.6157104849498,30.8973528756005,14.1677138212604));
#48068=CARTESIAN_POINT('Ctrl Pts',(55.6260373096143,30.8939762516493,14.1670197493159));
#48069=CARTESIAN_POINT('Ctrl Pts',(55.6321280509547,30.8919521359551,14.1666114449781));
#48070=CARTESIAN_POINT('Ctrl Pts',(55.654021322371,30.884558891136,14.1651472453134));
#48071=CARTESIAN_POINT('Ctrl Pts',(55.6697666015426,30.8790207147876,14.164100719619));
#48072=CARTESIAN_POINT('Ctrl Pts',(55.7087729369854,30.8647481716934,14.1615200318356));
#48073=CARTESIAN_POINT('Ctrl Pts',(55.7319443247293,30.8557754283044,14.15999763892));
#48074=CARTESIAN_POINT('Ctrl Pts',(55.8299279452719,30.8157119594405,14.1535813619349));
#48075=CARTESIAN_POINT('Ctrl Pts',(55.9029815175782,30.7805102437794,14.1488492733601));
#48076=CARTESIAN_POINT('Ctrl Pts',(56.1108091448868,30.6642749660863,14.1350039842979));
#48077=CARTESIAN_POINT('Ctrl Pts',(56.2383666573575,30.5716711063742,14.125953151526));
#48078=CARTESIAN_POINT('Ctrl Pts',(56.3712962370987,30.4488429112459,14.1148004757563));
#48079=CARTESIAN_POINT('Ctrl Pts',(56.3885619678539,30.4323039960369,14.1133149742629));
#48080=CARTESIAN_POINT('Ctrl Pts',(56.4122406139927,30.4087915245124,14.1112229612347));
#48081=CARTESIAN_POINT('Ctrl Pts',(56.4189078774842,30.4020761540111,14.1106276554891));
#48082=CARTESIAN_POINT('Ctrl Pts',(56.4310237459086,30.3896979354768,14.1095341736236));
#48083=CARTESIAN_POINT('Ctrl Pts',(56.4364871788882,30.3840498167529,14.1090366547162));
#48084=CARTESIAN_POINT('Ctrl Pts',(56.4474848064315,30.372545162153,14.1080260519428));
#48085=CARTESIAN_POINT('Ctrl Pts',(56.4530171694596,30.3666870853055,14.1075129032463));
#48086=CARTESIAN_POINT('Ctrl Pts',(56.4665795690965,30.3521507761058,14.1062430040035));
#48087=CARTESIAN_POINT('Ctrl Pts',(56.4745681483055,30.3434344494269,14.1054845206256));
#48088=CARTESIAN_POINT('Ctrl Pts',(56.5040737073018,30.3106607382167,14.1026432068695));
#48089=CARTESIAN_POINT('Ctrl Pts',(56.5250823153939,30.2861543525517,14.1005395553245));
#48090=CARTESIAN_POINT('Ctrl Pts',(56.5761712050679,30.2235470815933,14.0952134833179));
#48091=CARTESIAN_POINT('Ctrl Pts',(56.6054713863942,30.184839286137,14.0919628863608));
#48092=CARTESIAN_POINT('Ctrl Pts',(56.6909706981619,30.0628865969941,14.0818539904205));
#48093=CARTESIAN_POINT('Ctrl Pts',(56.7423178351698,29.9764401368831,14.0748600572816));
#48094=CARTESIAN_POINT('Ctrl Pts',(56.8326119972608,29.7944332696938,14.0607016244154));
#48095=CARTESIAN_POINT('Ctrl Pts',(56.8711091598477,29.698960423908,14.0535589849105));
#48096=CARTESIAN_POINT('Ctrl Pts',(56.9069235399736,29.5856012709779,14.0456828312359));
#48097=CARTESIAN_POINT('Ctrl Pts',(56.9115833245341,29.5702065138135,14.0446258691389));
#48098=CARTESIAN_POINT('Ctrl Pts',(56.9178671854335,29.5485028785489,14.0431550855166));
#48099=CARTESIAN_POINT('Ctrl Pts',(56.9196472053074,29.5422403145689,14.0427329388972));
#48100=CARTESIAN_POINT('Ctrl Pts',(56.9224769082443,29.5320961065047,14.0420528931355));
#48101=CARTESIAN_POINT('Ctrl Pts',(56.9235455541656,29.5282198699761,14.0417939226578));
#48102=CARTESIAN_POINT('Ctrl Pts',(56.9257832120055,29.5200064995344,14.0412470983112));
#48103=CARTESIAN_POINT('Ctrl Pts',(56.9269493089306,29.5156685958802,14.0409594185336));
#48104=CARTESIAN_POINT('Ctrl Pts',(56.9298032364856,29.5049070625014,14.0402484436156));
#48105=CARTESIAN_POINT('Ctrl Pts',(56.9314736750158,29.4984788049915,14.0398261360066));
#48106=CARTESIAN_POINT('Ctrl Pts',(56.9376052688793,29.4743892912769,14.0382520609044));
#48107=CARTESIAN_POINT('Ctrl Pts',(56.9418567036914,29.4566749117992,14.0371116100608));
#48108=CARTESIAN_POINT('Ctrl Pts',(56.9520129039967,29.4116477696508,14.0342500877002));
#48109=CARTESIAN_POINT('Ctrl Pts',(56.957587712514,29.3842639307407,14.0325443456957));
#48110=CARTESIAN_POINT('Ctrl Pts',(56.9804611718324,29.2584376636158,14.0248269580536));
#48111=CARTESIAN_POINT('Ctrl Pts',(56.9909225705665,29.1588925964334,14.019051067913));
#48112=CARTESIAN_POINT('Ctrl Pts',(56.9977696671333,28.9274055886509,14.0056013002485));
#48113=CARTESIAN_POINT('Ctrl Pts',(56.9886291764605,28.7957891929518,13.9979230552837));
#48114=CARTESIAN_POINT('Ctrl Pts',(56.9625220767595,28.6420521826928,13.9883231958293));
#48115=CARTESIAN_POINT('Ctrl Pts',(56.958010266346,28.618142357595,13.986812694045));
#48116=CARTESIAN_POINT('Ctrl Pts',(56.9510706069042,28.5847326540622,13.9846749048522));
#48117=CARTESIAN_POINT('Ctrl Pts',(56.9490082401293,28.5751584340065,13.9840591369458));
#48118=CARTESIAN_POINT('Ctrl Pts',(56.9453022650103,28.5585491549572,13.9829852732039));
#48119=CARTESIAN_POINT('Ctrl Pts',(56.9436907758777,28.5515070609331,13.9825282034758));
#48120=CARTESIAN_POINT('Ctrl Pts',(56.9402473566488,28.536826755339,13.9815716081935));
#48121=CARTESIAN_POINT('Ctrl Pts',(56.9384084954687,28.5291903130069,13.9810718687408));
#48122=CARTESIAN_POINT('Ctrl Pts',(56.9339404194312,28.5111052241157,13.9798831912338));
#48123=CARTESIAN_POINT('Ctrl Pts',(56.9312715777554,28.5006667112456,13.9791929961317));
#48124=CARTESIAN_POINT('Ctrl Pts',(56.9220201957624,28.465666265351,13.9768646592819));
#48125=CARTESIAN_POINT('Ctrl Pts',(56.9150528139011,28.4412095254745,13.9752142498988));
#48126=CARTESIAN_POINT('Ctrl Pts',(56.8972836167096,28.3830779824912,13.9712332257385));
#48127=CARTESIAN_POINT('Ctrl Pts',(56.8860503800644,28.3495450753956,13.9688893963111));
#48128=CARTESIAN_POINT('Ctrl Pts',(56.8386151878298,28.2195256923073,13.9596138727579));
#48129=CARTESIAN_POINT('Ctrl Pts',(56.7958536810452,28.1256138335141,13.9524923847739));
#48130=CARTESIAN_POINT('Ctrl Pts',(56.6864896171579,27.9276452527475,13.9367378893781));
#48131=CARTESIAN_POINT('Ctrl Pts',(56.6170847408471,27.8255919943081,13.9281112117561));
#48132=CARTESIAN_POINT('Ctrl Pts',(56.5286799635785,27.7184332618856,13.9189118166904));
#48133=CARTESIAN_POINT('Ctrl Pts',(56.518510803645,27.7064000960918,13.9178768736967));
#48134=CARTESIAN_POINT('Ctrl Pts',(56.5039748214759,27.689607321279,13.9164313571804));
#48135=CARTESIAN_POINT('Ctrl Pts',(56.4997261206788,27.6847468677807,13.9160128256075));
#48136=CARTESIAN_POINT('Ctrl Pts',(56.4925355464219,27.6766010991317,13.9153112783626));
#48137=CARTESIAN_POINT('Ctrl Pts',(56.4896062637499,27.673304786914,13.9150273535929));
#48138=CARTESIAN_POINT('Ctrl Pts',(56.4836010006278,27.6665920481546,13.9144491389884));
#48139=CARTESIAN_POINT('Ctrl Pts',(56.4805241053374,27.6631765001843,13.9141549203355));
#48140=CARTESIAN_POINT('Ctrl Pts',(56.4726441312357,27.6544898073523,13.9134065112992));
#48141=CARTESIAN_POINT('Ctrl Pts',(56.4678244947929,27.6492336723389,13.9129535428838));
#48142=CARTESIAN_POINT('Ctrl Pts',(56.4480440695992,27.6278926889008,13.9111133418582));
#48143=CARTESIAN_POINT('Ctrl Pts',(56.4328456155094,27.6120289496164,13.9097429641106));
#48144=CARTESIAN_POINT('Ctrl Pts',(56.3919524378469,27.5707335288503,13.9061585261536));
#48145=CARTESIAN_POINT('Ctrl Pts',(56.3658223821017,27.5457428828289,13.9039714492178));
#48146=CARTESIAN_POINT('Ctrl Pts',(56.2038638338668,27.3990651491109,13.8909187544325));
#48147=CARTESIAN_POINT('Ctrl Pts',(56.0525544717185,27.2957648713558,13.8807073310655));
#48148=CARTESIAN_POINT('Ctrl Pts',(55.8421425156038,27.1909671641845,13.8665783800287));
#48149=CARTESIAN_POINT('Ctrl Pts',(55.7940697417436,27.169356305483,13.8633616022349));
#48150=CARTESIAN_POINT('Ctrl Pts',(55.7316148496795,27.1442031919948,13.8591678784783));
#48151=CARTESIAN_POINT('Ctrl Pts',(55.7179692857853,27.1388814740622,13.8582507974157));
#48152=CARTESIAN_POINT('Ctrl Pts',(55.696155441944,27.1306497590218,13.8567829176943));
#48153=CARTESIAN_POINT('Ctrl Pts',(55.6880244855881,27.1276418541832,13.856235375724));
#48154=CARTESIAN_POINT('Ctrl Pts',(55.6733587239375,27.1223249419516,13.8552469480946));
#48155=CARTESIAN_POINT('Ctrl Pts',(55.666830967928,27.1199967944287,13.8548067035874));
#48156=CARTESIAN_POINT('Ctrl Pts',(55.6514822166297,27.1146126041592,13.8537708004094));
#48157=CARTESIAN_POINT('Ctrl Pts',(55.642651696652,27.1115843934909,13.8531742374692));
#48158=CARTESIAN_POINT('Ctrl Pts',(55.6169676863278,27.1029777038107,13.8514372466277));
#48159=CARTESIAN_POINT('Ctrl Pts',(55.6000609227542,27.0975622024356,13.8502915367412));
#48160=CARTESIAN_POINT('Ctrl Pts',(55.444625152373,27.0500517563864,13.8397342686215));
#48161=CARTESIAN_POINT('Ctrl Pts',(55.3019966260477,27.0229384485427,13.8298256084381));
#48162=CARTESIAN_POINT('Ctrl Pts',(55.0291351005587,27.0012962381262,13.8107699328795));
#48163=CARTESIAN_POINT('Ctrl Pts',(54.8998543217901,27.0035927520551,13.8017145598568));
#48164=CARTESIAN_POINT('Ctrl Pts',(54.7563237048571,27.0201291054974,13.7921506511831));
#48165=CARTESIAN_POINT('Ctrl Pts',(54.7409755193925,27.0220785533364,13.7911345961937));
#48166=CARTESIAN_POINT('Ctrl Pts',(54.7199326459483,27.025000463303,13.7897520890081));
#48167=CARTESIAN_POINT('Ctrl Pts',(54.7142176621014,27.0258193218226,13.7893776877286));
#48168=CARTESIAN_POINT('Ctrl Pts',(54.7044500361928,27.0272621580412,13.7887397132935));
#48169=CARTESIAN_POINT('Ctrl Pts',(54.700395655348,27.0278738347646,13.7884754685129));
#48170=CARTESIAN_POINT('Ctrl Pts',(54.6919788284793,27.0291702205632,13.787928121352));
#48171=CARTESIAN_POINT('Ctrl Pts',(54.6876167445176,27.0298569179614,13.787645142103));
#48172=CARTESIAN_POINT('Ctrl Pts',(54.677080001698,27.0315515300813,13.7869631880806));
#48173=CARTESIAN_POINT('Ctrl Pts',(54.6709076673694,27.0325740310885,13.78656502541));
#48174=CARTESIAN_POINT('Ctrl Pts',(54.6493148870433,27.0362555234082,13.7851764295812));
#48175=CARTESIAN_POINT('Ctrl Pts',(54.6339205443326,27.0390669859573,13.7841941392111));
#48176=CARTESIAN_POINT('Ctrl Pts',(54.5393207514004,27.0574966126828,13.7781964887587));
#48177=CARTESIAN_POINT('Ctrl Pts',(54.4610819511533,27.0777317899205,13.7734019205983));
#48178=CARTESIAN_POINT('Ctrl Pts',(54.2899824146538,27.1332567081432,13.7628691405398));
#48179=CARTESIAN_POINT('Ctrl Pts',(54.1981001170324,27.1708438163722,13.7571753820321));
#48180=CARTESIAN_POINT('Ctrl Pts',(54.0244365034281,27.2574966584921,13.7457803729509));
#48181=CARTESIAN_POINT('Ctrl Pts',(53.9426256203644,27.3058931363041,13.7401039602952));
#48182=CARTESIAN_POINT('Ctrl Pts',(53.851878610867,27.3687172585093,13.7332514870052));
#48183=CARTESIAN_POINT('Ctrl Pts',(53.8392827210759,27.3776555592461,13.732287294808));
#48184=CARTESIAN_POINT('Ctrl Pts',(53.8188989617653,27.392479190798,13.7307047886843));
#48185=CARTESIAN_POINT('Ctrl Pts',(53.8110481068422,27.3982771135814,13.7300898140024));
#48186=CARTESIAN_POINT('Ctrl Pts',(53.7972281024202,27.4086408960748,13.7289973695291));
#48187=CARTESIAN_POINT('Ctrl Pts',(53.7912415726967,27.4131833448164,13.7285208139995));
#48188=CARTESIAN_POINT('Ctrl Pts',(53.7850295944423,27.4179524101621,13.7280227860304));
#48189=CARTESIAN_POINT('Ctrl Pts',(53.7847783156711,27.4181454172935,13.7280026344184));
#48190=CARTESIAN_POINT('Ctrl Pts',(53.7843290172851,27.4184906934568,13.7279665915702));
#48191=CARTESIAN_POINT('Ctrl Pts',(53.7841309802507,27.418642939842,13.7279507012242));
#48192=CARTESIAN_POINT('Ctrl Pts',(53.7837751966178,27.4189165645815,13.7279221466534));
#48193=CARTESIAN_POINT('Ctrl Pts',(53.7836174395383,27.4190379293856,13.7279094829599));
#48194=CARTESIAN_POINT('Ctrl Pts',(53.7833329639721,27.4192568483408,13.7278866428393));
#48195=CARTESIAN_POINT('Ctrl Pts',(53.7832062390315,27.4193543941343,13.7278764667405));
#48196=CARTESIAN_POINT('Ctrl Pts',(53.7829770460267,27.4195308580267,13.7278580595973));
#48197=CARTESIAN_POINT('Ctrl Pts',(53.7828745739527,27.419609770817,13.7278498287644));
#48198=CARTESIAN_POINT('Ctrl Pts',(53.7826888056261,27.4197528580603,13.7278349055229));
#48199=CARTESIAN_POINT('Ctrl Pts',(53.7826055066662,27.4198170292156,13.7278282132389));
#48200=CARTESIAN_POINT('Ctrl Pts',(53.7823839664693,27.4199877254125,13.7278104128041));
#48201=CARTESIAN_POINT('Ctrl Pts',(53.7822457341113,27.4200942620307,13.7277993041961));
#48202=CARTESIAN_POINT('Ctrl Pts',(53.7819749860418,27.4203029860524,13.7277775427791));
#48203=CARTESIAN_POINT('Ctrl Pts',(53.7818424692788,27.420405171935,13.7277668900339));
#48204=CARTESIAN_POINT('Ctrl Pts',(53.7815827204365,27.4206055207184,13.7277460060535));
#48205=CARTESIAN_POINT('Ctrl Pts',(53.7814554872659,27.4207036823922,13.7277357748621));
#48206=CARTESIAN_POINT('Ctrl Pts',(53.7812059146623,27.4208962782861,13.7277157029389));
#48207=CARTESIAN_POINT('Ctrl Pts',(53.7810835744424,27.4209907112716,13.7277058622609));
#48208=CARTESIAN_POINT('Ctrl Pts',(53.7808434341293,27.4211761173116,13.7276865432656));
#48209=CARTESIAN_POINT('Ctrl Pts',(53.7807256331334,27.4212670894179,13.7276770649804));
#48210=CARTESIAN_POINT('Ctrl Pts',(53.7804942496461,27.4214458172252,13.7276584452005));
#48211=CARTESIAN_POINT('Ctrl Pts',(53.780380666441,27.4215335720038,13.7276493037423));
#48212=CARTESIAN_POINT('Ctrl Pts',(53.7801574257056,27.4217060870522,13.727631334325));
#48213=CARTESIAN_POINT('Ctrl Pts',(53.7800477675759,27.4217908464616,13.7276225064019));
#48214=CARTESIAN_POINT('Ctrl Pts',(53.7798321099569,27.4219575732693,13.7276051428055));
#48215=CARTESIAN_POINT('Ctrl Pts',(53.7797261098431,27.422039539958,13.7275966071578));
#48216=CARTESIAN_POINT('Ctrl Pts',(53.7795175236842,27.4222008669263,13.7275798086416));
#48217=CARTESIAN_POINT('Ctrl Pts',(53.7794149371728,27.4222802264898,13.7275715458042));
#48218=CARTESIAN_POINT('Ctrl Pts',(53.779212954302,27.4224365092483,13.7275552750751));
#48219=CARTESIAN_POINT('Ctrl Pts',(53.7791135574443,27.4225134318541,13.7275472672055));
#48220=CARTESIAN_POINT('Ctrl Pts',(53.7715419549009,27.4283741919388,13.7269371910812));
#48221=CARTESIAN_POINT('Ctrl Pts',(53.7641110412985,27.4342109574254,13.726333042846));
#48222=CARTESIAN_POINT('Ctrl Pts',(53.7486875278689,27.4465038722832,13.7250676024798));
#48223=CARTESIAN_POINT('Ctrl Pts',(53.740702795094,27.4529694040054,13.7244059474242));
#48224=CARTESIAN_POINT('Ctrl Pts',(53.7199595064664,27.4700330098056,13.7226696883172));
#48225=CARTESIAN_POINT('Ctrl Pts',(53.7072827697899,27.4807288617268,13.721591190327));
#48226=CARTESIAN_POINT('Ctrl Pts',(53.6697467192044,27.513209405967,13.7183444825198));
#48227=CARTESIAN_POINT('Ctrl Pts',(53.6452949459689,27.5354543127234,13.7161579741097));
#48228=CARTESIAN_POINT('Ctrl Pts',(53.509867458539,27.6649532553078,13.703631876999));
#48229=CARTESIAN_POINT('Ctrl Pts',(53.4110929036486,27.78418493134,13.6928006453438));
#48230=CARTESIAN_POINT('Ctrl Pts',(53.2813515487948,27.9839689921873,13.6762697187608));
#48231=CARTESIAN_POINT('Ctrl Pts',(53.2401232236364,28.0571805440688,13.6705112347364));
#48232=CARTESIAN_POINT('Ctrl Pts',(53.1990242983824,28.1423134841901,13.6643025314381));
#48233=CARTESIAN_POINT('Ctrl Pts',(53.1944976359306,28.1518839334948,13.6636112806525));
#48234=CARTESIAN_POINT('Ctrl Pts',(53.1877714475442,28.1664026466545,13.6625732420881));
#48235=CARTESIAN_POINT('Ctrl Pts',(53.1855156060419,28.1713243942352,13.6622231835562));
#48236=CARTESIAN_POINT('Ctrl Pts',(53.1815029059856,28.1801741671808,13.6615971028701));
#48237=CARTESIAN_POINT('Ctrl Pts',(53.1797387002814,28.1840987321243,13.661320643007));
#48238=CARTESIAN_POINT('Ctrl Pts',(53.1759057898713,28.192699547708,13.6607173661997));
#48239=CARTESIAN_POINT('Ctrl Pts',(53.1738423640646,28.1973780480107,13.660390868863));
#48240=CARTESIAN_POINT('Ctrl Pts',(53.1680040285132,28.210754646661,13.6594619496137));
#48241=CARTESIAN_POINT('Ctrl Pts',(53.1642730549121,28.2194719359409,13.6588621097547));
#48242=CARTESIAN_POINT('Ctrl Pts',(53.139384588578,28.2787886881304,13.6548156630093));
#48243=CARTESIAN_POINT('Ctrl Pts',(53.120257471211,28.3302204271598,13.651479776779));
#48244=CARTESIAN_POINT('Ctrl Pts',(53.0384007306736,28.5816045754939,13.6356996351405));
#48245=CARTESIAN_POINT('Ctrl Pts',(53.005322673042,28.7897894775224,13.6240476812006));
#48246=CARTESIAN_POINT('Ctrl Pts',(53.0052501195981,28.9993092490871,13.6112224443046));
#48247=CARTESIAN_POINT('Ctrl Pts',(53.0466869980082,29.4044698737233,13.5836009930267));
#48248=CARTESIAN_POINT('Ctrl Pts',(53.0322541803675,29.3347692305246,13.5881317496805));
#48249=CARTESIAN_POINT('Ctrl Pts',(53.0215445661767,29.2642383494607,13.5926625063343));
#48250=CARTESIAN_POINT('Ctrl Pts',(53.0146376983758,29.1932979404689,13.5971932629881));
#48251=CARTESIAN_POINT('Ctrl Pts',(53.0083611430925,29.1288314685893,13.6013105481937));
#48252=CARTESIAN_POINT('Ctrl Pts',(53.0052243749933,29.0640272252075,13.6054278333992));
#48253=CARTESIAN_POINT('Ctrl Pts',(53.0052501577945,28.9992065763071,13.6095451186048));
#48254=CARTESIAN_POINT('Ctrl Pts',(53.04668699692,29.404469868468,13.4272582639285));
#48255=CARTESIAN_POINT('Ctrl Pts',(53.0192622797945,29.2720272299845,13.4356299227296));
#48256=CARTESIAN_POINT('Ctrl Pts',(53.0053718659343,29.1371047871859,13.4433896989916));
#48257=CARTESIAN_POINT('Ctrl Pts',(53.0051306974257,28.8675449949671,13.4590561681005));
#48258=CARTESIAN_POINT('Ctrl Pts',(53.018560705128,28.7336554613748,13.4669297628423));
#48259=CARTESIAN_POINT('Ctrl Pts',(53.0484658429314,28.5867336035516,13.4762350552335));
#48260=CARTESIAN_POINT('Ctrl Pts',(53.0517831798354,28.5713674296968,13.4772161475346));
#48261=CARTESIAN_POINT('Ctrl Pts',(53.0574723139598,28.5464466642276,13.47882084617));
#48262=CARTESIAN_POINT('Ctrl Pts',(53.0597338740793,28.5368674115602,13.4794409523941));
#48263=CARTESIAN_POINT('Ctrl Pts',(53.0638944896611,28.5198098907924,13.4805511858727));
#48264=CARTESIAN_POINT('Ctrl Pts',(53.0657662261264,28.5123251150224,13.4810404316407));
#48265=CARTESIAN_POINT('Ctrl Pts',(53.0698130200128,28.4965324892311,13.4820772087865));
#48266=CARTESIAN_POINT('Ctrl Pts',(53.0719983959439,28.4882274693868,13.4826250625314));
#48267=CARTESIAN_POINT('Ctrl Pts',(53.077958904894,28.4661560585519,13.4840881899181));
#48268=CARTESIAN_POINT('Ctrl Pts',(53.0818282409135,28.4524158418302,13.4850064759762));
#48269=CARTESIAN_POINT('Ctrl Pts',(53.1013726919866,28.3857627910998,13.4894981975022));
#48270=CARTESIAN_POINT('Ctrl Pts',(53.1190902137219,28.3334788812946,13.4931370802024));
#48271=CARTESIAN_POINT('Ctrl Pts',(53.2144773091795,28.0862362499409,13.5109178671461));
#48272=CARTESIAN_POINT('Ctrl Pts',(53.3203980659002,27.9036564916009,13.5259805171546));
#48273=CARTESIAN_POINT('Ctrl Pts',(53.4700172669804,27.7197952147096,13.5418939049268));
#48274=CARTESIAN_POINT('Ctrl Pts',(53.4876654878434,27.6989942525256,13.5437037653887));
#48275=CARTESIAN_POINT('Ctrl Pts',(53.511049054234,27.67255245965,13.5460098610623));
#48276=CARTESIAN_POINT('Ctrl Pts',(53.5163986154985,27.6665762757419,13.5465314356923));
#48277=CARTESIAN_POINT('Ctrl Pts',(53.525003110516,27.6570797785728,13.5473606073883));
#48278=CARTESIAN_POINT('Ctrl Pts',(53.5282348740401,27.6535387267781,13.5476698696107));
#48279=CARTESIAN_POINT('Ctrl Pts',(53.5344311426885,27.6467984224367,13.548258638127));
#48280=CARTESIAN_POINT('Ctrl Pts',(53.537393388527,27.6435972259601,13.5485382981469));
#48281=CARTESIAN_POINT('Ctrl Pts',(53.5444140103239,27.6360600234444,13.5491968940579));
#48282=CARTESIAN_POINT('Ctrl Pts',(53.5484813299337,27.6317323413894,13.549575156563));
#48283=CARTESIAN_POINT('Ctrl Pts',(53.5620244630688,27.6174506201933,13.5508240906368));
#48284=CARTESIAN_POINT('Ctrl Pts',(53.5715840587647,27.6075760861822,13.5516886481452));
#48285=CARTESIAN_POINT('Ctrl Pts',(53.6249367112101,27.5535935064197,13.556426194913));
#48286=CARTESIAN_POINT('Ctrl Pts',(53.6706750253964,27.5114478695419,13.5601670286191));
#48287=CARTESIAN_POINT('Ctrl Pts',(53.8394122124819,27.369956842267,13.5731934873786));
#48288=CARTESIAN_POINT('Ctrl Pts',(53.9721501891463,27.2831621438011,13.582129913193));
#48289=CARTESIAN_POINT('Ctrl Pts',(54.1680317258645,27.186018662626,13.5952015002929));
#48290=CARTESIAN_POINT('Ctrl Pts',(54.223512991292,27.1615859118838,13.5988859279352));
#48291=CARTESIAN_POINT('Ctrl Pts',(54.2941428846151,27.1342500855928,13.6035988951816));
#48292=CARTESIAN_POINT('Ctrl Pts',(54.3083308202188,27.1289439515654,13.6045466458279));
#48293=CARTESIAN_POINT('Ctrl Pts',(54.3309177685287,27.1207886872144,13.6060576764053));
#48294=CARTESIAN_POINT('Ctrl Pts',(54.3392779023909,27.1178330317896,13.6066174342552));
#48295=CARTESIAN_POINT('Ctrl Pts',(54.3541876162418,27.1126734043429,13.6076166906297));
#48296=CARTESIAN_POINT('Ctrl Pts',(54.3607295054006,27.1104475274632,13.6080554605506));
#48297=CARTESIAN_POINT('Ctrl Pts',(54.3758990358787,27.1053738906735,13.6090737192456));
#48298=CARTESIAN_POINT('Ctrl Pts',(54.3845347784986,27.1025510114365,13.6096540116386));
#48299=CARTESIAN_POINT('Ctrl Pts',(54.4089693702275,27.0947481116549,13.611297824848));
#48300=CARTESIAN_POINT('Ctrl Pts',(54.4248111023746,27.089905848361,13.6123657909032));
#48301=CARTESIAN_POINT('Ctrl Pts',(54.5340505284384,27.0579973552965,13.6197471721428));
#48302=CARTESIAN_POINT('Ctrl Pts',(54.6292445131402,27.0375987859738,13.6262743641295));
#48303=CARTESIAN_POINT('Ctrl Pts',(54.8431431712336,27.0078849615611,13.641107386835));
#48304=CARTESIAN_POINT('Ctrl Pts',(54.9619691336942,27.0020815866556,13.6494632201937));
#48305=CARTESIAN_POINT('Ctrl Pts',(55.1068628280687,27.0079411007819,13.6594701311226));
#48306=CARTESIAN_POINT('Ctrl Pts',(55.1331009846328,27.0095220325701,13.6612740240867));
#48307=CARTESIAN_POINT('Ctrl Pts',(55.2022938617599,27.0150654913943,13.6659980517488));
#48308=CARTESIAN_POINT('Ctrl Pts',(55.2451674067815,27.019903695524,13.6688915489856));
#48309=CARTESIAN_POINT('Ctrl Pts',(55.2961918153411,27.0273446895328,13.672269569159));
#48310=CARTESIAN_POINT('Ctrl Pts',(55.3045223271595,27.0286135022251,13.6728189731656));
#48311=CARTESIAN_POINT('Ctrl Pts',(55.3181553356886,27.0307784130053,13.6737143493731));
#48312=CARTESIAN_POINT('Ctrl Pts',(55.3234625934568,27.0316432161366,13.6740619860121));
#48313=CARTESIAN_POINT('Ctrl Pts',(55.3330086123248,27.0332383657885,13.6746855192151));
#48314=CARTESIAN_POINT('Ctrl Pts',(55.3372485439355,27.0339609662236,13.67496183725));
#48315=CARTESIAN_POINT('Ctrl Pts',(55.3465541257768,27.0355778815793,13.6755669026442));
#48316=CARTESIAN_POINT('Ctrl Pts',(55.3516186586799,27.0364780770946,13.6758953165495));
#48317=CARTESIAN_POINT('Ctrl Pts',(55.366150214895,27.0391190155327,13.676835214478));
#48318=CARTESIAN_POINT('Ctrl Pts',(55.3756083509271,27.0409087334696,13.6774440198634));
#48319=CARTESIAN_POINT('Ctrl Pts',(55.4424588569501,27.0540604696559,13.6817285841596));
#48320=CARTESIAN_POINT('Ctrl Pts',(55.4993457718579,27.0678753394493,13.6852781593405));
#48321=CARTESIAN_POINT('Ctrl Pts',(55.6460229120549,27.1104085328351,13.6943691825458));
#48322=CARTESIAN_POINT('Ctrl Pts',(55.7345296956808,27.1430214324681,13.6997974645792));
#48323=CARTESIAN_POINT('Ctrl Pts',(55.9394549824077,27.2354857316176,13.712869705305));
#48324=CARTESIAN_POINT('Ctrl Pts',(56.0529258671097,27.3007569638729,13.7205440317705));
#48325=CARTESIAN_POINT('Ctrl Pts',(56.1720307479055,27.385806650501,13.7296264899733));
#48326=CARTESIAN_POINT('Ctrl Pts',(56.184754887258,27.3951224100962,13.7306106306991));
#48327=CARTESIAN_POINT('Ctrl Pts',(56.2052510559006,27.4105049149619,13.7322193300444));
#48328=CARTESIAN_POINT('Ctrl Pts',(56.2130910667286,27.4164802523002,13.7328403591743));
#48329=CARTESIAN_POINT('Ctrl Pts',(56.2269891012955,27.4272365531428,13.7339516201237));
#48330=CARTESIAN_POINT('Ctrl Pts',(56.2330643162668,27.4319950562254,13.734440964218));
#48331=CARTESIAN_POINT('Ctrl Pts',(56.2458350416459,27.4421180348539,13.735477297017));
#48332=CARTESIAN_POINT('Ctrl Pts',(56.2525238451077,27.4474906821569,13.7360246041238));
#48333=CARTESIAN_POINT('Ctrl Pts',(56.2702192578666,27.4618929567417,13.7374847216203));
#48334=CARTESIAN_POINT('Ctrl Pts',(56.2811640520132,27.4709974185492,13.7384005225917));
#48335=CARTESIAN_POINT('Ctrl Pts',(56.3337016055214,27.5156611000157,13.7428595047627));
#48336=CARTESIAN_POINT('Ctrl Pts',(56.3739132129935,27.5528015091451,13.7464669815222));
#48337=CARTESIAN_POINT('Ctrl Pts',(56.556403682939,27.7358218331011,13.763802763068));
#48338=CARTESIAN_POINT('Ctrl Pts',(56.6772807696819,27.9012527193196,13.7783918612653));
#48339=CARTESIAN_POINT('Ctrl Pts',(56.7861187992832,28.1112451127015,13.794354833922));
#48340=CARTESIAN_POINT('Ctrl Pts',(56.8005066069445,28.1407666972846,13.7965425201784));
#48341=CARTESIAN_POINT('Ctrl Pts',(56.8176827240047,28.1783377419043,13.7992446313139));
#48342=CARTESIAN_POINT('Ctrl Pts',(56.8211564665033,28.186066045576,13.7997961540347));
#48343=CARTESIAN_POINT('Ctrl Pts',(56.8265787406386,28.1983379128634,13.80066486956));
#48344=CARTESIAN_POINT('Ctrl Pts',(56.8285597596163,28.202866884079,13.8009839597641));
#48345=CARTESIAN_POINT('Ctrl Pts',(56.8320695862194,28.2109729247638,13.8015523151733));
#48346=CARTESIAN_POINT('Ctrl Pts',(56.8336047561259,28.2145470778719,13.8018019570369));
#48347=CARTESIAN_POINT('Ctrl Pts',(56.837253417559,28.2231108163822,13.802397834299));
#48348=CARTESIAN_POINT('Ctrl Pts',(56.839357041771,28.2281045417277,13.8027434733792));
#48349=CARTESIAN_POINT('Ctrl Pts',(56.8456536612356,28.2432237912973,13.8037846017817));
#48350=CARTESIAN_POINT('Ctrl Pts',(56.8497836678832,28.2533755548553,13.8044764418035));
#48351=CARTESIAN_POINT('Ctrl Pts',(56.859138853412,28.2769252653885,13.8060658507437));
#48352=CARTESIAN_POINT('Ctrl Pts',(56.8643032978211,28.2903468541546,13.8069601953942));
#48353=CARTESIAN_POINT('Ctrl Pts',(56.8814524795775,28.3363945866847,13.8099932493751));
#48354=CARTESIAN_POINT('Ctrl Pts',(56.8927300162752,28.3692790308099,13.8120991616735));
#48355=CARTESIAN_POINT('Ctrl Pts',(56.9515715872095,28.5566820118012,13.8238511790861));
#48356=CARTESIAN_POINT('Ctrl Pts',(56.9810729004658,28.7162409482339,13.832959407114));
#48357=CARTESIAN_POINT('Ctrl Pts',(56.9928851853073,28.9084136673114,13.8443856836901));
#48358=CARTESIAN_POINT('Ctrl Pts',(56.9940632644929,28.9392464334113,13.8462308312626));
#48359=CARTESIAN_POINT('Ctrl Pts',(56.9952141605428,29.0160012475613,13.8508679486389));
#48360=CARTESIAN_POINT('Ctrl Pts',(56.9943172901175,29.0619163826329,13.8536811574656));
#48361=CARTESIAN_POINT('Ctrl Pts',(56.9910834041304,29.1216931360445,13.8574134479113));
#48362=CARTESIAN_POINT('Ctrl Pts',(56.9901832593468,29.1356205006884,13.8582879469259));
#48363=CARTESIAN_POINT('Ctrl Pts',(56.9884985263497,29.1580307726393,13.8597034805317));
#48364=CARTESIAN_POINT('Ctrl Pts',(56.9878056026295,29.1665202598075,13.8602416567928));
#48365=CARTESIAN_POINT('Ctrl Pts',(56.9863800870205,29.1827059892552,13.8612715399131));
#48366=CARTESIAN_POINT('Ctrl Pts',(56.9856570820741,29.1904029366585,13.861762938823));
#48367=CARTESIAN_POINT('Ctrl Pts',(56.9838990273516,29.2080184094293,13.862891435862));
#48368=CARTESIAN_POINT('Ctrl Pts',(56.9828343110241,29.217933702026,13.8635294490617));
#48369=CARTESIAN_POINT('Ctrl Pts',(56.9793022726372,29.2486544276286,13.865515160001));
#48370=CARTESIAN_POINT('Ctrl Pts',(56.9765815480504,29.269428728191,13.8668707172512));
#48371=CARTESIAN_POINT('Ctrl Pts',(56.9618187864692,29.3698397011017,13.873486858702));
#48372=CARTESIAN_POINT('Ctrl Pts',(56.9452896746838,29.4487310778269,13.8788856539736));
#48373=CARTESIAN_POINT('Ctrl Pts',(56.8886021908327,29.655929187901,13.893580012467));
#48374=CARTESIAN_POINT('Ctrl Pts',(56.8401780429224,29.7815385032808,13.9030534175969));
#48375=CARTESIAN_POINT('Ctrl Pts',(56.7734796273103,29.9132225485684,13.9132134275387));
#48376=CARTESIAN_POINT('Ctrl Pts',(56.7673345101703,29.9250589994415,13.9141285064394));
#48377=CARTESIAN_POINT('Ctrl Pts',(56.7378299908922,29.980521977619,13.9184224612474));
#48378=CARTESIAN_POINT('Ctrl Pts',(56.7129689835823,30.0233350305033,13.9217553112083));
#48379=CARTESIAN_POINT('Ctrl Pts',(56.6818623218586,30.0725872427281,13.9255742071527));
#48380=CARTESIAN_POINT('Ctrl Pts',(56.6771368589783,30.079961214984,13.9261455423294));
#48381=CARTESIAN_POINT('Ctrl Pts',(56.6693770470305,30.0918964434607,13.9270692865281));
#48382=CARTESIAN_POINT('Ctrl Pts',(56.6663722647528,30.096476650632,13.9274235372464));
#48383=CARTESIAN_POINT('Ctrl Pts',(56.660971340531,30.1046358303036,13.9280540850271));
#48384=CARTESIAN_POINT('Ctrl Pts',(56.6585824444064,30.1082194673971,13.9283308477906));
#48385=CARTESIAN_POINT('Ctrl Pts',(56.6533596955507,30.1159995154923,13.928931288231));
#48386=CARTESIAN_POINT('Ctrl Pts',(56.6505214688519,30.1201928778897,13.9292546690646));
#48387=CARTESIAN_POINT('Ctrl Pts',(56.642453529663,30.1320156897458,13.930165841753));
#48388=CARTESIAN_POINT('Ctrl Pts',(56.6371865936775,30.1396197542288,13.9307512041576));
#48389=CARTESIAN_POINT('Ctrl Pts',(56.6033230585753,30.1877904326045,13.9344569672262));
#48390=CARTESIAN_POINT('Ctrl Pts',(56.5732711193595,30.2273181466497,13.9374869289217));
#48391=CARTESIAN_POINT('Ctrl Pts',(56.4502927154589,30.3771220173194,13.9491032961354));
#48392=CARTESIAN_POINT('Ctrl Pts',(56.3469964045756,30.4783166965125,13.9572751912039));
#48393=CARTESIAN_POINT('Ctrl Pts',(56.1621380870861,30.6238081508515,13.9711097313542));
#48394=CARTESIAN_POINT('Ctrl Pts',(56.0868261923672,30.6751488308281,13.976563788154));
#48395=CARTESIAN_POINT('Ctrl Pts',(55.9950733333197,30.7288987283495,13.9831670697934));
#48396=CARTESIAN_POINT('Ctrl Pts',(55.9817807042995,30.7364816094512,13.9841225584316));
#48397=CARTESIAN_POINT('Ctrl Pts',(55.9599074599513,30.7486279330233,13.9856936264227));
#48398=CARTESIAN_POINT('Ctrl Pts',(55.9513782630393,30.7532830276627,13.986305948046));
#48399=CARTESIAN_POINT('Ctrl Pts',(55.9360282549451,30.761515820783,13.987407576762));
#48400=CARTESIAN_POINT('Ctrl Pts',(55.9292200480779,30.765116704491,13.9878960549306));
#48401=CARTESIAN_POINT('Ctrl Pts',(55.9147108471562,30.7726834631291,13.9889368796685));
#48402=CARTESIAN_POINT('Ctrl Pts',(55.9070045519298,30.7766387739934,13.9894895833196));
#48403=CARTESIAN_POINT('Ctrl Pts',(55.886229306153,30.7871314196129,13.990979440889));
#48404=CARTESIAN_POINT('Ctrl Pts',(55.8731140758901,30.7935754474795,13.9919198039706));
#48405=CARTESIAN_POINT('Ctrl Pts',(55.8062178986304,30.8255365602756,13.9967163606685));
#48406=CARTESIAN_POINT('Ctrl Pts',(55.7513897082779,30.8487788723939,14.0006492634164));
#48407=CARTESIAN_POINT('Ctrl Pts',(55.5783829187453,30.9131505817495,14.0130711142128));
#48408=CARTESIAN_POINT('Ctrl Pts',(55.457325362907,30.9456410000043,14.0217995351282));
#48409=CARTESIAN_POINT('Ctrl Pts',(55.3065832885331,30.9712457652461,14.0324465720854));
#48410=CARTESIAN_POINT('Ctrl Pts',(55.2790315711577,30.9753340498615,14.0343825333049));
#48411=CARTESIAN_POINT('Ctrl Pts',(55.235974155518,30.980804293473,14.0373856139143));
#48412=CARTESIAN_POINT('Ctrl Pts',(55.2205227664561,30.9825839642448,14.0384588020913));
#48413=CARTESIAN_POINT('Ctrl Pts',(55.1932647908902,30.9854008923412,14.040342648024));
#48414=CARTESIAN_POINT('Ctrl Pts',(55.1814668635183,30.9865139739101,14.0411549362191));
#48415=CARTESIAN_POINT('Ctrl Pts',(55.1213401029865,30.9916465357524,14.0452769500359));
#48416=CARTESIAN_POINT('Ctrl Pts',(55.0728817523399,30.9940081356515,14.0485411204418));
#48417=CARTESIAN_POINT('Ctrl Pts',(55.0156722412972,30.9947074484053,14.0522915149576));
#48418=CARTESIAN_POINT('Ctrl Pts',(55.0069622553196,30.9947568667458,14.0528596719106));
#48419=CARTESIAN_POINT('Ctrl Pts',(54.9927887817969,30.9947444467984,14.0537793105317));
#48420=CARTESIAN_POINT('Ctrl Pts',(54.9873254888367,30.9947172150906,14.0541326077435));
#48421=CARTESIAN_POINT('Ctrl Pts',(54.9775566148965,30.9946283857934,14.0547621333201));
#48422=CARTESIAN_POINT('Ctrl Pts',(54.9732510681428,30.9945752928206,14.0550388210311));
#48423=CARTESIAN_POINT('Ctrl Pts',(54.9638717464374,30.9944292572019,14.0556398788227));
#48424=CARTESIAN_POINT('Ctrl Pts',(54.9587981493436,30.9943308957053,14.0559639470099));
#48425=CARTESIAN_POINT('Ctrl Pts',(54.9444267149429,30.9939974111246,14.0568790233002));
#48426=CARTESIAN_POINT('Ctrl Pts',(54.9351299238276,30.9937166164576,14.0574675687562));
#48427=CARTESIAN_POINT('Ctrl Pts',(54.8751566660358,30.9914852688371,14.0612441873773));
#48428=CARTESIAN_POINT('Ctrl Pts',(54.8245635905017,30.9876675931011,14.0643377812585));
#48429=CARTESIAN_POINT('Ctrl Pts',(54.6226861112882,30.9646643647558,14.0765048208363));
#48430=CARTESIAN_POINT('Ctrl Pts',(54.4736773815441,30.9300938729643,14.0851209043516));
#48431=CARTESIAN_POINT('Ctrl Pts',(54.2526950064088,30.8512990205875,14.0989745782191));
#48432=CARTESIAN_POINT('Ctrl Pts',(54.1771218585655,30.818967290988,14.103915184312));
#48433=CARTESIAN_POINT('Ctrl Pts',(54.0903332878911,30.7753196808222,14.1099499694336));
#48434=CARTESIAN_POINT('Ctrl Pts',(54.0769818442792,30.7684148159326,14.1108887313059));
#48435=CARTESIAN_POINT('Ctrl Pts',(54.0552030109209,30.756837792662,14.1124378017198));
#48436=CARTESIAN_POINT('Ctrl Pts',(54.0467290286795,30.7522542139551,14.1130450066679));
#48437=CARTESIAN_POINT('Ctrl Pts',(54.0322029104018,30.7442604761362,14.1140937577726));
#48438=CARTESIAN_POINT('Ctrl Pts',(54.0261347194341,30.7408797283479,14.11453425608));
#48439=CARTESIAN_POINT('Ctrl Pts',(54.0128680127404,30.7333974277856,14.1155026228115));
#48440=CARTESIAN_POINT('Ctrl Pts',(54.0056771701003,30.7292825996562,14.1160309592713));
#48441=CARTESIAN_POINT('Ctrl Pts',(53.991026900061,30.7207776613804,14.1171145565142));
#48442=CARTESIAN_POINT('Ctrl Pts',(53.9835700034755,30.7163835627802,14.1176699529132));
#48443=CARTESIAN_POINT('Ctrl Pts',(53.9652660689358,30.705436557167,14.1190428794947));
#48444=CARTESIAN_POINT('Ctrl Pts',(53.954452547315,30.698828617189,14.1198623862227));
#48445=CARTESIAN_POINT('Ctrl Pts',(53.9245763020348,30.6801785073752,14.1221503794187));
#48446=CARTESIAN_POINT('Ctrl Pts',(53.9056541627246,30.6679157854479,14.1236267852478));
#48447=CARTESIAN_POINT('Ctrl Pts',(53.8444220468922,30.6267430168411,14.1284957860482));
#48448=CARTESIAN_POINT('Ctrl Pts',(53.8030202578763,30.5965249831906,14.1319343696131));
#48449=CARTESIAN_POINT('Ctrl Pts',(53.6628183512369,30.485674246185,14.1440927774701));
#48450=CARTESIAN_POINT('Ctrl Pts',(53.5706230262519,30.3971969852112,14.1530507991673));
#48451=CARTESIAN_POINT('Ctrl Pts',(53.4355569263155,30.2401190356787,14.1674093788836));
#48452=CARTESIAN_POINT('Ctrl Pts',(53.3872642776358,30.1766323853783,14.1728652343878));
#48453=CARTESIAN_POINT('Ctrl Pts',(53.3370318731402,30.1016694239624,14.1787911452356));
#48454=CARTESIAN_POINT('Ctrl Pts',(53.3312375955971,30.092872618301,14.1794788637904));
#48455=CARTESIAN_POINT('Ctrl Pts',(53.3225771294647,30.0794949114825,14.1805126591863));
#48456=CARTESIAN_POINT('Ctrl Pts',(53.3196595307607,30.0749477473832,14.1808619681279));
#48457=CARTESIAN_POINT('Ctrl Pts',(53.3144517963359,30.0667583255159,14.1814872574659));
#48458=CARTESIAN_POINT('Ctrl Pts',(53.3121549471321,30.0631204778881,14.1817636705519));
#48459=CARTESIAN_POINT('Ctrl Pts',(53.3071490676496,30.0551348367984,14.1823674880994));
#48460=CARTESIAN_POINT('Ctrl Pts',(53.3044450126459,30.0507840354969,14.1826945687266));
#48461=CARTESIAN_POINT('Ctrl Pts',(53.2967607423014,30.0383132132239,14.1836268244172));
#48462=CARTESIAN_POINT('Ctrl Pts',(53.2918218084368,30.0301677397863,14.1842293882498));
#48463=CARTESIAN_POINT('Ctrl Pts',(53.2582925747111,29.9739659044742,14.1883457272394));
#48464=CARTESIAN_POINT('Ctrl Pts',(53.2316728004694,29.9247564554568,14.1917443531438));
#48465=CARTESIAN_POINT('Ctrl Pts',(53.1342445573405,29.7250124835798,14.2049986892035));
#48466=CARTESIAN_POINT('Ctrl Pts',(53.0803647391669,29.5671103438876,14.214353633724));
#48467=CARTESIAN_POINT('Ctrl Pts',(53.0466869970968,29.404469869322,14.2242573078582));
#48468=CARTESIAN_POINT('Origin',(55.,29.,3.45145488139523));
#48469=CARTESIAN_POINT('',(53.0466869980082,29.4044698737233,15.1816708487869));
#48470=CARTESIAN_POINT('',(53.0466869327998,29.4044695588112,15.0243707259923));
#48471=CARTESIAN_POINT('',(53.0466869980082,29.4044698737233,3.45145488139523));
#48472=CARTESIAN_POINT('Ctrl Pts',(53.0466869980082,29.4044698737233,15.1816708487869));
#48473=CARTESIAN_POINT('Ctrl Pts',(53.0470224670368,29.4060899598109,15.1815647121178));
#48474=CARTESIAN_POINT('Ctrl Pts',(53.0473599534689,29.4077096374892,15.181458690835));
#48475=CARTESIAN_POINT('Ctrl Pts',(53.048812389329,29.4146370526371,15.181005606289));
#48476=CARTESIAN_POINT('Ctrl Pts',(53.0499469795097,29.4199407058099,15.1806596578178));
#48477=CARTESIAN_POINT('Ctrl Pts',(53.053369592957,29.4356267288989,15.1796390761652));
#48478=CARTESIAN_POINT('Ctrl Pts',(53.055719044283,29.4459957011679,15.1789678051049));
#48479=CARTESIAN_POINT('Ctrl Pts',(53.0797470144503,29.5482398675821,15.1723775328184));
#48480=CARTESIAN_POINT('Ctrl Pts',(53.1078416497406,29.6384982890581,15.1667878124747));
#48481=CARTESIAN_POINT('Ctrl Pts',(53.1638986225485,29.7818569058069,15.1577953700304));
#48482=CARTESIAN_POINT('Ctrl Pts',(53.188038245344,29.8362793946939,15.1543534888154));
#48483=CARTESIAN_POINT('Ctrl Pts',(53.2380289368913,29.9366171738472,15.1478322163256));
#48484=CARTESIAN_POINT('Ctrl Pts',(53.2633349986028,29.9827451920892,15.1447598892344));
#48485=CARTESIAN_POINT('Ctrl Pts',(53.3232484735195,30.0823990999518,15.13787460351));
#48486=CARTESIAN_POINT('Ctrl Pts',(53.3586559090021,30.1353730470149,15.1340456154438));
#48487=CARTESIAN_POINT('Ctrl Pts',(53.4110610019801,30.2061910497867,15.128621603843));
#48488=CARTESIAN_POINT('Ctrl Pts',(53.4259468885532,30.2255532260649,15.1271052657307));
#48489=CARTESIAN_POINT('Ctrl Pts',(53.4479212305432,30.2530744765511,15.1248985445183));
#48490=CARTESIAN_POINT('Ctrl Pts',(53.4547267438086,30.261457374144,15.1242193182452));
#48491=CARTESIAN_POINT('Ctrl Pts',(53.4666025441957,30.275845432215,15.1230410148455));
#48492=CARTESIAN_POINT('Ctrl Pts',(53.4716409286319,30.2818766986242,15.1225432267889));
#48493=CARTESIAN_POINT('Ctrl Pts',(53.4813756062181,30.2933907481243,15.121585394034));
#48494=CARTESIAN_POINT('Ctrl Pts',(53.4860662890743,30.2988781287734,15.12112558254));
#48495=CARTESIAN_POINT('Ctrl Pts',(53.4971772144188,30.3117342545164,15.120040376206));
#48496=CARTESIAN_POINT('Ctrl Pts',(53.5036219846617,30.3190814641071,15.1194139775259));
#48497=CARTESIAN_POINT('Ctrl Pts',(53.5262921221019,30.344546076252,15.1172209308533));
#48498=CARTESIAN_POINT('Ctrl Pts',(53.5427940905725,30.3624132676657,15.1156428080782));
#48499=CARTESIAN_POINT('Ctrl Pts',(53.6537600583608,30.4782367687602,15.1051444187163));
#48500=CARTESIAN_POINT('Ctrl Pts',(53.7576937575479,30.5665915035616,15.0958034167235));
#48501=CARTESIAN_POINT('Ctrl Pts',(53.9492604224329,30.6983156180562,15.079614273548));
#48502=CARTESIAN_POINT('Ctrl Pts',(54.0325944635387,30.7471284376168,15.0728630546955));
#48503=CARTESIAN_POINT('Ctrl Pts',(54.1559212260418,30.8078272938131,15.0635277169891));
#48504=CARTESIAN_POINT('Ctrl Pts',(54.1932589666301,30.8247953180536,15.0607826245665));
#48505=CARTESIAN_POINT('Ctrl Pts',(54.2390008357661,30.8439038001829,15.0575384920683));
#48506=CARTESIAN_POINT('Ctrl Pts',(54.2469269658911,30.8471551001205,15.0569805903791));
#48507=CARTESIAN_POINT('Ctrl Pts',(54.2587483829884,30.8519155078261,15.0561550606406));
#48508=CARTESIAN_POINT('Ctrl Pts',(54.262627734672,30.8534635553317,15.0558851965462));
#48509=CARTESIAN_POINT('Ctrl Pts',(54.270131840966,30.8564307649859,15.0553652338167));
#48510=CARTESIAN_POINT('Ctrl Pts',(54.2737559163352,30.8578515136133,15.0551150456948));
#48511=CARTESIAN_POINT('Ctrl Pts',(54.2819766427312,30.8610465596035,15.0545496354718));
#48512=CARTESIAN_POINT('Ctrl Pts',(54.2865757182341,30.8628144389725,15.0542347968642));
#48513=CARTESIAN_POINT('Ctrl Pts',(54.2990359684272,30.8675512308249,15.0533856816806));
#48514=CARTESIAN_POINT('Ctrl Pts',(54.3069095339833,30.8704875795197,15.0528532906089));
#48515=CARTESIAN_POINT('Ctrl Pts',(54.3449108715701,30.8843868085517,15.0503026453744));
#48516=CARTESIAN_POINT('Ctrl Pts',(54.3752832874809,30.8946727184954,15.0483210694459));
#48517=CARTESIAN_POINT('Ctrl Pts',(54.6011299184018,30.9651356977874,15.0339125865283));
#48518=CARTESIAN_POINT('Ctrl Pts',(54.8045874155427,30.9956676910153,15.0225965721283));
#48519=CARTESIAN_POINT('Ctrl Pts',(55.063939897846,30.9944775996404,15.0070201188638));
#48520=CARTESIAN_POINT('Ctrl Pts',(55.118688714962,30.9919692218243,15.0036763476619));
#48521=CARTESIAN_POINT('Ctrl Pts',(55.1874496559725,30.9859740740519,14.9993748379639));
#48522=CARTESIAN_POINT('Ctrl Pts',(55.2016238507265,30.9845851462249,14.9984827100107));
#48523=CARTESIAN_POINT('Ctrl Pts',(55.2243119224057,30.9821163817143,14.9970455071506));
#48524=CARTESIAN_POINT('Ctrl Pts',(55.2328359829634,30.9811331582019,14.9965034529015));
#48525=CARTESIAN_POINT('Ctrl Pts',(55.2490133844807,30.9791612983959,14.995470633942));
#48526=CARTESIAN_POINT('Ctrl Pts',(55.2566678686109,30.9781831849489,14.9949802073708));
#48527=CARTESIAN_POINT('Ctrl Pts',(55.2740848560142,30.9758547978881,14.9938602427892));
#48528=CARTESIAN_POINT('Ctrl Pts',(55.2838433546837,30.9744765470646,14.9932298385799));
#48529=CARTESIAN_POINT('Ctrl Pts',(55.3091818810254,30.9707061124449,14.9915852238612));
#48530=CARTESIAN_POINT('Ctrl Pts',(55.3247442363619,30.9682015076241,14.9905675160397));
#48531=CARTESIAN_POINT('Ctrl Pts',(55.4692664154368,30.9431814353208,14.9810433865531));
#48532=CARTESIAN_POINT('Ctrl Pts',(55.5957222696909,30.9082107956794,14.9721351533866));
#48533=CARTESIAN_POINT('Ctrl Pts',(55.8062786988101,30.8270005304312,14.9564621732478));
#48534=CARTESIAN_POINT('Ctrl Pts',(55.8921918203495,30.7866198611483,14.9498115676859));
#48535=CARTESIAN_POINT('Ctrl Pts',(56.02522746143,30.7120931189279,14.9393431915314));
#48536=CARTESIAN_POINT('Ctrl Pts',(56.0743057259755,30.6817320689865,14.9354426665937));
#48537=CARTESIAN_POINT('Ctrl Pts',(56.1299361369377,30.6438868393105,14.9310328157275));
#48538=CARTESIAN_POINT('Ctrl Pts',(56.1378300131961,30.6384329354282,14.9304073600285));
#48539=CARTESIAN_POINT('Ctrl Pts',(56.1498897723805,30.6299716146594,14.9294526632382));
#48540=CARTESIAN_POINT('Ctrl Pts',(56.1540837705836,30.6270047956683,14.9291208068982));
#48541=CARTESIAN_POINT('Ctrl Pts',(56.1617683302979,30.6215241014703,14.9285131135054));
#48542=CARTESIAN_POINT('Ctrl Pts',(56.1652622123637,30.6190151457151,14.928236962584));
#48543=CARTESIAN_POINT('Ctrl Pts',(56.1731119339761,30.6133396887155,14.9276168401683));
#48544=CARTESIAN_POINT('Ctrl Pts',(56.1774630757785,30.6101668446562,14.9272733084638));
#48545=CARTESIAN_POINT('Ctrl Pts',(56.1902208486627,30.6007845327608,14.9262664887576));
#48546=CARTESIAN_POINT('Ctrl Pts',(56.1985917433874,30.5945264603346,14.9256064295306));
#48547=CARTESIAN_POINT('Ctrl Pts',(56.2640150478082,30.5448097249438,14.9204487135644));
#48548=CARTESIAN_POINT('Ctrl Pts',(56.318741931028,30.4983635156922,14.916139683763));
#48549=CARTESIAN_POINT('Ctrl Pts',(56.4978979214821,30.3288772682684,14.9015893367329));
#48550=CARTESIAN_POINT('Ctrl Pts',(56.6085814031798,30.1925102403982,14.891723002521));
#48551=CARTESIAN_POINT('Ctrl Pts',(56.722676280292,30.0066191030003,14.8785112448309));
#48552=CARTESIAN_POINT('Ctrl Pts',(56.7440804584488,29.9690606385643,14.8758572313731));
#48553=CARTESIAN_POINT('Ctrl Pts',(56.770387149474,29.9192007653189,14.87233846652));
#48554=CARTESIAN_POINT('Ctrl Pts',(56.7764120171962,29.9075026380439,14.8715132401188));
#48555=CARTESIAN_POINT('Ctrl Pts',(56.7860668617947,29.8882918027939,14.8701582055884));
#48556=CARTESIAN_POINT('Ctrl Pts',(56.7897662804536,29.8808142935112,14.8696308211571));
#48557=CARTESIAN_POINT('Ctrl Pts',(56.7968271033006,29.866314339404,14.8686081224534));
#48558=CARTESIAN_POINT('Ctrl Pts',(56.8001945202945,29.8592949785211,14.8681130274366));
#48559=CARTESIAN_POINT('Ctrl Pts',(56.8078698867733,29.8430525820942,14.866967290632));
#48560=CARTESIAN_POINT('Ctrl Pts',(56.8121484703279,29.8338159862046,14.8663156563821));
#48561=CARTESIAN_POINT('Ctrl Pts',(56.8257232313318,29.8039127854338,14.8642054954654));
#48562=CARTESIAN_POINT('Ctrl Pts',(56.8347377230418,29.7831210007921,14.8627374827386));
#48563=CARTESIAN_POINT('Ctrl Pts',(56.9084418751415,29.6048615727444,14.8501397812045));
#48564=CARTESIAN_POINT('Ctrl Pts',(56.9530696874973,29.4398905981779,14.8383145967836));
#48565=CARTESIAN_POINT('Ctrl Pts',(56.990086119627,29.1702572158588,14.8193602346738));
#48566=CARTESIAN_POINT('Ctrl Pts',(56.9961894599312,29.0682839503516,14.8122975621214));
#48567=CARTESIAN_POINT('Ctrl Pts',(56.994269453784,28.9547150492043,14.8048267434208));
#48568=CARTESIAN_POINT('Ctrl Pts',(56.9939732964893,28.943150293604,14.8040706430821));
#48569=CARTESIAN_POINT('Ctrl Pts',(56.9933865923527,28.9260531873612,14.8029603609363));
#48570=CARTESIAN_POINT('Ctrl Pts',(56.9931735891566,28.9205186629455,14.8026021164631));
#48571=CARTESIAN_POINT('Ctrl Pts',(56.9927554370513,28.9107162610247,14.8019697674695));
#48572=CARTESIAN_POINT('Ctrl Pts',(56.9925596248488,28.9064480862396,14.8016951563733));
#48573=CARTESIAN_POINT('Ctrl Pts',(56.9921047054893,28.8971824680362,14.8011006065749));
#48574=CARTESIAN_POINT('Ctrl Pts',(56.9918405076977,28.8921853640459,14.8007809519491));
#48575=CARTESIAN_POINT('Ctrl Pts',(56.9910633811949,28.8784659977468,14.7999059583668));
#48576=CARTESIAN_POINT('Ctrl Pts',(56.9905119389645,28.8697459056586,14.7993527026527));
#48577=CARTESIAN_POINT('Ctrl Pts',(56.9873980599879,28.8251586075112,14.7965373413393));
#48578=CARTESIAN_POINT('Ctrl Pts',(56.9839232481805,28.789359360743,14.7943216636943));
#48579=CARTESIAN_POINT('Ctrl Pts',(56.9570975552413,28.5737898798137,14.7811460681651));
#48580=CARTESIAN_POINT('Ctrl Pts',(56.9102979242465,28.3977864552719,14.7710179168197));
#48581=CARTESIAN_POINT('Ctrl Pts',(56.8128589983795,28.1647445950081,14.7560057494288));
#48582=CARTESIAN_POINT('Ctrl Pts',(56.7818567324052,28.1005033283168,14.7516908206727));
#48583=CARTESIAN_POINT('Ctrl Pts',(56.7400643474081,28.0245819070587,14.7462981885722));
#48584=CARTESIAN_POINT('Ctrl Pts',(56.7324875679599,28.0111869765984,14.7453353145438));
#48585=CARTESIAN_POINT('Ctrl Pts',(56.7203197491604,27.9902448185969,14.7438111552698));
#48586=CARTESIAN_POINT('Ctrl Pts',(56.7158321648822,27.9826379485921,14.743253579194));
#48587=CARTESIAN_POINT('Ctrl Pts',(56.707347649005,27.9684717332072,14.742207669382));
#48588=CARTESIAN_POINT('Ctrl Pts',(56.7033630471215,27.9619051648476,14.7417197888606));
#48589=CARTESIAN_POINT('Ctrl Pts',(56.694382684137,27.9472965695562,14.7406274589596));
#48590=CARTESIAN_POINT('Ctrl Pts',(56.6893674205685,27.9392668073359,14.7400223050317));
#48591=CARTESIAN_POINT('Ctrl Pts',(56.6765342626566,27.9190419694735,14.7384858723168));
#48592=CARTESIAN_POINT('Ctrl Pts',(56.6686404410841,27.9068959529194,14.7375518152628));
#48593=CARTESIAN_POINT('Ctrl Pts',(56.6210719546175,27.8354196463711,14.731986339785));
#48594=CARTESIAN_POINT('Ctrl Pts',(56.5783728242281,27.7781739700948,14.7272423631001));
#48595=CARTESIAN_POINT('Ctrl Pts',(56.4283787549943,27.5980969860731,14.7113443557333));
#48596=CARTESIAN_POINT('Ctrl Pts',(56.3091114502449,27.4861254197318,14.6997853696989));
#48597=CARTESIAN_POINT('Ctrl Pts',(56.1356396186382,27.3592538635945,14.6850801299537));
#48598=CARTESIAN_POINT('Ctrl Pts',(56.092530704955,27.3302386652636,14.6815793239745));
#48599=CARTESIAN_POINT('Ctrl Pts',(56.0403740439414,27.2980196950469,14.6775630778841));
#48600=CARTESIAN_POINT('Ctrl Pts',(56.0323790324984,27.2931582817371,14.6769533273823));
#48601=CARTESIAN_POINT('Ctrl Pts',(56.0199853427721,27.2857411702807,14.6760175170521));
#48602=CARTESIAN_POINT('Ctrl Pts',(56.0156107266987,27.2831458163414,14.6756889969856));
#48603=CARTESIAN_POINT('Ctrl Pts',(56.0075154551249,27.2783848565416,14.6750844408483));
#48604=CARTESIAN_POINT('Ctrl Pts',(56.0037977354804,27.2762145721247,14.6748081142109));
#48605=CARTESIAN_POINT('Ctrl Pts',(55.99535933784,27.2713250657538,14.6741838596373));
#48606=CARTESIAN_POINT('Ctrl Pts',(55.9906345346999,27.2686131396879,14.673836398588));
#48607=CARTESIAN_POINT('Ctrl Pts',(55.978371738512,27.2616412135329,14.6729397845214));
#48608=CARTESIAN_POINT('Ctrl Pts',(55.9708169210206,27.257410822533,14.6723924523817));
#48609=CARTESIAN_POINT('Ctrl Pts',(55.9216739961126,27.2303115716273,14.6688631748919));
#48610=CARTESIAN_POINT('Ctrl Pts',(55.8793049003513,27.2088819757356,14.6659636077121));
#48611=CARTESIAN_POINT('Ctrl Pts',(55.8193476125214,27.1811976653523,14.6620007681012));
#48612=CARTESIAN_POINT('Ctrl Pts',(55.802378914537,27.1736482946895,14.6608944315436));
#48613=CARTESIAN_POINT('Ctrl Pts',(55.6639361306865,27.1143571042289,14.6519720393256));
#48614=CARTESIAN_POINT('Ctrl Pts',(55.5377023741406,27.0745548605659,14.6444580527923));
#48615=CARTESIAN_POINT('Ctrl Pts',(55.3302621046573,27.0311585553832,14.6319688700782));
#48616=CARTESIAN_POINT('Ctrl Pts',(55.2511625191969,27.0195139544978,14.6271798609614));
#48617=CARTESIAN_POINT('Ctrl Pts',(55.1507973913819,27.0108486752994,14.6209522199962));
#48618=CARTESIAN_POINT('Ctrl Pts',(55.1299850358691,27.0093803262718,14.6196529582574));
#48619=CARTESIAN_POINT('Ctrl Pts',(55.0992133985729,27.0076939548044,14.617718768137));
#48620=CARTESIAN_POINT('Ctrl Pts',(55.08926893795,27.0072236133591,14.6170916676523));
#48621=CARTESIAN_POINT('Ctrl Pts',(55.071598864522,27.006520404196,14.6159736114701));
#48622=CARTESIAN_POINT('Ctrl Pts',(55.0638745826813,27.0062579576968,14.6154835845938));
#48623=CARTESIAN_POINT('Ctrl Pts',(55.0476260098276,27.0058004047641,14.6144500005336));
#48624=CARTESIAN_POINT('Ctrl Pts',(55.039101621038,27.005615051705,14.6139061503018));
#48625=CARTESIAN_POINT('Ctrl Pts',(55.0165822687428,27.0052698245226,14.6124650602729));
#48626=CARTESIAN_POINT('Ctrl Pts',(55.002586557658,27.0052025822507,14.6115649664495));
#48627=CARTESIAN_POINT('Ctrl Pts',(54.9423175960707,27.0055472793374,14.60766900895));
#48628=CARTESIAN_POINT('Ctrl Pts',(54.8960702830593,27.0074220349251,14.6046283759));
#48629=CARTESIAN_POINT('Ctrl Pts',(54.6809195074619,27.0236540446459,14.5902348815082));
#48630=CARTESIAN_POINT('Ctrl Pts',(54.5142360685767,27.0578948832675,14.5782882415939));
#48631=CARTESIAN_POINT('Ctrl Pts',(54.3066928393707,27.1289454451837,14.5631209403966));
#48632=CARTESIAN_POINT('Ctrl Pts',(54.2600803563821,27.1468838258741,14.5597009203411));
#48633=CARTESIAN_POINT('Ctrl Pts',(54.1973096322782,27.1737872746396,14.5551176632957));
#48634=CARTESIAN_POINT('Ctrl Pts',(54.1805320085016,27.1812540014247,14.5538949244316));
#48635=CARTESIAN_POINT('Ctrl Pts',(54.1518227375656,27.1945087500848,14.5518094447632));
#48636=CARTESIAN_POINT('Ctrl Pts',(54.1398415253075,27.2001859143369,14.550941194762));
#48637=CARTESIAN_POINT('Ctrl Pts',(54.1226532505167,27.2085412359049,14.5496995451603));
#48638=CARTESIAN_POINT('Ctrl Pts',(54.1174002805988,27.2111233805302,14.549320616206));
#48639=CARTESIAN_POINT('Ctrl Pts',(54.108264524747,27.2156641808923,14.5486626326446));
#48640=CARTESIAN_POINT('Ctrl Pts',(54.1043766705967,27.2176124645689,14.5483829491101));
#48641=CARTESIAN_POINT('Ctrl Pts',(54.0961799444754,27.2217536044502,14.5477940257345));
#48642=CARTESIAN_POINT('Ctrl Pts',(54.0918726588997,27.2239494180637,14.5474849721714));
#48643=CARTESIAN_POINT('Ctrl Pts',(54.0802783229576,27.2299133080003,14.5466540801106));
#48644=CARTESIAN_POINT('Ctrl Pts',(54.0730063696024,27.23371076119,14.5461340336098));
#48645=CARTESIAN_POINT('Ctrl Pts',(54.0401312137691,27.2511373024455,14.5437870080365));
#48646=CARTESIAN_POINT('Ctrl Pts',(54.0148022803011,27.2652797114822,14.5419897966795));
#48647=CARTESIAN_POINT('Ctrl Pts',(53.8105682327205,27.3852307943931,14.5275153567077));
#48648=CARTESIAN_POINT('Ctrl Pts',(53.6488833095392,27.5178618052388,14.5160367210116));
#48649=CARTESIAN_POINT('Ctrl Pts',(53.4739728698963,27.7141933839252,14.5002475205211));
#48650=CARTESIAN_POINT('Ctrl Pts',(53.4390770486406,27.7567879622548,14.4968884947703));
#48651=CARTESIAN_POINT('Ctrl Pts',(53.3974142753498,27.8121658395127,14.4925697712738));
#48652=CARTESIAN_POINT('Ctrl Pts',(53.3889620749612,27.8236549038843,14.4916763415755));
#48653=CARTESIAN_POINT('Ctrl Pts',(53.3756209184998,27.8422030106943,14.4902375384475));
#48654=CARTESIAN_POINT('Ctrl Pts',(53.3706529698515,27.8492048312158,14.4896951978067));
#48655=CARTESIAN_POINT('Ctrl Pts',(53.3613063049198,27.8625598609991,14.4886621558874));
#48656=CARTESIAN_POINT('Ctrl Pts',(53.3569189387276,27.8689068475726,14.4881717949501));
#48657=CARTESIAN_POINT('Ctrl Pts',(53.3470163653832,27.8834116105564,14.4870524304576));
#48658=CARTESIAN_POINT('Ctrl Pts',(53.3415245540366,27.8915850428766,14.4864225641524));
#48659=CARTESIAN_POINT('Ctrl Pts',(53.3274149942888,27.9129238532495,14.4847802759296));
#48660=CARTESIAN_POINT('Ctrl Pts',(53.3188922402634,27.9261509291702,14.4837643729607));
#48661=CARTESIAN_POINT('Ctrl Pts',(53.2398224855917,28.0521135241842,14.474107398011));
#48662=CARTESIAN_POINT('Ctrl Pts',(53.1805722656838,28.1715168978081,14.4650506855469));
#48663=CARTESIAN_POINT('Ctrl Pts',(53.0959067780878,28.3959401859881,14.4483853649842));
#48664=CARTESIAN_POINT('Ctrl Pts',(53.066270254425,28.4988515215815,14.4408763443914));
#48665=CARTESIAN_POINT('Ctrl Pts',(53.0361616183748,28.6473587463756,14.4305583528831));
#48666=CARTESIAN_POINT('Ctrl Pts',(53.0287668261489,28.691361855593,14.4275653105527));
#48667=CARTESIAN_POINT('Ctrl Pts',(53.0216615227814,28.7444902083758,14.4240563189061));
#48668=CARTESIAN_POINT('Ctrl Pts',(53.0205300394347,28.7534091109344,14.4234707796412));
#48669=CARTESIAN_POINT('Ctrl Pts',(53.0188622654596,28.7673072562234,14.4225641552479));
#48670=CARTESIAN_POINT('Ctrl Pts',(53.0182843774749,28.772281250233,14.4222408408804));
#48671=CARTESIAN_POINT('Ctrl Pts',(53.0172435746198,28.7815437692101,14.4216409861906));
#48672=CARTESIAN_POINT('Ctrl Pts',(53.0167758427499,28.7858315855335,14.4213641922033));
#48673=CARTESIAN_POINT('Ctrl Pts',(53.0157374101552,28.7956463645899,14.4207326196536));
#48674=CARTESIAN_POINT('Ctrl Pts',(53.0151758913133,28.80117421414,14.4203783546339));
#48675=CARTESIAN_POINT('Ctrl Pts',(53.0137635028851,28.8156810281445,14.4194522778057));
#48676=CARTESIAN_POINT('Ctrl Pts',(53.0129504080065,28.8246636604479,14.4188824905126));
#48677=CARTESIAN_POINT('Ctrl Pts',(53.0076044433637,28.8885459938445,14.4148541971869));
#48678=CARTESIAN_POINT('Ctrl Pts',(53.0052860625162,28.9436125615935,14.4115069438421));
#48679=CARTESIAN_POINT('Ctrl Pts',(53.0051882323728,29.0948294972808,14.4024882069693));
#48680=CARTESIAN_POINT('Ctrl Pts',(53.0120736301616,29.1908332932345,14.3969496620502));
#48681=CARTESIAN_POINT('Ctrl Pts',(53.0316091386433,29.3256930481689,14.3890273030344));
#48682=CARTESIAN_POINT('Ctrl Pts',(53.0385576087489,29.3652105038048,14.386688994918));
#48683=CARTESIAN_POINT('Ctrl Pts',(53.0466870452705,29.4044701019679,14.3843322575863));
#48684=CARTESIAN_POINT('',(53.0052501615731,28.9991971327588,14.249733584776));
#48685=CARTESIAN_POINT('Ctrl Pts',(53.0466869970968,29.404469869322,14.2242573078582));
#48686=CARTESIAN_POINT('Ctrl Pts',(53.040725367752,29.375679274519,14.2260104549135));
#48687=CARTESIAN_POINT('Ctrl Pts',(53.0353967871213,29.3467400824718,14.2277788712771));
#48688=CARTESIAN_POINT('Ctrl Pts',(53.0243618871024,29.2783333519043,14.231984850153));
#48689=CARTESIAN_POINT('Ctrl Pts',(53.019196515761,29.2388150623199,14.2344347376859));
#48690=CARTESIAN_POINT('Ctrl Pts',(53.0138972638999,29.1860067588108,14.2377471311623));
#48691=CARTESIAN_POINT('Ctrl Pts',(53.0127073123571,29.1728304169053,14.2385767742036));
#48692=CARTESIAN_POINT('Ctrl Pts',(53.0109796151204,29.1513120324257,14.2399372250438));
#48693=CARTESIAN_POINT('Ctrl Pts',(53.0103630697111,29.1429765883835,14.2404655713147));
#48694=CARTESIAN_POINT('Ctrl Pts',(53.0092998729139,29.1272605095596,14.2414644008461));
#48695=CARTESIAN_POINT('Ctrl Pts',(53.0088418363709,29.1198807669603,14.2419345208487));
#48696=CARTESIAN_POINT('Ctrl Pts',(53.0079989932211,29.1049598385266,14.2428873418051));
#48697=CARTESIAN_POINT('Ctrl Pts',(53.0076159563652,29.09741867791,14.2433700899416));
#48698=CARTESIAN_POINT('Ctrl Pts',(53.0066687223206,29.0764165808719,14.244717925102));
#48699=CARTESIAN_POINT('Ctrl Pts',(53.0061980781166,29.0629520294684,14.2455858999131));
#48700=CARTESIAN_POINT('Ctrl Pts',(53.005447988207,29.0327244597251,14.2475434846741));
#48701=CARTESIAN_POINT('Ctrl Pts',(53.0052434143432,29.0159608454436,14.2486353362988));
#48702=CARTESIAN_POINT('Ctrl Pts',(53.0052501615731,28.9991971327588,14.249733584776));
#48703=CARTESIAN_POINT('Ctrl Pts',(53.0052501609099,28.9991987822212,14.2497334767141));
#48704=CARTESIAN_POINT('Ctrl Pts',(53.0053246644065,28.8137113382107,14.2618853925284));
#48705=CARTESIAN_POINT('Ctrl Pts',(53.0312721441039,28.6291575593077,14.2748853711652));
#48706=CARTESIAN_POINT('Ctrl Pts',(53.1040908771866,28.3748505603294,14.2932407346553));
#48707=CARTESIAN_POINT('Ctrl Pts',(53.1303690160143,28.3001672407954,14.2986699861498));
#48708=CARTESIAN_POINT('Ctrl Pts',(53.1663243404648,28.2146027170922,14.3047952468782));
#48709=CARTESIAN_POINT('Ctrl Pts',(53.1717628123662,28.2020249835474,14.305693077749));
#48710=CARTESIAN_POINT('Ctrl Pts',(53.1797408127415,28.1840838033772,14.3069690547199));
#48711=CARTESIAN_POINT('Ctrl Pts',(53.1821751904497,28.1786744173794,14.3073531513019));
#48712=CARTESIAN_POINT('Ctrl Pts',(53.1864408348969,28.1693076805571,14.3080170638155));
#48713=CARTESIAN_POINT('Ctrl Pts',(53.1882610004978,28.1653453564037,14.3082975427918));
#48714=CARTESIAN_POINT('Ctrl Pts',(53.1918573983875,28.1575835444411,14.3088462156829));
#48715=CARTESIAN_POINT('Ctrl Pts',(53.1936326222042,28.1537836862946,14.3091144716429));
#48716=CARTESIAN_POINT('Ctrl Pts',(53.1985749526546,28.1432910740531,14.3098543151022));
#48717=CARTESIAN_POINT('Ctrl Pts',(53.2017673977033,28.1366102287286,14.3103243759331));
#48718=CARTESIAN_POINT('Ctrl Pts',(53.2146432621076,28.1100460769859,14.3121899812013));
#48719=CARTESIAN_POINT('Ctrl Pts',(53.2246202659834,28.090305786585,14.3135686415586));
#48720=CARTESIAN_POINT('Ctrl Pts',(53.3354139651265,27.8798607475237,14.3282262007319));
#48721=CARTESIAN_POINT('Ctrl Pts',(53.4662080156965,27.7065280515995,14.3400863159308));
#48722=CARTESIAN_POINT('Ctrl Pts',(53.6487888635769,27.5321433858319,14.3552415069585));
#48723=CARTESIAN_POINT('Ctrl Pts',(53.6760230284697,27.5075324732154,14.3574683069494));
#48724=CARTESIAN_POINT('Ctrl Pts',(53.7174944090601,27.4720844625924,14.3608225240116));
#48725=CARTESIAN_POINT('Ctrl Pts',(53.7312242632586,27.4606642409316,14.3619272588977));
#48726=CARTESIAN_POINT('Ctrl Pts',(53.7534974503018,27.4426382840054,14.3637115088071));
#48727=CARTESIAN_POINT('Ctrl Pts',(53.7619444950756,27.435914746434,14.3643863979676));
#48728=CARTESIAN_POINT('Ctrl Pts',(53.777834958953,27.4234759005362,14.3656529456451));
#48729=CARTESIAN_POINT('Ctrl Pts',(53.7852649646029,27.4177438852326,14.366243930374));
#48730=CARTESIAN_POINT('Ctrl Pts',(53.7987118637462,27.4075205663011,14.3673114594031));
#48731=CARTESIAN_POINT('Ctrl Pts',(53.8047142283885,27.4030103773841,14.3677872559044));
#48732=CARTESIAN_POINT('Ctrl Pts',(53.8174100215412,27.3935824046972,14.3687921926577));
#48733=CARTESIAN_POINT('Ctrl Pts',(53.824108975014,27.3886723357454,14.3693216184123));
#48734=CARTESIAN_POINT('Ctrl Pts',(53.8413625459517,27.3761910414697,14.3706831822829));
#48735=CARTESIAN_POINT('Ctrl Pts',(53.8519606769851,27.3686809069383,14.3715176305469));
#48736=CARTESIAN_POINT('Ctrl Pts',(53.8937067553167,27.3397067435328,14.3747976821944));
#48737=CARTESIAN_POINT('Ctrl Pts',(53.9253876418756,27.319028138314,14.3772723654842));
#48738=CARTESIAN_POINT('Ctrl Pts',(54.1275229559937,27.195141398671,14.3929823955489));
#48739=CARTESIAN_POINT('Ctrl Pts',(54.3120421664303,27.1170725062956,14.4071372283339));
#48740=CARTESIAN_POINT('Ctrl Pts',(54.5583117727563,27.0539865963618,14.4245638823944));
#48741=CARTESIAN_POINT('Ctrl Pts',(54.6121753874919,27.0425399306265,14.4282802423395));
#48742=CARTESIAN_POINT('Ctrl Pts',(54.6758045606403,27.0317482541399,14.4325093229748));
#48743=CARTESIAN_POINT('Ctrl Pts',(54.6851721342161,27.0302281752847,14.4331278668094));
#48744=CARTESIAN_POINT('Ctrl Pts',(54.6996050249004,27.0279917383704,14.4340742560793));
#48745=CARTESIAN_POINT('Ctrl Pts',(54.704662693833,27.0272279396747,14.4344046480424));
#48746=CARTESIAN_POINT('Ctrl Pts',(54.7139802870532,27.0258574519073,14.4350109532414));
#48747=CARTESIAN_POINT('Ctrl Pts',(54.7182392201102,27.0252450937009,14.4352871701495));
#48748=CARTESIAN_POINT('Ctrl Pts',(54.7278595110274,27.0238936249648,14.4359090563574));
#48749=CARTESIAN_POINT('Ctrl Pts',(54.7332219071396,27.0231625504315,14.4362542742205));
#48750=CARTESIAN_POINT('Ctrl Pts',(54.7490728202296,27.0210672117067,14.4372706869758));
#48751=CARTESIAN_POINT('Ctrl Pts',(54.7595694807707,27.0197645071737,14.4379385604191));
#48752=CARTESIAN_POINT('Ctrl Pts',(54.868931029553,27.0070744290167,14.4448474175373));
#48753=CARTESIAN_POINT('Ctrl Pts',(54.9685201262177,27.0030157942425,14.450721636958));
#48754=CARTESIAN_POINT('Ctrl Pts',(55.1716179412225,27.009944127616,14.4625753700099));
#48755=CARTESIAN_POINT('Ctrl Pts',(55.2747921886321,27.0215501178099,14.4685348556598));
#48756=CARTESIAN_POINT('Ctrl Pts',(55.4292858191351,27.0512516705974,14.4778352207209));
#48757=CARTESIAN_POINT('Ctrl Pts',(55.4815419551017,27.0635023678334,14.4810465237869));
#48758=CARTESIAN_POINT('Ctrl Pts',(55.5556634637849,27.0840649084069,14.4857385798045));
#48759=CARTESIAN_POINT('Ctrl Pts',(55.5779774706556,27.0906778329818,14.4871691596413));
#48760=CARTESIAN_POINT('Ctrl Pts',(55.6176548622142,27.103195797205,14.4897485847687));
#48761=CARTESIAN_POINT('Ctrl Pts',(55.6350623518291,27.1089528067584,14.4908926849355));
#48762=CARTESIAN_POINT('Ctrl Pts',(55.6613228049286,27.118041150515,14.4926386631151));
#48763=CARTESIAN_POINT('Ctrl Pts',(55.6702358105484,27.1211969457125,14.4932347894402));
#48764=CARTESIAN_POINT('Ctrl Pts',(55.6863472835309,27.1270307119562,14.4943189270248));
#48765=CARTESIAN_POINT('Ctrl Pts',(55.6935534003728,27.1296871315962,14.4948062186628));
#48766=CARTESIAN_POINT('Ctrl Pts',(55.7090214788684,27.1354908771771,14.4958574438798));
#48767=CARTESIAN_POINT('Ctrl Pts',(55.7172781907303,27.1386516393852,14.4964218152924));
#48768=CARTESIAN_POINT('Ctrl Pts',(55.73951709598,27.1473348862068,14.4979508167069));
#48769=CARTESIAN_POINT('Ctrl Pts',(55.7534580969242,27.1529606298484,14.4989188715005));
#48770=CARTESIAN_POINT('Ctrl Pts',(55.8219923878431,27.1815219284064,14.5037262846639));
#48771=CARTESIAN_POINT('Ctrl Pts',(55.8756042850608,27.2067209030127,14.5076411152743));
#48772=CARTESIAN_POINT('Ctrl Pts',(56.0482596555304,27.2974628405327,14.520772528181));
#48773=CARTESIAN_POINT('Ctrl Pts',(56.1617265122295,27.3727739338602,14.5302875380155));
#48774=CARTESIAN_POINT('Ctrl Pts',(56.330718030919,27.5116801609606,14.5454914255561));
#48775=CARTESIAN_POINT('Ctrl Pts',(56.3914499721474,27.5682960389631,14.5512045018767));
#48776=CARTESIAN_POINT('Ctrl Pts',(56.4593854929884,27.6400467315979,14.557745936076));
#48777=CARTESIAN_POINT('Ctrl Pts',(56.4701484411296,27.6516890165338,14.5587870933634));
#48778=CARTESIAN_POINT('Ctrl Pts',(56.4849856181495,27.6681273231459,14.5602276376931));
#48779=CARTESIAN_POINT('Ctrl Pts',(56.4891773707381,27.6728158098745,14.5606352162866));
#48780=CARTESIAN_POINT('Ctrl Pts',(56.49627850638,27.6808344508043,14.5613265935474));
#48781=CARTESIAN_POINT('Ctrl Pts',(56.4991990986591,27.684154576377,14.561611211378));
#48782=CARTESIAN_POINT('Ctrl Pts',(56.504801347771,27.6905660715276,14.5621576310641));
#48783=CARTESIAN_POINT('Ctrl Pts',(56.5074845491426,27.6936560008499,14.5624195530706));
#48784=CARTESIAN_POINT('Ctrl Pts',(56.5139107807156,27.7011025060543,14.5630474306968));
#48785=CARTESIAN_POINT('Ctrl Pts',(56.5176445666459,27.7054670637592,14.5634127171132));
#48786=CARTESIAN_POINT('Ctrl Pts',(56.5312236968103,27.7214797000593,14.5647432072247));
#48787=CARTESIAN_POINT('Ctrl Pts',(56.5409545136199,27.733224808045,14.5657005286848));
#48788=CARTESIAN_POINT('Ctrl Pts',(56.6342286097396,27.8484721863339,14.5749281809192));
#48789=CARTESIAN_POINT('Ctrl Pts',(56.707368598885,27.9599893859013,14.5825857304154));
#48790=CARTESIAN_POINT('Ctrl Pts',(56.8340411388648,28.2030047558217,14.5985027339655));
#48791=CARTESIAN_POINT('Ctrl Pts',(56.8857658330866,28.3345765345478,14.6067412839686));
#48792=CARTESIAN_POINT('Ctrl Pts',(56.9279053956793,28.4876287967668,14.616589803726));
#48793=CARTESIAN_POINT('Ctrl Pts',(56.9323940524154,28.5048266373916,14.6176994434686));
#48794=CARTESIAN_POINT('Ctrl Pts',(56.9388898675969,28.531149412194,14.6194033927348));
#48795=CARTESIAN_POINT('Ctrl Pts',(56.9410638034397,28.540232560335,14.6199923703701));
#48796=CARTESIAN_POINT('Ctrl Pts',(56.9449075838716,28.5568059780862,14.621069000158));
#48797=CARTESIAN_POINT('Ctrl Pts',(56.9465981536306,28.5642912940174,14.6215559811152));
#48798=CARTESIAN_POINT('Ctrl Pts',(56.9501630308908,28.5805104216208,14.6226128199122));
#48799=CARTESIAN_POINT('Ctrl Pts',(56.9520219416241,28.5892474119579,14.623183155736));
#48800=CARTESIAN_POINT('Ctrl Pts',(56.9569323960075,28.6131132581165,14.6247440374216));
#48801=CARTESIAN_POINT('Ctrl Pts',(56.9598670916731,28.6282652632737,14.6257382528747));
#48802=CARTESIAN_POINT('Ctrl Pts',(56.9741944138705,28.7071297318096,14.6309309320337));
#48803=CARTESIAN_POINT('Ctrl Pts',(56.982655906263,28.771328660021,14.6352203386183));
#48804=CARTESIAN_POINT('Ctrl Pts',(57.0019543244248,29.0050041288652,14.6510615840544));
#48805=CARTESIAN_POINT('Ctrl Pts',(56.9942720472674,29.1752527466829,14.6631062258711));
#48806=CARTESIAN_POINT('Ctrl Pts',(56.9560955699289,29.3943209878762,14.6783280036037));
#48807=CARTESIAN_POINT('Ctrl Pts',(56.9450072694434,29.445810169866,14.6818777778332));
#48808=CARTESIAN_POINT('Ctrl Pts',(56.9295553825495,29.5058969481292,14.6859424971687));
#48809=CARTESIAN_POINT('Ctrl Pts',(56.9271530388352,29.5149726882374,14.6865543155088));
#48810=CARTESIAN_POINT('Ctrl Pts',(56.9233486493168,29.5289456268321,14.6874926144979));
#48811=CARTESIAN_POINT('Ctrl Pts',(56.9219918097328,29.5338548376574,14.6878215755629));
#48812=CARTESIAN_POINT('Ctrl Pts',(56.9194536113817,29.5429032359507,14.6884265409755));
#48813=CARTESIAN_POINT('Ctrl Pts',(56.9182776640426,29.5470437771399,14.6887028389852));
#48814=CARTESIAN_POINT('Ctrl Pts',(56.9155853791141,29.5564079453343,14.6893265232576));
#48815=CARTESIAN_POINT('Ctrl Pts',(56.914061075659,29.5616291896187,14.6896734463339));
#48816=CARTESIAN_POINT('Ctrl Pts',(56.9100630397513,29.5751184432691,14.6905677432495));
#48817=CARTESIAN_POINT('Ctrl Pts',(56.9075569439705,29.5833768519755,14.6911133117998));
#48818=CARTESIAN_POINT('Ctrl Pts',(56.891085870825,29.6364132728549,14.6946060667833));
#48819=CARTESIAN_POINT('Ctrl Pts',(56.8755975894105,29.6807070429271,14.6974728144533));
#48820=CARTESIAN_POINT('Ctrl Pts',(56.851433863643,29.7427013622904,14.7014673662404));
#48821=CARTESIAN_POINT('Ctrl Pts',(56.8440375626336,29.7608798654152,14.7026364426345));
#48822=CARTESIAN_POINT('Ctrl Pts',(56.8165545793273,29.8256712537723,14.7068048569867));
#48823=CARTESIAN_POINT('Ctrl Pts',(56.7949583681512,29.8716239774689,14.7097646614618));
#48824=CARTESIAN_POINT('Ctrl Pts',(56.7277345569171,30.0015414198841,14.7182687370513));
#48825=CARTESIAN_POINT('Ctrl Pts',(56.6778005400033,30.0831141937596,14.7237844735192));
#48826=CARTESIAN_POINT('Ctrl Pts',(56.593791004895,30.2005182071573,14.7323514863034));
#48827=CARTESIAN_POINT('Ctrl Pts',(56.5639169876408,30.2391839609559,14.73528577473));
#48828=CARTESIAN_POINT('Ctrl Pts',(56.5118993934418,30.3016295410715,14.7402533278628));
#48829=CARTESIAN_POINT('Ctrl Pts',(56.4905397403674,30.326035571464,14.7422571011955));
#48830=CARTESIAN_POINT('Ctrl Pts',(56.4605798585478,30.3586295807714,14.7450260981036));
#48831=CARTESIAN_POINT('Ctrl Pts',(56.4524867667053,30.3672783344635,14.7457701213043));
#48832=CARTESIAN_POINT('Ctrl Pts',(56.4387566114817,30.3816917061996,14.7470260632406));
#48833=CARTESIAN_POINT('Ctrl Pts',(56.4331606877759,30.3874952244938,14.7475362157439));
#48834=CARTESIAN_POINT('Ctrl Pts',(56.4220436102186,30.3988857095545,14.7485464149961));
#48835=CARTESIAN_POINT('Ctrl Pts',(56.4165243300478,30.4044743063722,14.7490463754638));
#48836=CARTESIAN_POINT('Ctrl Pts',(56.4042928118695,30.4167139974182,14.75015100402));
#48837=CARTESIAN_POINT('Ctrl Pts',(56.3975660605672,30.423350256699,14.7507563057259));
#48838=CARTESIAN_POINT('Ctrl Pts',(56.3737162199602,30.4465471860753,14.7528949600637));
#48839=CARTESIAN_POINT('Ctrl Pts',(56.3563444342309,30.4628481497572,14.7544393821512));
#48840=CARTESIAN_POINT('Ctrl Pts',(56.2213538722951,30.5850457478265,14.766345224979));
#48841=CARTESIAN_POINT('Ctrl Pts',(56.091819722919,30.6768978488232,14.777295261799));
#48842=CARTESIAN_POINT('Ctrl Pts',(55.8823443019209,30.7907911426206,14.7939126937327));
#48843=CARTESIAN_POINT('Ctrl Pts',(55.8096070013011,30.8248294247372,14.7994956919807));
#48844=CARTESIAN_POINT('Ctrl Pts',(55.712047432857,30.8634984069749,14.8066003386343));
#48845=CARTESIAN_POINT('Ctrl Pts',(55.6889132402556,30.8721742767818,14.8082576532146));
#48846=CARTESIAN_POINT('Ctrl Pts',(55.6499565973372,30.8859639884705,14.810996342969));
#48847=CARTESIAN_POINT('Ctrl Pts',(55.6342210924585,30.8913136686688,14.8120885510323));
#48848=CARTESIAN_POINT('Ctrl Pts',(55.6123282979792,30.8984527047916,14.8135870550372));
#48849=CARTESIAN_POINT('Ctrl Pts',(55.6062269937731,30.9004098114821,14.8140024204481));
#48850=CARTESIAN_POINT('Ctrl Pts',(55.5958776648937,30.9036746372742,14.8147030487002));
#48851=CARTESIAN_POINT('Ctrl Pts',(55.5916345383749,30.9049976090554,14.8149891831189));
#48852=CARTESIAN_POINT('Ctrl Pts',(55.5835017130842,30.9075035626529,14.815535437933));
#48853=CARTESIAN_POINT('Ctrl Pts',(55.5796127869433,30.9086888454212,14.8157956958974));
#48854=CARTESIAN_POINT('Ctrl Pts',(55.5692577525946,30.9118103285,14.8164862310585));
#48855=CARTESIAN_POINT('Ctrl Pts',(55.5627853258593,30.9137256337259,14.8169153115698));
#48856=CARTESIAN_POINT('Ctrl Pts',(55.5394624277458,30.9204987324453,14.8184527635663));
#48857=CARTESIAN_POINT('Ctrl Pts',(55.5225572277172,30.925167287593,14.8195508502358));
#48858=CARTESIAN_POINT('Ctrl Pts',(55.2914919004626,30.9857104175249,14.8343660863571));
#48859=CARTESIAN_POINT('Ctrl Pts',(55.0695206893635,31.0057952110265,14.846496059263));
#48860=CARTESIAN_POINT('Ctrl Pts',(54.8119480454818,30.9862090764469,14.8619981961419));
#48861=CARTESIAN_POINT('Ctrl Pts',(54.7752291828745,30.9823894354443,14.8642373229086));
#48862=CARTESIAN_POINT('Ctrl Pts',(54.7125864811099,30.9741103358519,14.8681217300302));
#48863=CARTESIAN_POINT('Ctrl Pts',(54.6866056030445,30.9701527862442,14.869751877021));
#48864=CARTESIAN_POINT('Ctrl Pts',(54.6499549078552,30.9638266585787,14.8720818428361));
#48865=CARTESIAN_POINT('Ctrl Pts',(54.6392140216405,30.9618817960723,14.8727683699272));
#48866=CARTESIAN_POINT('Ctrl Pts',(54.6207475921886,30.9583812880662,14.8739553091861));
#48867=CARTESIAN_POINT('Ctrl Pts',(54.6130142345525,30.9568678219887,14.8744543803629));
#48868=CARTESIAN_POINT('Ctrl Pts',(54.5982382282599,30.9538850521817,14.8754118726171));
#48869=CARTESIAN_POINT('Ctrl Pts',(54.5911941495911,30.9524233897456,14.8758700443441));
#48870=CARTESIAN_POINT('Ctrl Pts',(54.5746980224023,30.9489072198302,14.876947098327));
#48871=CARTESIAN_POINT('Ctrl Pts',(54.5652527704239,30.9468220166742,14.8775669473071));
#48872=CARTESIAN_POINT('Ctrl Pts',(54.5327938568077,30.939408157388,14.8797081708378));
#48873=CARTESIAN_POINT('Ctrl Pts',(54.5098606333127,30.9337396162421,14.8812402928767));
#48874=CARTESIAN_POINT('Ctrl Pts',(54.3382652637259,30.8880768436519,14.8928542988055));
#48875=CARTESIAN_POINT('Ctrl Pts',(54.1946057359321,30.8314065391958,14.9034896723543));
#48876=CARTESIAN_POINT('Ctrl Pts',(53.95550996692,30.7034737471099,14.9223898720556));
#48877=CARTESIAN_POINT('Ctrl Pts',(53.8571713263389,30.6391250578482,14.9305621243993));
#48878=CARTESIAN_POINT('Ctrl Pts',(53.7565545725706,30.5598038464128,14.9389783200573));
#48879=CARTESIAN_POINT('Ctrl Pts',(53.7481142292371,30.5530378616514,14.9396846612649));
#48880=CARTESIAN_POINT('Ctrl Pts',(53.7355510532793,30.5427979378009,14.9407360123452));
#48881=CARTESIAN_POINT('Ctrl Pts',(53.7313867463494,30.5393755324979,14.9410845003608));
#48882=CARTESIAN_POINT('Ctrl Pts',(53.7242434772513,30.5334562154517,14.941682201046));
#48883=CARTESIAN_POINT('Ctrl Pts',(53.7212578981565,30.5309674418176,14.9419319864272));
#48884=CARTESIAN_POINT('Ctrl Pts',(53.714476488922,30.5252807933089,14.9424992727809));
#48885=CARTESIAN_POINT('Ctrl Pts',(53.7106853119231,30.5220774725254,14.9428163734158));
#48886=CARTESIAN_POINT('Ctrl Pts',(53.7003885010503,30.5133111980925,14.9436776235038));
#48887=CARTESIAN_POINT('Ctrl Pts',(53.6939065657217,30.5077203910676,14.9442197957987));
#48888=CARTESIAN_POINT('Ctrl Pts',(53.6619900706613,30.4798314411295,14.9468906122155));
#48889=CARTESIAN_POINT('Ctrl Pts',(53.6370879056476,30.4569291686295,14.9489783049751));
#48890=CARTESIAN_POINT('Ctrl Pts',(53.4671678835173,30.2924836710184,14.96335221065));
#48891=CARTESIAN_POINT('Ctrl Pts',(53.3438682042306,30.130192216475,14.9745757778029));
#48892=CARTESIAN_POINT('Ctrl Pts',(53.2210529777984,29.9040795709367,14.9900312903674));
#48893=CARTESIAN_POINT('Ctrl Pts',(53.1969619226494,29.8550235447499,14.9933659389943));
#48894=CARTESIAN_POINT('Ctrl Pts',(53.1691731835517,29.7920247493577,14.9976571524138));
#48895=CARTESIAN_POINT('Ctrl Pts',(53.1635700945524,29.7789449411288,14.9985484981535));
#48896=CARTESIAN_POINT('Ctrl Pts',(53.1548144174318,29.757886077951,14.9999847391649));
#48897=CARTESIAN_POINT('Ctrl Pts',(53.151572468519,29.7499445302369,15.0005266210572));
#48898=CARTESIAN_POINT('Ctrl Pts',(53.1455112899721,29.7348188510598,15.0015593057555));
#48899=CARTESIAN_POINT('Ctrl Pts',(53.1426823269921,29.727638769101,15.0020497717463));
#48900=CARTESIAN_POINT('Ctrl Pts',(53.1363338799046,29.711247763869,15.0031700976402));
#48901=CARTESIAN_POINT('Ctrl Pts',(53.1328409068122,29.7020268540378,15.0038008258223));
#48902=CARTESIAN_POINT('Ctrl Pts',(53.1239363997985,29.6779837083138,15.0054468430742));
#48903=CARTESIAN_POINT('Ctrl Pts',(53.1186322052068,29.663122717046,15.0064656392795));
#48904=CARTESIAN_POINT('Ctrl Pts',(53.0860852110435,29.5683993679536,15.0129695959839));
#48905=CARTESIAN_POINT('Ctrl Pts',(53.0637744386948,29.4869905985863,15.0186105520578));
#48906=CARTESIAN_POINT('Ctrl Pts',(53.0466869327998,29.4044695588112,15.0243707259923));
#48907=CARTESIAN_POINT('Origin',(55.,29.,3.45145488139523));
#48908=CARTESIAN_POINT('',(53.0466870408509,29.4044700806242,15.9845144320741));
#48909=CARTESIAN_POINT('',(53.0466869980082,29.4044698737233,15.8273167122946));
#48910=CARTESIAN_POINT('',(53.0466869980082,29.4044698737233,3.45145488139523));
#48911=CARTESIAN_POINT('',(53.0052506493574,29.0017284253212,15.2092031079544));
#48912=CARTESIAN_POINT('Ctrl Pts',(53.0466870408509,29.4044700806242,15.9845144320741));
#48913=CARTESIAN_POINT('Ctrl Pts',(53.0534501350343,29.4371311849806,15.9822259750689));
#48914=CARTESIAN_POINT('Ctrl Pts',(53.0610339691148,29.4696302032199,15.9799208471347));
#48915=CARTESIAN_POINT('Ctrl Pts',(53.1040382957387,29.6350350901668,15.9680638067916));
#48916=CARTESIAN_POINT('Ctrl Pts',(53.1523155091381,29.7642026943096,15.9583574580738));
#48917=CARTESIAN_POINT('Ctrl Pts',(53.2238469535253,29.908211952473,15.9476090852829));
#48918=CARTESIAN_POINT('Ctrl Pts',(53.2345585205531,29.9288622557103,15.9460705215691));
#48919=CARTESIAN_POINT('Ctrl Pts',(53.2492230067567,29.9559626042592,15.9440595427439));
#48920=CARTESIAN_POINT('Ctrl Pts',(53.2528543757088,29.9625833744256,15.943568904757));
#48921=CARTESIAN_POINT('Ctrl Pts',(53.2588018968879,29.9732824469627,15.9427773021417));
#48922=CARTESIAN_POINT('Ctrl Pts',(53.2610949478323,29.9773734068887,15.9424749214682));
#48923=CARTESIAN_POINT('Ctrl Pts',(53.2655699058029,29.9852914376546,15.9418903069871));
#48924=CARTESIAN_POINT('Ctrl Pts',(53.2677500801846,29.9891193984707,15.9416079745063));
#48925=CARTESIAN_POINT('Ctrl Pts',(53.2730285419103,29.9983163678438,15.9409302996695));
#48926=CARTESIAN_POINT('Ctrl Pts',(53.2761392426007,30.0036782746023,15.9405357439184));
#48927=CARTESIAN_POINT('Ctrl Pts',(53.2870089281247,30.0222147109915,15.9391732866053));
#48928=CARTESIAN_POINT('Ctrl Pts',(53.2948945772483,30.0353148595139,15.938213124837));
#48929=CARTESIAN_POINT('Ctrl Pts',(53.343389813394,30.1138209627918,15.9324675225151));
#48930=CARTESIAN_POINT('Ctrl Pts',(53.3876118386438,30.1769288407111,15.9278833103945));
#48931=CARTESIAN_POINT('Ctrl Pts',(53.486728981154,30.3022642533455,15.9185110263194));
#48932=CARTESIAN_POINT('Ctrl Pts',(53.542074866669,30.3639413888214,15.913741320745));
#48933=CARTESIAN_POINT('Ctrl Pts',(53.6829839979068,30.5025619302817,15.9022121878352));
#48934=CARTESIAN_POINT('Ctrl Pts',(53.7716685449202,30.5758871146582,15.8954103428522));
#48935=CARTESIAN_POINT('Ctrl Pts',(53.8791629502807,30.6501519871727,15.8873025739885));
#48936=CARTESIAN_POINT('Ctrl Pts',(53.8922701190462,30.6589791322843,15.8863164312488));
#48937=CARTESIAN_POINT('Ctrl Pts',(53.9137297484089,30.6730636170399,15.8847051046488));
#48938=CARTESIAN_POINT('Ctrl Pts',(53.9220189414534,30.6784164435489,15.8840834696314));
#48939=CARTESIAN_POINT('Ctrl Pts',(53.9368620272109,30.687846196439,15.8829715330225));
#48940=CARTESIAN_POINT('Ctrl Pts',(53.9434005540701,30.6919470264057,15.8824821232514));
#48941=CARTESIAN_POINT('Ctrl Pts',(53.9572525233911,30.70052308865,15.8814460772464));
#48942=CARTESIAN_POINT('Ctrl Pts',(53.9645713334985,30.7049893101813,15.8808991251948));
#48943=CARTESIAN_POINT('Ctrl Pts',(53.9840974056889,30.7167327848268,15.8794409636563));
#48944=CARTESIAN_POINT('Ctrl Pts',(53.9963538553849,30.7239268936921,15.8785267777463));
#48945=CARTESIAN_POINT('Ctrl Pts',(54.0559112429152,30.7580346033474,15.8740889179072));
#48946=CARTESIAN_POINT('Ctrl Pts',(54.1042194388631,30.7831336168473,15.8705016855517));
#48947=CARTESIAN_POINT('Ctrl Pts',(54.3347580624309,30.891178503412,15.8534279706695));
#48948=CARTESIAN_POINT('Ctrl Pts',(54.5277408838768,30.9483460970599,15.8391144621655));
#48949=CARTESIAN_POINT('Ctrl Pts',(54.7618318124214,30.980811382159,15.8231176007144));
#48950=CARTESIAN_POINT('Ctrl Pts',(54.7978175241762,30.9848074088325,15.8207001693762));
#48951=CARTESIAN_POINT('Ctrl Pts',(54.8426205144947,30.9885512147939,15.8177577070384));
#48952=CARTESIAN_POINT('Ctrl Pts',(54.8513513611765,30.9892229199449,15.817187470535));
#48953=CARTESIAN_POINT('Ctrl Pts',(54.8650825849914,30.9901884175931,15.8162959156915));
#48954=CARTESIAN_POINT('Ctrl Pts',(54.8700800040111,30.9905208972444,15.8159725345064));
#48955=CARTESIAN_POINT('Ctrl Pts',(54.87934240885,30.9911020966014,15.815375264312));
#48956=CARTESIAN_POINT('Ctrl Pts',(54.8836069091706,30.9913559356111,15.8151011059494));
#48957=CARTESIAN_POINT('Ctrl Pts',(54.8933957273366,30.9919070501149,15.8144736724289));
#48958=CARTESIAN_POINT('Ctrl Pts',(54.8989204853775,30.9921950458559,15.8141209145496));
#48959=CARTESIAN_POINT('Ctrl Pts',(54.9159684543779,30.9930126250906,15.8130364009741));
#48960=CARTESIAN_POINT('Ctrl Pts',(54.9274953565567,30.993465253249,15.8123087558535));
#48961=CARTESIAN_POINT('Ctrl Pts',(55.0374492139618,30.9968278183815,15.805416124932));
#48962=CARTESIAN_POINT('Ctrl Pts',(55.1359744870044,30.9925461058079,15.7996054702781));
#48963=CARTESIAN_POINT('Ctrl Pts',(55.4071790849199,30.9605393757481,15.7836772705975));
#48964=CARTESIAN_POINT('Ctrl Pts',(55.5771099911548,30.9174066372552,15.7737027239332));
#48965=CARTESIAN_POINT('Ctrl Pts',(55.7598115976644,30.8445063784477,15.7615588943813));
#48966=CARTESIAN_POINT('Ctrl Pts',(55.7802302008728,30.8359624770948,15.7601818824313));
#48967=CARTESIAN_POINT('Ctrl Pts',(55.8097383194006,30.8230340387689,15.7581609173275));
#48968=CARTESIAN_POINT('Ctrl Pts',(55.8189438780761,30.8189173073606,15.7575259989864));
#48969=CARTESIAN_POINT('Ctrl Pts',(55.8351867585324,30.8115051803805,15.7563976322834));
#48970=CARTESIAN_POINT('Ctrl Pts',(55.8422368318634,30.8082381083408,15.7559051576322));
#48971=CARTESIAN_POINT('Ctrl Pts',(55.85685327556,30.8013606828087,15.7548783926994));
#48972=CARTESIAN_POINT('Ctrl Pts',(55.8644163210114,30.7977436596643,15.7543438807363));
#48973=CARTESIAN_POINT('Ctrl Pts',(55.8839589700011,30.7882455640918,15.7529542086075));
#48974=CARTESIAN_POINT('Ctrl Pts',(55.8959026011397,30.7822918316445,15.7520965508992));
#48975=CARTESIAN_POINT('Ctrl Pts',(55.9478661968136,30.7557344104761,15.748327764671));
#48976=CARTESIAN_POINT('Ctrl Pts',(55.9872392887986,30.7339007171338,15.7453740607433));
#48977=CARTESIAN_POINT('Ctrl Pts',(56.1613594710533,30.6294912511017,15.7318519517475));
#48978=CARTESIAN_POINT('Ctrl Pts',(56.2867291783249,30.5324199910015,15.7207727388125));
#48979=CARTESIAN_POINT('Ctrl Pts',(56.460691935294,30.3611849223542,15.703823897267));
#48980=CARTESIAN_POINT('Ctrl Pts',(56.518102047975,30.2968480913344,15.6979082115625));
#48981=CARTESIAN_POINT('Ctrl Pts',(56.5777142852303,30.2206382502073,15.6915534019287));
#48982=CARTESIAN_POINT('Ctrl Pts',(56.5841837717373,30.212230131959,15.6908606936952));
#48983=CARTESIAN_POINT('Ctrl Pts',(56.5938560517245,30.1994497951508,15.6898209049963));
#48984=CARTESIAN_POINT('Ctrl Pts',(56.5971084927256,30.1951156382712,15.6894705377689));
#48985=CARTESIAN_POINT('Ctrl Pts',(56.6029120278979,30.18731592684,15.6888441305743));
#48986=CARTESIAN_POINT('Ctrl Pts',(56.605469596442,30.1838553354578,15.6885676508327));
#48987=CARTESIAN_POINT('Ctrl Pts',(56.611039517791,30.1762675465147,15.6879645938516));
#48988=CARTESIAN_POINT('Ctrl Pts',(56.614047214767,30.1721370477773,15.6876383344927));
#48989=CARTESIAN_POINT('Ctrl Pts',(56.6225805559452,30.1603230022554,15.6867107748798));
#48990=CARTESIAN_POINT('Ctrl Pts',(56.6280675237954,30.1526115028084,15.6861120448344));
#48991=CARTESIAN_POINT('Ctrl Pts',(56.6647310587047,30.100299594614,15.6820934982729));
#48992=CARTESIAN_POINT('Ctrl Pts',(56.6941292149109,30.0544743047909,15.6787826600966));
#48993=CARTESIAN_POINT('Ctrl Pts',(56.8176808598636,29.8433488409794,15.6641769424767));
#48994=CARTESIAN_POINT('Ctrl Pts',(56.8897746777335,29.6663039204156,15.6535483530655));
#48995=CARTESIAN_POINT('Ctrl Pts',(56.9467241252387,29.4374617147852,15.6392995017148));
#48996=CARTESIAN_POINT('Ctrl Pts',(56.9562161822891,29.3928426336596,15.6365045817793));
#48997=CARTESIAN_POINT('Ctrl Pts',(56.9665989153019,29.3342306254704,15.6327932903754));
#48998=CARTESIAN_POINT('Ctrl Pts',(56.9688837792124,29.3204965727755,15.6319208657096));
#48999=CARTESIAN_POINT('Ctrl Pts',(56.9723333091103,29.2983308672023,15.6305078811102));
#49000=CARTESIAN_POINT('Ctrl Pts',(56.9735881319035,29.2899135570232,15.6299701606428));
#49001=CARTESIAN_POINT('Ctrl Pts',(56.9758802335732,29.2738332695984,15.6289406112517));
#49002=CARTESIAN_POINT('Ctrl Pts',(56.9769268937505,29.2661717697013,15.6284490866766));
#49003=CARTESIAN_POINT('Ctrl Pts',(56.9792231719078,29.248601956768,15.6273195320291));
#49004=CARTESIAN_POINT('Ctrl Pts',(56.9804429719575,29.2386900207149,15.6266805808522));
#49005=CARTESIAN_POINT('Ctrl Pts',(56.9839997451104,29.2078814544076,15.6246890254546));
#49006=CARTESIAN_POINT('Ctrl Pts',(56.9860807145653,29.1869572869407,15.6233284949867));
#49007=CARTESIAN_POINT('Ctrl Pts',(56.9945800824859,29.0851812835282,15.6166700943837));
#49008=CARTESIAN_POINT('Ctrl Pts',(56.996393345391,29.004031556856,15.6112319951362));
#49009=CARTESIAN_POINT('Ctrl Pts',(56.9880004560141,28.7867542701175,15.5963534135569));
#49010=CARTESIAN_POINT('Ctrl Pts',(56.9687821502761,28.6514132046081,15.5867284902775));
#49011=CARTESIAN_POINT('Ctrl Pts',(56.9330922752534,28.5077412321302,15.5765523338113));
#49012=CARTESIAN_POINT('Ctrl Pts',(56.9301718377433,28.4964117514736,15.575750404459));
#49013=CARTESIAN_POINT('Ctrl Pts',(56.9146388582822,28.4382744397134,15.5716399734323));
#49014=CARTESIAN_POINT('Ctrl Pts',(56.9004215788212,28.3919077080542,15.5683770756143));
#49015=CARTESIAN_POINT('Ctrl Pts',(56.8816726531832,28.3378735509759,15.5646279514439));
#49016=CARTESIAN_POINT('Ctrl Pts',(56.8787638608648,28.3296644348544,15.5640598538804));
#49017=CARTESIAN_POINT('Ctrl Pts',(56.8739430684001,28.3163372299478,15.5631402918558));
#49018=CARTESIAN_POINT('Ctrl Pts',(56.8720636785446,28.3112075842859,15.5627870123391));
#49019=CARTESIAN_POINT('Ctrl Pts',(56.8686653355209,28.3020487362003,15.5621575055048));
#49020=CARTESIAN_POINT('Ctrl Pts',(56.8671543920099,28.2980166808585,15.5618808189604));
#49021=CARTESIAN_POINT('Ctrl Pts',(56.8638342554452,28.2892432321268,15.5612797489023));
#49022=CARTESIAN_POINT('Ctrl Pts',(56.8620200237999,28.2845038454396,15.5609556673785));
#49023=CARTESIAN_POINT('Ctrl Pts',(56.8568292159944,28.2710971625509,15.5600405159956));
#49024=CARTESIAN_POINT('Ctrl Pts',(56.8534100218288,28.262446352638,15.5594519094221));
#49025=CARTESIAN_POINT('Ctrl Pts',(56.8309519575169,28.2067683237267,15.5556739162163));
#49026=CARTESIAN_POINT('Ctrl Pts',(56.8101835803972,28.1604537358058,15.5525790881391));
#49027=CARTESIAN_POINT('Ctrl Pts',(56.7199514788576,27.978192611782,15.5404008722918));
#49028=CARTESIAN_POINT('Ctrl Pts',(56.6367555386292,27.849625815281,15.5317757344369));
#49029=CARTESIAN_POINT('Ctrl Pts',(56.4875525998059,27.6684805830844,15.517916657112));
#49030=CARTESIAN_POINT('Ctrl Pts',(56.4315492555174,27.6084465321837,15.5129814421806));
#49031=CARTESIAN_POINT('Ctrl Pts',(56.3611385516219,27.5417291466275,15.506955369004));
#49032=CARTESIAN_POINT('Ctrl Pts',(56.3501473945844,27.5315470615806,15.5060195929095));
#49033=CARTESIAN_POINT('Ctrl Pts',(56.3319128979894,27.5150326173022,15.5044744510278));
#49034=CARTESIAN_POINT('Ctrl Pts',(56.3247364724658,27.5086270188727,15.5038681616673));
#49035=CARTESIAN_POINT('Ctrl Pts',(56.3117381518173,27.4971927065506,15.5027731176742));
#49036=CARTESIAN_POINT('Ctrl Pts',(56.3059329314384,27.4921452602886,15.5022851512732));
#49037=CARTESIAN_POINT('Ctrl Pts',(56.2934817572786,27.4814452182999,15.5012407892012));
#49038=CARTESIAN_POINT('Ctrl Pts',(56.2868276418939,27.4758024086326,15.5006840078356));
#49039=CARTESIAN_POINT('Ctrl Pts',(56.2687115359405,27.4606428144417,15.499171627257));
#49040=CARTESIAN_POINT('Ctrl Pts',(56.2571797806631,27.4512106387898,15.4982126490977));
#49041=CARTESIAN_POINT('Ctrl Pts',(56.1959274170714,27.4022452814668,15.4931372888402));
#49042=CARTESIAN_POINT('Ctrl Pts',(56.1444500015157,27.3649785179587,15.4889330350341));
#49043=CARTESIAN_POINT('Ctrl Pts',(55.9714154918429,27.2518906334691,15.4749868454011));
#49044=CARTESIAN_POINT('Ctrl Pts',(55.843464214561,27.1866897421248,15.4649205047184));
#49045=CARTESIAN_POINT('Ctrl Pts',(55.6353437436458,27.1074649680234,15.4494865270663));
#49046=CARTESIAN_POINT('Ctrl Pts',(55.5593948870377,27.0836412670851,15.4440426721734));
#49047=CARTESIAN_POINT('Ctrl Pts',(55.4720000030585,27.0618683069888,15.4381280082817));
#49048=CARTESIAN_POINT('Ctrl Pts',(55.4617611815757,27.0594034203216,15.4374404415707));
#49049=CARTESIAN_POINT('Ctrl Pts',(55.4462411529914,27.0557969296875,15.4364068284634));
#49050=CARTESIAN_POINT('Ctrl Pts',(55.4409742285562,27.0545955493417,15.4360575516247));
#49051=CARTESIAN_POINT('Ctrl Pts',(55.4315040594452,27.0524758490768,15.4354322959159));
#49052=CARTESIAN_POINT('Ctrl Pts',(55.4273026843721,27.0515497212559,15.4351558845729));
#49053=CARTESIAN_POINT('Ctrl Pts',(55.418091824202,27.0495505559698,15.4345520429127));
#49054=CARTESIAN_POINT('Ctrl Pts',(55.4130811973027,27.0484832224577,15.4342249366142));
#49055=CARTESIAN_POINT('Ctrl Pts',(55.3987405173231,27.0454861642834,15.4332925347245));
#49056=CARTESIAN_POINT('Ctrl Pts',(55.3894005251443,27.0436039323051,15.4326898516438));
#49057=CARTESIAN_POINT('Ctrl Pts',(55.325107144906,27.0311259542079,15.4285704144821));
#49058=CARTESIAN_POINT('Ctrl Pts',(55.269737052041,27.0227790114455,15.4251690080409));
#49059=CARTESIAN_POINT('Ctrl Pts',(55.0042995182457,26.9941257679317,15.4092468672784));
#49060=CARTESIAN_POINT('Ctrl Pts',(54.7922557163921,27.0049055286503,15.3975101998206));
#49061=CARTESIAN_POINT('Ctrl Pts',(54.5582014891221,27.0545850658182,15.382836870463));
#49062=CARTESIAN_POINT('Ctrl Pts',(54.530703447624,27.0610348601485,15.3810881705825));
#49063=CARTESIAN_POINT('Ctrl Pts',(54.4921638618881,27.0709423334816,15.3785980930345));
#49064=CARTESIAN_POINT('Ctrl Pts',(54.4810004990371,27.0739157513201,15.3778721463226));
#49065=CARTESIAN_POINT('Ctrl Pts',(54.4629202958088,27.0789000989385,15.376688541359));
#49066=CARTESIAN_POINT('Ctrl Pts',(54.4559873073951,27.0808518487103,15.3762327931316));
#49067=CARTESIAN_POINT('Ctrl Pts',(54.4414986093018,27.0850154728945,15.3752763365451));
#49068=CARTESIAN_POINT('Ctrl Pts',(54.4339451336591,27.0872346124377,15.374775400383));
#49069=CARTESIAN_POINT('Ctrl Pts',(54.4159893938189,27.0926255113846,15.373579016903));
#49070=CARTESIAN_POINT('Ctrl Pts',(54.4055996284835,27.095837712119,15.3728822684409));
#49071=CARTESIAN_POINT('Ctrl Pts',(54.371265208435,27.1067612598061,15.3705645862299));
#49072=CARTESIAN_POINT('Ctrl Pts',(54.3474409678094,27.1148403304547,15.3689317570972));
#49073=CARTESIAN_POINT('Ctrl Pts',(54.2905365306493,27.135345199287,15.3649704802703));
#49074=CARTESIAN_POINT('Ctrl Pts',(54.2576222284266,27.1482033232074,15.3626285420471));
#49075=CARTESIAN_POINT('Ctrl Pts',(54.130245812673,27.201905258266,15.3533645567618));
#49076=CARTESIAN_POINT('Ctrl Pts',(54.0386690722697,27.2491557563958,15.3462532360143));
#49077=CARTESIAN_POINT('Ctrl Pts',(53.8752255940669,27.3501883854994,15.3328686656728));
#49078=CARTESIAN_POINT('Ctrl Pts',(53.8025292375411,27.4021699292104,15.3266267412755));
#49079=CARTESIAN_POINT('Ctrl Pts',(53.6995333120882,27.4868069335144,15.3175483810126));
#49080=CARTESIAN_POINT('Ctrl Pts',(53.6664419616967,27.5158873090291,15.3145923673441));
#49081=CARTESIAN_POINT('Ctrl Pts',(53.6281598744205,27.5518445960922,15.3111513013047));
#49082=CARTESIAN_POINT('Ctrl Pts',(53.6220187445413,27.5576869030329,15.3105986162566));
#49083=CARTESIAN_POINT('Ctrl Pts',(53.6120318939036,27.5673098116783,15.3096989903351));
#49084=CARTESIAN_POINT('Ctrl Pts',(53.6081640073724,27.5710671077591,15.3093503589827));
#49085=CARTESIAN_POINT('Ctrl Pts',(53.601237937294,27.5778499518201,15.3087257825006));
#49086=CARTESIAN_POINT('Ctrl Pts',(53.5981742763906,27.5808697349148,15.308449409225));
#49087=CARTESIAN_POINT('Ctrl Pts',(53.5914776804509,27.5875132687538,15.3078450921271));
#49088=CARTESIAN_POINT('Ctrl Pts',(53.5878489549749,27.5911411291165,15.3075174760076));
#49089=CARTESIAN_POINT('Ctrl Pts',(53.5782661296107,27.600795891496,15.3066517625548));
#49090=CARTESIAN_POINT('Ctrl Pts',(53.572336281025,27.6068468687897,15.3061155051506));
#49091=CARTESIAN_POINT('Ctrl Pts',(53.5362854811462,27.6441059908498,15.3028504882215));
#49092=CARTESIAN_POINT('Ctrl Pts',(53.5071480075697,27.6762544377816,15.3001907736147));
#49093=CARTESIAN_POINT('Ctrl Pts',(53.4119825141931,27.7883970691601,15.2913279090634));
#49094=CARTESIAN_POINT('Ctrl Pts',(53.3511480315519,27.87258188765,15.285348102138));
#49095=CARTESIAN_POINT('Ctrl Pts',(53.2314424707286,28.068795988012,15.2719943369466));
#49096=CARTESIAN_POINT('Ctrl Pts',(53.1761208474975,28.182444958832,15.2646170027063));
#49097=CARTESIAN_POINT('Ctrl Pts',(53.1233638528613,28.3233486405983,15.2553547423411));
#49098=CARTESIAN_POINT('Ctrl Pts',(53.1152454490691,28.34630244452,15.2538433016772));
#49099=CARTESIAN_POINT('Ctrl Pts',(53.10445248795,28.3786923770328,15.2517043961847));
#49100=CARTESIAN_POINT('Ctrl Pts',(53.1014240848476,28.3880089692199,15.2510884670508));
#49101=CARTESIAN_POINT('Ctrl Pts',(53.0962817208661,28.4042345478716,15.250014401317));
#49102=CARTESIAN_POINT('Ctrl Pts',(53.0941364250883,28.411133468548,15.2495572917936));
#49103=CARTESIAN_POINT('Ctrl Pts',(53.0897372543244,28.4255563614228,15.2486006907876));
#49104=CARTESIAN_POINT('Ctrl Pts',(53.087490248292,28.4330822827254,15.2481009858164));
#49105=CARTESIAN_POINT('Ctrl Pts',(53.0822672106087,28.4509603538222,15.2469125324399));
#49106=CARTESIAN_POINT('Ctrl Pts',(53.0793304922248,28.4613236416942,15.2462225282671));
#49107=CARTESIAN_POINT('Ctrl Pts',(53.0733145933244,28.4832277387007,15.2447616236886));
#49108=CARTESIAN_POINT('Ctrl Pts',(53.0702548607665,28.4947734035954,15.24399012784));
#49109=CARTESIAN_POINT('Ctrl Pts',(53.0579613454037,28.5429036158068,15.2407676024948));
#49110=CARTESIAN_POINT('Ctrl Pts',(53.0496633357835,28.579716974646,15.238287252437));
#49111=CARTESIAN_POINT('Ctrl Pts',(53.0175812102494,28.7435842007438,15.2271734272461));
#49112=CARTESIAN_POINT('Ctrl Pts',(53.0051388531737,28.872519698558,15.2182084608135));
#49113=CARTESIAN_POINT('Ctrl Pts',(53.005250747999,29.0017274667166,15.2092030022871));
#49114=CARTESIAN_POINT('Ctrl Pts',(53.0052507488189,29.0017284132713,15.2092029363146));
#49115=CARTESIAN_POINT('Ctrl Pts',(53.0053490353139,29.1151601460515,15.2012970280619));
#49116=CARTESIAN_POINT('Ctrl Pts',(53.0151226269909,29.2283926494983,15.1933979671947));
#49117=CARTESIAN_POINT('Ctrl Pts',(53.0359402980613,29.3486704232499,15.185359270907));
#49118=CARTESIAN_POINT('Ctrl Pts',(53.0374623744913,29.3571381404936,15.1847953083819));
#49119=CARTESIAN_POINT('Ctrl Pts',(53.0400384497655,29.3709555337908,15.1838785633237));
#49120=CARTESIAN_POINT('Ctrl Pts',(53.0410596639462,29.3763111051693,15.1835241010534));
#49121=CARTESIAN_POINT('Ctrl Pts',(53.0430796951611,29.3866736988947,15.1828400092167));
#49122=CARTESIAN_POINT('Ctrl Pts',(53.0440758022868,29.3916812008686,15.1825102357848));
#49123=CARTESIAN_POINT('Ctrl Pts',(53.045617923212,29.3992809505369,15.1820110196316));
#49124=CARTESIAN_POINT('Ctrl Pts',(53.0461498747513,29.4018759355602,15.1818407854086));
#49125=CARTESIAN_POINT('Ctrl Pts',(53.0466869980082,29.4044698737233,15.1816708487869));
#49126=CARTESIAN_POINT('Ctrl Pts',(53.0466869327998,29.4044695588112,15.0243707259923));
#49127=CARTESIAN_POINT('Ctrl Pts',(53.0376291222587,29.360726490131,15.0274241010433));
#49128=CARTESIAN_POINT('Ctrl Pts',(53.0300389624832,29.3166708117229,15.0305098276839));
#49129=CARTESIAN_POINT('Ctrl Pts',(53.0114370908261,29.1817155653926,15.0399673408109));
#49130=CARTESIAN_POINT('Ctrl Pts',(53.0051945752177,29.0903027661733,15.0463852547253));
#49131=CARTESIAN_POINT('Ctrl Pts',(53.005258330144,28.9857281837005,15.0535820183753));
#49132=CARTESIAN_POINT('Ctrl Pts',(53.0053944644802,28.9726726926802,15.0544777782754));
#49133=CARTESIAN_POINT('Ctrl Pts',(53.0066601161836,28.9101641215504,15.0587510993224));
#49134=CARTESIAN_POINT('Ctrl Pts',(53.0095007899479,28.8607585952538,15.0620825136977));
#49135=CARTESIAN_POINT('Ctrl Pts',(53.015003364643,28.8027879233336,15.06589997914));
#49136=CARTESIAN_POINT('Ctrl Pts',(53.0158882634707,28.7940755740842,15.0664712486255));
#49137=CARTESIAN_POINT('Ctrl Pts',(53.0174198902035,28.7799234829607,15.067394907984));
#49138=CARTESIAN_POINT('Ctrl Pts',(53.0180316898803,28.7744801904085,15.0677491390117));
#49139=CARTESIAN_POINT('Ctrl Pts',(53.0191645775542,28.7647615238637,15.0683796656477));
#49140=CARTESIAN_POINT('Ctrl Pts',(53.0196770963515,28.7604852615998,15.0686564268264));
#49141=CARTESIAN_POINT('Ctrl Pts',(53.02082234174,28.7511848059899,15.0692568798577));
#49142=CARTESIAN_POINT('Ctrl Pts',(53.0214603495527,28.7461613569629,15.0695802747634));
#49143=CARTESIAN_POINT('Ctrl Pts',(53.0233179578874,28.7319678328385,15.0704915273097));
#49144=CARTESIAN_POINT('Ctrl Pts',(53.0245822472553,28.7228035927355,15.0710769548237));
#49145=CARTESIAN_POINT('Ctrl Pts',(53.0330382705838,28.6645083316185,15.0747841463435));
#49146=CARTESIAN_POINT('Ctrl Pts',(53.0419992811613,28.6156470413761,15.0778153908479));
#49147=CARTESIAN_POINT('Ctrl Pts',(53.0840940814233,28.4262714373364,15.0894423992174));
#49148=CARTESIAN_POINT('Ctrl Pts',(53.1306133781078,28.2891841467318,15.0976228415291));
#49149=CARTESIAN_POINT('Ctrl Pts',(53.2298702494432,28.0759181891185,15.1114576526866));
#49150=CARTESIAN_POINT('Ctrl Pts',(53.2737978282334,27.9962522544171,15.1169018513406));
#49151=CARTESIAN_POINT('Ctrl Pts',(53.3312822318091,27.9070029308792,15.123494153909));
#49152=CARTESIAN_POINT('Ctrl Pts',(53.3397132761916,27.8942380195203,15.1244493039887));
#49153=CARTESIAN_POINT('Ctrl Pts',(53.3537372969032,27.8735271597694,15.1260199269429));
#49154=CARTESIAN_POINT('Ctrl Pts',(53.3592430846853,27.8655227252657,15.1266321452406));
#49155=CARTESIAN_POINT('Ctrl Pts',(53.3692179839382,27.8512455029686,15.1277336605262));
#49156=CARTESIAN_POINT('Ctrl Pts',(53.3736653957638,27.8449577363907,15.1282221292872));
#49157=CARTESIAN_POINT('Ctrl Pts',(53.38319256003,27.8316523144574,15.1292630115287));
#49158=CARTESIAN_POINT('Ctrl Pts',(53.3882818263358,27.8246416984359,15.1298157825676));
#49159=CARTESIAN_POINT('Ctrl Pts',(53.4020806255106,27.8058915860757,15.1313060119466));
#49160=CARTESIAN_POINT('Ctrl Pts',(53.4108736669392,27.7942144840833,15.1322466822229));
#49161=CARTESIAN_POINT('Ctrl Pts',(53.4561611198195,27.7354288929138,15.1370476690013));
#49162=CARTESIAN_POINT('Ctrl Pts',(53.4946217080038,27.6898803311271,15.1409848655225));
#49163=CARTESIAN_POINT('Ctrl Pts',(53.6201292770321,27.5540767633319,15.1534290333));
#49164=CARTESIAN_POINT('Ctrl Pts',(53.7136770413483,27.4702601931502,15.1621765930002));
#49165=CARTESIAN_POINT('Ctrl Pts',(53.8321937887245,27.3826742081028,15.1724379731407));
#49166=CARTESIAN_POINT('Ctrl Pts',(53.8501486889396,27.3698601140367,15.173971687895));
#49167=CARTESIAN_POINT('Ctrl Pts',(53.9339655076504,27.3121154789667,15.1810263965228));
#49168=CARTESIAN_POINT('Ctrl Pts',(54.0022790661451,27.270855829103,15.1864850847642));
#49169=CARTESIAN_POINT('Ctrl Pts',(54.082213250937,27.2288969523772,15.1924136502432));
#49170=CARTESIAN_POINT('Ctrl Pts',(54.0915789911015,27.2240749440972,15.1931014046576));
#49171=CARTESIAN_POINT('Ctrl Pts',(54.1058056185925,27.2168922747006,15.1941352431392));
#49172=CARTESIAN_POINT('Ctrl Pts',(54.1106384482421,27.2144768879472,15.1944845596983));
#49173=CARTESIAN_POINT('Ctrl Pts',(54.1193372725627,27.2101734071464,15.1951098570643));
#49174=CARTESIAN_POINT('Ctrl Pts',(54.1231995988337,27.2082781662431,15.1953862706113));
#49175=CARTESIAN_POINT('Ctrl Pts',(54.1316740624742,27.204153718096,15.1959900826017));
#49176=CARTESIAN_POINT('Ctrl Pts',(54.1362886588485,27.2019297781827,15.196317157254));
#49177=CARTESIAN_POINT('Ctrl Pts',(54.1495082651488,27.1956214094208,15.1972493787525));
#49178=CARTESIAN_POINT('Ctrl Pts',(54.158134171207,27.1915807388752,15.1978519146674));
#49179=CARTESIAN_POINT('Ctrl Pts',(54.2175845710579,27.164249693858,15.2019675270229));
#49180=CARTESIAN_POINT('Ctrl Pts',(54.2693447546239,27.1430408594128,15.2053655007225));
#49181=CARTESIAN_POINT('Ctrl Pts',(54.4123228501189,27.0913614894308,15.2144327433584));
#49182=CARTESIAN_POINT('Ctrl Pts',(54.5049609822851,27.0652639078608,15.2199709222166));
#49183=CARTESIAN_POINT('Ctrl Pts',(54.7279497816268,27.0195175219057,15.2332051288297));
#49184=CARTESIAN_POINT('Ctrl Pts',(54.8590548620189,27.0058961729545,15.2409290077794));
#49185=CARTESIAN_POINT('Ctrl Pts',(55.0062864408515,27.0051977337203,15.2500662951122));
#49186=CARTESIAN_POINT('Ctrl Pts',(55.0220354675471,27.0053095435629,15.2510491834752));
#49187=CARTESIAN_POINT('Ctrl Pts',(55.0476308021818,27.0057944140287,15.2526562393269));
#49188=CARTESIAN_POINT('Ctrl Pts',(55.0574787656746,27.0060539630259,15.2532768894091));
#49189=CARTESIAN_POINT('Ctrl Pts',(55.0750361561066,27.0066468755158,15.2543877281854));
#49190=CARTESIAN_POINT('Ctrl Pts',(55.0827463833307,27.0069520485085,15.2548770317168));
#49191=CARTESIAN_POINT('Ctrl Pts',(55.099028542845,27.0076911447072,15.2559135461434));
#49192=CARTESIAN_POINT('Ctrl Pts',(55.107599813629,27.0081356714095,15.2564610770654));
#49193=CARTESIAN_POINT('Ctrl Pts',(55.1303957097441,27.0094654882322,15.2579224268753));
#49194=CARTESIAN_POINT('Ctrl Pts',(55.144613961042,27.010447922634,15.2588392452766));
#49195=CARTESIAN_POINT('Ctrl Pts',(55.2135564245036,27.0159545398855,15.2633115950144));
#49196=CARTESIAN_POINT('Ctrl Pts',(55.26808394779,27.0225843209741,15.2669318907946));
#49197=CARTESIAN_POINT('Ctrl Pts',(55.525689021111,27.0647560464535,15.2844429337309));
#49198=CARTESIAN_POINT('Ctrl Pts',(55.7226781541907,27.1293767307577,15.2992176856752));
#49199=CARTESIAN_POINT('Ctrl Pts',(55.9335362417546,27.2369131548663,15.3151598451062));
#49200=CARTESIAN_POINT('Ctrl Pts',(55.9604914490807,27.2514515855585,15.3171967860309));
#49201=CARTESIAN_POINT('Ctrl Pts',(55.9943719038012,27.2707452319232,15.319745894495));
#49202=CARTESIAN_POINT('Ctrl Pts',(56.0016149641621,27.2749304346016,15.3202901847875));
#49203=CARTESIAN_POINT('Ctrl Pts',(56.0130332067034,27.2816243120533,15.3211469098));
#49204=CARTESIAN_POINT('Ctrl Pts',(56.0172257990867,27.2841028708837,15.3214612023679));
#49205=CARTESIAN_POINT('Ctrl Pts',(56.0251364000081,27.2888186094297,15.3220536131763));
#49206=CARTESIAN_POINT('Ctrl Pts',(56.0288561464624,27.2910525402203,15.3223319191023));
#49207=CARTESIAN_POINT('Ctrl Pts',(56.0375170010559,27.2962924301282,15.3229793531829));
#49208=CARTESIAN_POINT('Ctrl Pts',(56.0424523559679,27.299307758982,15.3233478704364));
#49209=CARTESIAN_POINT('Ctrl Pts',(56.0583285469679,27.3091026318202,15.3245322018731));
#49210=CARTESIAN_POINT('Ctrl Pts',(56.0692171646043,27.3159667763766,15.3253427380342));
#49211=CARTESIAN_POINT('Ctrl Pts',(56.0948972803195,27.3325049197619,15.3272521025473));
#49212=CARTESIAN_POINT('Ctrl Pts',(56.1096283706402,27.3422711857799,15.328345602296));
#49213=CARTESIAN_POINT('Ctrl Pts',(56.1631489071019,27.3787868295846,15.3323194392121));
#49214=CARTESIAN_POINT('Ctrl Pts',(56.2011192174906,27.4067138528786,15.3351407445395));
#49215=CARTESIAN_POINT('Ctrl Pts',(56.3644628416342,27.5360139565463,15.3474546357497));
#49216=CARTESIAN_POINT('Ctrl Pts',(56.478262811641,27.6510168399532,15.3565659347542));
#49217=CARTESIAN_POINT('Ctrl Pts',(56.6116750995397,27.8232501927843,15.3696245467974));
#49218=CARTESIAN_POINT('Ctrl Pts',(56.6444395921615,27.8694893740611,15.3730758778743));
#49219=CARTESIAN_POINT('Ctrl Pts',(56.6832475001944,27.9295208172102,15.3775260676406));
#49220=CARTESIAN_POINT('Ctrl Pts',(56.6911652830976,27.9420738237988,15.3784549456834));
#49221=CARTESIAN_POINT('Ctrl Pts',(56.7035518898214,27.9622062301939,15.3799425790555));
#49222=CARTESIAN_POINT('Ctrl Pts',(56.7081120149612,27.9697290209262,15.3804979968454));
#49223=CARTESIAN_POINT('Ctrl Pts',(56.716561936661,27.9838790780014,15.3815419780149));
#49224=CARTESIAN_POINT('Ctrl Pts',(56.7204634999068,27.9904991563575,15.3820301037449));
#49225=CARTESIAN_POINT('Ctrl Pts',(56.7291102541959,28.0053664876959,15.3831257522241));
#49226=CARTESIAN_POINT('Ctrl Pts',(56.7338348578466,28.0136254385232,15.3837339993377));
#49227=CARTESIAN_POINT('Ctrl Pts',(56.7476335180598,28.03815197783,15.3855393231576));
#49228=CARTESIAN_POINT('Ctrl Pts',(56.7565388008986,28.0545128592441,15.3867423394837));
#49229=CARTESIAN_POINT('Ctrl Pts',(56.825706938564,28.185940143541,15.3963990124893));
#49230=CARTESIAN_POINT('Ctrl Pts',(56.8748178513817,28.3064972601989,15.4052445394534));
#49231=CARTESIAN_POINT('Ctrl Pts',(56.9528892802432,28.5687966936549,15.4242542246605));
#49232=CARTESIAN_POINT('Ctrl Pts',(56.9788923783932,28.7106847281869,15.4344034918505));
#49233=CARTESIAN_POINT('Ctrl Pts',(56.9904672661758,28.8685595625478,15.444867303577));
#49234=CARTESIAN_POINT('Ctrl Pts',(56.9913675577762,28.8829880137083,15.4458157475121));
#49235=CARTESIAN_POINT('Ctrl Pts',(56.9924004720642,28.9030483516967,15.4471223244563));
#49236=CARTESIAN_POINT('Ctrl Pts',(56.9926661930258,28.9086725221637,15.4474873222747));
#49237=CARTESIAN_POINT('Ctrl Pts',(56.9930826344096,28.9183564000096,15.4481134330865));
#49238=CARTESIAN_POINT('Ctrl Pts',(56.9932447712145,28.9224155444112,15.4483751652129));
#49239=CARTESIAN_POINT('Ctrl Pts',(56.9935584386156,28.9309196528592,15.4489219764759));
#49240=CARTESIAN_POINT('Ctrl Pts',(56.993707505286,28.9353646658576,15.4492069094866));
#49241=CARTESIAN_POINT('Ctrl Pts',(56.9940354922301,28.9462295261276,15.4499012935754));
#49242=CARTESIAN_POINT('Ctrl Pts',(56.994198279306,28.9526498821564,15.4503098580233));
#49243=CARTESIAN_POINT('Ctrl Pts',(56.9946730631908,28.9757844855206,15.4517760403744));
#49244=CARTESIAN_POINT('Ctrl Pts',(56.9948059672532,28.9925022509453,15.4528242552352));
#49245=CARTESIAN_POINT('Ctrl Pts',(56.9946135989172,29.0341191891389,15.4554099233105));
#49246=CARTESIAN_POINT('Ctrl Pts',(56.9940323189497,29.0590148665882,15.4569355487784));
#49247=CARTESIAN_POINT('Ctrl Pts',(56.9895650880044,29.165138032552,15.4633730860939));
#49248=CARTESIAN_POINT('Ctrl Pts',(56.981180216457,29.2461032509164,15.4681220971931));
#49249=CARTESIAN_POINT('Ctrl Pts',(56.9422466077599,29.4808812464962,15.4819584700742));
#49250=CARTESIAN_POINT('Ctrl Pts',(56.8985065291685,29.6318508819898,15.4909856366232));
#49251=CARTESIAN_POINT('Ctrl Pts',(56.8283669327761,29.7979098839537,15.5020932747695));
#49252=CARTESIAN_POINT('Ctrl Pts',(56.8187879330774,29.8195097346748,15.50356116403));
#49253=CARTESIAN_POINT('Ctrl Pts',(56.80479022424,29.8496184656033,15.5056422782307));
#49254=CARTESIAN_POINT('Ctrl Pts',(56.8006901748169,29.8582739538353,15.5062446638891));
#49255=CARTESIAN_POINT('Ctrl Pts',(56.7934115569063,29.8733578724643,15.5073018244246));
#49256=CARTESIAN_POINT('Ctrl Pts',(56.7902603349002,29.8797993617595,15.507755652913));
#49257=CARTESIAN_POINT('Ctrl Pts',(56.7835638454093,29.8933028667214,15.5087121037417));
#49258=CARTESIAN_POINT('Ctrl Pts',(56.7800112178942,29.9003610740036,15.5092149751998));
#49259=CARTESIAN_POINT('Ctrl Pts',(56.7713975869396,29.9172240164427,15.5104235594198));
#49260=CARTESIAN_POINT('Ctrl Pts',(56.766297028686,29.9270081476235,15.5111306434992));
#49261=CARTESIAN_POINT('Ctrl Pts',(56.748432962206,29.960593106725,15.5135783306971));
#49262=CARTESIAN_POINT('Ctrl Pts',(56.7352679005363,29.9841758661671,15.5153329787346));
#49263=CARTESIAN_POINT('Ctrl Pts',(56.7023055933076,30.0405032114287,15.5196137407792));
#49264=CARTESIAN_POINT('Ctrl Pts',(56.6820377059062,30.0729585755317,15.5221558557782));
#49265=CARTESIAN_POINT('Ctrl Pts',(56.5982478551581,30.1989191153789,15.5323255567253));
#49266=CARTESIAN_POINT('Ctrl Pts',(56.5277661155212,30.2875281498299,15.5401781797339));
#49267=CARTESIAN_POINT('Ctrl Pts',(56.3762794460756,30.4479167359367,15.5555547476907));
#49268=CARTESIAN_POINT('Ctrl Pts',(56.2961709985651,30.520050409855,15.5630480774395));
#49269=CARTESIAN_POINT('Ctrl Pts',(56.1978656022446,30.5951186077054,15.5712424467446));
#49270=CARTESIAN_POINT('Ctrl Pts',(56.1849866435476,30.6047093404324,15.572297617456));
#49271=CARTESIAN_POINT('Ctrl Pts',(56.1667281799059,30.6179663917015,15.5737663453386));
#49272=CARTESIAN_POINT('Ctrl Pts',(56.1614447964174,30.6217632004028,15.5741881974828));
#49273=CARTESIAN_POINT('Ctrl Pts',(56.1528669377008,30.6278641057177,15.5748678964775));
#49274=CARTESIAN_POINT('Ctrl Pts',(56.1495839610035,30.630184173653,15.5751268126029));
#49275=CARTESIAN_POINT('Ctrl Pts',(56.1426170368713,30.6350761618882,15.5756736447723));
#49276=CARTESIAN_POINT('Ctrl Pts',(56.1389313692111,30.637645592038,15.5759613861409));
#49277=CARTESIAN_POINT('Ctrl Pts',(56.1297719580966,30.6439851154093,15.5766727251106));
#49278=CARTESIAN_POINT('Ctrl Pts',(56.1242879366608,30.6477403847283,15.577095332943));
#49279=CARTESIAN_POINT('Ctrl Pts',(56.1036760748113,30.6617038655529,15.5786718391155));
#49280=CARTESIAN_POINT('Ctrl Pts',(56.0884266084257,30.6717320922745,15.5798143755022));
#49281=CARTESIAN_POINT('Ctrl Pts',(56.0494277507255,30.6966182829233,15.5826822258811));
#49282=CARTESIAN_POINT('Ctrl Pts',(56.0254984834328,30.7111882481179,15.5843921240233));
#49283=CARTESIAN_POINT('Ctrl Pts',(55.9144181694639,30.7756550107634,15.5921415723413));
#49284=CARTESIAN_POINT('Ctrl Pts',(55.8238783142742,30.8194336799641,15.5979433860182));
#49285=CARTESIAN_POINT('Ctrl Pts',(55.6084960152647,30.9041868501124,15.6113859764733));
#49286=CARTESIAN_POINT('Ctrl Pts',(55.4821567912092,30.940029454509,15.6190312079532));
#49287=CARTESIAN_POINT('Ctrl Pts',(55.3292675381673,30.9675372734213,15.6285944111241));
#49288=CARTESIAN_POINT('Ctrl Pts',(55.3052354230689,30.9714084535927,15.6301055298876));
#49289=CARTESIAN_POINT('Ctrl Pts',(55.2714415011369,30.9762193771607,15.6322440523846));
#49290=CARTESIAN_POINT('Ctrl Pts',(55.2617338360955,30.9775284849541,15.6328599259822));
#49291=CARTESIAN_POINT('Ctrl Pts',(55.2448503756882,30.9796787745711,15.6339339219029));
#49292=CARTESIAN_POINT('Ctrl Pts',(55.2376788645123,30.9805525774661,15.6343910174821));
#49293=CARTESIAN_POINT('Ctrl Pts',(55.2227010559496,30.9822950067479,15.6353476157858));
#49294=CARTESIAN_POINT('Ctrl Pts',(55.214894071865,30.9831565215827,15.6358473321383));
#49295=CARTESIAN_POINT('Ctrl Pts',(55.1963681511624,30.9850902133622,15.6370358610923));
#49296=CARTESIAN_POINT('Ctrl Pts',(55.1856453028863,30.9861217032208,15.6377259298965));
#49297=CARTESIAN_POINT('Ctrl Pts',(55.149595684472,30.9892950305221,15.6400533929149));
#49298=CARTESIAN_POINT('Ctrl Pts',(55.1242373064698,30.9910395728451,15.6417030422273));
#49299=CARTESIAN_POINT('Ctrl Pts',(55.0635576408155,30.9940503629637,15.6456819013906));
#49300=CARTESIAN_POINT('Ctrl Pts',(55.0282234420616,30.9948633057558,15.648024306871));
#49301=CARTESIAN_POINT('Ctrl Pts',(54.8899487516295,30.9943703041964,15.6572911436484));
#49302=CARTESIAN_POINT('Ctrl Pts',(54.7872033187004,30.9860356059246,15.6644049771679));
#49303=CARTESIAN_POINT('Ctrl Pts',(54.563776474529,30.9503713726648,15.6801653432667));
#49304=CARTESIAN_POINT('Ctrl Pts',(54.4440370191278,30.9196744314123,15.6888060340609));
#49305=CARTESIAN_POINT('Ctrl Pts',(54.3130936552536,30.8728145338205,15.6980153577458));
#49306=CARTESIAN_POINT('Ctrl Pts',(54.2983576958312,30.8673437600483,15.6990479028453));
#49307=CARTESIAN_POINT('Ctrl Pts',(54.2776680678751,30.8593831608111,15.7004906675542));
#49308=CARTESIAN_POINT('Ctrl Pts',(54.2716598962553,30.8570379250098,15.7009088056684));
#49309=CARTESIAN_POINT('Ctrl Pts',(54.2615641560586,30.853040609973,15.7016098840766));
#49310=CARTESIAN_POINT('Ctrl Pts',(54.2574705332348,30.851404059111,15.7018937307964));
#49311=CARTESIAN_POINT('Ctrl Pts',(54.2491178855321,30.8480326730328,15.7024719721427));
#49312=CARTESIAN_POINT('Ctrl Pts',(54.2448593842566,30.8462966614054,15.7027662945351));
#49313=CARTESIAN_POINT('Ctrl Pts',(54.2343542928674,30.8419717518811,15.7034912290836));
#49314=CARTESIAN_POINT('Ctrl Pts',(54.2281147350903,30.8393657669244,15.7039208307253));
#49315=CARTESIAN_POINT('Ctrl Pts',(54.2033444814168,30.8288720955499,15.7056228612084));
#49316=CARTESIAN_POINT('Ctrl Pts',(54.1849197152366,30.8207353898419,15.7068812054709));
#49317=CARTESIAN_POINT('Ctrl Pts',(54.0365231350092,30.7524965475627,15.7169783921562));
#49318=CARTESIAN_POINT('Ctrl Pts',(53.9132279582904,30.6788297710545,15.7251526225547));
#49319=CARTESIAN_POINT('Ctrl Pts',(53.7829812108933,30.5805976911614,15.734646900052));
#49320=CARTESIAN_POINT('Ctrl Pts',(53.7672692879489,30.5683745638605,15.7358074220821));
#49321=CARTESIAN_POINT('Ctrl Pts',(53.6696529324222,30.4900605023783,15.743127462459));
#49322=CARTESIAN_POINT('Ctrl Pts',(53.5929139277952,30.417818086796,15.7493881697009));
#49323=CARTESIAN_POINT('Ctrl Pts',(53.5116934176174,30.3282384734495,15.7568929020904));
#49324=CARTESIAN_POINT('Ctrl Pts',(53.5012883543632,30.3164867287231,15.757872518066));
#49325=CARTESIAN_POINT('Ctrl Pts',(53.4845907105408,30.2971734589775,15.7594752789262));
#49326=CARTESIAN_POINT('Ctrl Pts',(53.4782133472366,30.2896858823703,15.7600949378891));
#49327=CARTESIAN_POINT('Ctrl Pts',(53.4669331329581,30.2762417704714,15.7612046739681));
#49328=CARTESIAN_POINT('Ctrl Pts',(53.4620089404592,30.2703033391976,15.7616938726205));
#49329=CARTESIAN_POINT('Ctrl Pts',(53.4516735838924,30.2576910159417,15.7627308677088));
#49330=CARTESIAN_POINT('Ctrl Pts',(53.4462708571174,30.2510104432699,15.7632789884445));
#49331=CARTESIAN_POINT('Ctrl Pts',(53.4319956777335,30.2331237982327,15.7647435861003));
#49332=CARTESIAN_POINT('Ctrl Pts',(53.4232003557133,30.221857078656,15.765663086126));
#49333=CARTESIAN_POINT('Ctrl Pts',(53.3812305055252,30.1668862202387,15.7701356318137));
#49334=CARTESIAN_POINT('Ctrl Pts',(53.3497504438594,30.121924047546,15.7737533029853));
#49335=CARTESIAN_POINT('Ctrl Pts',(53.2816383736695,30.0155613755344,15.78222626844));
#49336=CARTESIAN_POINT('Ctrl Pts',(53.2463742546062,29.9533764934821,15.7871201842216));
#49337=CARTESIAN_POINT('Ctrl Pts',(53.1838448417862,29.8278538269155,15.7968350799041));
#49338=CARTESIAN_POINT('Ctrl Pts',(53.1563731239664,29.7647229573151,15.801645506378));
#49339=CARTESIAN_POINT('Ctrl Pts',(53.0999240048787,29.6141667059374,15.8128243982356));
#49340=CARTESIAN_POINT('Ctrl Pts',(53.0736221236358,29.5258914375472,15.8191605622914));
#49341=CARTESIAN_POINT('Ctrl Pts',(53.0511813086901,29.4257303638222,15.8259024611584));
#49342=CARTESIAN_POINT('Ctrl Pts',(53.0489394772819,29.4153353859556,15.8265968235746));
#49343=CARTESIAN_POINT('Ctrl Pts',(53.0467495290295,29.4047717676867,15.8272967139322));
#49344=CARTESIAN_POINT('Ctrl Pts',(53.0467182547747,29.4046208225388,15.8273067135856));
#49345=CARTESIAN_POINT('Ctrl Pts',(53.0466869980082,29.4044698737233,15.8273167122946));
#49346=CARTESIAN_POINT('Origin',(55.,29.,3.45145488139523));
#49347=CARTESIAN_POINT('',(53.046686998698,29.4044698770549,16.7848524498588));
#49348=CARTESIAN_POINT('',(53.0466869925414,29.4044698473222,16.6248055079682));
#49349=CARTESIAN_POINT('',(53.0466869980082,29.4044698737233,3.45145488139523));
#49350=CARTESIAN_POINT('Ctrl Pts',(53.046686998698,29.4044698770549,16.7848524498588));
#49351=CARTESIAN_POINT('Ctrl Pts',(53.0473705149442,29.4077707932567,16.7846504639398));
#49352=CARTESIAN_POINT('Ctrl Pts',(53.048062443288,29.4110701929009,16.7844482656876));
#49353=CARTESIAN_POINT('Ctrl Pts',(53.0602391405275,29.4684096166467,16.7809288766104));
#49354=CARTESIAN_POINT('Ctrl Pts',(53.0739547274212,29.5219468704672,16.7775578590536));
#49355=CARTESIAN_POINT('Ctrl Pts',(53.093988482993,29.5885164108423,16.7732256058865));
#49356=CARTESIAN_POINT('Ctrl Pts',(53.098250161206,29.602145333603,16.7723311577031));
#49357=CARTESIAN_POINT('Ctrl Pts',(53.1053088717664,29.6238965137048,16.770891102513));
#49358=CARTESIAN_POINT('Ctrl Pts',(53.1080127330734,29.6320486605423,16.7703485378006));
#49359=CARTESIAN_POINT('Ctrl Pts',(53.1132451521605,29.647489945067,16.7693153208745));
#49360=CARTESIAN_POINT('Ctrl Pts',(53.1157635219392,29.654782388912,16.7688250107219));
#49361=CARTESIAN_POINT('Ctrl Pts',(53.1215902313444,29.6713427903041,16.767706112983));
#49362=CARTESIAN_POINT('Ctrl Pts',(53.1249249564342,29.6806011874579,16.7670766653315));
#49363=CARTESIAN_POINT('Ctrl Pts',(53.1337621247913,29.7045783631893,16.7654361871325));
#49364=CARTESIAN_POINT('Ctrl Pts',(53.1393701416055,29.7192572443075,16.7644216881598));
#49365=CARTESIAN_POINT('Ctrl Pts',(53.1929729923203,29.8547382862848,16.7549613145506));
#49366=CARTESIAN_POINT('Ctrl Pts',(53.2524860251078,29.9706223155998,16.7461195822069));
#49367=CARTESIAN_POINT('Ctrl Pts',(53.3610768887371,30.1392758471369,16.7321918515968));
#49368=CARTESIAN_POINT('Ctrl Pts',(53.4024499896321,30.1966003254097,16.727249496158));
#49369=CARTESIAN_POINT('Ctrl Pts',(53.4819910523746,30.295309292532,16.7184595056697));
#49370=CARTESIAN_POINT('Ctrl Pts',(53.5190364879144,30.337507107203,16.7146000730754));
#49371=CARTESIAN_POINT('Ctrl Pts',(53.5715054469016,30.3924164580435,16.7094920025527));
#49372=CARTESIAN_POINT('Ctrl Pts',(53.5854095794868,30.406539827671,16.7081699822837));
#49373=CARTESIAN_POINT('Ctrl Pts',(53.6093822823076,30.4301753892688,16.7059470282432));
#49374=CARTESIAN_POINT('Ctrl Pts',(53.6193434194752,30.43979398281,16.7050393147285));
#49375=CARTESIAN_POINT('Ctrl Pts',(53.6337679137596,30.4534350760634,16.7037485930727));
#49376=CARTESIAN_POINT('Ctrl Pts',(53.6381502808744,30.4575421018179,16.7033595348484));
#49377=CARTESIAN_POINT('Ctrl Pts',(53.6457699642133,30.464618677093,16.7026884921108));
#49378=CARTESIAN_POINT('Ctrl Pts',(53.6489986463229,30.4675974253779,16.7024058199935));
#49379=CARTESIAN_POINT('Ctrl Pts',(53.6557133918333,30.4737514414887,16.7018214317487));
#49380=CARTESIAN_POINT('Ctrl Pts',(53.6592008959342,30.4769250352797,16.7015198380407));
#49381=CARTESIAN_POINT('Ctrl Pts',(53.6683878641594,30.4852257241798,16.7007303010491));
#49382=CARTESIAN_POINT('Ctrl Pts',(53.6741057542279,30.490332441318,16.7002438537992));
#49383=CARTESIAN_POINT('Ctrl Pts',(53.6979893345979,30.5114169041511,16.6982317444918));
#49384=CARTESIAN_POINT('Ctrl Pts',(53.7164163415951,30.5270972286205,16.6967264770743));
#49385=CARTESIAN_POINT('Ctrl Pts',(53.8644110482558,30.6484600670704,16.6849622493311));
#49386=CARTESIAN_POINT('Ctrl Pts',(54.0065288925773,30.7378183482786,16.6755522791111));
#49387=CARTESIAN_POINT('Ctrl Pts',(54.2167920207878,30.8357007838572,16.6619415093971));
#49388=CARTESIAN_POINT('Ctrl Pts',(54.2767260802871,30.8601306304453,16.6580998674304));
#49389=CARTESIAN_POINT('Ctrl Pts',(54.3626510169625,30.8903733480591,16.6525663728397));
#49390=CARTESIAN_POINT('Ctrl Pts',(54.3877350558922,30.898646008298,16.6509482132753));
#49391=CARTESIAN_POINT('Ctrl Pts',(54.4323406533457,30.9123809793309,16.6480610175726));
#49392=CARTESIAN_POINT('Ctrl Pts',(54.4517953380515,30.9180484211611,16.6467985681853));
#49393=CARTESIAN_POINT('Ctrl Pts',(54.4808204171494,30.9260262058763,16.6449088762474));
#49394=CARTESIAN_POINT('Ctrl Pts',(54.4903274158068,30.9285637755451,16.6442889412856));
#49395=CARTESIAN_POINT('Ctrl Pts',(54.5073212005192,30.9329652567805,16.643178897985));
#49396=CARTESIAN_POINT('Ctrl Pts',(54.5148008080795,30.9348562801469,16.6426896699732));
#49397=CARTESIAN_POINT('Ctrl Pts',(54.5306305026254,30.9387608449992,16.6416528085416));
#49398=CARTESIAN_POINT('Ctrl Pts',(54.5389829822338,30.940763933279,16.6411048520127));
#49399=CARTESIAN_POINT('Ctrl Pts',(54.5612571514811,30.9459538128896,16.6396411598183));
#49400=CARTESIAN_POINT('Ctrl Pts',(54.5752003659685,30.949045095031,16.6387224076357));
#49401=CARTESIAN_POINT('Ctrl Pts',(54.637039086391,30.9620599787507,16.6346358467582));
#49402=CARTESIAN_POINT('Ctrl Pts',(54.6852534319062,30.9703689751216,16.6314176886647));
#49403=CARTESIAN_POINT('Ctrl Pts',(54.7567159234007,30.9799946399306,16.6265978493644));
#49404=CARTESIAN_POINT('Ctrl Pts',(54.7797622740632,30.9826903931219,16.6250360001261));
#49405=CARTESIAN_POINT('Ctrl Pts',(54.8211578790237,30.9868018404937,16.6222179346312));
#49406=CARTESIAN_POINT('Ctrl Pts',(54.8394899157393,30.9883668026405,16.6209655201859));
#49407=CARTESIAN_POINT('Ctrl Pts',(54.9847570689201,30.9987459156168,16.611008911908));
#49408=CARTESIAN_POINT('Ctrl Pts',(55.1122469751788,30.9956489301273,16.6020502653037));
#49409=CARTESIAN_POINT('Ctrl Pts',(55.3026256359539,30.9727162131075,16.5888054589628));
#49410=CARTESIAN_POINT('Ctrl Pts',(55.366285797496,30.9618939551428,16.5844048501245));
#49411=CARTESIAN_POINT('Ctrl Pts',(55.4429918157718,30.944988935424,16.5792186881644));
#49412=CARTESIAN_POINT('Ctrl Pts',(55.4566371335069,30.9418306472086,16.5783007095968));
#49413=CARTESIAN_POINT('Ctrl Pts',(55.4760641829041,30.9371180316722,16.5770014254847));
#49414=CARTESIAN_POINT('Ctrl Pts',(55.4818735736244,30.9356810781081,16.5766138744825));
#49415=CARTESIAN_POINT('Ctrl Pts',(55.4919124966708,30.9331499534369,16.5759459715793));
#49416=CARTESIAN_POINT('Ctrl Pts',(55.4961450336239,30.9320679993103,16.575664933799));
#49417=CARTESIAN_POINT('Ctrl Pts',(55.5049953147444,30.9297746200873,16.5750784867965));
#49418=CARTESIAN_POINT('Ctrl Pts',(55.5096122862517,30.9285605178737,16.574773232089));
#49419=CARTESIAN_POINT('Ctrl Pts',(55.5218866767057,30.9252856257193,16.5739634037597));
#49420=CARTESIAN_POINT('Ctrl Pts',(55.5295363350761,30.9231957047473,16.5734604687426));
#49421=CARTESIAN_POINT('Ctrl Pts',(55.5626493230453,30.9139365367559,16.5712902806018));
#49422=CARTESIAN_POINT('Ctrl Pts',(55.5879823938107,30.9063064260557,16.5696476104942));
#49423=CARTESIAN_POINT('Ctrl Pts',(55.8136501057351,30.8334101305179,16.5551114939945));
#49424=CARTESIAN_POINT('Ctrl Pts',(56.0026354425854,30.7372869754487,16.5434942664095));
#49425=CARTESIAN_POINT('Ctrl Pts',(56.2177767877406,30.580854148709,16.5275237372436));
#49426=CARTESIAN_POINT('Ctrl Pts',(56.2610902157996,30.5465221558145,16.524152513996));
#49427=CARTESIAN_POINT('Ctrl Pts',(56.3137331457803,30.5011118207985,16.5198200287775));
#49428=CARTESIAN_POINT('Ctrl Pts',(56.3244452608945,30.4916689348158,16.5189255631614));
#49429=CARTESIAN_POINT('Ctrl Pts',(56.3414364869799,30.4763636014501,16.5174854865406));
#49430=CARTESIAN_POINT('Ctrl Pts',(56.3477808443583,30.4705740797913,16.5169429179931));
#49431=CARTESIAN_POINT('Ctrl Pts',(56.3597526978606,30.4595066581819,16.515909698067));
#49432=CARTESIAN_POINT('Ctrl Pts',(56.3653873633034,30.4542367173274,16.5154193887792));
#49433=CARTESIAN_POINT('Ctrl Pts',(56.3781391693547,30.4421708736491,16.5143004990087));
#49434=CARTESIAN_POINT('Ctrl Pts',(56.385236833727,30.4353547671904,16.5136710585063));
#49435=CARTESIAN_POINT('Ctrl Pts',(56.4035362126393,30.4175191586215,16.5120306112103));
#49436=CARTESIAN_POINT('Ctrl Pts',(56.4146584978254,30.4064194880906,16.5110161362069));
#49437=CARTESIAN_POINT('Ctrl Pts',(56.5165894435594,30.3022632870349,16.5015535272999));
#49438=CARTESIAN_POINT('Ctrl Pts',(56.5982104028425,30.2006853610274,16.4927093080987));
#49439=CARTESIAN_POINT('Ctrl Pts',(56.7292230403294,30.0003875490554,16.4760908341323));
#49440=CARTESIAN_POINT('Ctrl Pts',(56.7814598942167,29.9040958844398,16.4684053515834));
#49441=CARTESIAN_POINT('Ctrl Pts',(56.8437258272161,29.7627175415939,16.4578824112201));
#49442=CARTESIAN_POINT('Ctrl Pts',(56.8605058075648,29.7208202428746,16.4548540523711));
#49443=CARTESIAN_POINT('Ctrl Pts',(56.8789186336949,29.6699057098751,16.451309489791));
#49444=CARTESIAN_POINT('Ctrl Pts',(56.8819281517953,29.6614040603197,16.4507220875718));
#49445=CARTESIAN_POINT('Ctrl Pts',(56.8865208927137,29.6481447515475,16.4498132145359));
#49446=CARTESIAN_POINT('Ctrl Pts',(56.8881439659113,29.6434011679587,16.4494894970489));
#49447=CARTESIAN_POINT('Ctrl Pts',(56.8911298792098,29.6345659463069,16.4488892876068));
#49448=CARTESIAN_POINT('Ctrl Pts',(56.8924973247266,29.6304760397204,16.4486125391023));
#49449=CARTESIAN_POINT('Ctrl Pts',(56.8955934637248,29.6211149289821,16.4479815751847));
#49450=CARTESIAN_POINT('Ctrl Pts',(56.8973134387888,29.6158409303445,16.4476278694876));
#49451=CARTESIAN_POINT('Ctrl Pts',(56.9017628670033,29.6020019653963,16.4467042255336));
#49452=CARTESIAN_POINT('Ctrl Pts',(56.90445650002,29.5934254926012,16.4461362945954));
#49453=CARTESIAN_POINT('Ctrl Pts',(56.9230274567938,29.5328669202895,16.4421557205374));
#49454=CARTESIAN_POINT('Ctrl Pts',(56.9368338632843,29.4802681401315,16.4388513616038));
#49455=CARTESIAN_POINT('Ctrl Pts',(56.959416274603,29.3772607638437,16.4325585114556));
#49456=CARTESIAN_POINT('Ctrl Pts',(56.9684362348361,29.3269511541557,16.4295652887979));
#49457=CARTESIAN_POINT('Ctrl Pts',(56.9869603761347,29.1945289522752,16.4217753928369));
#49458=CARTESIAN_POINT('Ctrl Pts',(56.9933116541355,29.1120782333297,16.4170105030146));
#49459=CARTESIAN_POINT('Ctrl Pts',(56.9958274017511,28.9418224076345,16.4070142896063));
#49460=CARTESIAN_POINT('Ctrl Pts',(56.991343565272,28.8541924701125,16.4017821409044));
#49461=CARTESIAN_POINT('Ctrl Pts',(56.9785580648322,28.7454131546871,16.395018614302));
#49462=CARTESIAN_POINT('Ctrl Pts',(56.9756460596507,28.7237228452262,16.393656848677));
#49463=CARTESIAN_POINT('Ctrl Pts',(56.9708622998961,28.6920514054342,16.3916473262227));
#49464=CARTESIAN_POINT('Ctrl Pts',(56.9692701960676,28.6820291981181,16.3910083205457));
#49465=CARTESIAN_POINT('Ctrl Pts',(56.9663267336948,28.6643709363987,16.389876777756));
#49466=CARTESIAN_POINT('Ctrl Pts',(56.9650071801711,28.6567297404387,16.3893852504248));
#49467=CARTESIAN_POINT('Ctrl Pts',(56.962342135679,28.6418162483501,16.3884221710889));
#49468=CARTESIAN_POINT('Ctrl Pts',(56.9610006864978,28.6345433506538,16.3879507540536));
#49469=CARTESIAN_POINT('Ctrl Pts',(56.9572683841659,28.6149204330259,16.3866740134778));
#49470=CARTESIAN_POINT('Ctrl Pts',(56.9548011327827,28.6025854558701,16.3858662875173));
#49471=CARTESIAN_POINT('Ctrl Pts',(56.9450646693022,28.5561941261973,16.3828084782362));
#49472=CARTESIAN_POINT('Ctrl Pts',(56.9370210980891,28.5223084300253,16.380534086293));
#49473=CARTESIAN_POINT('Ctrl Pts',(56.881347545963,28.3123849184692,16.3661792143959));
#49474=CARTESIAN_POINT('Ctrl Pts',(56.8106530116329,28.1433817345567,16.3533360541871));
#49475=CARTESIAN_POINT('Ctrl Pts',(56.6833842180433,27.9276702164961,16.3360099263615));
#49476=CARTESIAN_POINT('Ctrl Pts',(56.6457581492161,27.8707721356431,16.3313518807412));
#49477=CARTESIAN_POINT('Ctrl Pts',(56.5967439052245,27.8043229189547,16.3258968957257));
#49478=CARTESIAN_POINT('Ctrl Pts',(56.5880734703435,27.7928308062458,16.3249529657946));
#49479=CARTESIAN_POINT('Ctrl Pts',(56.5755827017754,27.7766426011678,16.3236237470804));
#49480=CARTESIAN_POINT('Ctrl Pts',(56.5718644731194,27.7718687953404,16.3232318231915));
#49481=CARTESIAN_POINT('Ctrl Pts',(56.5654177367583,27.7636691173335,16.3225588413691));
#49482=CARTESIAN_POINT('Ctrl Pts',(56.5626995809244,27.7602351984057,16.3222770686008));
#49483=CARTESIAN_POINT('Ctrl Pts',(56.5570122738429,27.7530986946551,16.3216916482766));
#49484=CARTESIAN_POINT('Ctrl Pts',(56.5540412023467,27.7493977336054,16.3213881401283));
#49485=CARTESIAN_POINT('Ctrl Pts',(56.5461497599975,27.7396391845484,16.3205879897887));
#49486=CARTESIAN_POINT('Ctrl Pts',(56.5412069421259,27.7335997347668,16.3200929175765));
#49487=CARTESIAN_POINT('Ctrl Pts',(56.5200570009195,27.7080646243609,16.3179995269098));
#49488=CARTESIAN_POINT('Ctrl Pts',(56.5035136476127,27.6888489208012,16.3164237044337));
#49489=CARTESIAN_POINT('Ctrl Pts',(56.3452890152304,27.51199960473,16.3018588965334));
#49490=CARTESIAN_POINT('Ctrl Pts',(56.1796882752731,27.3775607955234,16.2901809722933));
#49491=CARTESIAN_POINT('Ctrl Pts',(55.9643419860151,27.2534584359322,16.2752593322375));
#49492=CARTESIAN_POINT('Ctrl Pts',(55.9321870505075,27.2360867449525,16.2730418908035));
#49493=CARTESIAN_POINT('Ctrl Pts',(55.8762991378782,27.2078483797508,16.269191800827));
#49494=CARTESIAN_POINT('Ctrl Pts',(55.8527962931578,27.1965460932352,16.2675739211466));
#49495=CARTESIAN_POINT('Ctrl Pts',(55.8191815357387,27.1811851108778,16.2652585011433));
#49496=CARTESIAN_POINT('Ctrl Pts',(55.8092469305589,27.1767431921701,16.2645740244299));
#49497=CARTESIAN_POINT('Ctrl Pts',(55.79206229399,27.169227789693,16.2633895139526));
#49498=CARTESIAN_POINT('Ctrl Pts',(55.7848294240865,27.1661155064174,16.2628908065538));
#49499=CARTESIAN_POINT('Ctrl Pts',(55.7709470783642,27.1602391409029,16.2619332337006));
#49500=CARTESIAN_POINT('Ctrl Pts',(55.7643006779694,27.1574680768745,16.2614746131039));
#49501=CARTESIAN_POINT('Ctrl Pts',(55.748666045773,27.1510487265375,16.260395318362));
#49502=CARTESIAN_POINT('Ctrl Pts',(55.7396659794475,27.1474299222136,16.2597736673114));
#49503=CARTESIAN_POINT('Ctrl Pts',(55.7085098296015,27.135165687043,16.2576202161656));
#49504=CARTESIAN_POINT('Ctrl Pts',(55.6862264610941,27.1268512186896,16.2560775054092));
#49505=CARTESIAN_POINT('Ctrl Pts',(55.5213574464728,27.0686712615615,16.2446404063663));
#49506=CARTESIAN_POINT('Ctrl Pts',(55.3736910792937,27.0347562595619,16.2342156075911));
#49507=CARTESIAN_POINT('Ctrl Pts',(55.1389188332706,27.0082673285828,16.2177487144301));
#49508=CARTESIAN_POINT('Ctrl Pts',(55.0536621031402,27.0041494343057,16.2118036362858));
#49509=CARTESIAN_POINT('Ctrl Pts',(54.9428131343688,27.0059057067328,16.2042901932319));
#49510=CARTESIAN_POINT('Ctrl Pts',(54.9172356810205,27.0068034259631,16.2025718680887));
#49511=CARTESIAN_POINT('Ctrl Pts',(54.8746436909906,27.0091196670412,16.1997433742915));
#49512=CARTESIAN_POINT('Ctrl Pts',(54.8576178844072,27.0102648206072,16.1986214931631));
#49513=CARTESIAN_POINT('Ctrl Pts',(54.8341546733036,27.0121456779245,16.1970894477872));
#49514=CARTESIAN_POINT('Ctrl Pts',(54.8277035914137,27.012694429995,16.1966696847085));
#49515=CARTESIAN_POINT('Ctrl Pts',(54.8168154048531,27.0136740353514,16.195963807799));
#49516=CARTESIAN_POINT('Ctrl Pts',(54.8123769013735,27.0140883685486,16.1956767926037));
#49517=CARTESIAN_POINT('Ctrl Pts',(54.8039069002132,27.0149076911272,16.195130523713));
#49518=CARTESIAN_POINT('Ctrl Pts',(54.7998752084606,27.0153100879351,16.1948711229679));
#49519=CARTESIAN_POINT('Ctrl Pts',(54.7902848010281,27.0162968120632,16.1942554916693));
#49520=CARTESIAN_POINT('Ctrl Pts',(54.7847272240995,27.0168922277757,16.1938998730537));
#49521=CARTESIAN_POINT('Ctrl Pts',(54.7650467696054,27.0190844177865,16.1926443511984));
#49522=CARTESIAN_POINT('Ctrl Pts',(54.750938143285,27.0208088059089,16.191751210422));
#49523=CARTESIAN_POINT('Ctrl Pts',(54.5920295626162,27.0419571703747,16.1817575986078));
#49524=CARTESIAN_POINT('Ctrl Pts',(54.4497435299318,27.0770849236533,16.1734064550476));
#49525=CARTESIAN_POINT('Ctrl Pts',(54.1923503502196,27.1715781825362,16.1574616719917));
#49526=CARTESIAN_POINT('Ctrl Pts',(54.0766900076913,27.2271726503802,16.1499362229217));
#49527=CARTESIAN_POINT('Ctrl Pts',(53.9512779231385,27.3030750479341,16.1408503125363));
#49528=CARTESIAN_POINT('Ctrl Pts',(53.9355292029729,27.3129095538098,16.1396919383558));
#49529=CARTESIAN_POINT('Ctrl Pts',(53.9119313723182,27.3281075024208,16.1379285744878));
#49530=CARTESIAN_POINT('Ctrl Pts',(53.9039792688119,27.3333097426913,16.1373295147433));
#49531=CARTESIAN_POINT('Ctrl Pts',(53.8896652359821,27.3428206769313,16.136242255194));
#49532=CARTESIAN_POINT('Ctrl Pts',(53.883290418788,27.3471097115843,16.1357547948308));
#49533=CARTESIAN_POINT('Ctrl Pts',(53.8696629597413,27.3563932094912,16.1347056759883));
#49534=CARTESIAN_POINT('Ctrl Pts',(53.8624183148006,27.3613990687755,16.134143595276));
#49535=CARTESIAN_POINT('Ctrl Pts',(53.8430215607499,27.3749923482477,16.1326268013637));
#49536=CARTESIAN_POINT('Ctrl Pts',(53.8309321913598,27.3836679127855,16.1316687551628));
#49537=CARTESIAN_POINT('Ctrl Pts',(53.7728269335032,27.4263582834322,16.1270012236523));
#49538=CARTESIAN_POINT('Ctrl Pts',(53.7281960716767,27.4622042819646,16.1232215057134));
#49539=CARTESIAN_POINT('Ctrl Pts',(53.564243397828,27.6059094000608,16.108563118275));
#49540=CARTESIAN_POINT('Ctrl Pts',(53.456585018566,27.7261304637871,16.0972139560425));
#49541=CARTESIAN_POINT('Ctrl Pts',(53.3283951179911,27.9097016548184,16.0817586892576));
#49542=CARTESIAN_POINT('Ctrl Pts',(53.2947233113002,27.9631555857376,16.077456762131));
#49543=CARTESIAN_POINT('Ctrl Pts',(53.2568228139543,28.0301790206476,16.0723740707819));
#49544=CARTESIAN_POINT('Ctrl Pts',(53.2501300884162,28.0423075900775,16.0714662997064));
#49545=CARTESIAN_POINT('Ctrl Pts',(53.2407400725064,28.0597513277486,16.0701788162971));
#49546=CARTESIAN_POINT('Ctrl Pts',(53.2379395876584,28.0650100729875,16.069793008775));
#49547=CARTESIAN_POINT('Ctrl Pts',(53.2331285073647,28.0741427006845,16.0691271223121));
#49548=CARTESIAN_POINT('Ctrl Pts',(53.2311070019716,28.0780107521239,16.0688463690211));
#49549=CARTESIAN_POINT('Ctrl Pts',(53.226895548703,28.0861339986264,16.0682594717182));
#49550=CARTESIAN_POINT('Ctrl Pts',(53.2247082082337,28.0903904579852,16.0679534884231));
#49551=CARTESIAN_POINT('Ctrl Pts',(53.2189133266554,28.1017675463824,16.0671396226325));
#49552=CARTESIAN_POINT('Ctrl Pts',(53.2153331281141,28.1089021152602,16.0666334077133));
#49553=CARTESIAN_POINT('Ctrl Pts',(53.1998643606763,28.1401952533789,16.0644303853692));
#49554=CARTESIAN_POINT('Ctrl Pts',(53.1884221764369,28.1645728772,16.0627590835511));
#49555=CARTESIAN_POINT('Ctrl Pts',(53.09912068626,28.3652996467371,16.0493004481448));
#49556=CARTESIAN_POINT('Ctrl Pts',(53.0466992427891,28.5518680042743,16.0385865915237));
#49557=CARTESIAN_POINT('Ctrl Pts',(53.0127802526994,28.8130240365448,16.0229282389335));
#49558=CARTESIAN_POINT('Ctrl Pts',(53.0074127724654,28.883394428305,16.0186573924036));
#49559=CARTESIAN_POINT('Ctrl Pts',(53.005428202742,28.9692368710182,16.0133141479646));
#49560=CARTESIAN_POINT('Ctrl Pts',(53.0052505792685,28.9845807777245,16.0123540104904));
#49561=CARTESIAN_POINT('Ctrl Pts',(53.0052496691705,29.0087471519639,16.0108332130472));
#49562=CARTESIAN_POINT('Ctrl Pts',(53.0053078649336,29.017569214441,16.010276234499));
#49563=CARTESIAN_POINT('Ctrl Pts',(53.0055262108525,29.0340716527731,16.0092308615406));
#49564=CARTESIAN_POINT('Ctrl Pts',(53.0056722098719,29.0417520772478,16.0087429160464));
#49565=CARTESIAN_POINT('Ctrl Pts',(53.0060974962549,29.0589087799409,16.0076496815384));
#49566=CARTESIAN_POINT('Ctrl Pts',(53.0063999828318,29.0683842470709,16.0070436825613));
#49567=CARTESIAN_POINT('Ctrl Pts',(53.0074904048594,29.0963002992091,16.005251607672));
#49568=CARTESIAN_POINT('Ctrl Pts',(53.0084667367059,29.114732113191,16.0040597225994));
#49569=CARTESIAN_POINT('Ctrl Pts',(53.0158019178629,29.2243793139538,15.9969158706723));
#49570=CARTESIAN_POINT('Ctrl Pts',(53.0281673395051,29.3150326305598,15.9907810223551));
#49571=CARTESIAN_POINT('Ctrl Pts',(53.0466870408509,29.4044700806242,15.9845144320741));
#49572=CARTESIAN_POINT('',(53.0052507646772,29.0017466193016,15.8519165719564));
#49573=CARTESIAN_POINT('Ctrl Pts',(53.0466869980082,29.4044698737233,15.8273167122946));
#49574=CARTESIAN_POINT('Ctrl Pts',(53.0456184424675,29.3993094809065,15.82765853191));
#49575=CARTESIAN_POINT('Ctrl Pts',(53.0445703257718,29.3941448016429,15.8279992478323));
#49576=CARTESIAN_POINT('Ctrl Pts',(53.0427035097501,29.3847551573521,15.8286160926387));
#49577=CARTESIAN_POINT('Ctrl Pts',(53.0418780067912,29.3805316578891,15.8288925951965));
#49578=CARTESIAN_POINT('Ctrl Pts',(53.0401030767234,29.3712919003011,15.8294954045698));
#49579=CARTESIAN_POINT('Ctrl Pts',(53.0391592372855,29.3662746643889,15.8298213954536));
#49580=CARTESIAN_POINT('Ctrl Pts',(53.0372473892707,29.3558924974828,15.8304933076919));
#49581=CARTESIAN_POINT('Ctrl Pts',(53.0362820895715,29.3505271039116,15.8308390787137));
#49582=CARTESIAN_POINT('Ctrl Pts',(53.0338503748553,29.3366856194693,15.8317274689985));
#49583=CARTESIAN_POINT('Ctrl Pts',(53.0324167517075,29.3282037809664,15.8322683670757));
#49584=CARTESIAN_POINT('Ctrl Pts',(53.013969231259,29.2145940953637,15.8394699185221));
#49585=CARTESIAN_POINT('Ctrl Pts',(53.0053440331463,29.10826508465,15.8457172851574));
#49586=CARTESIAN_POINT('Ctrl Pts',(53.0052507646772,29.0017466193016,15.8519165719564));
#49587=CARTESIAN_POINT('Ctrl Pts',(53.0052507657883,29.0017478878248,15.8519164981294));
#49588=CARTESIAN_POINT('Ctrl Pts',(53.0051093436462,28.8403521130213,15.8613095998475));
#49589=CARTESIAN_POINT('Ctrl Pts',(53.0245544374861,28.6795460303851,15.870580099587));
#49590=CARTESIAN_POINT('Ctrl Pts',(53.0672282899422,28.5063299825751,15.8815629752095));
#49591=CARTESIAN_POINT('Ctrl Pts',(53.0715056526317,28.4898763927981,15.8826157811221));
#49592=CARTESIAN_POINT('Ctrl Pts',(53.0797596380104,28.4597147202466,15.8845645221717));
#49593=CARTESIAN_POINT('Ctrl Pts',(53.0836741129222,28.4459906957321,15.8854584571496));
#49594=CARTESIAN_POINT('Ctrl Pts',(53.0901792353015,28.4240781767898,15.8868978811729));
#49595=CARTESIAN_POINT('Ctrl Pts',(53.0926761362893,28.4158621952565,15.8874403327134));
#49596=CARTESIAN_POINT('Ctrl Pts',(53.0975170602289,28.4002952774349,15.8884734607162));
#49597=CARTESIAN_POINT('Ctrl Pts',(53.0998508416654,28.3929413012384,15.8889637959835));
#49598=CARTESIAN_POINT('Ctrl Pts',(53.1052591967136,28.3762358194421,15.8900829274264));
#49599=CARTESIAN_POINT('Ctrl Pts',(53.1083604298594,28.3668932194674,15.8907125850152));
#49600=CARTESIAN_POINT('Ctrl Pts',(53.1165947697249,28.3426876288607,15.8923539716098));
#49601=CARTESIAN_POINT('Ctrl Pts',(53.1218346171657,28.3278619293213,15.8933691753787));
#49602=CARTESIAN_POINT('Ctrl Pts',(53.1721208950162,28.190762376242,15.9028511894069));
#49603=CARTESIAN_POINT('Ctrl Pts',(53.2288636056454,28.0731386423043,15.9117159283036));
#49604=CARTESIAN_POINT('Ctrl Pts',(53.3351842360839,27.8986837442372,15.9259023947575));
#49605=CARTESIAN_POINT('Ctrl Pts',(53.37720369887,27.8376570293225,15.931083915525));
#49606=CARTESIAN_POINT('Ctrl Pts',(53.4552514148529,27.7368137124046,15.9399158919349));
#49607=CARTESIAN_POINT('Ctrl Pts',(53.489674658915,27.6958504963349,15.9435878306713));
#49608=CARTESIAN_POINT('Ctrl Pts',(53.5450073275289,27.6351391981811,15.9491076753616));
#49609=CARTESIAN_POINT('Ctrl Pts',(53.5647651062883,27.6143775087489,15.9510102321847));
#49610=CARTESIAN_POINT('Ctrl Pts',(53.5903604319765,27.588616827809,15.9533821248557));
#49611=CARTESIAN_POINT('Ctrl Pts',(53.5957876145509,27.5832171120518,15.9538799431939));
#49612=CARTESIAN_POINT('Ctrl Pts',(53.6041624457859,27.5749800632388,15.9546401466377));
#49613=CARTESIAN_POINT('Ctrl Pts',(53.6070878870238,27.5721204027751,15.9549042168737));
#49614=CARTESIAN_POINT('Ctrl Pts',(53.6131082598438,27.5662715120836,15.9554445913871));
#49615=CARTESIAN_POINT('Ctrl Pts',(53.6162040351187,27.5632833250053,15.9557208058892));
#49616=CARTESIAN_POINT('Ctrl Pts',(53.6232149086716,27.5565597851309,15.9563426337679));
#49617=CARTESIAN_POINT('Ctrl Pts',(53.6271355454588,27.5528303372736,15.956687796091));
#49618=CARTESIAN_POINT('Ctrl Pts',(53.6387613556214,27.541861222155,15.9577038922058));
#49619=CARTESIAN_POINT('Ctrl Pts',(53.6465091073372,27.5346666736312,15.9583715076284));
#49620=CARTESIAN_POINT('Ctrl Pts',(53.7153705472041,27.4717342354335,15.9642256051505));
#49621=CARTESIAN_POINT('Ctrl Pts',(53.7798468220845,27.419778895783,15.9691601250023));
#49622=CARTESIAN_POINT('Ctrl Pts',(53.9620610243514,27.2907728495076,15.9822610241051));
#49623=CARTESIAN_POINT('Ctrl Pts',(54.0850066333442,27.2219218087822,15.9902650108258));
#49624=CARTESIAN_POINT('Ctrl Pts',(54.2719581495117,27.1417922956407,16.0024145830526));
#49625=CARTESIAN_POINT('Ctrl Pts',(54.3308821238767,27.1197710539724,16.0062359469742));
#49626=CARTESIAN_POINT('Ctrl Pts',(54.4049500821644,27.0960131957975,16.0110790991412));
#49627=CARTESIAN_POINT('Ctrl Pts',(54.4192070524495,27.091615948398,16.012013022368));
#49628=CARTESIAN_POINT('Ctrl Pts',(54.4418816802873,27.0849000794189,16.013501605518));
#49629=CARTESIAN_POINT('Ctrl Pts',(54.4502677242869,27.0824760273333,16.0140528452591));
#49630=CARTESIAN_POINT('Ctrl Pts',(54.4660727150047,27.0780196710631,16.0150931841408));
#49631=CARTESIAN_POINT('Ctrl Pts',(54.4734880532289,27.075975078724,16.0155818761158));
#49632=CARTESIAN_POINT('Ctrl Pts',(54.4901960317847,27.0714720972271,16.0166843881663));
#49633=CARTESIAN_POINT('Ctrl Pts',(54.4994949381191,27.0690378989992,16.0172989731665));
#49634=CARTESIAN_POINT('Ctrl Pts',(54.5233093838449,27.0629875085177,16.0188755775652));
#49635=CARTESIAN_POINT('Ctrl Pts',(54.537848464713,27.0594672705629,16.0198406334626));
#49636=CARTESIAN_POINT('Ctrl Pts',(54.6317880676586,27.0378379617853,16.0260933976371));
#49637=CARTESIAN_POINT('Ctrl Pts',(54.7121849052481,27.0244445475794,16.031529174913));
#49638=CARTESIAN_POINT('Ctrl Pts',(54.9455556621049,27.0001154572308,16.0475336698631));
#49639=CARTESIAN_POINT('Ctrl Pts',(55.0992520022739,27.0018393962555,16.0583875260599));
#49640=CARTESIAN_POINT('Ctrl Pts',(55.3016285231695,27.0275322873061,16.0723361147082));
#49641=CARTESIAN_POINT('Ctrl Pts',(55.3517704300118,27.0358545932164,16.075758134992));
#49642=CARTESIAN_POINT('Ctrl Pts',(55.410658578202,27.0479565383794,16.0796962343169));
#49643=CARTESIAN_POINT('Ctrl Pts',(55.4197600113891,27.0498934170656,16.0803025657274));
#49644=CARTESIAN_POINT('Ctrl Pts',(55.4338044568427,27.0529851014715,16.0812342593709));
#49645=CARTESIAN_POINT('Ctrl Pts',(55.4387570307523,27.0540951741629,16.0815620486359));
#49646=CARTESIAN_POINT('Ctrl Pts',(55.4479033307149,27.0561819249338,16.0821659295712));
#49647=CARTESIAN_POINT('Ctrl Pts',(55.4520981085789,27.0571532733041,16.082442306671));
#49648=CARTESIAN_POINT('Ctrl Pts',(55.4616070913419,27.0593876507695,16.0830675204893));
#49649=CARTESIAN_POINT('Ctrl Pts',(55.4669192678329,27.0606589274221,16.0834158841143));
#49650=CARTESIAN_POINT('Ctrl Pts',(55.4806846852887,27.0640130194205,16.0843163907903));
#49651=CARTESIAN_POINT('Ctrl Pts',(55.4891297367667,27.0661294090049,16.084866686632));
#49652=CARTESIAN_POINT('Ctrl Pts',(55.5444459598084,27.0803775850238,16.0884586122785));
#49653=CARTESIAN_POINT('Ctrl Pts',(55.590880168795,27.0941581688365,16.0914144803056));
#49654=CARTESIAN_POINT('Ctrl Pts',(55.6476450413812,27.113279265236,16.0950059125877));
#49655=CARTESIAN_POINT('Ctrl Pts',(55.6584877042439,27.1170360647042,16.0956908919734));
#49656=CARTESIAN_POINT('Ctrl Pts',(55.711955962851,27.1360802402875,16.0990663431069));
#49657=CARTESIAN_POINT('Ctrl Pts',(55.7540862625891,27.1527229855558,16.1017187435115));
#49658=CARTESIAN_POINT('Ctrl Pts',(55.9092876909186,27.2202276968184,16.1115807550486));
#49659=CARTESIAN_POINT('Ctrl Pts',(56.0180984212386,27.2801547622904,16.1186983446739));
#49660=CARTESIAN_POINT('Ctrl Pts',(56.1696622857658,27.3830804485953,16.1296682968205));
#49661=CARTESIAN_POINT('Ctrl Pts',(56.2171706859668,27.4185344742452,16.1332765141344));
#49662=CARTESIAN_POINT('Ctrl Pts',(56.2743224744466,27.4652874101441,16.1378760007654));
#49663=CARTESIAN_POINT('Ctrl Pts',(56.2855151809648,27.4746504649457,16.1387897517996));
#49664=CARTESIAN_POINT('Ctrl Pts',(56.3031831038444,27.4897628281704,16.1402535373996));
#49665=CARTESIAN_POINT('Ctrl Pts',(56.3097254916999,27.495433068983,16.1408003472013));
#49666=CARTESIAN_POINT('Ctrl Pts',(56.3220183844732,27.5062281689726,16.1418369683236));
#49667=CARTESIAN_POINT('Ctrl Pts',(56.3277765366456,27.5113441102529,16.142326405381));
#49668=CARTESIAN_POINT('Ctrl Pts',(56.3407366928316,27.5229938251691,16.1434368923207));
#49669=CARTESIAN_POINT('Ctrl Pts',(56.3479207984152,27.5295471324476,16.1440587536812));
#49670=CARTESIAN_POINT('Ctrl Pts',(56.3663043556554,27.5465644531971,16.1456665381532));
#49671=CARTESIAN_POINT('Ctrl Pts',(56.3774314693018,27.5571053376125,16.1466557053096));
#49672=CARTESIAN_POINT('Ctrl Pts',(56.45435191277,27.6316738985952,16.1536082345949));
#49673=CARTESIAN_POINT('Ctrl Pts',(56.5157686080941,27.7000395847004,16.1597616422413));
#49674=CARTESIAN_POINT('Ctrl Pts',(56.6605648876017,27.8854852918218,16.1758908241453));
#49675=CARTESIAN_POINT('Ctrl Pts',(56.7364082231354,28.0077791680692,16.186043299444));
#49676=CARTESIAN_POINT('Ctrl Pts',(56.8199025109903,28.181809117412,16.1992306266099));
#49677=CARTESIAN_POINT('Ctrl Pts',(56.8396612364857,28.2272588317221,16.2025647506368));
#49678=CARTESIAN_POINT('Ctrl Pts',(56.8610762565936,28.2820110019831,16.2064154335477));
#49679=CARTESIAN_POINT('Ctrl Pts',(56.8643840125117,28.2906444502721,16.2070178130887));
#49680=CARTESIAN_POINT('Ctrl Pts',(56.8694100149325,28.3040406710662,16.2079447466192));
#49681=CARTESIAN_POINT('Ctrl Pts',(56.8711703030554,28.3087873772885,16.2082716894991));
#49682=CARTESIAN_POINT('Ctrl Pts',(56.8743947095208,28.3175847409548,16.2088747945427));
#49683=CARTESIAN_POINT('Ctrl Pts',(56.8758637714997,28.3216334145851,16.2091512361691));
#49684=CARTESIAN_POINT('Ctrl Pts',(56.879171923112,28.3308434665858,16.2097775881101));
#49685=CARTESIAN_POINT('Ctrl Pts',(56.8810028658543,28.3360076783692,16.2101270180079));
#49686=CARTESIAN_POINT('Ctrl Pts',(56.8857065035791,28.3494499851625,16.2110321289913));
#49687=CARTESIAN_POINT('Ctrl Pts',(56.8885460101602,28.357739683981,16.2115859314993));
#49688=CARTESIAN_POINT('Ctrl Pts',(56.9069535038081,28.4126565560172,16.2152275790398));
#49689=CARTESIAN_POINT('Ctrl Pts',(56.9208493730226,28.4598310005638,16.2182270273091));
#49690=CARTESIAN_POINT('Ctrl Pts',(56.9360826378166,28.5196162287657,16.2219237973167));
#49691=CARTESIAN_POINT('Ctrl Pts',(56.9390618649206,28.5317867559535,16.2226709879493));
#49692=CARTESIAN_POINT('Ctrl Pts',(56.9728129473247,28.6755146481478,16.2314401926524));
#49693=CARTESIAN_POINT('Ctrl Pts',(56.9902577892416,28.8098454730723,16.2391210105582));
#49694=CARTESIAN_POINT('Ctrl Pts',(56.9962201969134,29.0256685820198,16.2518384705449));
#49695=CARTESIAN_POINT('Ctrl Pts',(56.993543213177,29.1064765045103,16.2566788736578));
#49696=CARTESIAN_POINT('Ctrl Pts',(56.9840093091887,29.2077858605768,16.2629686432462));
#49697=CARTESIAN_POINT('Ctrl Pts',(56.9817137466075,29.2286448722807,16.2642753085243));
#49698=CARTESIAN_POINT('Ctrl Pts',(56.9778416813111,29.2593634888168,16.2662184359281));
#49699=CARTESIAN_POINT('Ctrl Pts',(56.9765195019449,29.2692541333232,16.266846963416));
#49700=CARTESIAN_POINT('Ctrl Pts',(56.9740412621945,29.2867898815336,16.2679666249332));
#49701=CARTESIAN_POINT('Ctrl Pts',(56.9729148491761,29.2944390194358,16.2684568204636));
#49702=CARTESIAN_POINT('Ctrl Pts',(56.9704545903423,29.3104976107706,16.2694897990369));
#49703=CARTESIAN_POINT('Ctrl Pts',(56.969111315947,29.3189054415072,16.2700328693401));
#49704=CARTESIAN_POINT('Ctrl Pts',(56.9654267056438,29.3410568769526,16.2714696689978));
#49705=CARTESIAN_POINT('Ctrl Pts',(56.9629950755614,29.3547847877656,16.2723662219427));
#49706=CARTESIAN_POINT('Ctrl Pts',(56.9519632366188,29.4134764264499,16.276226299209));
#49707=CARTESIAN_POINT('Ctrl Pts',(56.9419610538658,29.4581592889818,16.2792335787092));
#49708=CARTESIAN_POINT('Ctrl Pts',(56.8825649743854,29.6863586175012,16.2949580354118));
#49709=CARTESIAN_POINT('Ctrl Pts',(56.8086646675245,29.8624666252785,16.3084558762451));
#49710=CARTESIAN_POINT('Ctrl Pts',(56.6830430005983,30.0720790042431,16.3252012724145));
#49711=CARTESIAN_POINT('Ctrl Pts',(56.6531771657305,30.1175838011226,16.3288733808365));
#49712=CARTESIAN_POINT('Ctrl Pts',(56.61597346764,30.169507105781,16.3330588810635));
#49713=CARTESIAN_POINT('Ctrl Pts',(56.6104068330511,30.1771605494221,16.3336756838335));
#49714=CARTESIAN_POINT('Ctrl Pts',(56.601751158043,30.1888847274772,16.3346199793788));
#49715=CARTESIAN_POINT('Ctrl Pts',(56.5987006816378,30.1929835704907,16.3349500014956));
#49716=CARTESIAN_POINT('Ctrl Pts',(56.5930520797948,30.200512869864,16.335555958806));
#49717=CARTESIAN_POINT('Ctrl Pts',(56.590458613593,30.2039466262005,16.335832195089));
#49718=CARTESIAN_POINT('Ctrl Pts',(56.5845740858773,30.2116855585267,16.3364545388998));
#49719=CARTESIAN_POINT('Ctrl Pts',(56.5812765859484,30.215985726383,16.3368001919897));
#49720=CARTESIAN_POINT('Ctrl Pts',(56.5714714149679,30.2286650118085,16.3378190876345));
#49721=CARTESIAN_POINT('Ctrl Pts',(56.564914253742,30.2370058647142,16.3384889845447));
#49722=CARTESIAN_POINT('Ctrl Pts',(56.5044820789306,30.3126272672709,16.3445632649717));
#49723=CARTESIAN_POINT('Ctrl Pts',(56.4463585816557,30.3764110358905,16.3496937990699));
#49724=CARTESIAN_POINT('Ctrl Pts',(56.2851697870585,30.5317686743795,16.3628112542214));
#49725=CARTESIAN_POINT('Ctrl Pts',(56.1764379899719,30.6167776780792,16.3706626054413));
#49726=CARTESIAN_POINT('Ctrl Pts',(56.0069665063753,30.7230606888814,16.3826161142804));
#49727=CARTESIAN_POINT('Ctrl Pts',(55.9525922704674,30.7537064993419,16.3864090681107));
#49728=CARTESIAN_POINT('Ctrl Pts',(55.8836384871072,30.7884155547747,16.3912162481201));
#49729=CARTESIAN_POINT('Ctrl Pts',(55.8703280790984,30.7949306918662,16.3921439862725));
#49730=CARTESIAN_POINT('Ctrl Pts',(55.8490836385608,30.8050374943899,16.3936249666681));
#49731=CARTESIAN_POINT('Ctrl Pts',(55.8411963801974,30.8087266315008,16.3941748491635));
#49732=CARTESIAN_POINT('Ctrl Pts',(55.8262938681619,30.815578480666,16.3952140323911));
#49733=CARTESIAN_POINT('Ctrl Pts',(55.8192839551839,30.8187524774128,16.3957029359699));
#49734=CARTESIAN_POINT('Ctrl Pts',(55.803446289644,30.8258134237068,16.396807810897));
#49735=CARTESIAN_POINT('Ctrl Pts',(55.7946084056116,30.8296770411454,16.3974245610209));
#49736=CARTESIAN_POINT('Ctrl Pts',(55.7718929435755,30.8394118351872,16.3990104255696));
#49737=CARTESIAN_POINT('Ctrl Pts',(55.7579764276244,30.8451900526467,16.3999826374789));
#49738=CARTESIAN_POINT('Ctrl Pts',(55.6658497387135,30.8822235133429,16.4064240857066));
#49739=CARTESIAN_POINT('Ctrl Pts',(55.5858028016728,30.9086521379401,16.412052121815));
#49740=CARTESIAN_POINT('Ctrl Pts',(55.3847268201818,30.961197526918,16.4262481425568));
#49741=CARTESIAN_POINT('Ctrl Pts',(55.2624764953858,30.9812654972897,16.434941119093));
#49742=CARTESIAN_POINT('Ctrl Pts',(55.0700453721811,30.9947236744574,16.4482915915325));
#49743=CARTESIAN_POINT('Ctrl Pts',(55.0007102877229,30.995953487212,16.4530298627083));
#49744=CARTESIAN_POINT('Ctrl Pts',(54.9169405620533,30.9930728381702,16.4585683039943));
#49745=CARTESIAN_POINT('Ctrl Pts',(54.9024408539262,30.992415732405,16.4595201282042));
#49746=CARTESIAN_POINT('Ctrl Pts',(54.8818878658535,30.9912593857453,16.460858433786));
#49747=CARTESIAN_POINT('Ctrl Pts',(54.8758281075853,30.9908906953949,16.461251670957));
#49748=CARTESIAN_POINT('Ctrl Pts',(54.8653965885547,30.9902082034325,16.4619261835779));
#49749=CARTESIAN_POINT('Ctrl Pts',(54.8610240334727,30.9899076495183,16.4622081825729));
#49750=CARTESIAN_POINT('Ctrl Pts',(54.8519267968819,30.9892522052942,16.462793321303));
#49751=CARTESIAN_POINT('Ctrl Pts',(54.8472023621686,30.9888948923337,16.46309632605));
#49752=CARTESIAN_POINT('Ctrl Pts',(54.8347356467625,30.987907340576,16.4638936871355));
#49753=CARTESIAN_POINT('Ctrl Pts',(54.8269956053571,30.9872486973983,16.4643864930584));
#49754=CARTESIAN_POINT('Ctrl Pts',(54.7943196443121,30.9842757612931,16.4664582354515));
#49755=CARTESIAN_POINT('Ctrl Pts',(54.7694234152813,30.9815371002198,16.468015246375));
#49756=CARTESIAN_POINT('Ctrl Pts',(54.5340336729235,30.9511466752183,16.4825883654055));
#49757=CARTESIAN_POINT('Ctrl Pts',(54.3291516015137,30.8905254229942,16.4942834611104));
#49758=CARTESIAN_POINT('Ctrl Pts',(54.1046961950376,30.7829175919944,16.5092270911453));
#49759=CARTESIAN_POINT('Ctrl Pts',(54.0721731723033,30.7662109692837,16.5114454499886));
#49760=CARTESIAN_POINT('Ctrl Pts',(54.0172613934515,30.7360682258792,16.515296992248));
#49761=CARTESIAN_POINT('Ctrl Pts',(53.9946432127787,30.7230686830316,16.5169153914755));
#49762=CARTESIAN_POINT('Ctrl Pts',(53.9629591009696,30.7040223571419,16.519231427417));
#49763=CARTESIAN_POINT('Ctrl Pts',(53.9536771687933,30.6983387604725,16.5199159908968));
#49764=CARTESIAN_POINT('Ctrl Pts',(53.9377608565675,30.6884127367668,16.5211006038205));
#49765=CARTESIAN_POINT('Ctrl Pts',(53.931104166181,30.6842064187867,16.5215993262792));
#49766=CARTESIAN_POINT('Ctrl Pts',(53.9184082989524,30.676078400386,16.522556894751));
#49767=CARTESIAN_POINT('Ctrl Pts',(53.9123650988404,30.6721631892768,16.5230154957149));
#49768=CARTESIAN_POINT('Ctrl Pts',(53.8982318417188,30.6628976402545,16.524094693499));
#49769=CARTESIAN_POINT('Ctrl Pts',(53.890159403155,30.6575208839386,16.5247162667857));
#49770=CARTESIAN_POINT('Ctrl Pts',(53.8624348668058,30.6387612492481,16.5268691908446));
#49771=CARTESIAN_POINT('Ctrl Pts',(53.8429836575419,30.6250864491029,16.5284114452237));
#49772=CARTESIAN_POINT('Ctrl Pts',(53.701675760247,30.5219195468145,16.5398568095811));
#49773=CARTESIAN_POINT('Ctrl Pts',(53.5901219031113,30.4191942603955,16.5502913885636));
#49774=CARTESIAN_POINT('Ctrl Pts',(53.4355440712499,30.2404671346425,16.5667609675963));
#49775=CARTESIAN_POINT('Ctrl Pts',(53.3840105141943,30.1725445283333,16.5726991143893));
#49776=CARTESIAN_POINT('Ctrl Pts',(53.3228525960863,30.0802120750893,16.5802047619668));
#49777=CARTESIAN_POINT('Ctrl Pts',(53.3091413713342,30.0586211628707,16.5819219463752));
#49778=CARTESIAN_POINT('Ctrl Pts',(53.2869843573526,30.0222014629899,16.5847487648326));
#49779=CARTESIAN_POINT('Ctrl Pts',(53.2783070726536,30.0075177086968,16.5858700946251));
#49780=CARTESIAN_POINT('Ctrl Pts',(53.2665974380612,29.9871094268052,16.5874015175642));
#49781=CARTESIAN_POINT('Ctrl Pts',(53.2634033247451,29.9814792165496,16.5878211995808));
#49782=CARTESIAN_POINT('Ctrl Pts',(53.2580560243589,29.971945789255,16.588526979446));
#49783=CARTESIAN_POINT('Ctrl Pts',(53.2558884291839,29.9680507535276,16.58881397811));
#49784=CARTESIAN_POINT('Ctrl Pts',(53.2517754072555,29.9606012460005,16.5893602456651));
#49785=CARTESIAN_POINT('Ctrl Pts',(53.2498277351428,29.9570480784841,16.589619661434));
#49786=CARTESIAN_POINT('Ctrl Pts',(53.2452187597631,29.9485787326357,16.5902353674182));
#49787=CARTESIAN_POINT('Ctrl Pts',(53.2425672520202,29.9436572212489,16.590591045347));
#49788=CARTESIAN_POINT('Ctrl Pts',(53.2332452772804,29.926178965255,16.5918469836628));
#49789=CARTESIAN_POINT('Ctrl Pts',(53.2266882273536,29.9135617712372,16.5927404757286));
#49790=CARTESIAN_POINT('Ctrl Pts',(53.1543099606901,29.770574106496,16.6027310574458));
#49791=CARTESIAN_POINT('Ctrl Pts',(53.1028523696274,29.6334035079832,16.6110794161731));
#49792=CARTESIAN_POINT('Ctrl Pts',(53.0594626196383,29.4628561496766,16.6213130063293));
#49793=CARTESIAN_POINT('Ctrl Pts',(53.0527458528725,29.4337300029892,16.6230547010837));
#49794=CARTESIAN_POINT('Ctrl Pts',(53.0466869925414,29.4044698473222,16.6248055079682));
#49795=CARTESIAN_POINT('Origin',(55.,29.,3.45145488139523));
#49796=CARTESIAN_POINT('',(53.0466869985623,29.4044698763992,17.581803907097));
#49797=CARTESIAN_POINT('',(53.0466869493682,29.4044696388253,17.4239266846335));
#49798=CARTESIAN_POINT('',(53.0466869980082,29.4044698737233,3.45145488139523));
#49799=CARTESIAN_POINT('',(53.0052506867316,28.9983447914819,16.808800702469));
#49800=CARTESIAN_POINT('Ctrl Pts',(53.0466869985623,29.4044698763992,17.581803907097));
#49801=CARTESIAN_POINT('Ctrl Pts',(53.0535381681538,29.4375563419659,17.5797310997435));
#49802=CARTESIAN_POINT('Ctrl Pts',(53.0612300479194,29.4704689730775,17.5776932705287));
#49803=CARTESIAN_POINT('Ctrl Pts',(53.0938908516641,29.5957598515763,17.5699744739283));
#49804=CARTESIAN_POINT('Ctrl Pts',(53.1246568243288,29.686492379341,17.5644613216537));
#49805=CARTESIAN_POINT('Ctrl Pts',(53.2128129037564,29.895674240343,17.5512636247914));
#49806=CARTESIAN_POINT('Ctrl Pts',(53.2756234352799,30.0113303012941,17.543550655876));
#49807=CARTESIAN_POINT('Ctrl Pts',(53.3581799806064,30.133006073438,17.5344254532823));
#49808=CARTESIAN_POINT('Ctrl Pts',(53.3671788955301,30.1459367160742,17.5334422965875));
#49809=CARTESIAN_POINT('Ctrl Pts',(53.3820533089232,30.1667789607287,17.5318348883462));
#49810=CARTESIAN_POINT('Ctrl Pts',(53.3878360472386,30.1747561543626,17.5312141567916));
#49811=CARTESIAN_POINT('Ctrl Pts',(53.3982526552653,30.1889039278494,17.5301032269704));
#49812=CARTESIAN_POINT('Ctrl Pts',(53.4028637108962,30.1950911167491,17.5296139144155));
#49813=CARTESIAN_POINT('Ctrl Pts',(53.4126786850509,30.2081027513415,17.5285774380986));
#49814=CARTESIAN_POINT('Ctrl Pts',(53.417890966705,30.2149206631241,17.5280299546567));
#49815=CARTESIAN_POINT('Ctrl Pts',(53.4318737956573,30.2329682867523,17.5265688674668));
#49816=CARTESIAN_POINT('Ctrl Pts',(53.4407208178199,30.2441378555194,17.5256522661133));
#49817=CARTESIAN_POINT('Ctrl Pts',(53.4842138998157,30.2978562227251,17.5211827777587));
#49818=CARTESIAN_POINT('Ctrl Pts',(53.5204830046658,30.3390544333428,17.5175652268632));
#49819=CARTESIAN_POINT('Ctrl Pts',(53.7005121844257,30.5272965410038,17.5000923933763));
#49820=CARTESIAN_POINT('Ctrl Pts',(53.8647087262536,30.6529955110114,17.4853582103319));
#49821=CARTESIAN_POINT('Ctrl Pts',(54.0724913873703,30.7662736313456,17.4694116497016));
#49822=CARTESIAN_POINT('Ctrl Pts',(54.100143311368,30.7805204186495,17.4673420523021));
#49823=CARTESIAN_POINT('Ctrl Pts',(54.1356841566394,30.7977921003784,17.4647582678335));
#49824=CARTESIAN_POINT('Ctrl Pts',(54.1432728207524,30.8014207891586,17.4642109214754));
#49825=CARTESIAN_POINT('Ctrl Pts',(54.1553006938363,30.807078986864,17.4633504928221));
#49826=CARTESIAN_POINT('Ctrl Pts',(54.1597246844119,30.8091403422196,17.4630355261175));
#49827=CARTESIAN_POINT('Ctrl Pts',(54.1680937508903,30.8130025816279,17.4624425959009));
#49828=CARTESIAN_POINT('Ctrl Pts',(54.1720370909655,30.8148068188967,17.4621644396664));
#49829=CARTESIAN_POINT('Ctrl Pts',(54.1812359971743,30.8189794662923,17.4615183580629));
#49830=CARTESIAN_POINT('Ctrl Pts',(54.1864959767656,30.8213379689892,17.4611510354285));
#49831=CARTESIAN_POINT('Ctrl Pts',(54.2034378144508,30.8288464209236,17.4599744664441));
#49832=CARTESIAN_POINT('Ctrl Pts',(54.2151591899121,30.8339071594355,17.4591704019459));
#49833=CARTESIAN_POINT('Ctrl Pts',(54.2430500915498,30.8456327461047,17.4572787816351));
#49834=CARTESIAN_POINT('Ctrl Pts',(54.25926050137,30.8521982714125,17.4561964220564));
#49835=CARTESIAN_POINT('Ctrl Pts',(54.3187665994462,30.8753931554573,17.4522779180653));
#49836=CARTESIAN_POINT('Ctrl Pts',(54.3625547026584,30.890725390171,17.4494990516173));
#49837=CARTESIAN_POINT('Ctrl Pts',(54.5585261018975,30.9517604376265,17.4373591276503));
#49838=CARTESIAN_POINT('Ctrl Pts',(54.7153106748265,30.9807126760047,17.4283769401918));
#49839=CARTESIAN_POINT('Ctrl Pts',(54.9333902267673,30.9945293017382,17.4153048114855));
#49840=CARTESIAN_POINT('Ctrl Pts',(54.9930409514654,30.9956288600365,17.4116769903123));
#49841=CARTESIAN_POINT('Ctrl Pts',(55.0677068979847,30.9936575140025,17.4070284306335));
#49842=CARTESIAN_POINT('Ctrl Pts',(55.082761010887,30.9930893363719,17.406085786113));
#49843=CARTESIAN_POINT('Ctrl Pts',(55.1066445569654,30.9919168639485,17.4045810847275));
#49844=CARTESIAN_POINT('Ctrl Pts',(55.1154790846982,30.9914242218461,17.4040224995904));
#49845=CARTESIAN_POINT('Ctrl Pts',(55.1319745795703,30.9903942445524,17.4029756780733));
#49846=CARTESIAN_POINT('Ctrl Pts',(55.1396363132616,30.9898714118591,17.4024879021486));
#49847=CARTESIAN_POINT('Ctrl Pts',(55.1567146650854,30.9886068735467,17.4013970752679));
#49848=CARTESIAN_POINT('Ctrl Pts',(55.166129370669,30.9878425015409,17.4007933287865));
#49849=CARTESIAN_POINT('Ctrl Pts',(55.1937551486907,30.9854019626926,17.3990144784027));
#49850=CARTESIAN_POINT('Ctrl Pts',(55.2119486220281,30.9835422244071,17.3978336941341));
#49851=CARTESIAN_POINT('Ctrl Pts',(55.2531565645805,30.978756544452,17.3951373853378));
#49852=CARTESIAN_POINT('Ctrl Pts',(55.2761503950709,30.9756787678862,17.3936173216041));
#49853=CARTESIAN_POINT('Ctrl Pts',(55.3518863522303,30.9641933982191,17.3885581173148));
#49854=CARTESIAN_POINT('Ctrl Pts',(55.4043411466839,30.9540693785939,17.3849688916255));
#49855=CARTESIAN_POINT('Ctrl Pts',(55.5638922877239,30.9165758966246,17.3738002372527));
#49856=CARTESIAN_POINT('Ctrl Pts',(55.6691691546217,30.8824045962201,17.366065227641));
#49857=CARTESIAN_POINT('Ctrl Pts',(55.8568452662251,30.8037445639532,17.351914665903));
#49858=CARTESIAN_POINT('Ctrl Pts',(55.9400158894148,30.7618321367739,17.3455051536004));
#49859=CARTESIAN_POINT('Ctrl Pts',(56.0291031993863,30.7088262697652,17.3386962997571));
#49860=CARTESIAN_POINT('Ctrl Pts',(56.0381973701369,30.7033164261879,17.3380019966732));
#49861=CARTESIAN_POINT('Ctrl Pts',(56.0518635063517,30.6948864694617,17.33696029324));
#49862=CARTESIAN_POINT('Ctrl Pts',(56.0564681614387,30.6920200961869,17.3366095885707));
#49863=CARTESIAN_POINT('Ctrl Pts',(56.0647052140231,30.6868458403245,17.335982824003));
#49864=CARTESIAN_POINT('Ctrl Pts',(56.0683418732225,30.6845449607527,17.3357063220728));
#49865=CARTESIAN_POINT('Ctrl Pts',(56.0762766320209,30.6794886835234,17.3351035033189));
#49866=CARTESIAN_POINT('Ctrl Pts',(56.0805716037684,30.6767285520455,17.3347775024975));
#49867=CARTESIAN_POINT('Ctrl Pts',(56.0927817748795,30.6688153754126,17.3338514191313));
#49868=CARTESIAN_POINT('Ctrl Pts',(56.1006711648465,30.663622481183,17.333253893963));
#49869=CARTESIAN_POINT('Ctrl Pts',(56.1533820446094,30.6283884115258,17.3292652751113));
#49870=CARTESIAN_POINT('Ctrl Pts',(56.1970099180198,30.5965924183431,17.3259813070043));
#49871=CARTESIAN_POINT('Ctrl Pts',(56.3836949436426,30.4485763496265,17.3117513026923));
#49872=CARTESIAN_POINT('Ctrl Pts',(56.5115330081187,30.3146334040807,17.3014375781602));
#49873=CARTESIAN_POINT('Ctrl Pts',(56.6489110046309,30.123704920779,17.2872816866688));
#49874=CARTESIAN_POINT('Ctrl Pts',(56.6770544045998,30.0812530293964,17.2841701925491));
#49875=CARTESIAN_POINT('Ctrl Pts',(56.7110752607927,30.0254066092997,17.2800961808225));
#49876=CARTESIAN_POINT('Ctrl Pts',(56.7184739950843,30.012958228827,17.2791893039776));
#49877=CARTESIAN_POINT('Ctrl Pts',(56.730066196122,29.9929617571221,17.2777339692156));
#49878=CARTESIAN_POINT('Ctrl Pts',(56.7343474153583,29.9854649324761,17.2771886705749));
#49879=CARTESIAN_POINT('Ctrl Pts',(56.7419801946523,29.9718954016438,17.2762021199146));
#49880=CARTESIAN_POINT('Ctrl Pts',(56.7453490196844,29.9658325257545,17.2757614926161));
#49881=CARTESIAN_POINT('Ctrl Pts',(56.7532029653917,29.9515224935127,17.2747218119821));
#49882=CARTESIAN_POINT('Ctrl Pts',(56.7576615909594,29.9432610562505,17.2741218332623));
#49883=CARTESIAN_POINT('Ctrl Pts',(56.7705014750913,29.9190627372125,17.2723649969866));
#49884=CARTESIAN_POINT('Ctrl Pts',(56.7787252845113,29.9030438059255,17.2712026703299));
#49885=CARTESIAN_POINT('Ctrl Pts',(56.7968455484423,29.8665397520384,17.2685547410683));
#49886=CARTESIAN_POINT('Ctrl Pts',(56.8066105386457,29.8459925288005,17.2670648289233));
#49887=CARTESIAN_POINT('Ctrl Pts',(56.8374970839021,29.7780272323461,17.2621372635663));
#49888=CARTESIAN_POINT('Ctrl Pts',(56.8571181352503,29.7299543749127,17.258652379659));
#49889=CARTESIAN_POINT('Ctrl Pts',(56.9184682066805,29.5610965237657,17.246424303392));
#49890=CARTESIAN_POINT('Ctrl Pts',(56.9504561619717,29.4371105736198,17.2374449395276));
#49891=CARTESIAN_POINT('Ctrl Pts',(56.9825844734383,29.2335147737168,17.2231647760945));
#49892=CARTESIAN_POINT('Ctrl Pts',(56.9902294348302,29.1554347421957,17.2178021227409));
#49893=CARTESIAN_POINT('Ctrl Pts',(56.9936658735568,29.0665921570856,17.2119636188883));
#49894=CARTESIAN_POINT('Ctrl Pts',(56.9939892182602,29.056081545185,17.211277095355));
#49895=CARTESIAN_POINT('Ctrl Pts',(56.9943527715682,29.0401712751975,17.2102447357551));
#49896=CARTESIAN_POINT('Ctrl Pts',(56.9944541913453,29.0347733963088,17.2098956806203));
#49897=CARTESIAN_POINT('Ctrl Pts',(56.9945970495816,29.0250734938898,17.2092706584106));
#49898=CARTESIAN_POINT('Ctrl Pts',(56.9946464868534,29.0207717076191,17.2089942603481));
#49899=CARTESIAN_POINT('Ctrl Pts',(56.9947243286119,29.0113440975971,17.2083902563178));
#49900=CARTESIAN_POINT('Ctrl Pts',(56.9947468936236,29.0062183196711,17.2080629756295));
#49901=CARTESIAN_POINT('Ctrl Pts',(56.9947549257927,28.9915519540209,17.2071295754828));
#49902=CARTESIAN_POINT('Ctrl Pts',(56.9946917054074,28.9820113263388,17.2065260772961));
#49903=CARTESIAN_POINT('Ctrl Pts',(56.993783157081,28.9161835186509,17.2023852998064));
#49904=CARTESIAN_POINT('Ctrl Pts',(56.9906238214904,28.8599480384416,17.198964739783));
#49905=CARTESIAN_POINT('Ctrl Pts',(56.975669469355,28.7085549220737,17.1898942195664));
#49906=CARTESIAN_POINT('Ctrl Pts',(56.9593900436916,28.6139913383113,17.1843726036092));
#49907=CARTESIAN_POINT('Ctrl Pts',(56.9048245527289,28.3934266316467,17.1711625266656));
#49908=CARTESIAN_POINT('Ctrl Pts',(56.8607571770135,28.2693400215482,17.1634458349897));
#49909=CARTESIAN_POINT('Ctrl Pts',(56.7981092238956,28.1362414063239,17.1543165136526));
#49910=CARTESIAN_POINT('Ctrl Pts',(56.7912324572086,28.1220695065229,17.1533334531046));
#49911=CARTESIAN_POINT('Ctrl Pts',(56.77978296218,28.0991685858964,17.1517261710412));
#49912=CARTESIAN_POINT('Ctrl Pts',(56.7753120427761,28.0903892182327,17.1511054685904));
#49913=CARTESIAN_POINT('Ctrl Pts',(56.76722380808,28.0747934731403,17.1499945711783));
#49914=CARTESIAN_POINT('Ctrl Pts',(56.7636316076198,28.0679642415244,17.1495052617317));
#49915=CARTESIAN_POINT('Ctrl Pts',(56.7559605674234,28.0535837570758,17.148468771439));
#49916=CARTESIAN_POINT('Ctrl Pts',(56.7518724462376,28.0460376592555,17.1479212707881));
#49917=CARTESIAN_POINT('Ctrl Pts',(56.740867253046,28.0260329418747,17.1464600888447));
#49918=CARTESIAN_POINT('Ctrl Pts',(56.7338652603423,28.0136218450065,17.1455434092596));
#49919=CARTESIAN_POINT('Ctrl Pts',(56.6992519433195,27.9537769300455,17.1410728918009));
#49920=CARTESIAN_POINT('Ctrl Pts',(56.6698261923115,27.9074253324099,17.1374543538894));
#49921=CARTESIAN_POINT('Ctrl Pts',(56.5211582989487,27.6933027768657,17.1199678266363));
#49922=CARTESIAN_POINT('Ctrl Pts',(56.3783633923795,27.5434727421367,17.1052191104057));
#49923=CARTESIAN_POINT('Ctrl Pts',(56.1906809541047,27.3992929842158,17.089274136507));
#49924=CARTESIAN_POINT('Ctrl Pts',(56.1657183216661,27.3810234314543,17.0872162566158));
#49925=CARTESIAN_POINT('Ctrl Pts',(56.1334515375371,27.3585416095927,17.0846449066322));
#49926=CARTESIAN_POINT('Ctrl Pts',(56.1265333593992,27.3537859703194,17.0840986509278));
#49927=CARTESIAN_POINT('Ctrl Pts',(56.1155488961026,27.3463367914275,17.0832395438774));
#49928=CARTESIAN_POINT('Ctrl Pts',(56.1115024952881,27.3436143108617,17.0829248176192));
#49929=CARTESIAN_POINT('Ctrl Pts',(56.1038385121663,27.3384985961421,17.0823320733395));
#49930=CARTESIAN_POINT('Ctrl Pts',(56.1002231481101,27.3361023466941,17.0820538643899));
#49931=CARTESIAN_POINT('Ctrl Pts',(56.0917790326205,27.3305451749219,17.0814073035615));
#49932=CARTESIAN_POINT('Ctrl Pts',(56.0869443507301,27.327393396685,17.0810395573126));
#49933=CARTESIAN_POINT('Ctrl Pts',(56.0713401172818,27.3173170694722,17.0798602398985));
#49934=CARTESIAN_POINT('Ctrl Pts',(56.0605172982703,27.3104750455651,17.0790538845301));
#49935=CARTESIAN_POINT('Ctrl Pts',(55.9651537695647,27.2514651179554,17.0720428720727));
#49936=CARTESIAN_POINT('Ctrl Pts',(55.8768797952597,27.2055688613344,17.0661920095469));
#49937=CARTESIAN_POINT('Ctrl Pts',(55.6282143070381,27.099034524664,17.0504248779519));
#49938=CARTESIAN_POINT('Ctrl Pts',(55.4628842776193,27.0521664452302,17.0406303679596));
#49939=CARTESIAN_POINT('Ctrl Pts',(55.2712991874232,27.0236566834948,17.0286779132244));
#49940=CARTESIAN_POINT('Ctrl Pts',(55.2489388964172,27.0207159082614,17.027275287131));
#49941=CARTESIAN_POINT('Ctrl Pts',(55.2164400850321,27.0170011409015,17.0252236209845));
#49942=CARTESIAN_POINT('Ctrl Pts',(55.2063374220252,27.0159244853656,17.0245840145233));
#49943=CARTESIAN_POINT('Ctrl Pts',(55.1884826768431,27.0141595216324,17.0234502209378));
#49944=CARTESIAN_POINT('Ctrl Pts',(55.1807339086403,27.0134393096412,17.0229570389746));
#49945=CARTESIAN_POINT('Ctrl Pts',(55.1646618709513,27.0120403005558,17.0219316872968));
#49946=CARTESIAN_POINT('Ctrl Pts',(55.1563381695954,27.0113683921812,17.0213993129675));
#49947=CARTESIAN_POINT('Ctrl Pts',(55.134851106143,27.0097696433391,17.0200214397622));
#49948=CARTESIAN_POINT('Ctrl Pts',(55.1216824918756,27.0089211339618,17.0191735226355));
#49949=CARTESIAN_POINT('Ctrl Pts',(55.0649970952024,27.005833095605,17.0155080491662));
#49950=CARTESIAN_POINT('Ctrl Pts',(55.0214245833406,27.0048892852,17.0126507552212));
#49951=CARTESIAN_POINT('Ctrl Pts',(54.8190704443571,27.0071355050272,16.9991873921537));
#49952=CARTESIAN_POINT('Ctrl Pts',(54.6610791641538,27.0278534440817,16.9880583516065));
#49953=CARTESIAN_POINT('Ctrl Pts',(54.4228685544033,27.0885791987382,16.970985457503));
#49954=CARTESIAN_POINT('Ctrl Pts',(54.3399775022593,27.1155945106876,16.9650016216296));
#49955=CARTESIAN_POINT('Ctrl Pts',(54.2492525370051,27.1518878508919,16.9585836787932));
#49956=CARTESIAN_POINT('Ctrl Pts',(54.2394270271168,27.15590970026,16.9578904551627));
#49957=CARTESIAN_POINT('Ctrl Pts',(54.2246340220044,27.1621032284541,16.9568500476466));
#49958=CARTESIAN_POINT('Ctrl Pts',(54.2196426841745,27.164216950726,16.9564995713297));
#49959=CARTESIAN_POINT('Ctrl Pts',(54.2107042831989,27.1680452102899,16.9558730486546));
#49960=CARTESIAN_POINT('Ctrl Pts',(54.206754110838,27.1697521915009,16.9555965617919));
#49961=CARTESIAN_POINT('Ctrl Pts',(54.2027934097233,27.1714789541209,16.9553197365329));
#49962=CARTESIAN_POINT('Ctrl Pts',(54.2027774475001,27.1714859134837,16.9553186208917));
#49963=CARTESIAN_POINT('Ctrl Pts',(54.2027457625764,27.1714997282734,16.9553164063629));
#49964=CARTESIAN_POINT('Ctrl Pts',(54.2027300387601,27.1715065841795,16.955315307397));
#49965=CARTESIAN_POINT('Ctrl Pts',(54.2026988231264,27.1715201953148,16.9553131256925));
#49966=CARTESIAN_POINT('Ctrl Pts',(54.2026833324532,27.1715269500379,16.9553120430336));
#49967=CARTESIAN_POINT('Ctrl Pts',(54.2026525813444,27.1715403595539,16.9553098938193));
#49968=CARTESIAN_POINT('Ctrl Pts',(54.2026373204142,27.1715470145555,16.9553088272291));
#49969=CARTESIAN_POINT('Ctrl Pts',(54.2026070256313,27.171560225986,16.9553067099308));
#49970=CARTESIAN_POINT('Ctrl Pts',(54.2025919911115,27.171566782699,16.9553056591759));
#49971=CARTESIAN_POINT('Ctrl Pts',(54.2025621435818,27.1715797999605,16.9553035731585));
#49972=CARTESIAN_POINT('Ctrl Pts',(54.202547331179,27.1715862602377,16.9553025379383));
#49973=CARTESIAN_POINT('Ctrl Pts',(54.2025179247056,27.1715990859941,16.9553004827678));
#49974=CARTESIAN_POINT('Ctrl Pts',(54.2025033308667,27.1716054513659,16.9552994628335));
#49975=CARTESIAN_POINT('Ctrl Pts',(54.2024743579551,27.1716180888482,16.9552974379851));
#49976=CARTESIAN_POINT('Ctrl Pts',(54.2024599790974,27.1716243608588,16.9552964330859));
#49977=CARTESIAN_POINT('Ctrl Pts',(54.2024314323554,27.171636813255,16.955294438042));
#49978=CARTESIAN_POINT('Ctrl Pts',(54.2024172647329,27.1716429935205,16.9552934479155));
#49979=CARTESIAN_POINT('Ctrl Pts',(54.2023891377923,27.171655263573,16.9552914822301));
#49980=CARTESIAN_POINT('Ctrl Pts',(54.2023751781523,27.1716613534948,16.9552905066487));
#49981=CARTESIAN_POINT('Ctrl Pts',(54.2023474637385,27.1716734443429,16.9552885698126));
#49982=CARTESIAN_POINT('Ctrl Pts',(54.2023337087108,27.1716794453745,16.9552876085402));
#49983=CARTESIAN_POINT('Ctrl Pts',(54.202306399932,27.1716913599916,16.9552857000709));
#49984=CARTESIAN_POINT('Ctrl Pts',(54.2022928460989,27.1716972736077,16.9552847528682));
#49985=CARTESIAN_POINT('Ctrl Pts',(54.2022659365562,27.1717090147535,16.9552828723178));
#49986=CARTESIAN_POINT('Ctrl Pts',(54.2022525807084,27.1717148423384,16.9552819389602));
#49987=CARTESIAN_POINT('Ctrl Pts',(54.2022260638523,27.1717264128393,16.95528008587));
#49988=CARTESIAN_POINT('Ctrl Pts',(54.2022129028588,27.1717321557438,16.9552791661382));
#49989=CARTESIAN_POINT('Ctrl Pts',(54.2021867718216,27.1717435585663,16.9552773400276));
#49990=CARTESIAN_POINT('Ctrl Pts',(54.2021738022083,27.1717492182916,16.9552764336786));
#49991=CARTESIAN_POINT('Ctrl Pts',(54.2021477040113,27.1717606074448,16.9552746098798));
#49992=CARTESIAN_POINT('Ctrl Pts',(54.202134575331,27.1717663369189,16.9552736924234));
#49993=CARTESIAN_POINT('Ctrl Pts',(54.2021083594329,27.1717777781088,16.9552718604166));
#49994=CARTESIAN_POINT('Ctrl Pts',(54.2020952722161,27.1717834898229,16.9552709458663));
#49995=CARTESIAN_POINT('Ctrl Pts',(54.2020691376536,27.1717948961843,16.9552691195604));
#49996=CARTESIAN_POINT('Ctrl Pts',(54.2020560909416,27.1718005905539,16.9552682078491));
#49997=CARTESIAN_POINT('Ctrl Pts',(54.2020300393818,27.1718119613529,16.9552663873605));
#49998=CARTESIAN_POINT('Ctrl Pts',(54.2020170336725,27.1718176381574,16.955265478523));
#49999=CARTESIAN_POINT('Ctrl Pts',(54.2019910627921,27.1718289744019,16.9552636636891));
#50000=CARTESIAN_POINT('Ctrl Pts',(54.2019780975008,27.1718346338934,16.9552627576844));
#50001=CARTESIAN_POINT('Ctrl Pts',(54.2019522079513,27.1718459352929,16.9552609485507));
#50002=CARTESIAN_POINT('Ctrl Pts',(54.2019392832992,27.1718515773718,16.9552600453941));
#50003=CARTESIAN_POINT('Ctrl Pts',(54.2019134729174,27.1718628448645,16.9552582418092));
#50004=CARTESIAN_POINT('Ctrl Pts',(54.201900587917,27.1718684699589,16.9552573414317));
#50005=CARTESIAN_POINT('Ctrl Pts',(54.2018748580515,27.17187970295,16.9552555434897));
#50006=CARTESIAN_POINT('Ctrl Pts',(54.2018620128074,27.1718853110112,16.9552546458986));
#50007=CARTESIAN_POINT('Ctrl Pts',(54.2018363625221,27.1718965099035,16.9552528535338));
#50008=CARTESIAN_POINT('Ctrl Pts',(54.2018235570324,27.1719021009293,16.9552519587288));
#50009=CARTESIAN_POINT('Ctrl Pts',(54.2017979855248,27.171913266067,16.9552501718851));
#50010=CARTESIAN_POINT('Ctrl Pts',(54.2017852197049,27.1719188400915,16.9552492798603));
#50011=CARTESIAN_POINT('Ctrl Pts',(54.2017597250103,27.1719299723268,16.9552474984002));
#50012=CARTESIAN_POINT('Ctrl Pts',(54.2017469974417,27.1719355299664,16.9552466090563));
#50013=CARTESIAN_POINT('Ctrl Pts',(54.201721582803,27.1719466278773,16.9552448332063));
#50014=CARTESIAN_POINT('Ctrl Pts',(54.2017088946066,27.1719521686396,16.9552439466216));
#50015=CARTESIAN_POINT('Ctrl Pts',(54.201683555894,27.1719632340239,16.955242176093));
#50016=CARTESIAN_POINT('Ctrl Pts',(54.2016709058875,27.1719687584223,16.9552412921847));
#50017=CARTESIAN_POINT('Ctrl Pts',(54.2016456455027,27.1719797902253,16.9552395271451));
#50018=CARTESIAN_POINT('Ctrl Pts',(54.2016330344284,27.1719852979329,16.9552386459652));
#50019=CARTESIAN_POINT('Ctrl Pts',(54.2016078487016,27.1719962977517,16.9552368861581));
#50020=CARTESIAN_POINT('Ctrl Pts',(54.2015952750726,27.1720017894151,16.9552360076024));
#50021=CARTESIAN_POINT('Ctrl Pts',(54.2015701672082,27.1720127558445,16.9552342532515));
#50022=CARTESIAN_POINT('Ctrl Pts',(54.2015576319523,27.1720182310555,16.9552333773849));
#50023=CARTESIAN_POINT('Ctrl Pts',(54.1967690964865,27.1741098498789,16.9548987931142));
#50024=CARTESIAN_POINT('Ctrl Pts',(54.192001225686,27.176214731155,16.9545662203758));
#50025=CARTESIAN_POINT('Ctrl Pts',(54.1781245656607,27.1824059861494,16.953599785945));
#50026=CARTESIAN_POINT('Ctrl Pts',(54.1690379795318,27.1865421540539,16.9529688485702));
#50027=CARTESIAN_POINT('Ctrl Pts',(54.1482171172537,27.1962090614782,16.9515266383903));
#50028=CARTESIAN_POINT('Ctrl Pts',(54.1365048537253,27.2017864474003,16.9507179441833));
#50029=CARTESIAN_POINT('Ctrl Pts',(54.0119497578688,27.2625972458452,16.9421368224733));
#50030=CARTESIAN_POINT('Ctrl Pts',(53.9044964916336,27.3282667851673,16.9348896110096));
#50031=CARTESIAN_POINT('Ctrl Pts',(53.6977385654398,27.4831782467005,16.9198861400974));
#50032=CARTESIAN_POINT('Ctrl Pts',(53.5997672214793,27.5731238130959,16.9121501946306));
#50033=CARTESIAN_POINT('Ctrl Pts',(53.4952419008201,27.6902963111776,16.9024836744009));
#50034=CARTESIAN_POINT('Ctrl Pts',(53.4793644126827,27.7087649244213,16.9009716779454));
#50035=CARTESIAN_POINT('Ctrl Pts',(53.4575913232255,27.7350499350715,16.898833272468));
#50036=CARTESIAN_POINT('Ctrl Pts',(53.4514086539015,27.7426265350641,16.8982184170669));
#50037=CARTESIAN_POINT('Ctrl Pts',(53.440758260902,27.7558758515742,16.897145696228));
#50038=CARTESIAN_POINT('Ctrl Pts',(53.4362651284139,27.761527978995,16.8966888514168));
#50039=CARTESIAN_POINT('Ctrl Pts',(53.4269466128665,27.7733817435062,16.8957322868379));
#50040=CARTESIAN_POINT('Ctrl Pts',(53.4221269977021,27.7795877370038,16.8952323508454));
#50041=CARTESIAN_POINT('Ctrl Pts',(53.4107759066309,27.7943836477883,16.894042398161));
#50042=CARTESIAN_POINT('Ctrl Pts',(53.4042772726416,27.8029983385437,16.893351117135));
#50043=CARTESIAN_POINT('Ctrl Pts',(53.3826411528737,27.8321688481488,16.8910152409741));
#50044=CARTESIAN_POINT('Ctrl Pts',(53.3678289568953,27.8529617155225,16.8893582696848));
#50045=CARTESIAN_POINT('Ctrl Pts',(53.3139491573439,27.9317538349862,16.8831062916893));
#50046=CARTESIAN_POINT('Ctrl Pts',(53.2775445556309,27.9915047351612,16.8784161761032));
#50047=CARTESIAN_POINT('Ctrl Pts',(53.2164548514914,28.1047635971426,16.8696291260683));
#50048=CARTESIAN_POINT('Ctrl Pts',(53.1908559343621,28.1576944646641,16.8655616077109));
#50049=CARTESIAN_POINT('Ctrl Pts',(53.1427675624629,28.2694702538247,16.8570952172123));
#50050=CARTESIAN_POINT('Ctrl Pts',(53.1206511797414,28.3284092350215,16.8526976972126));
#50051=CARTESIAN_POINT('Ctrl Pts',(53.0775342578781,28.4622378848971,16.8429585405376));
#50052=CARTESIAN_POINT('Ctrl Pts',(53.0580484270442,28.5375181385459,16.8376449679266));
#50053=CARTESIAN_POINT('Ctrl Pts',(53.040968361574,28.6240572391024,16.8318525687653));
#50054=CARTESIAN_POINT('Ctrl Pts',(53.0390156215005,28.6343797071378,16.8311667096999));
#50055=CARTESIAN_POINT('Ctrl Pts',(53.0361832923671,28.6500276804763,16.8301351486327));
#50056=CARTESIAN_POINT('Ctrl Pts',(53.03524365311,28.655341930869,16.8297862347986));
#50057=CARTESIAN_POINT('Ctrl Pts',(53.0335937438138,28.6648992613888,16.8291613612945));
#50058=CARTESIAN_POINT('Ctrl Pts',(53.0328756258493,28.6691408652251,16.8288849715844));
#50059=CARTESIAN_POINT('Ctrl Pts',(53.0315009213921,28.6774233448767,16.828347095018));
#50060=CARTESIAN_POINT('Ctrl Pts',(53.030843055287,28.6814638973008,16.8280855343157));
#50061=CARTESIAN_POINT('Ctrl Pts',(53.0293981313878,28.6905140507565,16.8275015017758));
#50062=CARTESIAN_POINT('Ctrl Pts',(53.0286177249731,28.6955247064408,16.8271793958916));
#50063=CARTESIAN_POINT('Ctrl Pts',(53.0267038510002,28.7081287718775,16.8263721617139));
#50064=CARTESIAN_POINT('Ctrl Pts',(53.0255950869262,28.7157259262221,16.8258883385404));
#50065=CARTESIAN_POINT('Ctrl Pts',(53.0117703005564,28.8144369969873,16.8196352878344));
#50066=CARTESIAN_POINT('Ctrl Pts',(53.0053270402533,28.9063285088114,16.8141802815779));
#50067=CARTESIAN_POINT('Ctrl Pts',(53.0052506867316,28.9983447914819,16.808800702469));
#50068=CARTESIAN_POINT('Ctrl Pts',(53.0052506883683,28.9983428202296,16.808800817715));
#50069=CARTESIAN_POINT('Ctrl Pts',(53.0051373356856,29.1347855826284,16.8008239164537));
#50070=CARTESIAN_POINT('Ctrl Pts',(53.0190227966867,29.2708706932225,16.793027499536));
#50071=CARTESIAN_POINT('Ctrl Pts',(53.046686998698,29.4044698770549,16.7848524498588));
#50072=CARTESIAN_POINT('Ctrl Pts',(53.0466869925414,29.4044698473222,16.6248055079682));
#50073=CARTESIAN_POINT('Ctrl Pts',(53.0380141080535,29.3625857410172,16.627311679928));
#50074=CARTESIAN_POINT('Ctrl Pts',(53.0306892831047,29.3204270586987,16.6298366943859));
#50075=CARTESIAN_POINT('Ctrl Pts',(53.016097694892,29.216771308831,16.6360937083062));
#50076=CARTESIAN_POINT('Ctrl Pts',(53.0103280254816,29.155120766903,16.6398574975813));
#50077=CARTESIAN_POINT('Ctrl Pts',(53.0067418712798,29.0785377137215,16.644631910438));
#50078=CARTESIAN_POINT('Ctrl Pts',(53.0062145424458,29.0637626142266,16.6455574981895));
#50079=CARTESIAN_POINT('Ctrl Pts',(53.0056378785134,29.0402861853452,16.6470358351619));
#50080=CARTESIAN_POINT('Ctrl Pts',(53.0054811477803,29.0315878557825,16.6475852455396));
#50081=CARTESIAN_POINT('Ctrl Pts',(53.0052930147921,29.0151932821328,16.6486240301248));
#50082=CARTESIAN_POINT('Ctrl Pts',(53.0052492435961,29.0074973183083,16.6491130106753));
#50083=CARTESIAN_POINT('Ctrl Pts',(53.0052509714746,28.9901440891952,16.6502187237599));
#50084=CARTESIAN_POINT('Ctrl Pts',(53.0053220645592,28.9804870745547,16.6508362399704));
#50085=CARTESIAN_POINT('Ctrl Pts',(53.0057460131162,28.9514979524699,16.6526967159222));
#50086=CARTESIAN_POINT('Ctrl Pts',(53.0063098203821,28.9321705291095,16.653946173717));
#50087=CARTESIAN_POINT('Ctrl Pts',(53.0082417662792,28.8879905375205,16.6568238571183));
#50088=CARTESIAN_POINT('Ctrl Pts',(53.0097942630168,28.8631496622685,16.6584575425616));
#50089=CARTESIAN_POINT('Ctrl Pts',(53.0166096057066,28.7793278987833,16.6640243318593));
#50090=CARTESIAN_POINT('Ctrl Pts',(53.0240331458528,28.7205585069491,16.6680193413029));
#50091=CARTESIAN_POINT('Ctrl Pts',(53.0573871997508,28.5264372437851,16.6814992160782));
#50092=CARTESIAN_POINT('Ctrl Pts',(53.0947158109967,28.3934567608155,16.6912276925873));
#50093=CARTESIAN_POINT('Ctrl Pts',(53.1496828980849,28.2546902706706,16.7014785847141));
#50094=CARTESIAN_POINT('Ctrl Pts',(53.1540131117373,28.2440288454328,16.7022665855961));
#50095=CARTESIAN_POINT('Ctrl Pts',(53.1765098094134,28.189985784901,16.7062613026342));
#50096=CARTESIAN_POINT('Ctrl Pts',(53.1961158324718,28.1472150338447,16.7094241255423));
#50097=CARTESIAN_POINT('Ctrl Pts',(53.2210916112852,28.0974552110499,16.7130731610436));
#50098=CARTESIAN_POINT('Ctrl Pts',(53.225016031919,28.0897615307207,16.7136364654033));
#50099=CARTESIAN_POINT('Ctrl Pts',(53.2314941476769,28.0772626495191,16.7145498319228));
#50100=CARTESIAN_POINT('Ctrl Pts',(53.2340177048106,28.072442075964,16.7149016699997));
#50101=CARTESIAN_POINT('Ctrl Pts',(53.2385729259767,28.0638265366592,16.7155296381796));
#50102=CARTESIAN_POINT('Ctrl Pts',(53.2405971714556,28.0600277777576,16.7158062178911));
#50103=CARTESIAN_POINT('Ctrl Pts',(53.2450427364248,28.051749774431,16.7164082513786));
#50104=CARTESIAN_POINT('Ctrl Pts',(53.2474689113033,28.0472732438913,16.7167333953908));
#50105=CARTESIAN_POINT('Ctrl Pts',(53.2544136559397,28.0345758047717,16.7176545933729));
#50106=CARTESIAN_POINT('Ctrl Pts',(53.2589731841233,28.0263772825995,16.7182481322152));
#50107=CARTESIAN_POINT('Ctrl Pts',(53.2894205873233,27.9725274605633,16.7221403205046));
#50108=CARTESIAN_POINT('Ctrl Pts',(53.3170460216686,27.9278765433461,16.7253377004572));
#50109=CARTESIAN_POINT('Ctrl Pts',(53.4404256656817,27.7450032083083,16.7385291408264));
#50110=CARTESIAN_POINT('Ctrl Pts',(53.5516896782469,27.6180835154592,16.7479816178534));
#50111=CARTESIAN_POINT('Ctrl Pts',(53.7272075343015,27.4626567812544,16.7619475594429));
#50112=CARTESIAN_POINT('Ctrl Pts',(53.779009037906,27.4212015512862,16.7659680280247));
#50113=CARTESIAN_POINT('Ctrl Pts',(53.8453794138403,27.3733099664234,16.7710585396867));
#50114=CARTESIAN_POINT('Ctrl Pts',(53.8580896429777,27.3643625467501,16.7720306862463));
#50115=CARTESIAN_POINT('Ctrl Pts',(53.8782873935378,27.3504944284185,16.7735719465051));
#50116=CARTESIAN_POINT('Ctrl Pts',(53.8857058947758,27.3454739515399,16.7741372932323));
#50117=CARTESIAN_POINT('Ctrl Pts',(53.8994798388177,27.3362870787299,16.7751857245628));
#50118=CARTESIAN_POINT('Ctrl Pts',(53.9058257852833,27.3321066896175,16.7756682747216));
#50119=CARTESIAN_POINT('Ctrl Pts',(53.9199717302421,27.3229035311781,16.7767429534923));
#50120=CARTESIAN_POINT('Ctrl Pts',(53.9277831567242,27.3178987350833,16.777335733035));
#50121=CARTESIAN_POINT('Ctrl Pts',(53.9504072728413,27.3036250431982,16.7790508641112));
#50122=CARTESIAN_POINT('Ctrl Pts',(53.9653069096655,27.2944962434085,16.780178295169));
#50123=CARTESIAN_POINT('Ctrl Pts',(54.1055675975932,27.2110749415363,16.7907748335484));
#50124=CARTESIAN_POINT('Ctrl Pts',(54.2385716978849,27.1505477905933,16.8007485881494));
#50125=CARTESIAN_POINT('Ctrl Pts',(54.3842491664793,27.1026498761366,16.8114250724037));
#50126=CARTESIAN_POINT('Ctrl Pts',(54.3915609796176,27.1002925121066,16.811960178837));
#50127=CARTESIAN_POINT('Ctrl Pts',(54.5136213425887,27.0617166462131,16.8208791403012));
#50128=CARTESIAN_POINT('Ctrl Pts',(54.631412340556,27.0359086378257,16.8292996491075));
#50129=CARTESIAN_POINT('Ctrl Pts',(54.7665220858822,27.0188977578712,16.8383183593856));
#50130=CARTESIAN_POINT('Ctrl Pts',(54.7822478558811,27.0171076501075,16.8393581526558));
#50131=CARTESIAN_POINT('Ctrl Pts',(54.8044281941343,27.01484986433,16.8408092347665));
#50132=CARTESIAN_POINT('Ctrl Pts',(54.8108658040319,27.0142261832951,16.8412285619085));
#50133=CARTESIAN_POINT('Ctrl Pts',(54.8216999854387,27.013229722933,16.8419310570466));
#50134=CARTESIAN_POINT('Ctrl Pts',(54.8260949280315,27.0128402036477,16.8422151395493));
#50135=CARTESIAN_POINT('Ctrl Pts',(54.835068249673,27.0120749053375,16.8427933006729));
#50136=CARTESIAN_POINT('Ctrl Pts',(54.8396466892665,27.0117003543164,16.8430873102334));
#50137=CARTESIAN_POINT('Ctrl Pts',(54.8513205337262,27.0107859306266,16.8438345433273));
#50138=CARTESIAN_POINT('Ctrl Pts',(54.8584176801825,27.0102681970044,16.8442865524473));
#50139=CARTESIAN_POINT('Ctrl Pts',(54.8873077878004,27.0083160368007,16.8461178346457));
#50140=CARTESIAN_POINT('Ctrl Pts',(54.9091217760328,27.0072015192836,16.8474804575923));
#50141=CARTESIAN_POINT('Ctrl Pts',(54.9667850861947,27.0052042773022,16.8510396497858));
#50142=CARTESIAN_POINT('Ctrl Pts',(55.0026485633602,27.0049294518526,16.853209704663));
#50143=CARTESIAN_POINT('Ctrl Pts',(55.2159691986194,27.0090476576258,16.8659591569947));
#50144=CARTESIAN_POINT('Ctrl Pts',(55.3921880979826,27.036144128805,16.8759121178361));
#50145=CARTESIAN_POINT('Ctrl Pts',(55.6173965315011,27.1023376317224,16.8899769536234));
#50146=CARTESIAN_POINT('Ctrl Pts',(55.6715641306788,27.1208242106551,16.8934616717058));
#50147=CARTESIAN_POINT('Ctrl Pts',(55.7387211851653,27.1470186274005,16.8979490914754));
#50148=CARTESIAN_POINT('Ctrl Pts',(55.7525221132542,27.1525803381787,16.8988803109771));
#50149=CARTESIAN_POINT('Ctrl Pts',(55.7743893686359,27.1616784260374,16.9003708475851));
#50150=CARTESIAN_POINT('Ctrl Pts',(55.7824968994221,27.1651147987,16.9009268044888));
#50151=CARTESIAN_POINT('Ctrl Pts',(55.7976354968249,27.171649866317,16.9019712644512));
#50152=CARTESIAN_POINT('Ctrl Pts',(55.8046719505285,27.1747357324274,16.902459325961));
#50153=CARTESIAN_POINT('Ctrl Pts',(55.8203708224177,27.1817289587022,16.9035541313588));
#50154=CARTESIAN_POINT('Ctrl Pts',(55.8290234549913,27.1856577026814,16.9041615945916));
#50155=CARTESIAN_POINT('Ctrl Pts',(55.8544989369083,27.197445176146,16.905962293666));
#50156=CARTESIAN_POINT('Ctrl Pts',(55.871240131674,27.20547696568,16.9071614234284));
#50157=CARTESIAN_POINT('Ctrl Pts',(56.0025668246039,27.2707533622711,16.9166963644473));
#50158=CARTESIAN_POINT('Ctrl Pts',(56.1114885289116,27.3386702315731,16.9254125530072));
#50159=CARTESIAN_POINT('Ctrl Pts',(56.3290853987426,27.5053776099329,16.9444453797473));
#50160=CARTESIAN_POINT('Ctrl Pts',(56.434935636503,27.6066840579594,16.9547608188785));
#50161=CARTESIAN_POINT('Ctrl Pts',(56.5379106090545,27.729543130681,16.9653535960946));
#50162=CARTESIAN_POINT('Ctrl Pts',(56.5469269254191,27.7405370934029,16.9662861729264));
#50163=CARTESIAN_POINT('Ctrl Pts',(56.5593236484277,27.7559869089346,16.9675744729361));
#50164=CARTESIAN_POINT('Ctrl Pts',(56.5628037806768,27.7603616833135,16.9679368207702));
#50165=CARTESIAN_POINT('Ctrl Pts',(56.568774647179,27.7679325965983,16.9685596016942));
#50166=CARTESIAN_POINT('Ctrl Pts',(56.5712740958414,27.7711217730762,16.9688206393008));
#50167=CARTESIAN_POINT('Ctrl Pts',(56.5765027963279,27.7778353771084,16.9693673855857));
#50168=CARTESIAN_POINT('Ctrl Pts',(56.5792299773671,27.7813613696304,16.9696529414121));
#50169=CARTESIAN_POINT('Ctrl Pts',(56.5858884975803,27.7900301085702,16.9703511633553));
#50170=CARTESIAN_POINT('Ctrl Pts',(56.5898067105022,27.7951829637067,16.9707629196622));
#50171=CARTESIAN_POINT('Ctrl Pts',(56.6039573566964,27.8139817586543,16.9722535952883));
#50172=CARTESIAN_POINT('Ctrl Pts',(56.6140400860481,27.8277401665352,16.973322693676));
#50173=CARTESIAN_POINT('Ctrl Pts',(56.6387976632642,27.8624482846744,16.9759701419054));
#50174=CARTESIAN_POINT('Ctrl Pts',(56.6532487273545,27.8835545442302,16.9775359238579));
#50175=CARTESIAN_POINT('Ctrl Pts',(56.7140531491889,27.9761321829212,16.9842421093809));
#50176=CARTESIAN_POINT('Ctrl Pts',(56.7562109410883,28.0502585149894,16.9892053458231));
#50177=CARTESIAN_POINT('Ctrl Pts',(56.8596637001564,28.2627587233095,17.0029379060831));
#50178=CARTESIAN_POINT('Ctrl Pts',(56.9101571472269,28.4057211532166,17.011671141));
#50179=CARTESIAN_POINT('Ctrl Pts',(56.9493510762836,28.5761800975825,17.0224449343882));
#50180=CARTESIAN_POINT('Ctrl Pts',(56.9542642902374,28.5994454620733,17.0239216831063));
#50181=CARTESIAN_POINT('Ctrl Pts',(56.960594471874,28.6323167694341,17.026019305295));
#50182=CARTESIAN_POINT('Ctrl Pts',(56.9623591145657,28.6418543014683,17.0266292333191));
#50183=CARTESIAN_POINT('Ctrl Pts',(56.9653124779692,28.6584941042941,17.0276957920694));
#50184=CARTESIAN_POINT('Ctrl Pts',(56.9665324386422,28.6655907022316,17.0281514316468));
#50185=CARTESIAN_POINT('Ctrl Pts',(56.9690059772508,28.6804612257381,17.0291078807471));
#50186=CARTESIAN_POINT('Ctrl Pts',(56.9702519985466,28.6882362656963,17.0296089192385));
#50187=CARTESIAN_POINT('Ctrl Pts',(56.9731104881044,28.7067748041533,17.03080595699));
#50188=CARTESIAN_POINT('Ctrl Pts',(56.9746809510815,28.7175444327702,17.0315032611491));
#50189=CARTESIAN_POINT('Ctrl Pts',(56.9797157501852,28.7541677090476,17.0338812872322));
#50190=CARTESIAN_POINT('Ctrl Pts',(56.9827609556198,28.7800753459827,17.0355750013085));
#50191=CARTESIAN_POINT('Ctrl Pts',(56.9888517118132,28.8424160542129,17.0396798796929));
#50192=CARTESIAN_POINT('Ctrl Pts',(56.991405309247,28.8788866331893,17.0421053732857));
#50193=CARTESIAN_POINT('Ctrl Pts',(57.0019582336632,29.1275005846225,17.0588033690762));
#50194=CARTESIAN_POINT('Ctrl Pts',(56.9770490507329,29.3396262579937,17.0740579853184));
#50195=CARTESIAN_POINT('Ctrl Pts',(56.9123455908051,29.5679720353296,17.0899547757384));
#50196=CARTESIAN_POINT('Ctrl Pts',(56.9050451818364,29.5919973700519,17.09161794996));
#50197=CARTESIAN_POINT('Ctrl Pts',(56.8948921114606,29.6232751424958,17.0937651781727));
#50198=CARTESIAN_POINT('Ctrl Pts',(56.8924482274647,29.6306565852133,17.094270588738));
#50199=CARTESIAN_POINT('Ctrl Pts',(56.8884452571021,29.6425142305224,17.0950801340207));
#50200=CARTESIAN_POINT('Ctrl Pts',(56.8869132979433,29.6469994070125,17.0953858018368));
#50201=CARTESIAN_POINT('Ctrl Pts',(56.8839341483183,29.6556209961786,17.0959722624333));
#50202=CARTESIAN_POINT('Ctrl Pts',(56.8824893043134,29.6597581263541,17.0962531807272));
#50203=CARTESIAN_POINT('Ctrl Pts',(56.8790117196527,29.6696113234977,17.0969211022267));
#50204=CARTESIAN_POINT('Ctrl Pts',(56.8769664933563,29.6753229984733,17.0973073767489));
#50205=CARTESIAN_POINT('Ctrl Pts',(56.8699485518084,29.694643725852,17.0986112321948));
#50206=CARTESIAN_POINT('Ctrl Pts',(56.8648534961166,29.7082082736441,17.0995219376815));
#50207=CARTESIAN_POINT('Ctrl Pts',(56.8346262951967,29.7860931888906,17.1047304345441));
#50208=CARTESIAN_POINT('Ctrl Pts',(56.8063128411885,29.8491360751404,17.1088656295736));
#50209=CARTESIAN_POINT('Ctrl Pts',(56.7364732628164,29.9852568689812,17.1178768485602));
#50210=CARTESIAN_POINT('Ctrl Pts',(56.6934886235885,30.0574344048988,17.1227136889816));
#50211=CARTESIAN_POINT('Ctrl Pts',(56.5767644940927,30.2279671591395,17.1347455847663));
#50212=CARTESIAN_POINT('Ctrl Pts',(56.4982561847613,30.3226156610323,17.1419845196874));
#50213=CARTESIAN_POINT('Ctrl Pts',(56.4003615471259,30.420656935306,17.1505816892507));
#50214=CARTESIAN_POINT('Ctrl Pts',(56.3890337108705,30.4317345836828,17.1515703891042));
#50215=CARTESIAN_POINT('Ctrl Pts',(56.3704299436187,30.4494988590162,17.1531850703969));
#50216=CARTESIAN_POINT('Ctrl Pts',(56.3632340364831,30.4562685634234,17.1538074781997));
#50217=CARTESIAN_POINT('Ctrl Pts',(56.3503265620258,30.4682320424015,17.1549202767601));
#50218=CARTESIAN_POINT('Ctrl Pts',(56.344634537416,30.4734466778667,17.1554097704689));
#50219=CARTESIAN_POINT('Ctrl Pts',(56.3325620530644,30.4843784326484,17.1564454527626));
#50220=CARTESIAN_POINT('Ctrl Pts',(56.3261747582456,30.4900877368197,17.1569919538823));
#50221=CARTESIAN_POINT('Ctrl Pts',(56.3091178883716,30.5051375349052,17.1584476342307));
#50222=CARTESIAN_POINT('Ctrl Pts',(56.298385306972,30.5144055672629,17.1593597719696));
#50223=CARTESIAN_POINT('Ctrl Pts',(56.2462767921634,30.558442337052,17.1637710365687));
#50224=CARTESIAN_POINT('Ctrl Pts',(56.2036015295455,30.5916314897093,17.1673328003718));
#50225=CARTESIAN_POINT('Ctrl Pts',(56.0743789040041,30.6839586024112,17.177980366284));
#50226=CARTESIAN_POINT('Ctrl Pts',(55.9844651183941,30.7380536603584,17.1852276320582));
#50227=CARTESIAN_POINT('Ctrl Pts',(55.7827564792034,30.8387174118643,17.2009338169644));
#50228=CARTESIAN_POINT('Ctrl Pts',(55.6701064714993,30.8826980467667,17.2093796052857));
#50229=CARTESIAN_POINT('Ctrl Pts',(55.5389408728829,30.9206304706546,17.2184226765959));
#50230=CARTESIAN_POINT('Ctrl Pts',(55.523665809749,30.9248513777666,17.2194638168261));
#50231=CARTESIAN_POINT('Ctrl Pts',(55.5020841950951,30.9305390171978,17.220916444607));
#50232=CARTESIAN_POINT('Ctrl Pts',(55.4958187876428,30.9321576458734,17.2213359928051));
#50233=CARTESIAN_POINT('Ctrl Pts',(55.4852677142603,30.9348287470336,17.2220387514561));
#50234=CARTESIAN_POINT('Ctrl Pts',(55.4809862693466,30.9358975295233,17.2223228779195));
#50235=CARTESIAN_POINT('Ctrl Pts',(55.4722415763028,30.9380496767025,17.2229010247945));
#50236=CARTESIAN_POINT('Ctrl Pts',(55.4677780796463,30.9391318482742,17.2231949767329));
#50237=CARTESIAN_POINT('Ctrl Pts',(55.4563937166237,30.941850383721,17.2239418854143));
#50238=CARTESIAN_POINT('Ctrl Pts',(55.4494676940967,30.9434651869639,17.2243936298259));
#50239=CARTESIAN_POINT('Ctrl Pts',(55.4212714050009,30.9498803615555,17.2262224577608));
#50240=CARTESIAN_POINT('Ctrl Pts',(55.3999308277264,30.954369065977,17.2275829472569));
#50241=CARTESIAN_POINT('Ctrl Pts',(55.3433942240956,30.9652958736434,17.2311352048808));
#50242=CARTESIAN_POINT('Ctrl Pts',(55.3080901475351,30.9711388141247,17.2333005866451));
#50243=CARTESIAN_POINT('Ctrl Pts',(55.0980752267453,31.0001159847246,17.245970158376));
#50244=CARTESIAN_POINT('Ctrl Pts',(54.9210794676328,31.0009651764872,17.2558551631142));
#50245=CARTESIAN_POINT('Ctrl Pts',(54.6883084873651,30.9711139540399,17.2699051524524));
#50246=CARTESIAN_POINT('Ctrl Pts',(54.6307107926752,30.9611390398661,17.2734618740002));
#50247=CARTESIAN_POINT('Ctrl Pts',(54.5590096546041,30.9454509240181,17.2780304184129));
#50248=CARTESIAN_POINT('Ctrl Pts',(54.5444185502863,30.9420858132495,17.2789674725467));
#50249=CARTESIAN_POINT('Ctrl Pts',(54.5212882255149,30.9364763163197,17.2804652431872));
#50250=CARTESIAN_POINT('Ctrl Pts',(54.5127234497355,30.9343389171067,17.2810225427306));
#50251=CARTESIAN_POINT('Ctrl Pts',(54.4967329731218,30.9302354430042,17.2820682033866));
#50252=CARTESIAN_POINT('Ctrl Pts',(54.4893038707121,30.9282831811266,17.2825561132701));
#50253=CARTESIAN_POINT('Ctrl Pts',(54.4727381446291,30.923827497939,17.2836488589577));
#50254=CARTESIAN_POINT('Ctrl Pts',(54.4636077529387,30.9213018133975,17.2842544018042));
#50255=CARTESIAN_POINT('Ctrl Pts',(54.4367751356201,30.9136730964898,17.2860437961668));
#50256=CARTESIAN_POINT('Ctrl Pts',(54.4191256025028,30.9083898618668,17.2872334306284));
#50257=CARTESIAN_POINT('Ctrl Pts',(54.3792166735737,30.8958385601036,17.2899529923729));
#50258=CARTESIAN_POINT('Ctrl Pts',(54.3570073171438,30.8884215944177,17.2914875716143));
#50259=CARTESIAN_POINT('Ctrl Pts',(54.2838986651823,30.8625672691579,17.2966105974432));
#50260=CARTESIAN_POINT('Ctrl Pts',(54.2336227992142,30.8424502972793,17.300250544259));
#50261=CARTESIAN_POINT('Ctrl Pts',(54.0305841217449,30.7514590585834,17.3154208767061));
#50262=CARTESIAN_POINT('Ctrl Pts',(53.8862893248748,30.6634355972053,17.3273994342522));
#50263=CARTESIAN_POINT('Ctrl Pts',(53.7257187867043,30.535127955614,17.3413232523151));
#50264=CARTESIAN_POINT('Ctrl Pts',(53.6973199133797,30.5111040529081,17.3438084178473));
#50265=CARTESIAN_POINT('Ctrl Pts',(53.6630297473393,30.4804107658478,17.3468207886061));
#50266=CARTESIAN_POINT('Ctrl Pts',(53.6564911355618,30.4744793759891,17.3473957404883));
#50267=CARTESIAN_POINT('Ctrl Pts',(53.6462928511885,30.4651040118555,17.3482930432789));
#50268=CARTESIAN_POINT('Ctrl Pts',(53.6426065425826,30.4616893696684,17.3486174996186));
#50269=CARTESIAN_POINT('Ctrl Pts',(53.6357814944816,30.4553192149326,17.349218363294));
#50270=CARTESIAN_POINT('Ctrl Pts',(53.6326394562746,30.4523674783387,17.3494950324541));
#50271=CARTESIAN_POINT('Ctrl Pts',(53.6264534166954,30.4465182356605,17.3500398643856));
#50272=CARTESIAN_POINT('Ctrl Pts',(53.6234090136276,30.443621307553,17.3503080637695));
#50273=CARTESIAN_POINT('Ctrl Pts',(53.6142464033956,30.4348472059722,17.3511155340885));
#50274=CARTESIAN_POINT('Ctrl Pts',(53.6081564176096,30.4289405107245,17.3516526061822));
#50275=CARTESIAN_POINT('Ctrl Pts',(53.5718989645209,30.3933225769464,17.3548538075152));
#50276=CARTESIAN_POINT('Ctrl Pts',(53.5426436525828,30.3626934488702,17.3574522319262));
#50277=CARTESIAN_POINT('Ctrl Pts',(53.4497529135049,30.259023961256,17.3658480041075));
#50278=CARTESIAN_POINT('Ctrl Pts',(53.390456506765,30.1822774291885,17.3714513667412));
#50279=CARTESIAN_POINT('Ctrl Pts',(53.2628713442118,29.9896545022768,17.3848682233645));
#50280=CARTESIAN_POINT('Ctrl Pts',(53.2002604625237,29.8706112451632,17.3926855861683));
#50281=CARTESIAN_POINT('Ctrl Pts',(53.1460897707639,29.7363137123425,17.401600684779));
#50282=CARTESIAN_POINT('Ctrl Pts',(53.1421844534187,29.7264037509495,17.4022588758078));
#50283=CARTESIAN_POINT('Ctrl Pts',(53.1325798627255,29.7014474042068,17.4039176519475));
#50284=CARTESIAN_POINT('Ctrl Pts',(53.1269829963,29.6863626667633,17.4049214253623));
#50285=CARTESIAN_POINT('Ctrl Pts',(53.1182202001915,29.6618394167378,17.4065558724073));
#50286=CARTESIAN_POINT('Ctrl Pts',(53.1149413045205,29.6524418268117,17.407182824668));
#50287=CARTESIAN_POINT('Ctrl Pts',(53.1092416056515,29.6357043226245,17.4083007139324));
#50288=CARTESIAN_POINT('Ctrl Pts',(53.106792854804,29.6283740878282,17.4087907231174));
#50289=CARTESIAN_POINT('Ctrl Pts',(53.1017318540653,29.6129260393603,17.4098243698434));
#50290=CARTESIAN_POINT('Ctrl Pts',(53.099128945284,29.6048053515303,17.4103683010345));
#50291=CARTESIAN_POINT('Ctrl Pts',(53.0923901178946,29.5833079294571,17.4118098377418));
#50292=CARTESIAN_POINT('Ctrl Pts',(53.0883428903512,29.5699040985341,17.4127103004647));
#50293=CARTESIAN_POINT('Ctrl Pts',(53.0798065221263,29.5405183789881,17.4146883867922));
#50294=CARTESIAN_POINT('Ctrl Pts',(53.0753751359511,29.5245209393451,17.415767794003));
#50295=CARTESIAN_POINT('Ctrl Pts',(53.0620579705738,29.4740029708086,17.419185008074));
#50296=CARTESIAN_POINT('Ctrl Pts',(53.0539040381943,29.439323265497,17.4215435341112));
#50297=CARTESIAN_POINT('Ctrl Pts',(53.0466869493682,29.4044696388254,17.4239266846335));
#50298=CARTESIAN_POINT('Origin',(55.,29.,3.45145488139523));
#50299=CARTESIAN_POINT('',(53.0466869980087,29.4044698737256,18.3839095910714));
#50300=CARTESIAN_POINT('',(53.0466869962288,29.4044698651299,18.2270410618393));
#50301=CARTESIAN_POINT('',(53.0466869980082,29.4044698737233,3.45145488139523));
#50302=CARTESIAN_POINT('Ctrl Pts',(53.0466869980087,29.4044698737256,18.3839095910714));
#50303=CARTESIAN_POINT('Ctrl Pts',(53.0663282740129,29.4993238104147,18.3771815173166));
#50304=CARTESIAN_POINT('Ctrl Pts',(53.0928528261563,29.5926220832049,18.3703852673977));
#50305=CARTESIAN_POINT('Ctrl Pts',(53.1449829312298,29.7355207600424,18.3599570166841));
#50306=CARTESIAN_POINT('Ctrl Pts',(53.1660641757064,29.7866128105735,18.356226466279));
#50307=CARTESIAN_POINT('Ctrl Pts',(53.1932258003383,29.8453903051281,18.3519834221063));
#50308=CARTESIAN_POINT('Ctrl Pts',(53.1972717429001,29.853983967166,18.3513643263843));
#50309=CARTESIAN_POINT('Ctrl Pts',(53.203591523263,29.8671622270098,18.350417273382));
#50310=CARTESIAN_POINT('Ctrl Pts',(53.2058218110092,29.8717673834286,18.3500867641168));
#50311=CARTESIAN_POINT('Ctrl Pts',(53.2099601354037,29.8802291511687,18.3494803481231));
#50312=CARTESIAN_POINT('Ctrl Pts',(53.2118629226712,29.884088156661,18.3492041369051));
#50313=CARTESIAN_POINT('Ctrl Pts',(53.216186318876,29.8927852925755,18.3485823939949));
#50314=CARTESIAN_POINT('Ctrl Pts',(53.218614127881,29.8976197434721,18.3482373127953));
#50315=CARTESIAN_POINT('Ctrl Pts',(53.2258420108211,29.9118676677859,18.3472216798123));
#50316=CARTESIAN_POINT('Ctrl Pts',(53.2306973362416,29.9212531191818,18.3465544418942));
#50317=CARTESIAN_POINT('Ctrl Pts',(53.2739837314391,30.0033220625778,18.3407317648595));
#50318=CARTESIAN_POINT('Ctrl Pts',(53.3168048136082,30.0736129052864,18.3358252444211));
#50319=CARTESIAN_POINT('Ctrl Pts',(53.4522314216923,30.2677982394056,18.3219299186714));
#50320=CARTESIAN_POINT('Ctrl Pts',(53.5550348327484,30.3838263831878,18.3131513860552));
#50321=CARTESIAN_POINT('Ctrl Pts',(53.7084272785613,30.5210186831608,18.3007611623597));
#50322=CARTESIAN_POINT('Ctrl Pts',(53.7479567672762,30.553719728598,18.2976253393918));
#50323=CARTESIAN_POINT('Ctrl Pts',(53.7968390382002,30.591080200683,18.2937894523554));
#50324=CARTESIAN_POINT('Ctrl Pts',(53.8050258461031,30.5972380130678,18.2931483975018));
#50325=CARTESIAN_POINT('Ctrl Pts',(53.8205970758861,30.608763388188,18.2919314856081));
#50326=CARTESIAN_POINT('Ctrl Pts',(53.8279716426294,30.6141438664713,18.2913561426259));
#50327=CARTESIAN_POINT('Ctrl Pts',(53.8355043801587,30.6195609084879,18.2907693836756));
#50328=CARTESIAN_POINT('Ctrl Pts',(53.8356259854771,30.6196483381388,18.2907599115318));
#50329=CARTESIAN_POINT('Ctrl Pts',(53.8358714539326,30.6198247787943,18.2907407918683));
#50330=CARTESIAN_POINT('Ctrl Pts',(53.8359953173427,30.6199137892236,18.2907311443365));
#50331=CARTESIAN_POINT('Ctrl Pts',(53.8362455233502,30.6200935481556,18.2907116566818));
#50332=CARTESIAN_POINT('Ctrl Pts',(53.836371866466,30.6201842961669,18.2907018165287));
#50333=CARTESIAN_POINT('Ctrl Pts',(53.8366272725509,30.6203677004834,18.2906819249176));
#50334=CARTESIAN_POINT('Ctrl Pts',(53.8367563359285,30.6204603561149,18.2906718734391));
#50335=CARTESIAN_POINT('Ctrl Pts',(53.8370174443922,30.620647760701,18.2906515388179));
#50336=CARTESIAN_POINT('Ctrl Pts',(53.8371494899267,30.6207425088938,18.2906412556528));
#50337=CARTESIAN_POINT('Ctrl Pts',(53.842977443031,30.624923230096,18.2901874111216));
#50338=CARTESIAN_POINT('Ctrl Pts',(53.8486947778472,30.6289791233919,18.2897427105465));
#50339=CARTESIAN_POINT('Ctrl Pts',(53.8615194070074,30.6379757095229,18.2887463094328));
#50340=CARTESIAN_POINT('Ctrl Pts',(53.8686376875887,30.6429004229695,18.2881940154142));
#50341=CARTESIAN_POINT('Ctrl Pts',(53.8873387805978,30.6556594179283,18.2867448721204));
#50342=CARTESIAN_POINT('Ctrl Pts',(53.8989721552239,30.6634183977424,18.2858452293157));
#50343=CARTESIAN_POINT('Ctrl Pts',(53.9515517668399,30.6976935934691,18.2817864778678));
#50344=CARTESIAN_POINT('Ctrl Pts',(53.9933778498125,30.7228228005966,18.2785771149641));
#50345=CARTESIAN_POINT('Ctrl Pts',(54.1823294197327,30.8271144889793,18.2641524755469));
#50346=CARTESIAN_POINT('Ctrl Pts',(54.3381275678869,30.8891378566349,18.2523757746302));
#50347=CARTESIAN_POINT('Ctrl Pts',(54.5477227223439,30.9434310501543,18.2374091253044));
#50348=CARTESIAN_POINT('Ctrl Pts',(54.5961015743428,30.9540587759604,18.2340182522851));
#50349=CARTESIAN_POINT('Ctrl Pts',(54.6627994641184,30.966127381721,18.2294700722904));
#50350=CARTESIAN_POINT('Ctrl Pts',(54.6808146832369,30.9691322624609,18.2282541488075));
#50351=CARTESIAN_POINT('Ctrl Pts',(54.7119196652734,30.9738823589965,18.2261791212927));
#50352=CARTESIAN_POINT('Ctrl Pts',(54.7249899163165,30.9757457636343,18.2253145780033));
#50353=CARTESIAN_POINT('Ctrl Pts',(54.7438707322264,30.9782465730511,18.2240772391273));
#50354=CARTESIAN_POINT('Ctrl Pts',(54.7496667828406,30.9789883749192,18.2236989659522));
#50355=CARTESIAN_POINT('Ctrl Pts',(54.7597805253145,30.980237628361,18.223041731113));
#50356=CARTESIAN_POINT('Ctrl Pts',(54.7640967337669,30.9807564492455,18.2227621448487));
#50357=CARTESIAN_POINT('Ctrl Pts',(54.7732215723239,30.9818230316452,18.2221730061112));
#50358=CARTESIAN_POINT('Ctrl Pts',(54.7780305150069,30.982367406146,18.2218636424506));
#50359=CARTESIAN_POINT('Ctrl Pts',(54.7910184728013,30.983789794659,18.2210310289626));
#50360=CARTESIAN_POINT('Ctrl Pts',(54.799201122105,30.9846347382581,18.2205095839159));
#50361=CARTESIAN_POINT('Ctrl Pts',(54.8364755475044,30.9882508165458,18.2181474714516));
#50362=CARTESIAN_POINT('Ctrl Pts',(54.8656224576978,30.9904332295135,18.2163370387361));
#50363=CARTESIAN_POINT('Ctrl Pts',(55.1021246800094,31.0029223530592,18.2018675931434));
#50364=CARTESIAN_POINT('Ctrl Pts',(55.3098961404352,30.9814424099518,18.1904007120756));
#50365=CARTESIAN_POINT('Ctrl Pts',(55.5638283585736,30.9141977573769,18.1746268899483));
#50366=CARTESIAN_POINT('Ctrl Pts',(55.6164115195397,30.897917671219,18.1712689328064));
#50367=CARTESIAN_POINT('Ctrl Pts',(55.6816887888239,30.8747083375326,18.1669514150592));
#50368=CARTESIAN_POINT('Ctrl Pts',(55.6950743901197,30.8697867608963,18.1660580763259));
#50369=CARTESIAN_POINT('Ctrl Pts',(55.7164311082431,30.8616733683527,18.1646193850239));
#50370=CARTESIAN_POINT('Ctrl Pts',(55.7244365482176,30.8585728253661,18.1640770643958));
#50371=CARTESIAN_POINT('Ctrl Pts',(55.7395985550381,30.852587669857,18.1630440380833));
#50372=CARTESIAN_POINT('Ctrl Pts',(55.7467589034668,30.8497130140884,18.1625536725862));
#50373=CARTESIAN_POINT('Ctrl Pts',(55.7630195683498,30.843075060168,18.1614342662883));
#50374=CARTESIAN_POINT('Ctrl Pts',(55.7721090007092,30.8392857919333,18.1608043624977));
#50375=CARTESIAN_POINT('Ctrl Pts',(55.7956498067761,30.8292666824433,18.1591619121793));
#50376=CARTESIAN_POINT('Ctrl Pts',(55.8100559535118,30.8229329497533,18.1581458834684));
#50377=CARTESIAN_POINT('Ctrl Pts',(55.9440632616849,30.7621138246413,18.1485901995602));
#50378=CARTESIAN_POINT('Ctrl Pts',(56.0580579763213,30.6961138418899,18.139645289434));
#50379=CARTESIAN_POINT('Ctrl Pts',(56.2425369075894,30.5634314574486,18.123862179558));
#50380=CARTESIAN_POINT('Ctrl Pts',(56.3162207716959,30.5019252089318,18.1171375627799));
#50381=CARTESIAN_POINT('Ctrl Pts',(56.4256787563422,30.3962924303059,18.1067029141482));
#50382=CARTESIAN_POINT('Ctrl Pts',(56.4644933032787,30.355526870813,18.1029014780861));
#50383=CARTESIAN_POINT('Ctrl Pts',(56.5078154723697,30.3059904508371,18.0985887702237));
#50384=CARTESIAN_POINT('Ctrl Pts',(56.51404373589,30.2987648481809,18.0979669675616));
#50385=CARTESIAN_POINT('Ctrl Pts',(56.5235385212463,30.2875885239057,18.0970166604509));
#50386=CARTESIAN_POINT('Ctrl Pts',(56.5268419478216,30.2836695448633,18.0966855771727));
#50387=CARTESIAN_POINT('Ctrl Pts',(56.5328903130045,30.27643776151,18.0960786185718));
#50388=CARTESIAN_POINT('Ctrl Pts',(56.5356396308803,30.273128821231,18.0958024347583));
#50389=CARTESIAN_POINT('Ctrl Pts',(56.5418152450407,30.2656470530566,18.095181390067));
#50390=CARTESIAN_POINT('Ctrl Pts',(56.5452353123318,30.2614692005419,18.094836975083));
#50391=CARTESIAN_POINT('Ctrl Pts',(56.5552671223081,30.2491126229863,18.0938251358267));
#50392=CARTESIAN_POINT('Ctrl Pts',(56.5618313171359,30.2408952875882,18.0931609886581));
#50393=CARTESIAN_POINT('Ctrl Pts',(56.6168362436764,30.1709098397934,18.0875744094962));
#50394=CARTESIAN_POINT('Ctrl Pts',(56.6616630319082,30.106376186782,18.0828786364954));
#50395=CARTESIAN_POINT('Ctrl Pts',(56.7691977368114,29.930223931931,18.0707445326249));
#50396=CARTESIAN_POINT('Ctrl Pts',(56.8251736495254,29.8149350803117,18.0634500423054));
#50397=CARTESIAN_POINT('Ctrl Pts',(56.8877653171004,29.6465666997486,18.0528156418698));
#50398=CARTESIAN_POINT('Ctrl Pts',(56.9039043478081,29.5973726190831,18.0497134993359));
#50399=CARTESIAN_POINT('Ctrl Pts',(56.9243442566134,29.5257777117091,18.045168280225));
#50400=CARTESIAN_POINT('Ctrl Pts',(56.9302036231324,29.5038421694369,18.0437717783187));
#50401=CARTESIAN_POINT('Ctrl Pts',(56.9400295493195,29.4643663619956,18.0412486308567));
#50402=CARTESIAN_POINT('Ctrl Pts',(56.9441357918232,29.4468632458685,18.040126430872));
#50403=CARTESIAN_POINT('Ctrl Pts',(56.9500239701917,29.4201453316535,18.0384071533119));
#50404=CARTESIAN_POINT('Ctrl Pts',(56.951978455162,29.4109692078438,18.0378155589075));
#50405=CARTESIAN_POINT('Ctrl Pts',(56.9552650180717,29.3949865450273,18.0367830588096));
#50406=CARTESIAN_POINT('Ctrl Pts',(56.956626475505,29.388186160273,18.0363430927333));
#50407=CARTESIAN_POINT('Ctrl Pts',(56.9596037717126,29.3729010865599,18.0353526619981));
#50408=CARTESIAN_POINT('Ctrl Pts',(56.9612000139744,29.3644127657066,18.0348015869995));
#50409=CARTESIAN_POINT('Ctrl Pts',(56.9653280602459,29.3416480653089,18.0333207129244));
#50410=CARTESIAN_POINT('Ctrl Pts',(56.9677593816375,29.3273542157921,18.0323877713829));
#50411=CARTESIAN_POINT('Ctrl Pts',(56.9780576131325,29.2625440692861,18.0281428204872));
#50412=CARTESIAN_POINT('Ctrl Pts',(56.9841358885803,29.2117671008798,18.0247755197651));
#50413=CARTESIAN_POINT('Ctrl Pts',(57.0030975515834,28.9773340406004,18.0090290832544));
#50414=CARTESIAN_POINT('Ctrl Pts',(56.9924650169005,28.7926890268494,17.9959561601167));
#50415=CARTESIAN_POINT('Ctrl Pts',(56.9461977734431,28.5592605768878,17.9796539652705));
#50416=CARTESIAN_POINT('Ctrl Pts',(56.9335677674824,28.5067922991434,17.9760140646675));
#50417=CARTESIAN_POINT('Ctrl Pts',(56.9162441932175,28.4458114560922,17.9718603196061));
#50418=CARTESIAN_POINT('Ctrl Pts',(56.9135989145825,28.4367452150573,17.9712448041018));
#50419=CARTESIAN_POINT('Ctrl Pts',(56.9094245963475,28.422807366722,17.9703020567034));
#50420=CARTESIAN_POINT('Ctrl Pts',(56.9079411188841,28.4179224164041,17.9699723081431));
#50421=CARTESIAN_POINT('Ctrl Pts',(56.9051725899797,28.4089302202114,17.9693666072098));
#50422=CARTESIAN_POINT('Ctrl Pts',(56.9038930070097,28.404821454783,17.9690903556613));
#50423=CARTESIAN_POINT('Ctrl Pts',(56.9009705559212,28.3955432785602,17.9684676693866));
#50424=CARTESIAN_POINT('Ctrl Pts',(56.8993198965764,28.3903764155592,17.968121691337));
#50425=CARTESIAN_POINT('Ctrl Pts',(56.8943708786245,28.3751003201572,17.9671009407073));
#50426=CARTESIAN_POINT('Ctrl Pts',(56.891012676707,28.36501046949,17.9664295319024));
#50427=CARTESIAN_POINT('Ctrl Pts',(56.8557710997816,28.2618853752652,17.959591379748));
#50428=CARTESIAN_POINT('Ctrl Pts',(56.8171248640251,28.1712888741321,17.9537823998474));
#50429=CARTESIAN_POINT('Ctrl Pts',(56.7131989377843,27.9702717075897,17.9405785148102));
#50430=CARTESIAN_POINT('Ctrl Pts',(56.6436605211539,27.8625599789595,17.9332479119037));
#50431=CARTESIAN_POINT('Ctrl Pts',(56.5269289198295,27.715032772372,17.9219907115163));
#50432=CARTESIAN_POINT('Ctrl Pts',(56.4874534903524,27.6695362610519,17.9183261496486));
#50433=CARTESIAN_POINT('Ctrl Pts',(56.4358830446294,27.6152680936827,17.9136632802926));
#50434=CARTESIAN_POINT('Ctrl Pts',(56.4256655237052,27.6047507868735,17.9127451694339));
#50435=CARTESIAN_POINT('Ctrl Pts',(56.4092214157461,27.5881934311821,17.9112760237213));
#50436=CARTESIAN_POINT('Ctrl Pts',(56.4030696495878,27.5820795717187,17.9107282554543));
#50437=CARTESIAN_POINT('Ctrl Pts',(56.3913814106349,27.5706138995664,17.9096908430322));
#50438=CARTESIAN_POINT('Ctrl Pts',(56.3858534243918,27.5652536330882,17.9092015803126));
#50439=CARTESIAN_POINT('Ctrl Pts',(56.3732925193085,27.5532141515733,17.9080928827734));
#50440=CARTESIAN_POINT('Ctrl Pts',(56.3662416824886,27.5465539933079,17.9074726468792));
#50441=CARTESIAN_POINT('Ctrl Pts',(56.3479843856686,27.529558550433,17.9058718433426));
#50442=CARTESIAN_POINT('Ctrl Pts',(56.3367076744035,27.5192999856403,17.904888078671));
#50443=CARTESIAN_POINT('Ctrl Pts',(56.2586290539391,27.449889738141,17.8981090283514));
#50444=CARTESIAN_POINT('Ctrl Pts',(56.1880504229011,27.3951569569671,17.8921346619723));
#50445=CARTESIAN_POINT('Ctrl Pts',(55.993042080647,27.2638613975576,17.8760376483664));
#50446=CARTESIAN_POINT('Ctrl Pts',(55.8634668076913,27.1959126267061,17.8657127289931));
#50447=CARTESIAN_POINT('Ctrl Pts',(55.6812203591201,27.1245127056362,17.8523373866328));
#50448=CARTESIAN_POINT('Ctrl Pts',(55.6341241274545,27.1080694293651,17.8489807377694));
#50449=CARTESIAN_POINT('Ctrl Pts',(55.5776056576967,27.0906846708512,17.8451076288189));
#50450=CARTESIAN_POINT('Ctrl Pts',(55.5687352309557,27.0880236489581,17.8445042220343));
#50451=CARTESIAN_POINT('Ctrl Pts',(55.5549841471116,27.0840026560994,17.8435760507969));
#50452=CARTESIAN_POINT('Ctrl Pts',(55.550116439522,27.0825993820483,17.8432488875649));
#50453=CARTESIAN_POINT('Ctrl Pts',(55.5411006858606,27.0800374592453,17.8426455808977));
#50454=CARTESIAN_POINT('Ctrl Pts',(55.5369542575908,27.0788737063963,17.842369156446));
#50455=CARTESIAN_POINT('Ctrl Pts',(55.5275282421993,27.0762610655953,17.8417431027127));
#50456=CARTESIAN_POINT('Ctrl Pts',(55.5222464449193,27.0748204793991,17.8413939519305));
#50457=CARTESIAN_POINT('Ctrl Pts',(55.5085100860416,27.0711346409395,17.8404900473232));
#50458=CARTESIAN_POINT('Ctrl Pts',(55.500046462024,27.0689231958935,17.8399371638316));
#50459=CARTESIAN_POINT('Ctrl Pts',(55.4438182761371,27.0546258996368,17.8362892556665));
#50460=CARTESIAN_POINT('Ctrl Pts',(55.3956302804157,27.0442565059558,17.8332830769496));
#50461=CARTESIAN_POINT('Ctrl Pts',(55.3330029806956,27.0331899908629,17.8294725779965));
#50462=CARTESIAN_POINT('Ctrl Pts',(55.3188757268696,27.0308502133203,17.8286192969761));
#50463=CARTESIAN_POINT('Ctrl Pts',(55.2641450783895,27.0223900899969,17.8253337585803));
#50464=CARTESIAN_POINT('Ctrl Pts',(55.223380569697,27.0173717162484,17.8229292921772));
#50465=CARTESIAN_POINT('Ctrl Pts',(55.0762660196611,27.0038563116771,17.8143198635165));
#50466=CARTESIAN_POINT('Ctrl Pts',(54.9694349096605,27.0026339342132,17.8081854199797));
#50467=CARTESIAN_POINT('Ctrl Pts',(54.813507427528,27.0133668790575,17.7989163739121));
#50468=CARTESIAN_POINT('Ctrl Pts',(54.7641426116709,27.0186213362915,17.7959369671255));
#50469=CARTESIAN_POINT('Ctrl Pts',(54.6931983924026,27.0288615539455,17.7915572649534));
#50470=CARTESIAN_POINT('Ctrl Pts',(54.671423722046,27.032374127849,17.7901996637063));
#50471=CARTESIAN_POINT('Ctrl Pts',(54.6324166209569,27.0393320822694,17.7877409009367));
#50472=CARTESIAN_POINT('Ctrl Pts',(54.6151628181644,27.0426455259808,17.7866438559577));
#50473=CARTESIAN_POINT('Ctrl Pts',(54.5888491503543,27.0480602014071,17.7849552869356));
#50474=CARTESIAN_POINT('Ctrl Pts',(54.5797561876686,27.0499976584629,17.7843689450596));
#50475=CARTESIAN_POINT('Ctrl Pts',(54.5639127651605,27.0534894126746,17.7833422152924));
#50476=CARTESIAN_POINT('Ctrl Pts',(54.5571561889739,27.0550154499253,17.7829027328036));
#50477=CARTESIAN_POINT('Ctrl Pts',(54.5419345314749,27.0585368334298,17.781908906117));
#50478=CARTESIAN_POINT('Ctrl Pts',(54.5334743185896,27.0605524020323,17.7813539246064));
#50479=CARTESIAN_POINT('Ctrl Pts',(54.5106806898762,27.066140547341,17.7798514926926));
#50480=CARTESIAN_POINT('Ctrl Pts',(54.4963735567035,27.06981706666,17.7789007387953));
#50481=CARTESIAN_POINT('Ctrl Pts',(54.4299525752821,27.0876740879398,17.774449977846));
#50482=CARTESIAN_POINT('Ctrl Pts',(54.3783918026737,27.1038072900062,17.7708878935433));
#50483=CARTESIAN_POINT('Ctrl Pts',(54.1571936289104,27.1830112142003,17.7551258569955));
#50484=CARTESIAN_POINT('Ctrl Pts',(53.9959348693765,27.2669082743935,17.742276924179));
#50485=CARTESIAN_POINT('Ctrl Pts',(53.8187888844234,27.3921851855131,17.7274157489341));
#50486=CARTESIAN_POINT('Ctrl Pts',(53.789912274838,27.413804493902,17.7249702690597));
#50487=CARTESIAN_POINT('Ctrl Pts',(53.744443646218,27.4498107388722,17.7211010926532));
#50488=CARTESIAN_POINT('Ctrl Pts',(53.7274759499059,27.4637086408299,17.719652887236));
#50489=CARTESIAN_POINT('Ctrl Pts',(53.7053019398326,27.4824904328981,17.7177583153406));
#50490=CARTESIAN_POINT('Ctrl Pts',(53.6998884102839,27.4871258442155,17.71729561654));
#50491=CARTESIAN_POINT('Ctrl Pts',(53.691024708216,27.4947982288816,17.7165379296553));
#50492=CARTESIAN_POINT('Ctrl Pts',(53.6875600375025,27.4978182426359,17.7162417375863));
#50493=CARTESIAN_POINT('Ctrl Pts',(53.6807911391025,27.503759713218,17.7156630739839));
#50494=CARTESIAN_POINT('Ctrl Pts',(53.6774861213605,27.5066801896993,17.7153805381141));
#50495=CARTESIAN_POINT('Ctrl Pts',(53.6693649423274,27.5139045710416,17.7146862191356));
#50496=CARTESIAN_POINT('Ctrl Pts',(53.6645598936171,27.5182209997099,17.7142753556603));
#50497=CARTESIAN_POINT('Ctrl Pts',(53.6480923970351,27.5331591011247,17.7128667310573));
#50498=CARTESIAN_POINT('Ctrl Pts',(53.6365346767694,27.5438960414061,17.7118771390249));
#50499=CARTESIAN_POINT('Ctrl Pts',(53.5367996368861,27.6387772250574,17.7033164147693));
#50500=CARTESIAN_POINT('Ctrl Pts',(53.4563667974212,27.7307138097244,17.696255679928));
#50501=CARTESIAN_POINT('Ctrl Pts',(53.3238248941312,27.9135978507516,17.6831400840354));
#50502=CARTESIAN_POINT('Ctrl Pts',(53.2695009990644,28.0024009818177,17.6771096479169));
#50503=CARTESIAN_POINT('Ctrl Pts',(53.1979406496193,28.1429680853764,17.6676298571703));
#50504=CARTESIAN_POINT('Ctrl Pts',(53.1754856925313,28.1918735416007,17.6643448911918));
#50505=CARTESIAN_POINT('Ctrl Pts',(53.1496525329729,28.2547199801584,17.6601097714238));
#50506=CARTESIAN_POINT('Ctrl Pts',(53.1444089602304,28.2678730072018,17.6592227268509));
#50507=CARTESIAN_POINT('Ctrl Pts',(53.1362199996939,28.2890675215343,17.657791772915));
#50508=CARTESIAN_POINT('Ctrl Pts',(53.1331855319149,28.297074245353,17.6572508370274));
#50509=CARTESIAN_POINT('Ctrl Pts',(53.1275131744374,28.3123371045532,17.6562188808308));
#50510=CARTESIAN_POINT('Ctrl Pts',(53.1248656726683,28.3195895199137,17.6557281900277));
#50511=CARTESIAN_POINT('Ctrl Pts',(53.1189235527814,28.3361651281563,17.6546058435977));
#50512=CARTESIAN_POINT('Ctrl Pts',(53.1156560433519,28.3454977581284,17.6539733080981));
#50513=CARTESIAN_POINT('Ctrl Pts',(53.1073248611403,28.3698727978348,17.6523194652743));
#50514=CARTESIAN_POINT('Ctrl Pts',(53.1023711758809,28.3849517953617,17.6512945957911));
#50515=CARTESIAN_POINT('Ctrl Pts',(53.0611082639427,28.5158020475714,17.6423840984435));
#50516=CARTESIAN_POINT('Ctrl Pts',(53.0352582612837,28.6345833017177,17.6341569402808));
#50517=CARTESIAN_POINT('Ctrl Pts',(53.0102373548337,28.8367212287986,17.6200434124739));
#50518=CARTESIAN_POINT('Ctrl Pts',(53.0051918952654,28.9190324141993,17.6142722512882));
#50519=CARTESIAN_POINT('Ctrl Pts',(53.0053057996264,29.0791465571617,17.6031814545234));
#50520=CARTESIAN_POINT('Ctrl Pts',(53.0099041912835,29.1568137953276,17.597864905554));
#50521=CARTESIAN_POINT('Ctrl Pts',(53.0202577197349,29.2444553877004,17.5920697090153));
#50522=CARTESIAN_POINT('Ctrl Pts',(53.0215726775749,29.2548789402342,17.5913838089206));
#50523=CARTESIAN_POINT('Ctrl Pts',(53.023687696584,29.2706406591957,17.5903521985442));
#50524=CARTESIAN_POINT('Ctrl Pts',(53.0244271467207,29.2759865759061,17.5900032759831));
#50525=CARTESIAN_POINT('Ctrl Pts',(53.0257950220923,29.2855884707871,17.5893783932969));
#50526=CARTESIAN_POINT('Ctrl Pts',(53.0264155245548,29.2898454567165,17.5891020030736));
#50527=CARTESIAN_POINT('Ctrl Pts',(53.0278057847463,29.2991719073525,17.5884979014875));
#50528=CARTESIAN_POINT('Ctrl Pts',(53.0285813170688,29.304240416175,17.5881705161606));
#50529=CARTESIAN_POINT('Ctrl Pts',(53.0308569600119,29.3187387979668,17.5872365168331));
#50530=CARTESIAN_POINT('Ctrl Pts',(53.0324052699432,29.3281611190893,17.5866325293694));
#50531=CARTESIAN_POINT('Ctrl Pts',(53.0378624988456,29.3599433479304,17.5846042947244));
#50532=CARTESIAN_POINT('Ctrl Pts',(53.0420850947042,29.3822458266942,17.5831962037013));
#50533=CARTESIAN_POINT('Ctrl Pts',(53.0466869985623,29.4044698763992,17.581803907097));
#50534=CARTESIAN_POINT('',(53.0052506561638,28.9983820491308,17.4520829507836));
#50535=CARTESIAN_POINT('Ctrl Pts',(53.0466869493682,29.4044696388254,17.4239266846335));
#50536=CARTESIAN_POINT('Ctrl Pts',(53.0190383160083,29.2709455589196,17.4330565230793));
#50537=CARTESIAN_POINT('Ctrl Pts',(53.0051399492086,29.1348711355884,17.4425822687156));
#50538=CARTESIAN_POINT('Ctrl Pts',(53.0052506561637,28.9983820492037,17.4520829507785));
#50539=CARTESIAN_POINT('Ctrl Pts',(53.0052506575382,28.9983803554686,17.4520830686754));
#50540=CARTESIAN_POINT('Ctrl Pts',(53.0053310699018,28.8993447299746,17.4589767034832));
#50541=CARTESIAN_POINT('Ctrl Pts',(53.012786828428,28.800437688623,17.4658212023425));
#50542=CARTESIAN_POINT('Ctrl Pts',(53.0287017229543,28.6949278439711,17.4728302018829));
#50543=CARTESIAN_POINT('Ctrl Pts',(53.0298844947448,28.6873807143479,17.4733298875341));
#50544=CARTESIAN_POINT('Ctrl Pts',(53.0319219811726,28.6748507582436,17.4741564985698));
#50545=CARTESIAN_POINT('Ctrl Pts',(53.0327523225448,28.6698641272487,17.4744846842174));
#50546=CARTESIAN_POINT('Ctrl Pts',(53.0342886996821,28.6608490421964,17.475076506032));
#50547=CARTESIAN_POINT('Ctrl Pts',(53.0349881813016,28.6568195205474,17.4753404968462));
#50548=CARTESIAN_POINT('Ctrl Pts',(53.0364490527759,28.6485547603198,17.4758808094941));
#50549=CARTESIAN_POINT('Ctrl Pts',(53.0372117462018,28.6443198765236,17.4761570409539));
#50550=CARTESIAN_POINT('Ctrl Pts',(53.0389655764266,28.6347591239462,17.4767792727686));
#50551=CARTESIAN_POINT('Ctrl Pts',(53.0399647065677,28.6294348125653,17.4771248194195));
#50552=CARTESIAN_POINT('Ctrl Pts',(53.0429832130151,28.6137031634454,17.4781431075827));
#50553=CARTESIAN_POINT('Ctrl Pts',(53.0450639162683,28.6033075869515,17.4788125093786));
#50554=CARTESIAN_POINT('Ctrl Pts',(53.0646406471603,28.5093955018075,17.4848322120176));
#50555=CARTESIAN_POINT('Ctrl Pts',(53.0873982127239,28.4270543455325,17.4899141819321));
#50556=CARTESIAN_POINT('Ctrl Pts',(53.139477273129,28.2768824443825,17.499230763486));
#50557=CARTESIAN_POINT('Ctrl Pts',(53.167420809382,28.2087366600188,17.5034786898085));
#50558=CARTESIAN_POINT('Ctrl Pts',(53.2339999848588,28.0689403702465,17.5124944829673));
#50559=CARTESIAN_POINT('Ctrl Pts',(53.2733797898052,27.9977978038413,17.5172631271533));
#50560=CARTESIAN_POINT('Ctrl Pts',(53.3428000653782,27.888681474978,17.5250670699337));
#50561=CARTESIAN_POINT('Ctrl Pts',(53.3700725708284,27.8490540857701,17.5280122363345));
#50562=CARTESIAN_POINT('Ctrl Pts',(53.4069314295075,27.799438308925,17.5318670402617));
#50563=CARTESIAN_POINT('Ctrl Pts',(53.4152274124654,27.7885084914231,17.5327270479576));
#50564=CARTESIAN_POINT('Ctrl Pts',(53.4288231608752,27.7709749483434,17.5341247754483));
#50565=CARTESIAN_POINT('Ctrl Pts',(53.4340534592386,27.7643177328621,17.5346597676375));
#50566=CARTESIAN_POINT('Ctrl Pts',(53.44414903138,27.7516349485523,17.5356873674046));
#50567=CARTESIAN_POINT('Ctrl Pts',(53.449007337628,27.7456040111901,17.5361796924097));
#50568=CARTESIAN_POINT('Ctrl Pts',(53.4601612331968,27.7319218046539,17.5373051281369));
#50569=CARTESIAN_POINT('Ctrl Pts',(53.4664789200553,27.7242888928893,17.5379391194459));
#50570=CARTESIAN_POINT('Ctrl Pts',(53.4833393142276,27.7042247082529,17.5396221845758));
#50571=CARTESIAN_POINT('Ctrl Pts',(53.4939778010449,27.6918752533793,17.5406751301765));
#50572=CARTESIAN_POINT('Ctrl Pts',(53.5115614693153,27.6719624636846,17.5424013538007));
#50573=CARTESIAN_POINT('Ctrl Pts',(53.5184159593737,27.664319768209,17.5430708809837));
#50574=CARTESIAN_POINT('Ctrl Pts',(53.6156408608556,27.5575841259913,17.5525207898834));
#50575=CARTESIAN_POINT('Ctrl Pts',(53.7157055005721,27.467815378602,17.5617198556858));
#50576=CARTESIAN_POINT('Ctrl Pts',(53.9244408597701,27.3154633923174,17.579711049901));
#50577=CARTESIAN_POINT('Ctrl Pts',(54.0315267343688,27.2516993155066,17.5884371149233));
#50578=CARTESIAN_POINT('Ctrl Pts',(54.1555274857664,27.1927754428589,17.5975646930363));
#50579=CARTESIAN_POINT('Ctrl Pts',(54.1672487399049,27.1873445486173,17.5984181835781));
#50580=CARTESIAN_POINT('Ctrl Pts',(54.1880835898724,27.1779357427103,17.5999178630465));
#50581=CARTESIAN_POINT('Ctrl Pts',(54.1971756134793,27.1739114400203,17.6005664947165));
#50582=CARTESIAN_POINT('Ctrl Pts',(54.2110747522833,27.1678832924025,17.6015488339026));
#50583=CARTESIAN_POINT('Ctrl Pts',(54.2158600966855,27.1658300814104,17.6018853871387));
#50584=CARTESIAN_POINT('Ctrl Pts',(54.2206660902525,27.1637902571315,17.6022216940722));
#50585=CARTESIAN_POINT('Ctrl Pts',(54.2206786884179,27.1637849102022,17.6022225756369));
#50586=CARTESIAN_POINT('Ctrl Pts',(54.2207039232623,27.1637742003039,17.6022243414379));
#50587=CARTESIAN_POINT('Ctrl Pts',(54.2207165598943,27.1637688373559,17.6022252256708));
#50588=CARTESIAN_POINT('Ctrl Pts',(54.2207418718281,27.1637580953568,17.602226996819));
#50589=CARTESIAN_POINT('Ctrl Pts',(54.2207545468393,27.1637527164301,17.6022278837139));
#50590=CARTESIAN_POINT('Ctrl Pts',(54.2207799348258,27.1637419427759,17.6022296601363));
#50591=CARTESIAN_POINT('Ctrl Pts',(54.2207926490437,27.163736547522,17.6022305497508));
#50592=CARTESIAN_POINT('Ctrl Pts',(54.2208181166296,27.1637257407132,17.6022323316952));
#50593=CARTESIAN_POINT('Ctrl Pts',(54.2208308690471,27.1637203295625,17.6022332239586));
#50594=CARTESIAN_POINT('Ctrl Pts',(54.2208564123642,27.1637094912463,17.6022350111539));
#50595=CARTESIAN_POINT('Ctrl Pts',(54.2208692047696,27.1637040634427,17.6022359061911));
#50596=CARTESIAN_POINT('Ctrl Pts',(54.2208948296117,27.1636931911664,17.6022376990422));
#50597=CARTESIAN_POINT('Ctrl Pts',(54.220907660359,27.1636877474114,17.6022385967379));
#50598=CARTESIAN_POINT('Ctrl Pts',(54.2209333618325,27.1636768432572,17.602240394902));
#50599=CARTESIAN_POINT('Ctrl Pts',(54.2209462329074,27.1636713827111,17.6022412953948));
#50600=CARTESIAN_POINT('Ctrl Pts',(54.2209720147674,27.1636604450916,17.6022430991341));
#50601=CARTESIAN_POINT('Ctrl Pts',(54.2209849256474,27.1636549679791,17.6022440023873));
#50602=CARTESIAN_POINT('Ctrl Pts',(54.2210107873937,27.1636439971125,17.6022458116664));
#50603=CARTESIAN_POINT('Ctrl Pts',(54.2210237384327,27.1636385032863,17.6022467177044));
#50604=CARTESIAN_POINT('Ctrl Pts',(54.2210496807063,27.1636274989068,17.6022485325678));
#50605=CARTESIAN_POINT('Ctrl Pts',(54.2210626721279,27.1636219882751,17.6022494414061));
#50606=CARTESIAN_POINT('Ctrl Pts',(54.221088695651,27.1636109500823,17.6022512619037));
#50607=CARTESIAN_POINT('Ctrl Pts',(54.2211017275756,27.1636054225971,17.6022521735505));
#50608=CARTESIAN_POINT('Ctrl Pts',(54.2211278324925,27.1635943505358,17.6022539996919));
#50609=CARTESIAN_POINT('Ctrl Pts',(54.2211409052794,27.1635888060479,17.6022549141721));
#50610=CARTESIAN_POINT('Ctrl Pts',(54.22116709213,27.1635776998954,17.6022567459947));
#50611=CARTESIAN_POINT('Ctrl Pts',(54.2211802060632,27.1635721382872,17.602257663328));
#50612=CARTESIAN_POINT('Ctrl Pts',(54.2212064748903,27.1635609980314,17.6022595008343));
#50613=CARTESIAN_POINT('Ctrl Pts',(54.2212196304669,27.1635554190954,17.602260421055));
#50614=CARTESIAN_POINT('Ctrl Pts',(54.2212459832692,27.163544243895,17.6022622643843));
#50615=CARTESIAN_POINT('Ctrl Pts',(54.2212591801162,27.1635386477924,17.6022631874663));
#50616=CARTESIAN_POINT('Ctrl Pts',(54.2212854599706,27.1635275041949,17.6022650256419));
#50617=CARTESIAN_POINT('Ctrl Pts',(54.2212985437312,27.1635219563777,17.6022659407885));
#50618=CARTESIAN_POINT('Ctrl Pts',(54.2213249053245,27.1635107787847,17.6022677846307));
#50619=CARTESIAN_POINT('Ctrl Pts',(54.2213381823626,27.1635051493506,17.6022687132703));
#50620=CARTESIAN_POINT('Ctrl Pts',(54.2213649339917,27.1634938070629,17.6022705843409));
#50621=CARTESIAN_POINT('Ctrl Pts',(54.2213784081539,27.163488094396,17.6022715267415));
#50622=CARTESIAN_POINT('Ctrl Pts',(54.2214055570371,27.1634765843835,17.6022734255431));
#50623=CARTESIAN_POINT('Ctrl Pts',(54.2214192315397,27.1634707871356,17.6022743819284));
#50624=CARTESIAN_POINT('Ctrl Pts',(54.2214467836432,27.1634591069002,17.6022763088758));
#50625=CARTESIAN_POINT('Ctrl Pts',(54.2214606621074,27.1634532235521,17.6022772794979));
#50626=CARTESIAN_POINT('Ctrl Pts',(54.2214886254689,27.163441369719,17.6022792351508));
#50627=CARTESIAN_POINT('Ctrl Pts',(54.2215027107765,27.1634353990655,17.60228022021));
#50628=CARTESIAN_POINT('Ctrl Pts',(54.2215310924091,27.1634233686951,17.6022822050563));
#50629=CARTESIAN_POINT('Ctrl Pts',(54.2215453876823,27.1634173094297,17.6022832047696));
#50630=CARTESIAN_POINT('Ctrl Pts',(54.2215741922858,27.1634051005644,17.6022852191354));
#50631=CARTESIAN_POINT('Ctrl Pts',(54.2215887020234,27.1633989507978,17.602286233816));
#50632=CARTESIAN_POINT('Ctrl Pts',(54.221617938954,27.1633865595075,17.6022882783528));
#50633=CARTESIAN_POINT('Ctrl Pts',(54.221632666116,27.1633803180032,17.6022893082064));
#50634=CARTESIAN_POINT('Ctrl Pts',(54.2216623412379,27.1633677418393,17.6022913833216));
#50635=CARTESIAN_POINT('Ctrl Pts',(54.221677289864,27.1633614069039,17.6022924286292));
#50636=CARTESIAN_POINT('Ctrl Pts',(54.2217074120727,27.1633486421346,17.6022945349418));
#50637=CARTESIAN_POINT('Ctrl Pts',(54.2217225853326,27.163342212444,17.6022955959236));
#50638=CARTESIAN_POINT('Ctrl Pts',(54.2217531610186,27.1633292564002,17.6022977338775));
#50639=CARTESIAN_POINT('Ctrl Pts',(54.2217685630084,27.1633227302387,17.6022988108185));
#50640=CARTESIAN_POINT('Ctrl Pts',(54.2257451600363,27.1616378176921,17.6025768587078));
#50641=CARTESIAN_POINT('Ctrl Pts',(54.2297117234843,27.1599722713291,17.6028530415225));
#50642=CARTESIAN_POINT('Ctrl Pts',(54.2386682606902,27.1562454903112,17.6034740649115));
#50643=CARTESIAN_POINT('Ctrl Pts',(54.2436612244966,27.1541916763677,17.6038184597301));
#50644=CARTESIAN_POINT('Ctrl Pts',(54.2584034658854,27.1481974414447,17.6048301849808));
#50645=CARTESIAN_POINT('Ctrl Pts',(54.268175811701,27.1443137377219,17.6054942394079));
#50646=CARTESIAN_POINT('Ctrl Pts',(54.3757655968861,27.1025377604369,17.6127378250549));
#50647=CARTESIAN_POINT('Ctrl Pts',(54.4764100865542,27.0723352431683,17.6189090372922));
#50648=CARTESIAN_POINT('Ctrl Pts',(54.6227855737681,27.0407282956951,17.6276321890022));
#50649=CARTESIAN_POINT('Ctrl Pts',(54.6669017465558,27.0327476206307,17.6302289151256));
#50650=CARTESIAN_POINT('Ctrl Pts',(54.8399505521809,27.0074312478132,17.640396164686));
#50651=CARTESIAN_POINT('Ctrl Pts',(54.9701665452203,27.0012379497982,17.6480321739293));
#50652=CARTESIAN_POINT('Ctrl Pts',(55.1186595281676,27.0086952332072,17.6572467609195));
#50653=CARTESIAN_POINT('Ctrl Pts',(55.137254736408,27.0098904907673,17.6584092137807));
#50654=CARTESIAN_POINT('Ctrl Pts',(55.1653170078396,27.0120894372619,17.6601775425317));
#50655=CARTESIAN_POINT('Ctrl Pts',(55.1747984436282,27.0129007026306,17.6607774370694));
#50656=CARTESIAN_POINT('Ctrl Pts',(55.191925084206,27.0144896439544,17.6618655886749));
#50657=CARTESIAN_POINT('Ctrl Pts',(55.1995723321909,27.0152437193823,17.6623531006616));
#50658=CARTESIAN_POINT('Ctrl Pts',(55.2159634796086,27.0169556964765,17.6634016380672));
#50659=CARTESIAN_POINT('Ctrl Pts',(55.224705756195,27.0179272835409,17.6639630813612));
#50660=CARTESIAN_POINT('Ctrl Pts',(55.2481767107033,27.0206930422779,17.6654764831163));
#50661=CARTESIAN_POINT('Ctrl Pts',(55.2628920422605,27.0225937526338,17.6664317492673));
#50662=CARTESIAN_POINT('Ctrl Pts',(55.3336380107139,27.0325353155998,17.6710562351777));
#50663=CARTESIAN_POINT('Ctrl Pts',(55.3893257329002,27.0427938204031,17.6747940950256));
#50664=CARTESIAN_POINT('Ctrl Pts',(55.6027961515303,27.0915891328643,17.6895109322272));
#50665=CARTESIAN_POINT('Ctrl Pts',(55.7560734251355,27.1469658488327,17.700975167431));
#50666=CARTESIAN_POINT('Ctrl Pts',(55.9422782234711,27.2412252414257,17.7153763809503));
#50667=CARTESIAN_POINT('Ctrl Pts',(55.9829017179762,27.2636009445861,17.7185447431241));
#50668=CARTESIAN_POINT('Ctrl Pts',(56.0377220973037,27.2963374453801,17.7228239905435));
#50669=CARTESIAN_POINT('Ctrl Pts',(56.0526153068573,27.3054988013607,17.7239868879664));
#50670=CARTESIAN_POINT('Ctrl Pts',(56.0781697105675,27.3216852018592,17.7259803515297));
#50671=CARTESIAN_POINT('Ctrl Pts',(56.0888872823697,27.3286188367388,17.7268158274645));
#50672=CARTESIAN_POINT('Ctrl Pts',(56.1043471453395,27.3388322876095,17.7280192898394));
#50673=CARTESIAN_POINT('Ctrl Pts',(56.1091426842319,27.3420303699639,17.7283923557106));
#50674=CARTESIAN_POINT('Ctrl Pts',(56.1175216589074,27.3476708230647,17.7290436772925));
#50675=CARTESIAN_POINT('Ctrl Pts',(56.1211110815544,27.3501041513765,17.7293225232524));
#50676=CARTESIAN_POINT('Ctrl Pts',(56.1287236711925,27.3553011646732,17.7299135220624));
#50677=CARTESIAN_POINT('Ctrl Pts',(56.1327446403439,27.3580679168016,17.7302254653136));
#50678=CARTESIAN_POINT('Ctrl Pts',(56.1436682042649,27.3656434386958,17.7310724180463));
#50679=CARTESIAN_POINT('Ctrl Pts',(56.1505506923276,27.3704812240284,17.7316055147836));
#50680=CARTESIAN_POINT('Ctrl Pts',(56.1827410347344,27.3934138371999,17.7340974171284));
#50681=CARTESIAN_POINT('Ctrl Pts',(56.2076554328252,27.4120566577362,17.7360218090352));
#50682=CARTESIAN_POINT('Ctrl Pts',(56.3937699748815,27.558236846224,17.7504499235633));
#50683=CARTESIAN_POINT('Ctrl Pts',(56.534834431795,27.7094265997486,17.7618160924564));
#50684=CARTESIAN_POINT('Ctrl Pts',(56.681139783878,27.9249152915941,17.777458158453));
#50685=CARTESIAN_POINT('Ctrl Pts',(56.7100716870995,27.971558406825,17.7808067421583));
#50686=CARTESIAN_POINT('Ctrl Pts',(56.7440476597548,28.0317395254409,17.7851136824006));
#50687=CARTESIAN_POINT('Ctrl Pts',(56.7509193465716,28.0442217771177,17.7860062213409));
#50688=CARTESIAN_POINT('Ctrl Pts',(56.7617146365337,28.0643383337482,17.787443929173));
#50689=CARTESIAN_POINT('Ctrl Pts',(56.7657237948351,28.0719263547986,17.7879860735772));
#50690=CARTESIAN_POINT('Ctrl Pts',(56.7732444982222,28.0863857184188,17.7890189621643));
#50691=CARTESIAN_POINT('Ctrl Pts',(56.776765389003,28.0932520440062,17.7895093675116));
#50692=CARTESIAN_POINT('Ctrl Pts',(56.7846910262917,28.1089317761663,17.790629141014));
#50693=CARTESIAN_POINT('Ctrl Pts',(56.7890704640952,28.1177576820218,17.7912593742738));
#50694=CARTESIAN_POINT('Ctrl Pts',(56.8002819012679,28.1407789470757,17.792903250329));
#50695=CARTESIAN_POINT('Ctrl Pts',(56.8070113335533,28.1550232199925,17.7939203852734));
#50696=CARTESIAN_POINT('Ctrl Pts',(56.8682703718384,28.2887702956405,17.8034727589273));
#50697=CARTESIAN_POINT('Ctrl Pts',(56.9110295851718,28.4132836362014,17.8124127544674));
#50698=CARTESIAN_POINT('Ctrl Pts',(56.9632725850951,28.6342687605549,17.8281845211868));
#50699=CARTESIAN_POINT('Ctrl Pts',(56.978565411335,28.7289316432631,17.8349027535602));
#50700=CARTESIAN_POINT('Ctrl Pts',(56.9919646082382,28.8804878471083,17.8453402503885));
#50701=CARTESIAN_POINT('Ctrl Pts',(56.9945470938814,28.936838950889,17.8491501643012));
#50702=CARTESIAN_POINT('Ctrl Pts',(56.9947709041649,29.0027727513714,17.8534711939293));
#50703=CARTESIAN_POINT('Ctrl Pts',(56.9947348070347,29.0123169206123,17.8540933146974));
#50704=CARTESIAN_POINT('Ctrl Pts',(56.9945740280993,29.0269868398502,17.8550440039881));
#50705=CARTESIAN_POINT('Ctrl Pts',(56.9944980849615,29.0321128261133,17.8553751545043));
#50706=CARTESIAN_POINT('Ctrl Pts',(56.994322068357,29.0415398341059,17.8559821766046));
#50707=CARTESIAN_POINT('Ctrl Pts',(56.9942278432773,29.0458408106386,17.8562583571489));
#50708=CARTESIAN_POINT('Ctrl Pts',(56.9939840170005,29.0555377282512,17.8568793199967));
#50709=CARTESIAN_POINT('Ctrl Pts',(56.9938264278445,29.0609333782337,17.8572236569441));
#50710=CARTESIAN_POINT('Ctrl Pts',(56.9932974282019,29.0768336343943,17.8582350529822));
#50711=CARTESIAN_POINT('Ctrl Pts',(56.9928648829864,29.0873362129997,17.858898839248));
#50712=CARTESIAN_POINT('Ctrl Pts',(56.9885803678744,29.1745875837308,17.8643814497677));
#50713=CARTESIAN_POINT('Ctrl Pts',(56.9803788827988,29.2510677792958,17.8689832328801));
#50714=CARTESIAN_POINT('Ctrl Pts',(56.9502425906742,29.4324783423043,17.8798039582074));
#50715=CARTESIAN_POINT('Ctrl Pts',(56.9242325719471,29.5364826414008,17.8859374371959));
#50716=CARTESIAN_POINT('Ctrl Pts',(56.8611302393796,29.7234456167472,17.897508191926));
#50717=CARTESIAN_POINT('Ctrl Pts',(56.8264860433627,29.8069233305392,17.9028893613067));
#50718=CARTESIAN_POINT('Ctrl Pts',(56.7764231232287,29.9076574456042,17.9098332291545));
#50719=CARTESIAN_POINT('Ctrl Pts',(56.7662041573711,29.9273855534195,17.9112153556383));
#50720=CARTESIAN_POINT('Ctrl Pts',(56.7508115781797,29.9559239570786,17.9132493580063));
#50721=CARTESIAN_POINT('Ctrl Pts',(56.7458961884439,29.9648721609598,17.9138921711154));
#50722=CARTESIAN_POINT('Ctrl Pts',(56.7371226612382,29.9805573354622,17.915028067297));
#50723=CARTESIAN_POINT('Ctrl Pts',(56.7332934513718,29.9873103043041,17.9155201145636));
#50724=CARTESIAN_POINT('Ctrl Pts',(56.725236657887,30.0013274568865,17.9165478282894));
#50725=CARTESIAN_POINT('Ctrl Pts',(56.7210023943069,30.0085876049615,17.9170837273449));
#50726=CARTESIAN_POINT('Ctrl Pts',(56.7098770974915,30.0273891974074,17.9184810481919));
#50727=CARTESIAN_POINT('Ctrl Pts',(56.7029151491255,30.0388879784544,17.9193450194241));
#50728=CARTESIAN_POINT('Ctrl Pts',(56.6740249701946,30.0855340224608,17.9228889918404));
#50729=CARTESIAN_POINT('Ctrl Pts',(56.6511219204021,30.1200623639201,17.9256043483224));
#50730=CARTESIAN_POINT('Ctrl Pts',(56.5261041751656,30.2963625699396,17.9399680452105));
#50731=CARTESIAN_POINT('Ctrl Pts',(56.4067711209741,30.4249650348056,17.9522781110881));
#50732=CARTESIAN_POINT('Ctrl Pts',(56.2202658086442,30.5794098049016,17.9690251889766));
#50733=CARTESIAN_POINT('Ctrl Pts',(56.1661190447471,30.6198000411304,17.9736363659764));
#50734=CARTESIAN_POINT('Ctrl Pts',(56.0981210486691,30.6653416873858,17.9790425256776));
#50735=CARTESIAN_POINT('Ctrl Pts',(56.0861328038122,30.6731850865667,17.9799818016131));
#50736=CARTESIAN_POINT('Ctrl Pts',(56.0689718464324,30.6841505941709,17.9813056588599));
#50737=CARTESIAN_POINT('Ctrl Pts',(56.0638681732421,30.687379194065,17.9816968045988));
#50738=CARTESIAN_POINT('Ctrl Pts',(56.055039858614,30.6929080369164,17.9823688803188));
#50739=CARTESIAN_POINT('Ctrl Pts',(56.0513221874479,30.6952192732507,17.9826505199787));
#50740=CARTESIAN_POINT('Ctrl Pts',(56.0435539934532,30.7000132925545,17.9832361121092));
#50741=CARTESIAN_POINT('Ctrl Pts',(56.03950218824,30.7024938572271,17.9835399225304));
#50742=CARTESIAN_POINT('Ctrl Pts',(56.0287526042198,30.7090222014675,17.9843417486125));
#50743=CARTESIAN_POINT('Ctrl Pts',(56.0220397206993,30.7130451307316,17.9848381824922));
#50744=CARTESIAN_POINT('Ctrl Pts',(55.9933191109478,30.7300280326622,17.9869446860678));
#50745=CARTESIAN_POINT('Ctrl Pts',(55.9710861694229,30.7426048446625,17.988531910429));
#50746=CARTESIAN_POINT('Ctrl Pts',(55.7793729537247,30.8462447649454,18.0019050651092));
#50747=CARTESIAN_POINT('Ctrl Pts',(55.5977660275354,30.9127827008792,18.0125997318855));
#50748=CARTESIAN_POINT('Ctrl Pts',(55.3385656942483,30.9671405592272,18.0283297222333));
#50749=CARTESIAN_POINT('Ctrl Pts',(55.2669619051846,30.9781300055519,18.0327093964411));
#50750=CARTESIAN_POINT('Ctrl Pts',(55.1795452669117,30.9867133314852,18.0381745538085));
#50751=CARTESIAN_POINT('Ctrl Pts',(55.1641493319842,30.9880446021534,18.0391413746449));
#50752=CARTESIAN_POINT('Ctrl Pts',(55.1399185658695,30.9898564287235,18.0406703818557));
#50753=CARTESIAN_POINT('Ctrl Pts',(55.1310931432675,30.9904573333141,18.0412288188772));
#50754=CARTESIAN_POINT('Ctrl Pts',(55.1145987996252,30.9914702248503,18.042275505755));
#50755=CARTESIAN_POINT('Ctrl Pts',(55.1069309050358,30.9918966640376,18.0427632962151));
#50756=CARTESIAN_POINT('Ctrl Pts',(55.089823695559,30.9927489923994,18.0438543403244));
#50757=CARTESIAN_POINT('Ctrl Pts',(55.0803834802504,30.9931521101139,18.044458290809));
#50758=CARTESIAN_POINT('Ctrl Pts',(55.0565244411337,30.994001165299,18.0459896168197));
#50759=CARTESIAN_POINT('Ctrl Pts',(55.0421031751652,30.9943577824104,18.046919738523));
#50760=CARTESIAN_POINT('Ctrl Pts',(54.9571838766018,30.9955362558557,18.0524244202368));
#50761=CARTESIAN_POINT('Ctrl Pts',(54.8866938513219,30.9927764287255,18.0571087171278));
#50762=CARTESIAN_POINT('Ctrl Pts',(54.6533071164275,30.9712159262342,18.0729996511112));
#50763=CARTESIAN_POINT('Ctrl Pts',(54.4926125923868,30.9360880585725,18.084622513298));
#50764=CARTESIAN_POINT('Ctrl Pts',(54.3050904240727,30.8701197511106,18.0982249773966));
#50765=CARTESIAN_POINT('Ctrl Pts',(54.2724542042124,30.8576664399839,18.100590829316));
#50766=CARTESIAN_POINT('Ctrl Pts',(54.226820196614,30.838866147518,18.1038814662716));
#50767=CARTESIAN_POINT('Ctrl Pts',(54.2135399501208,30.833225663482,18.1048369532052));
#50768=CARTESIAN_POINT('Ctrl Pts',(54.1902555979994,30.8230365586655,18.1065069898863));
#50769=CARTESIAN_POINT('Ctrl Pts',(54.1802258294138,30.818548490721,18.1072246316383));
#50770=CARTESIAN_POINT('Ctrl Pts',(54.1653006673944,30.8117212836476,18.1082894017579));
#50771=CARTESIAN_POINT('Ctrl Pts',(54.1603770977963,30.8094447682218,18.1086401374315));
#50772=CARTESIAN_POINT('Ctrl Pts',(54.1519381695338,30.8055009915392,18.109240330525));
#50773=CARTESIAN_POINT('Ctrl Pts',(54.1484183470432,30.8038435043014,18.1094903749864));
#50774=CARTESIAN_POINT('Ctrl Pts',(54.1404408438513,30.8000583369093,18.1100564124022));
#50775=CARTESIAN_POINT('Ctrl Pts',(54.1359862072817,30.7979243939776,18.1103720161398));
#50776=CARTESIAN_POINT('Ctrl Pts',(54.1239270093877,30.79209240298,18.1112252326808));
#50777=CARTESIAN_POINT('Ctrl Pts',(54.1163378599069,30.7883624615497,18.1117609292112));
#50778=CARTESIAN_POINT('Ctrl Pts',(54.0795671283573,30.7699990324613,18.1143514642539));
#50779=CARTESIAN_POINT('Ctrl Pts',(54.0507222224008,30.754698045739,18.1163682341222));
#50780=CARTESIAN_POINT('Ctrl Pts',(53.8445446736308,30.6387563692747,18.1307649890349));
#50781=CARTESIAN_POINT('Ctrl Pts',(53.6831845308571,30.5121560703674,18.1420502566199));
#50782=CARTESIAN_POINT('Ctrl Pts',(53.5063966227145,30.3233187905913,18.1575864865704));
#50783=CARTESIAN_POINT('Ctrl Pts',(53.4706512095115,30.2818405263651,18.1609272596754));
#50784=CARTESIAN_POINT('Ctrl Pts',(53.4278154519344,30.2277890798096,18.1652253853925));
#50785=CARTESIAN_POINT('Ctrl Pts',(53.4190921975894,30.2165363872221,18.1661172562577));
#50786=CARTESIAN_POINT('Ctrl Pts',(53.4053066393238,30.1983548134038,18.1675541428123));
#50787=CARTESIAN_POINT('Ctrl Pts',(53.4001671826546,30.1914848409589,18.1680961402357));
#50788=CARTESIAN_POINT('Ctrl Pts',(53.3904895710177,30.1783731550427,18.1691289145803));
#50789=CARTESIAN_POINT('Ctrl Pts',(53.3859429940054,30.1721378298651,18.169619353797));
#50790=CARTESIAN_POINT('Ctrl Pts',(53.3756716267862,30.1578782572735,18.1707394361714));
#50791=CARTESIAN_POINT('Ctrl Pts',(53.369969939187,30.1498376919417,18.1713699462091));
#50792=CARTESIAN_POINT('Ctrl Pts',(53.3553029427684,30.1288258405662,18.1730150195902));
#50793=CARTESIAN_POINT('Ctrl Pts',(53.3464315674151,30.1157901252531,18.1740330834592));
#50794=CARTESIAN_POINT('Ctrl Pts',(53.2654322607865,29.9936808876836,18.1835481770535));
#50795=CARTESIAN_POINT('Ctrl Pts',(53.2040521936149,29.8778877297199,18.1924460535315));
#50796=CARTESIAN_POINT('Ctrl Pts',(53.1185826541295,29.6694993110158,18.2080880314943));
#50797=CARTESIAN_POINT('Ctrl Pts',(53.0889773901164,29.5796150587301,18.2147178292819));
#50798=CARTESIAN_POINT('Ctrl Pts',(53.0588688089847,29.4602750038332,18.2231691213204));
#50799=CARTESIAN_POINT('Ctrl Pts',(53.0524777514281,29.4324352549098,18.2251158808612));
#50800=CARTESIAN_POINT('Ctrl Pts',(53.0466869962288,29.4044698651299,18.2270410618393));
#50801=CARTESIAN_POINT('Origin',(55.,29.,3.45145488139523));
#50802=CARTESIAN_POINT('',(53.0466869987623,29.4044698773653,19.1852189598335));
#50803=CARTESIAN_POINT('',(53.0466869973344,29.4044698704695,19.02544331564));
#50804=CARTESIAN_POINT('',(53.0466869980082,29.4044698737233,3.45145488139523));
#50805=CARTESIAN_POINT('',(53.0052500748225,29.0005463555814,18.4113483399464));
#50806=CARTESIAN_POINT('Ctrl Pts',(53.0466869987623,29.4044698773653,19.1852189598335));
#50807=CARTESIAN_POINT('Ctrl Pts',(53.0473612262886,29.4077259353972,19.1850147090984));
#50808=CARTESIAN_POINT('Ctrl Pts',(53.0480436373529,29.4109805106691,19.1848102091115));
#50809=CARTESIAN_POINT('Ctrl Pts',(53.0537663371002,29.4379375437896,19.1831134921491));
#50810=CARTESIAN_POINT('Ctrl Pts',(53.059229781962,29.461547012844,19.1816089637445));
#50811=CARTESIAN_POINT('Ctrl Pts',(53.0674968539547,29.4945245749462,19.179478881008));
#50812=CARTESIAN_POINT('Ctrl Pts',(53.0699414503623,29.5039811050769,19.1788647478418));
#50813=CARTESIAN_POINT('Ctrl Pts',(53.0743130575776,29.5203935582042,19.1777929312071));
#50814=CARTESIAN_POINT('Ctrl Pts',(53.0762085693706,29.5273577389787,19.1773362640326));
#50815=CARTESIAN_POINT('Ctrl Pts',(53.0802472017588,29.5418842465995,19.1763797217002));
#50816=CARTESIAN_POINT('Ctrl Pts',(53.0823973049675,29.5494444869004,19.1758796284688));
#50817=CARTESIAN_POINT('Ctrl Pts',(53.0876088770486,29.5673662731329,19.1746886584122));
#50818=CARTESIAN_POINT('Ctrl Pts',(53.090709932972,29.5777159573914,19.1739965114367));
#50819=CARTESIAN_POINT('Ctrl Pts',(53.1014437818026,29.6125092575854,19.1716546102347));
#50820=CARTESIAN_POINT('Ctrl Pts',(53.1094628792296,29.6368301176442,19.1699923927686));
#50821=CARTESIAN_POINT('Ctrl Pts',(53.1297722393553,29.6946575262177,19.1659776903143));
#50822=CARTESIAN_POINT('Ctrl Pts',(53.1424975298548,29.7280008717266,19.1636116926628));
#50823=CARTESIAN_POINT('Ctrl Pts',(53.1960533824514,29.8577686524445,19.1542000129544));
#50824=CARTESIAN_POINT('Ctrl Pts',(53.243551227458,29.9512484788758,19.14695833577));
#50825=CARTESIAN_POINT('Ctrl Pts',(53.361190148608,30.143647678873,19.1312465846423));
#50826=CARTESIAN_POINT('Ctrl Pts',(53.4334635779966,30.240804813961,19.1227893245507));
#50827=CARTESIAN_POINT('Ctrl Pts',(53.5246380934012,30.3426036864123,19.1137388689292));
#50828=CARTESIAN_POINT('Ctrl Pts',(53.53532376407,30.3542529214894,19.1127003753375));
#50829=CARTESIAN_POINT('Ctrl Pts',(53.5505732211759,30.3704858128896,19.1112507844475));
#50830=CARTESIAN_POINT('Ctrl Pts',(53.5550222216541,30.3751758336233,19.1108316703867));
#50831=CARTESIAN_POINT('Ctrl Pts',(53.5625455883242,30.3830299482655,19.1101294290633));
#50832=CARTESIAN_POINT('Ctrl Pts',(53.5656077672521,30.3862055934623,19.1098453887443));
#50833=CARTESIAN_POINT('Ctrl Pts',(53.5718806856916,30.3926679060776,19.1092672132134));
#50834=CARTESIAN_POINT('Ctrl Pts',(53.5750922835094,30.3959536786868,19.1089731476298));
#50835=CARTESIAN_POINT('Ctrl Pts',(53.5833095553217,30.4043028305138,19.1082255998842));
#50836=CARTESIAN_POINT('Ctrl Pts',(53.5883310888946,30.4093506110649,19.1077733341543));
#50837=CARTESIAN_POINT('Ctrl Pts',(53.6088891496666,30.4297960083727,19.1059396715377));
#50838=CARTESIAN_POINT('Ctrl Pts',(53.6246520842106,30.4449651299586,19.1045749792881));
#50839=CARTESIAN_POINT('Ctrl Pts',(53.6669604389453,30.4843599027799,19.101009056972));
#50840=CARTESIAN_POINT('Ctrl Pts',(53.6939172269262,30.5081335766629,19.0988344658239));
#50841=CARTESIAN_POINT('Ctrl Pts',(53.858719750057,30.6457406920399,19.0860061480243));
#50842=CARTESIAN_POINT('Ctrl Pts',(54.0107158702992,30.7413522000486,19.0759860422558));
#50843=CARTESIAN_POINT('Ctrl Pts',(54.2244025386128,30.8386444394249,19.0619063498638));
#50844=CARTESIAN_POINT('Ctrl Pts',(54.2763294469729,30.8596948317025,19.0584927976127));
#50845=CARTESIAN_POINT('Ctrl Pts',(54.3431604195879,30.8835639614664,19.0540744951304));
#50846=CARTESIAN_POINT('Ctrl Pts',(54.3573067972331,30.8884376768456,19.0531379388316));
#50847=CARTESIAN_POINT('Ctrl Pts',(54.3798000143404,30.8959050360664,19.0516461190086));
#50848=CARTESIAN_POINT('Ctrl Pts',(54.3881115561153,30.8986038176318,19.0510943015346));
#50849=CARTESIAN_POINT('Ctrl Pts',(54.4037010485234,30.9035527709367,19.0500581048983));
#50850=CARTESIAN_POINT('Ctrl Pts',(54.4109746994205,30.9058160414711,19.0495741631407));
#50851=CARTESIAN_POINT('Ctrl Pts',(54.4274078397576,30.9108263189888,19.0484796451272));
#50852=CARTESIAN_POINT('Ctrl Pts',(54.4365744262375,30.9135492209276,19.0478682994079));
#50853=CARTESIAN_POINT('Ctrl Pts',(54.4638797157178,30.9214469522576,19.0460446365198));
#50854=CARTESIAN_POINT('Ctrl Pts',(54.4820722140643,30.926430408249,19.0448261968074));
#50855=CARTESIAN_POINT('Ctrl Pts',(54.6334056875171,30.9655864948283,19.0346596194944));
#50856=CARTESIAN_POINT('Ctrl Pts',(54.7696566592804,30.9861647593858,19.0252692209402));
#50857=CARTESIAN_POINT('Ctrl Pts',(55.04164550012,30.9988709716941,19.0063281108385));
#50858=CARTESIAN_POINT('Ctrl Pts',(55.1766764946827,30.9914844926473,18.9968392517258));
#50859=CARTESIAN_POINT('Ctrl Pts',(55.3249319060831,30.9681659606946,18.986908721277));
#50860=CARTESIAN_POINT('Ctrl Pts',(55.3399006051719,30.9656361830665,18.9859120255489));
#50861=CARTESIAN_POINT('Ctrl Pts',(55.3604823329134,30.961915628234,18.9845511214463));
#50862=CARTESIAN_POINT('Ctrl Pts',(55.366120831676,30.9608712306551,18.9841792827924));
#50863=CARTESIAN_POINT('Ctrl Pts',(55.3757729757383,30.9590403159818,18.9835445467261));
#50864=CARTESIAN_POINT('Ctrl Pts',(55.3797888108251,30.9582657503111,18.9832809921011));
#50865=CARTESIAN_POINT('Ctrl Pts',(55.3881434546208,30.9566276578429,18.9827338333955));
#50866=CARTESIAN_POINT('Ctrl Pts',(55.3924818011706,30.955762043033,18.98245035858));
#50867=CARTESIAN_POINT('Ctrl Pts',(55.40299079337,30.9536288454599,18.9817651873235));
#50868=CARTESIAN_POINT('Ctrl Pts',(55.409158451742,30.9523464368005,18.9813643222031));
#50869=CARTESIAN_POINT('Ctrl Pts',(55.4308916211277,30.9477200608235,18.9799558891768));
#50870=CARTESIAN_POINT('Ctrl Pts',(55.4464235466126,30.9442188865876,18.9789567771364));
#50871=CARTESIAN_POINT('Ctrl Pts',(55.4846132961889,30.9351284304626,18.9765148384214));
#50872=CARTESIAN_POINT('Ctrl Pts',(55.5072185917325,30.9293266924921,18.9750822146106));
#50873=CARTESIAN_POINT('Ctrl Pts',(55.5999926576407,30.9037724682284,18.9692361598874));
#50874=CARTESIAN_POINT('Ctrl Pts',(55.6691592728681,30.8805765868043,18.9649562028322));
#50875=CARTESIAN_POINT('Ctrl Pts',(55.8944470716964,30.7910147613643,18.9508308234911));
#50876=CARTESIAN_POINT('Ctrl Pts',(56.0433440672059,30.7085657596047,18.9411217514176));
#50877=CARTESIAN_POINT('Ctrl Pts',(56.1983520944798,30.5948344255417,18.929260414512));
#50878=CARTESIAN_POINT('Ctrl Pts',(56.2164530149839,30.5810713406381,18.9278464005509));
#50879=CARTESIAN_POINT('Ctrl Pts',(56.2423216217464,30.5606948623709,18.9257810993182));
#50880=CARTESIAN_POINT('Ctrl Pts',(56.2502804955817,30.5543262661049,18.9251394256589));
#50881=CARTESIAN_POINT('Ctrl Pts',(56.2642331237616,30.5429850347085,18.9240032308046));
#50882=CARTESIAN_POINT('Ctrl Pts',(56.2702472678371,30.538037738261,18.9235097286749));
#50883=CARTESIAN_POINT('Ctrl Pts',(56.282639499884,30.5277214993771,18.9224849589668));
#50884=CARTESIAN_POINT('Ctrl Pts',(56.2890131970818,30.5223475426513,18.9219534941338));
#50885=CARTESIAN_POINT('Ctrl Pts',(56.3053395063284,30.5084060430735,18.9205806470208));
#50886=CARTESIAN_POINT('Ctrl Pts',(56.3152414125828,30.4997799940655,18.9197368799892));
#50887=CARTESIAN_POINT('Ctrl Pts',(56.3571811661686,30.4625094035105,18.9161144933386));
#50888=CARTESIAN_POINT('Ctrl Pts',(56.3883719288727,30.4329331428643,18.9132972883745));
#50889=CARTESIAN_POINT('Ctrl Pts',(56.469744892638,30.3506197720861,18.9056003616769));
#50890=CARTESIAN_POINT('Ctrl Pts',(56.5180328091014,30.2961089267274,18.9006491681735));
#50891=CARTESIAN_POINT('Ctrl Pts',(56.623998726839,30.1624224047797,18.888878393426));
#50892=CARTESIAN_POINT('Ctrl Pts',(56.6790438284208,30.0813920099518,18.8820144071344));
#50893=CARTESIAN_POINT('Ctrl Pts',(56.737621777617,29.9798342572689,18.8738978226494));
#50894=CARTESIAN_POINT('Ctrl Pts',(56.7470777350109,29.962872800663,18.8725578712145));
#50895=CARTESIAN_POINT('Ctrl Pts',(56.7619840039176,29.9351921859877,18.8703988597298));
#50896=CARTESIAN_POINT('Ctrl Pts',(56.7675876196233,29.9245572296108,18.8695758812791));
#50897=CARTESIAN_POINT('Ctrl Pts',(56.7943458862737,29.8726408353116,18.8655919107553));
#50898=CARTESIAN_POINT('Ctrl Pts',(56.8141542209255,29.8306770768205,18.862473742147));
#50899=CARTESIAN_POINT('Ctrl Pts',(56.8358816224618,29.780153988264,18.8588694745216));
#50900=CARTESIAN_POINT('Ctrl Pts',(56.8392293493898,29.7722285825898,18.8583083741708));
#50901=CARTESIAN_POINT('Ctrl Pts',(56.8446066222524,29.7592650835009,18.8573978576784));
#50902=CARTESIAN_POINT('Ctrl Pts',(56.8466670117456,29.7542400196845,18.8570466834973));
#50903=CARTESIAN_POINT('Ctrl Pts',(56.8503233490524,29.7452178133263,18.8564194208956));
#50904=CARTESIAN_POINT('Ctrl Pts',(56.8519269019202,29.7412238773746,18.8561428873038));
#50905=CARTESIAN_POINT('Ctrl Pts',(56.8554022931461,29.732486108511,18.8555403964567));
#50906=CARTESIAN_POINT('Ctrl Pts',(56.8572688685523,29.7277402832559,18.8552147526069));
#50907=CARTESIAN_POINT('Ctrl Pts',(56.8625307691064,29.7142096303184,18.8542907060947));
#50908=CARTESIAN_POINT('Ctrl Pts',(56.8658821618947,29.7054077034331,18.8536948431532));
#50909=CARTESIAN_POINT('Ctrl Pts',(56.8877957655498,29.646605916609,18.8497469092549));
#50910=CARTESIAN_POINT('Ctrl Pts',(56.904410385682,29.5958978490112,18.8464994719718));
#50911=CARTESIAN_POINT('Ctrl Pts',(56.9672952608692,29.3743061664164,18.8327347989551));
#50912=CARTESIAN_POINT('Ctrl Pts',(56.9927413634309,29.1983558426419,18.8228086119594));
#50913=CARTESIAN_POINT('Ctrl Pts',(56.9952531786524,28.9636582121487,18.8087497009117));
#50914=CARTESIAN_POINT('Ctrl Pts',(56.993367548543,28.9059741762281,18.8052366659452));
#50915=CARTESIAN_POINT('Ctrl Pts',(56.9878519494673,28.8335827366265,18.8007173255587));
#50916=CARTESIAN_POINT('Ctrl Pts',(56.9865519084127,28.8187223819696,18.7997837850739));
#50917=CARTESIAN_POINT('Ctrl Pts',(56.9842187287267,28.7951066312985,18.7982903704643));
#50918=CARTESIAN_POINT('Ctrl Pts',(56.9832939879066,28.7863409035592,18.7977338790707));
#50919=CARTESIAN_POINT('Ctrl Pts',(56.9814545716334,28.769947038771,18.7966889421048));
#50920=CARTESIAN_POINT('Ctrl Pts',(56.9805538615927,28.7623174742247,18.7962009419377));
#50921=CARTESIAN_POINT('Ctrl Pts',(56.9784419442129,28.7452744321718,18.7951069617425));
#50922=CARTESIAN_POINT('Ctrl Pts',(56.9772075871186,28.7358640617875,18.7945002672956));
#50923=CARTESIAN_POINT('Ctrl Pts',(56.9733679259799,28.7081281074441,18.7927040994539));
#50924=CARTESIAN_POINT('Ctrl Pts',(56.9705747103368,28.6898299726633,18.7915087767498));
#50925=CARTESIAN_POINT('Ctrl Pts',(56.9467229832438,28.5469396286167,18.7820906987389));
#50926=CARTESIAN_POINT('Ctrl Pts',(56.9141272656479,28.4245867032357,18.7734984083875));
#50927=CARTESIAN_POINT('Ctrl Pts',(56.8209758445084,28.1735056303051,18.7549115242551));
#50928=CARTESIAN_POINT('Ctrl Pts',(56.7577866594209,28.0464611547449,18.7449225827293));
#50929=CARTESIAN_POINT('Ctrl Pts',(56.6715104724981,27.9112217606078,18.7342548979639));
#50930=CARTESIAN_POINT('Ctrl Pts',(56.6611110832296,27.8954207381316,18.7330085065773));
#50931=CARTESIAN_POINT('Ctrl Pts',(56.646580868345,27.8740126946052,18.7313223563014));
#50932=CARTESIAN_POINT('Ctrl Pts',(56.6426435047852,27.8682764085016,18.7308708051146));
#50933=CARTESIAN_POINT('Ctrl Pts',(56.6363350020599,27.859187929455,18.7301559283263));
#50934=CARTESIAN_POINT('Ctrl Pts',(56.6339834313859,27.8558223188838,18.7298913196013));
#50935=CARTESIAN_POINT('Ctrl Pts',(56.6290834977863,27.8488553596692,18.7293438617016));
#50936=CARTESIAN_POINT('Ctrl Pts',(56.6265335648938,27.8452551847384,18.7290611324734));
#50937=CARTESIAN_POINT('Ctrl Pts',(56.6203515034614,27.836588020651,18.7283808212036));
#50938=CARTESIAN_POINT('Ctrl Pts',(56.6167074847994,27.8315294870879,18.7279840414686));
#50939=CARTESIAN_POINT('Ctrl Pts',(56.6039153994644,27.8139462473242,18.7266055126552));
#50940=CARTESIAN_POINT('Ctrl Pts',(56.5946447533087,27.8015108434554,18.7256317498743));
#50941=CARTESIAN_POINT('Ctrl Pts',(56.5371114815866,27.7261868642991,18.7197321273701));
#50942=CARTESIAN_POINT('Ctrl Pts',(56.4852750517037,27.6661062789453,18.7150193421612));
#50943=CARTESIAN_POINT('Ctrl Pts',(56.3814830028217,27.5593842549929,18.7062968685041));
#50944=CARTESIAN_POINT('Ctrl Pts',(56.3303943081412,27.512075170663,18.7022776433283));
#50945=CARTESIAN_POINT('Ctrl Pts',(56.1804514084427,27.3871344377957,18.690919920441));
#50946=CARTESIAN_POINT('Ctrl Pts',(56.0766023828346,27.3160397653366,18.6835217314814));
#50947=CARTESIAN_POINT('Ctrl Pts',(55.9529868977687,27.2475469319726,18.6747513305454));
#50948=CARTESIAN_POINT('Ctrl Pts',(55.9391162504912,27.2400748797364,18.6737680872499));
#50949=CARTESIAN_POINT('Ctrl Pts',(55.9164295509905,27.2281982264427,18.6721605653593));
#50950=CARTESIAN_POINT('Ctrl Pts',(55.9076666404438,27.2236931821994,18.671539807591));
#50951=CARTESIAN_POINT('Ctrl Pts',(55.8919821943532,27.2157761150218,18.6704288485784));
#50952=CARTESIAN_POINT('Ctrl Pts',(55.8850735128279,27.2123389636329,18.6699395332227));
#50953=CARTESIAN_POINT('Ctrl Pts',(55.8704396192563,27.2051640521082,18.6689030694874));
#50954=CARTESIAN_POINT('Ctrl Pts',(55.8627098989433,27.2014358957463,18.6683556015406));
#50955=CARTESIAN_POINT('Ctrl Pts',(55.8420838077113,27.1916511899194,18.6668945996668));
#50956=CARTESIAN_POINT('Ctrl Pts',(55.8291463843147,27.1856828242711,18.6659780687529));
#50957=CARTESIAN_POINT('Ctrl Pts',(55.7660912846575,27.1574091670254,18.6615095067478));
#50958=CARTESIAN_POINT('Ctrl Pts',(55.7151360724482,27.1370409904381,18.6578928442873));
#50959=CARTESIAN_POINT('Ctrl Pts',(55.4696618441733,27.0504738630547,18.640432294877));
#50960=CARTESIAN_POINT('Ctrl Pts',(55.2665651941625,27.0125004235771,18.6257111432123));
#50961=CARTESIAN_POINT('Ctrl Pts',(55.0300348456545,27.0052312618966,18.6097631508404));
#50962=CARTESIAN_POINT('Ctrl Pts',(54.9987746604324,27.005005472049,18.6076830294092));
#50963=CARTESIAN_POINT('Ctrl Pts',(54.9590951201889,27.005651647101,18.6050880841231));
#50964=CARTESIAN_POINT('Ctrl Pts',(54.9506708965019,27.0058422310436,18.6045397636911));
#50965=CARTESIAN_POINT('Ctrl Pts',(54.9373661608289,27.0062275915717,18.6036781548011));
#50966=CARTESIAN_POINT('Ctrl Pts',(54.9324848376813,27.0063869185538,18.6033629734354));
#50967=CARTESIAN_POINT('Ctrl Pts',(54.9232711550293,27.0067215332768,18.6027698765049));
#50968=CARTESIAN_POINT('Ctrl Pts',(54.9189388285235,27.0068930163214,18.6024917666173));
#50969=CARTESIAN_POINT('Ctrl Pts',(54.908853817549,27.0073251405435,18.6018461095837));
#50970=CARTESIAN_POINT('Ctrl Pts',(54.9031016690316,27.00759656758,18.6014791626053));
#50971=CARTESIAN_POINT('Ctrl Pts',(54.8846337437901,27.0085481829668,18.6003050273902));
#50972=CARTESIAN_POINT('Ctrl Pts',(54.8719229760259,27.0093252379516,18.5995029910424));
#50973=CARTESIAN_POINT('Ctrl Pts',(54.8418332689627,27.0114541332443,18.5976169243552));
#50974=CARTESIAN_POINT('Ctrl Pts',(54.8244626414741,27.0129121664063,18.5965380492067));
#50975=CARTESIAN_POINT('Ctrl Pts',(54.7611814264441,27.0190601094541,18.5926367822408));
#50976=CARTESIAN_POINT('Ctrl Pts',(54.7154156334403,27.0251153281871,18.589871127379));
#50977=CARTESIAN_POINT('Ctrl Pts',(54.5139592444471,27.0589194749927,18.5777870087624));
#50978=CARTESIAN_POINT('Ctrl Pts',(54.3616858640178,27.1035330096151,18.5688464610483));
#50979=CARTESIAN_POINT('Ctrl Pts',(54.1605800381065,27.1894559554453,18.5557719600474));
#50980=CARTESIAN_POINT('Ctrl Pts',(54.1060032905532,27.2157734372108,18.5520894513809));
#50981=CARTESIAN_POINT('Ctrl Pts',(54.0393784563446,27.2517256071935,18.5473783122144));
#50982=CARTESIAN_POINT('Ctrl Pts',(54.0261279657469,27.2590719877724,18.5464303739847));
#50983=CARTESIAN_POINT('Ctrl Pts',(54.0052565046965,27.2709564546964,18.5449191106362));
#50984=CARTESIAN_POINT('Ctrl Pts',(53.9975797343163,27.2753957526812,18.5443593094529));
#50985=CARTESIAN_POINT('Ctrl Pts',(53.9834439693576,27.2836964066747,18.5433210740231));
#50986=CARTESIAN_POINT('Ctrl Pts',(53.9769767070138,27.2875434232136,18.5428431628758));
#50987=CARTESIAN_POINT('Ctrl Pts',(53.9632465964651,27.2958162428832,18.5418222584892));
#50988=CARTESIAN_POINT('Ctrl Pts',(53.955989995881,27.3002520759287,18.5412789074299));
#50989=CARTESIAN_POINT('Ctrl Pts',(53.9406051945293,27.3097922235056,18.5401187577825));
#50990=CARTESIAN_POINT('Ctrl Pts',(53.9324850456039,27.3149090533706,18.539501510039));
#50991=CARTESIAN_POINT('Ctrl Pts',(53.9118109695318,27.3281460202252,18.5379172119835));
#50992=CARTESIAN_POINT('Ctrl Pts',(53.8993110106587,27.3363489475164,18.5369471371417));
#50993=CARTESIAN_POINT('Ctrl Pts',(53.8164262929565,27.3920839265698,18.530431822737));
#50994=CARTESIAN_POINT('Ctrl Pts',(53.7490557220949,27.4439229079121,18.524726697754));
#50995=CARTESIAN_POINT('Ctrl Pts',(53.596083468286,27.5779984125844,18.5107798769979));
#50996=CARTESIAN_POINT('Ctrl Pts',(53.5141063917076,27.6638907836862,18.5024455661607));
#50997=CARTESIAN_POINT('Ctrl Pts',(53.3954368462925,27.8127463847093,18.489285725354));
#50998=CARTESIAN_POINT('Ctrl Pts',(53.3536957451996,27.871337667361,18.4843836923746));
#50999=CARTESIAN_POINT('Ctrl Pts',(53.3096080021216,27.9408910531322,18.4789765428029));
#51000=CARTESIAN_POINT('Ctrl Pts',(53.30408006343,27.9497655271991,18.4782940068487));
#51001=CARTESIAN_POINT('Ctrl Pts',(53.2958104616855,27.9632769959848,18.4772664404504));
#51002=CARTESIAN_POINT('Ctrl Pts',(53.2930174853924,27.9678821452855,18.4769182342516));
#51003=CARTESIAN_POINT('Ctrl Pts',(53.2880274643022,27.9761855138605,18.476294104139));
#51004=CARTESIAN_POINT('Ctrl Pts',(53.2858237099634,27.9798795596938,18.4760177549317));
#51005=CARTESIAN_POINT('Ctrl Pts',(53.2810145613209,27.9880004902066,18.4754131201546));
#51006=CARTESIAN_POINT('Ctrl Pts',(53.2784143139336,27.9924303134935,18.4750851647352));
#51007=CARTESIAN_POINT('Ctrl Pts',(53.2710079325121,28.0051603229719,18.4741478983053));
#51008=CARTESIAN_POINT('Ctrl Pts',(53.2662444330619,28.0134853294479,18.473541242628));
#51009=CARTESIAN_POINT('Ctrl Pts',(53.2332995242657,28.0720377531291,18.4693159642909));
#51010=CARTESIAN_POINT('Ctrl Pts',(53.2072420711482,28.1234357631103,18.4658195759727));
#51011=CARTESIAN_POINT('Ctrl Pts',(53.0998465438268,28.3601652129511,18.4503351346781));
#51012=CARTESIAN_POINT('Ctrl Pts',(53.0447729023594,28.5560779080205,18.4390497704395));
#51013=CARTESIAN_POINT('Ctrl Pts',(53.0160515391722,28.7900292905039,18.4246625795518));
#51014=CARTESIAN_POINT('Ctrl Pts',(53.0128193889092,28.8232170409666,18.4226048395948));
#51015=CARTESIAN_POINT('Ctrl Pts',(53.0095320465334,28.868785031421,18.4197496550198));
#51016=CARTESIAN_POINT('Ctrl Pts',(53.0087579331777,28.8811090322041,18.4189744966872));
#51017=CARTESIAN_POINT('Ctrl Pts',(53.0077056049858,28.900779816542,18.4177321949085));
#51018=CARTESIAN_POINT('Ctrl Pts',(53.0073534894768,28.9081224566283,18.4172673536105));
#51019=CARTESIAN_POINT('Ctrl Pts',(53.0067283586573,28.9228605647168,18.4163320075453));
#51020=CARTESIAN_POINT('Ctrl Pts',(53.0064558966353,28.9302559379579,18.4158614931825));
#51021=CARTESIAN_POINT('Ctrl Pts',(53.0059888017183,28.9451929200034,18.4149087288716));
#51022=CARTESIAN_POINT('Ctrl Pts',(53.0057957876512,28.9527344546963,18.4144264364003));
#51023=CARTESIAN_POINT('Ctrl Pts',(53.0053782267271,28.973698648778,18.4130821811506));
#51024=CARTESIAN_POINT('Ctrl Pts',(53.0052463980734,28.9871225062247,18.4122173614862));
#51025=CARTESIAN_POINT('Ctrl Pts',(53.0052500748225,29.0005463555814,18.4113483399464));
#51026=CARTESIAN_POINT('Ctrl Pts',(53.0052500745292,29.0005452837287,18.4113484093351));
#51027=CARTESIAN_POINT('Ctrl Pts',(53.0052590846391,29.0335059519054,18.4092146306787));
#51028=CARTESIAN_POINT('Ctrl Pts',(53.0060850378228,29.0664600029808,18.4070558337636));
#51029=CARTESIAN_POINT('Ctrl Pts',(53.012837243978,29.201825273718,18.398079494748));
#51030=CARTESIAN_POINT('Ctrl Pts',(53.0258412931628,29.3037130880922,18.3910559369579));
#51031=CARTESIAN_POINT('Ctrl Pts',(53.046641082446,29.4042480853829,18.3839253224822));
#51032=CARTESIAN_POINT('Ctrl Pts',(53.0466640355231,29.404358980617,18.3839174568178));
#51033=CARTESIAN_POINT('Ctrl Pts',(53.0466869980087,29.4044698737256,18.3839095910714));
#51034=CARTESIAN_POINT('Ctrl Pts',(53.0466869962288,29.4044698651299,18.2270410618393));
#51035=CARTESIAN_POINT('Ctrl Pts',(53.0407025852386,29.3755692502392,18.2290306251703));
#51036=CARTESIAN_POINT('Ctrl Pts',(53.0353592981748,29.3465344503275,18.2309971371075));
#51037=CARTESIAN_POINT('Ctrl Pts',(53.0291327451794,29.3078996130939,18.2335620838893));
#51038=CARTESIAN_POINT('Ctrl Pts',(53.0276722830995,29.2984012296626,18.2341885508835));
#51039=CARTESIAN_POINT('Ctrl Pts',(53.0255360147488,29.2838061971304,18.2351444623848));
#51040=CARTESIAN_POINT('Ctrl Pts',(53.0248111973253,29.2787170281959,18.2354765322629));
#51041=CARTESIAN_POINT('Ctrl Pts',(53.023516034948,29.2693644358614,18.2360844291963));
#51042=CARTESIAN_POINT('Ctrl Pts',(53.0229398077778,29.2651019811977,18.2363605716051));
#51043=CARTESIAN_POINT('Ctrl Pts',(53.0216737041719,29.2555026155207,18.2369804420519));
#51044=CARTESIAN_POINT('Ctrl Pts',(53.0209916345264,29.2501647663337,18.2373237319712));
#51045=CARTESIAN_POINT('Ctrl Pts',(53.0190506529953,29.2344698249427,18.2383291803807));
#51046=CARTESIAN_POINT('Ctrl Pts',(53.0178513637173,29.2241053523241,18.2389881232356));
#51047=CARTESIAN_POINT('Ctrl Pts',(53.0091370429692,29.1432431205428,18.2440932978436));
#51048=CARTESIAN_POINT('Ctrl Pts',(53.0053031011992,29.0723912545005,18.2483552517889));
#51049=CARTESIAN_POINT('Ctrl Pts',(53.0051301413002,28.83900784537,18.2621308574038));
#51050=CARTESIAN_POINT('Ctrl Pts',(53.0248583520516,28.6771351772837,18.2713171826088));
#51051=CARTESIAN_POINT('Ctrl Pts',(53.0768676504811,28.4676071608181,18.2842867231159));
#51052=CARTESIAN_POINT('Ctrl Pts',(53.0918103494087,28.4163120081138,18.2875461999437));
#51053=CARTESIAN_POINT('Ctrl Pts',(53.1134714360907,28.3517299360444,18.2917886189302));
#51054=CARTESIAN_POINT('Ctrl Pts',(53.1183049004166,28.3378311149963,18.2927099377624));
#51055=CARTESIAN_POINT('Ctrl Pts',(53.1262347653306,28.3158166694844,18.2941830269197));
#51056=CARTESIAN_POINT('Ctrl Pts',(53.1292312233625,28.3076654241398,18.2947314997355));
#51057=CARTESIAN_POINT('Ctrl Pts',(53.1347137293017,28.2930468940223,18.2957207170945));
#51058=CARTESIAN_POINT('Ctrl Pts',(53.1371804383847,28.2865724671707,18.2961608137056));
#51059=CARTESIAN_POINT('Ctrl Pts',(53.1430422249385,28.2714245827083,18.2971952024989));
#51060=CARTESIAN_POINT('Ctrl Pts',(53.1464643992282,28.2627618506311,18.2977903904541));
#51061=CARTESIAN_POINT('Ctrl Pts',(53.1565471249258,28.2377529158072,18.2995194233414));
#51062=CARTESIAN_POINT('Ctrl Pts',(53.1633639949704,28.2214710846806,18.3006584761158));
#51063=CARTESIAN_POINT('Ctrl Pts',(53.2287448309737,28.0709509119039,18.3113165564617));
#51064=CARTESIAN_POINT('Ctrl Pts',(53.3016987081573,27.9434802639279,18.321345427733));
#51065=CARTESIAN_POINT('Ctrl Pts',(53.4125863212769,27.7913235569712,18.3344551193548));
#51066=CARTESIAN_POINT('Ctrl Pts',(53.4383076235699,27.7582681983959,18.3373773661658));
#51067=CARTESIAN_POINT('Ctrl Pts',(53.524402085484,27.6545354410124,18.3467513998617));
#51068=CARTESIAN_POINT('Ctrl Pts',(53.5886862966132,27.5872502709677,18.3531554281931));
#51069=CARTESIAN_POINT('Ctrl Pts',(53.6652994241423,27.5175307795837,18.3599592780833));
#51070=CARTESIAN_POINT('Ctrl Pts',(53.6732206427343,27.5104372568889,18.3606535856835));
#51071=CARTESIAN_POINT('Ctrl Pts',(53.6852677261663,27.4998213344304,18.361695294382));
#51072=CARTESIAN_POINT('Ctrl Pts',(53.6893517111335,27.4962520008137,18.362045999851));
#51073=CARTESIAN_POINT('Ctrl Pts',(53.6967020578062,27.4898806154345,18.3626727650686));
#51074=CARTESIAN_POINT('Ctrl Pts',(53.6999629625552,27.4870724458424,18.3629492668558));
#51075=CARTESIAN_POINT('Ctrl Pts',(53.7071123254989,27.4809558638196,18.3635520843739));
#51076=CARTESIAN_POINT('Ctrl Pts',(53.7110044002916,27.4776518230473,18.3638780841089));
#51077=CARTESIAN_POINT('Ctrl Pts',(53.7221326653525,27.4682781458621,18.3648041619869));
#51078=CARTESIAN_POINT('Ctrl Pts',(53.7293994518223,27.4622448118531,18.3654016827985));
#51079=CARTESIAN_POINT('Ctrl Pts',(53.7784653997161,27.4220925201614,18.3693902016324));
#51080=CARTESIAN_POINT('Ctrl Pts',(53.8215952317846,27.3896267105692,18.3726740802071));
#51081=CARTESIAN_POINT('Ctrl Pts',(54.0175782992013,27.2541976547176,18.3869028898807));
#51082=CARTESIAN_POINT('Ctrl Pts',(54.1829466849133,27.1709538031784,18.3972156162004));
#51083=CARTESIAN_POINT('Ctrl Pts',(54.4056218745212,27.0951806710256,18.4113712560602));
#51084=CARTESIAN_POINT('Ctrl Pts',(54.4544497524321,27.0806260660786,18.4144837913227));
#51085=CARTESIAN_POINT('Ctrl Pts',(54.5178054311023,27.0643539312551,18.4185589773504));
#51086=CARTESIAN_POINT('Ctrl Pts',(54.5318711944087,27.0609041514846,18.4194659462707));
#51087=CARTESIAN_POINT('Ctrl Pts',(54.5543798700972,27.0556428312966,18.4209213939677));
#51088=CARTESIAN_POINT('Ctrl Pts',(54.5627993107701,27.0537323788265,18.4214667125926));
#51089=CARTESIAN_POINT('Ctrl Pts',(54.5780045787958,27.0503857986823,18.4224532793849));
#51090=CARTESIAN_POINT('Ctrl Pts',(54.5847860335262,27.0489302858269,18.4228939026819));
#51091=CARTESIAN_POINT('Ctrl Pts',(54.6007633124383,27.045588131553,18.4239335472873));
#51092=CARTESIAN_POINT('Ctrl Pts',(54.6099650741759,27.0437309909132,18.4245334937821));
#51093=CARTESIAN_POINT('Ctrl Pts',(54.6368522229993,27.0385017474922,18.4262901436668));
#51094=CARTESIAN_POINT('Ctrl Pts',(54.6545701980414,27.0353041152861,18.42745231439));
#51095=CARTESIAN_POINT('Ctrl Pts',(54.6947645313817,27.028610590612,18.4300998358604));
#51096=CARTESIAN_POINT('Ctrl Pts',(54.7172619698113,27.0252584899838,18.4315894942432));
#51097=CARTESIAN_POINT('Ctrl Pts',(54.7912622744407,27.0155229480971,18.4365159578859));
#51098=CARTESIAN_POINT('Ctrl Pts',(54.8429540935004,27.0107648601882,18.4399999703326));
#51099=CARTESIAN_POINT('Ctrl Pts',(55.0223818338865,27.0012861503549,18.4522293164712));
#51100=CARTESIAN_POINT('Ctrl Pts',(55.1503411432454,27.0068239266349,18.4612110385858));
#51101=CARTESIAN_POINT('Ctrl Pts',(55.3544815594113,27.0354361229378,18.4754925726203));
#51102=CARTESIAN_POINT('Ctrl Pts',(55.4313875573193,27.0508781475049,18.4808543452591));
#51103=CARTESIAN_POINT('Ctrl Pts',(55.5173624180912,27.073481311968,18.486692022039));
#51104=CARTESIAN_POINT('Ctrl Pts',(55.5275107746108,27.0762353259464,18.4873785336689));
#51105=CARTESIAN_POINT('Ctrl Pts',(55.5428360415741,27.0805246184597,18.4884108788083));
#51106=CARTESIAN_POINT('Ctrl Pts',(55.5480290896857,27.0820008271946,18.4887599312577));
#51107=CARTESIAN_POINT('Ctrl Pts',(55.5573494601583,27.0846912391177,18.4893849504414));
#51108=CARTESIAN_POINT('Ctrl Pts',(55.5614788867583,27.0858977218983,18.489661348146));
#51109=CARTESIAN_POINT('Ctrl Pts',(55.5705199015236,27.0885709853777,18.490265353466));
#51110=CARTESIAN_POINT('Ctrl Pts',(55.5754297438452,27.0900433388983,18.4905926357886));
#51111=CARTESIAN_POINT('Ctrl Pts',(55.5894618585345,27.0943102814614,18.4915260460102));
#51112=CARTESIAN_POINT('Ctrl Pts',(55.598569978415,27.0971514575518,18.4921295525466));
#51113=CARTESIAN_POINT('Ctrl Pts',(55.6612785113328,27.1172074981358,18.4962705577758));
#51114=CARTESIAN_POINT('Ctrl Pts',(55.7141549468452,27.1366211181431,18.4996913224679));
#51115=CARTESIAN_POINT('Ctrl Pts',(55.8546172828006,27.1950515555501,18.5087618731247));
#51116=CARTESIAN_POINT('Ctrl Pts',(55.9403281595792,27.238184321841,18.5142833395687));
#51117=CARTESIAN_POINT('Ctrl Pts',(56.135410191401,27.3546637981494,18.5274931990627));
#51118=CARTESIAN_POINT('Ctrl Pts',(56.2412648990047,27.432982955264,18.5352098262511));
#51119=CARTESIAN_POINT('Ctrl Pts',(56.3503251252596,27.5317024327801,18.5443390757931));
#51120=CARTESIAN_POINT('Ctrl Pts',(56.361877498168,27.5424111184145,18.5453221375177));
#51121=CARTESIAN_POINT('Ctrl Pts',(56.3804471781398,27.5600381194265,18.5469294208817));
#51122=CARTESIAN_POINT('Ctrl Pts',(56.3875423191769,27.5668737194291,18.5475501234432));
#51123=CARTESIAN_POINT('Ctrl Pts',(56.4001036166386,27.5791562479326,18.5486610206546));
#51124=CARTESIAN_POINT('Ctrl Pts',(56.4055893890705,27.5845828983192,18.5491503297871));
#51125=CARTESIAN_POINT('Ctrl Pts',(56.4171097702815,27.5961121419487,18.5501868189951));
#51126=CARTESIAN_POINT('Ctrl Pts',(56.4231367428032,27.6022221111624,18.5507343188723));
#51127=CARTESIAN_POINT('Ctrl Pts',(56.4390654047547,27.6185799397475,18.5521954977465));
#51128=CARTESIAN_POINT('Ctrl Pts',(56.4488968846266,27.6288951818412,18.5531121750174));
#51129=CARTESIAN_POINT('Ctrl Pts',(56.4960551539321,27.6794475333306,18.5575826675015));
#51130=CARTESIAN_POINT('Ctrl Pts',(56.5318179060098,27.7211048590726,18.5612011819019));
#51131=CARTESIAN_POINT('Ctrl Pts',(56.6933115344229,27.9257214335051,18.578687386208));
#51132=CARTESIAN_POINT('Ctrl Pts',(56.7950169483812,28.1059811870624,18.5934357600824));
#51133=CARTESIAN_POINT('Ctrl Pts',(56.8782376999688,28.3275362617536,18.6093807727886));
#51134=CARTESIAN_POINT('Ctrl Pts',(56.8884400696301,28.3567436821395,18.611438929806));
#51135=CARTESIAN_POINT('Ctrl Pts',(56.9005429526428,28.3941662546026,18.6140105737047));
#51136=CARTESIAN_POINT('Ctrl Pts',(56.9030759141265,28.4021704984295,18.61455685502));
#51137=CARTESIAN_POINT('Ctrl Pts',(56.9070003598381,28.4148496130285,18.6154159929562));
#51138=CARTESIAN_POINT('Ctrl Pts',(56.9084253280006,28.4195138963993,18.6157307247132));
#51139=CARTESIAN_POINT('Ctrl Pts',(56.9110852607463,28.428336198533,18.6163234729626));
#51140=CARTESIAN_POINT('Ctrl Pts',(56.9123237569694,28.4324929739375,18.6166016804251));
#51141=CARTESIAN_POINT('Ctrl Pts',(56.9151785373924,28.4421899633094,18.6172482292355));
#51142=CARTESIAN_POINT('Ctrl Pts',(56.9167843472728,28.4477331848085,18.617615965024));
#51143=CARTESIAN_POINT('Ctrl Pts',(56.9218750043153,28.4655957182406,18.6187952154351));
#51144=CARTESIAN_POINT('Ctrl Pts',(56.9252653994951,28.4779419284413,18.6196015150863));
#51145=CARTESIAN_POINT('Ctrl Pts',(56.9532999380579,28.5840196062147,18.6264609482622));
#51146=CARTESIAN_POINT('Ctrl Pts',(56.9712048742252,28.6794120716764,18.6321776140071));
#51147=CARTESIAN_POINT('Ctrl Pts',(57.0016805624183,28.9487680762258,18.6479868402708));
#51148=CARTESIAN_POINT('Ctrl Pts',(56.9985166138154,29.1235952915863,18.6579373984282));
#51149=CARTESIAN_POINT('Ctrl Pts',(56.9694073378136,29.3177337735308,18.6700557836486));
#51150=CARTESIAN_POINT('Ctrl Pts',(56.9657508729171,29.3396225225335,18.6714363419178));
#51151=CARTESIAN_POINT('Ctrl Pts',(56.9599009750213,29.3713726336984,18.673461560028));
#51152=CARTESIAN_POINT('Ctrl Pts',(56.9579965327777,29.3812860299045,18.6740971303477));
#51153=CARTESIAN_POINT('Ctrl Pts',(56.9544928249464,29.3988054195163,18.6752262498478));
#51154=CARTESIAN_POINT('Ctrl Pts',(56.9529241865256,29.4064173769836,18.6757188209486));
#51155=CARTESIAN_POINT('Ctrl Pts',(56.9495720550315,29.4222162593013,18.6767453804029));
#51156=CARTESIAN_POINT('Ctrl Pts',(56.9477813846095,29.4304014888916,18.6772795880303));
#51157=CARTESIAN_POINT('Ctrl Pts',(56.9430097399748,29.4515730752197,18.6786675826109));
#51158=CARTESIAN_POINT('Ctrl Pts',(56.9399501624801,29.4645411120642,18.6795238557807));
#51159=CARTESIAN_POINT('Ctrl Pts',(56.926036172655,29.5209795520965,18.6832777698458));
#51160=CARTESIAN_POINT('Ctrl Pts',(56.9138495374494,29.5641049994275,18.6862175711223));
#51161=CARTESIAN_POINT('Ctrl Pts',(56.8521044768945,29.7574685807091,18.699734710844));
#51162=CARTESIAN_POINT('Ctrl Pts',(56.7862381142656,29.901880486207,18.7108250111487));
#51163=CARTESIAN_POINT('Ctrl Pts',(56.6592135092919,30.110617152795,18.7277915162128));
#51164=CARTESIAN_POINT('Ctrl Pts',(56.6096637734936,30.181289951954,18.7337132684562));
#51165=CARTESIAN_POINT('Ctrl Pts',(56.5490498850133,30.2568152501587,18.7400737030489));
#51166=CARTESIAN_POINT('Ctrl Pts',(56.5423433138017,30.2650364553803,18.7407664599797));
#51167=CARTESIAN_POINT('Ctrl Pts',(56.5321125695426,30.2773754344863,18.7418063069928));
#51168=CARTESIAN_POINT('Ctrl Pts',(56.5286368099669,30.2815328443955,18.7421566843741));
#51169=CARTESIAN_POINT('Ctrl Pts',(56.5223706122116,30.2889661742766,18.7427831021179));
#51170=CARTESIAN_POINT('Ctrl Pts',(56.5195864870218,30.2922472630651,18.7430595823234));
#51171=CARTESIAN_POINT('Ctrl Pts',(56.5134733665641,30.2994044929193,18.7436626314289));
#51172=CARTESIAN_POINT('Ctrl Pts',(56.510140093808,30.3032768570002,18.7439888825069));
#51173=CARTESIAN_POINT('Ctrl Pts',(56.5005906737215,30.31428488104,18.7449163955366));
#51174=CARTESIAN_POINT('Ctrl Pts',(56.4943384765876,30.3213892856868,18.7455150876824));
#51175=CARTESIAN_POINT('Ctrl Pts',(56.4518056362731,30.3690316003099,18.7495326948037));
#51176=CARTESIAN_POINT('Ctrl Pts',(56.4139267852265,30.40811907661,18.752842689817));
#51177=CARTESIAN_POINT('Ctrl Pts',(56.2367997439828,30.5765321205081,18.7674361109887));
#51178=CARTESIAN_POINT('Ctrl Pts',(56.0811087522357,30.6871097348985,18.7780543677325));
#51179=CARTESIAN_POINT('Ctrl Pts',(55.871404146068,30.7949312248483,18.7922999934147));
#51180=CARTESIAN_POINT('Ctrl Pts',(55.8299853814423,30.8144550322667,18.7951051890248));
#51181=CARTESIAN_POINT('Ctrl Pts',(55.7751261097204,30.8380428301046,18.7988282792918));
#51182=CARTESIAN_POINT('Ctrl Pts',(55.7622611121909,30.8434152848954,18.7997018705093));
#51183=CARTESIAN_POINT('Ctrl Pts',(55.7414502152256,30.8518508680827,18.8011162884634));
#51184=CARTESIAN_POINT('Ctrl Pts',(55.7335390250437,30.8549988017231,18.8016542651308));
#51185=CARTESIAN_POINT('Ctrl Pts',(55.7184060421686,30.8609084070653,18.8026840016023));
#51186=CARTESIAN_POINT('Ctrl Pts',(55.7111878566276,30.8636789344608,18.8031754550314));
#51187=CARTESIAN_POINT('Ctrl Pts',(55.6946172608157,30.8699288745247,18.8043044129638));
#51188=CARTESIAN_POINT('Ctrl Pts',(55.6852545432267,30.8733801909505,18.8049428351693));
#51189=CARTESIAN_POINT('Ctrl Pts',(55.6561235808694,30.8838709459333,18.8069310939632));
#51190=CARTESIAN_POINT('Ctrl Pts',(55.6362703897061,30.8906686198404,18.8082888191228));
#51191=CARTESIAN_POINT('Ctrl Pts',(55.5394806260597,30.9221120274313,18.8149233646866));
#51192=CARTESIAN_POINT('Ctrl Pts',(55.4612112935793,30.9423787615012,18.8203392730816));
#51193=CARTESIAN_POINT('Ctrl Pts',(55.2493265995765,30.9837133401762,18.8351085284237));
#51194=CARTESIAN_POINT('Ctrl Pts',(55.11444184238,30.9960415261751,18.8446422269414));
#51195=CARTESIAN_POINT('Ctrl Pts',(54.9668253165249,30.9945134605601,18.8547978023335));
#51196=CARTESIAN_POINT('Ctrl Pts',(54.9542996614176,30.9942657778632,18.8556570728379));
#51197=CARTESIAN_POINT('Ctrl Pts',(54.8926274306618,30.992464913638,18.8598734482139));
#51198=CARTESIAN_POINT('Ctrl Pts',(54.8435430683146,30.9892127617237,18.8631845260159));
#51199=CARTESIAN_POINT('Ctrl Pts',(54.7859086741132,30.9832471490268,18.8669830978606));
#51200=CARTESIAN_POINT('Ctrl Pts',(54.777198246606,30.9822875006682,18.8675547615788));
#51201=CARTESIAN_POINT('Ctrl Pts',(54.7630520033242,30.980634552783,18.8684789300756));
#51202=CARTESIAN_POINT('Ctrl Pts',(54.7576123326757,30.9799762133069,18.8688332792628));
#51203=CARTESIAN_POINT('Ctrl Pts',(54.7479017542589,30.9787603662588,18.8694639328039));
#51204=CARTESIAN_POINT('Ctrl Pts',(54.7436298833345,30.9782114338513,18.8697407035152));
#51205=CARTESIAN_POINT('Ctrl Pts',(54.7343407248548,30.9769871875198,18.8703410810926));
#51206=CARTESIAN_POINT('Ctrl Pts',(54.7293242250918,30.976306609899,18.870664391633));
#51207=CARTESIAN_POINT('Ctrl Pts',(54.715154561992,30.9743292782511,18.8715751654403));
#51208=CARTESIAN_POINT('Ctrl Pts',(54.7060076033033,30.9729879627099,18.8721602026378));
#51209=CARTESIAN_POINT('Ctrl Pts',(54.6479214046531,30.9640572388422,18.8758588437141));
#51210=CARTESIAN_POINT('Ctrl Pts',(54.5992653542875,30.9547104182692,18.8788824095813));
#51211=CARTESIAN_POINT('Ctrl Pts',(54.4112975053044,30.9112865687573,18.8904459816157));
#51212=CARTESIAN_POINT('Ctrl Pts',(54.2754714375952,30.8640415369295,18.8985754914798));
#51213=CARTESIAN_POINT('Ctrl Pts',(54.0628381808221,30.7632920782961,18.9124078370509));
#51214=CARTESIAN_POINT('Ctrl Pts',(53.9826262499427,30.7182603839796,18.9179098226958));
#51215=CARTESIAN_POINT('Ctrl Pts',(53.8929839932673,30.6594512359068,18.9245670447293));
#51216=CARTESIAN_POINT('Ctrl Pts',(53.8802565059526,30.6508898602387,18.925524723185));
#51217=CARTESIAN_POINT('Ctrl Pts',(53.8596209789639,30.6366605873085,18.9270986694933));
#51218=CARTESIAN_POINT('Ctrl Pts',(53.8516532853187,30.6310800125027,18.9277116591918));
#51219=CARTESIAN_POINT('Ctrl Pts',(53.8375988335926,30.6210822453082,18.9288024728939));
#51220=CARTESIAN_POINT('Ctrl Pts',(53.8314955973177,30.6166884598205,18.9292793991139));
#51221=CARTESIAN_POINT('Ctrl Pts',(53.8251649307816,30.6120763692274,18.9297775171614));
#51222=CARTESIAN_POINT('Ctrl Pts',(53.8249124851021,30.6118923637817,18.9297973861214));
#51223=CARTESIAN_POINT('Ctrl Pts',(53.8244569553259,30.6115601682289,18.9298332492671));
#51224=CARTESIAN_POINT('Ctrl Pts',(53.8242538559287,30.6114119989639,18.9298492426515));
#51225=CARTESIAN_POINT('Ctrl Pts',(53.8238852785896,30.6111430000358,18.9298782735545));
#51226=CARTESIAN_POINT('Ctrl Pts',(53.823719791243,30.6110221832642,18.9298913105751));
#51227=CARTESIAN_POINT('Ctrl Pts',(53.8234181170251,30.6108018697536,18.9299150808074));
#51228=CARTESIAN_POINT('Ctrl Pts',(53.8232819241786,30.6107023812554,18.9299258136994));
#51229=CARTESIAN_POINT('Ctrl Pts',(53.8230327537094,30.6105203144457,18.9299454530118));
#51230=CARTESIAN_POINT('Ctrl Pts',(53.8229197721184,30.6104377414894,18.9299543592271));
#51231=CARTESIAN_POINT('Ctrl Pts',(53.822712459295,30.6102861927797,18.9299707035706));
#51232=CARTESIAN_POINT('Ctrl Pts',(53.8226181254073,30.6102172206062,18.9299781415617));
#51233=CARTESIAN_POINT('Ctrl Pts',(53.8224446113756,30.610090332511,18.9299918241777));
#51234=CARTESIAN_POINT('Ctrl Pts',(53.8223654294075,30.6100324190119,18.9299980687106));
#51235=CARTESIAN_POINT('Ctrl Pts',(53.8221455068049,30.609871543251,18.9300154140449));
#51236=CARTESIAN_POINT('Ctrl Pts',(53.8220047753914,30.6097685683689,18.9300265153345));
#51237=CARTESIAN_POINT('Ctrl Pts',(53.821728154465,30.6095661057823,18.9300483394678));
#51238=CARTESIAN_POINT('Ctrl Pts',(53.8215922640638,30.6094666193337,18.9300590622619));
#51239=CARTESIAN_POINT('Ctrl Pts',(53.8213249348264,30.6092708534563,18.9300801598534));
#51240=CARTESIAN_POINT('Ctrl Pts',(53.8211934951526,30.6091745751084,18.9300905346105));
#51241=CARTESIAN_POINT('Ctrl Pts',(53.8209347144008,30.6089849718751,18.9301109636756));
#51242=CARTESIAN_POINT('Ctrl Pts',(53.8208073726633,30.6088916480173,18.9301210179408));
#51243=CARTESIAN_POINT('Ctrl Pts',(53.8205564681672,30.6087077239803,18.9301408309787));
#51244=CARTESIAN_POINT('Ctrl Pts',(53.8204329046768,30.6086171246157,18.9301505897242));
#51245=CARTESIAN_POINT('Ctrl Pts',(53.8201892656727,30.6084384401783,18.9301698344558));
#51246=CARTESIAN_POINT('Ctrl Pts',(53.820069189592,30.608350355901,18.9301793204105));
#51247=CARTESIAN_POINT('Ctrl Pts',(53.8198322599161,30.6081765104537,18.93019804031));
#51248=CARTESIAN_POINT('Ctrl Pts',(53.8197154058806,30.6080907500493,18.9302072742212));
#51249=CARTESIAN_POINT('Ctrl Pts',(53.819484677583,30.6079213774302,18.9302255090119));
#51250=CARTESIAN_POINT('Ctrl Pts',(53.8193708028546,30.6078377658539,18.9302345098665));
#51251=CARTESIAN_POINT('Ctrl Pts',(53.8191458103451,30.6076725301765,18.930252295975));
#51252=CARTESIAN_POINT('Ctrl Pts',(53.8190346921326,30.6075909066437,18.9302610812073));
#51253=CARTESIAN_POINT('Ctrl Pts',(53.8114118517275,30.601990219173,18.9308638350272));
#51254=CARTESIAN_POINT('Ctrl Pts',(53.8039390051373,30.5964186607103,18.9314598277423));
#51255=CARTESIAN_POINT('Ctrl Pts',(53.7883177230642,30.5846005913636,18.9327165883387));
#51256=CARTESIAN_POINT('Ctrl Pts',(53.780177935919,30.5783431502277,18.9333777721958));
#51257=CARTESIAN_POINT('Ctrl Pts',(53.7590295969497,30.5618241059551,18.935112414138));
#51258=CARTESIAN_POINT('Ctrl Pts',(53.7461001669936,30.5514629421171,18.9361897563826));
#51259=CARTESIAN_POINT('Ctrl Pts',(53.7078061444124,30.5199841641661,18.9394320252084));
#51260=CARTESIAN_POINT('Ctrl Pts',(53.6828360300003,30.4983977071286,18.9416151922173));
#51261=CARTESIAN_POINT('Ctrl Pts',(53.5441652558794,30.3723724950155,18.9541408431235));
#51262=CARTESIAN_POINT('Ctrl Pts',(53.4423683443152,30.2556400389244,18.9649756077121));
#51263=CARTESIAN_POINT('Ctrl Pts',(53.307567361331,30.0591266894262,18.9815128558532));
#51264=CARTESIAN_POINT('Ctrl Pts',(53.2644846681067,29.9869485312645,18.9872739244996));
#51265=CARTESIAN_POINT('Ctrl Pts',(53.2212344196793,29.9028469725585,18.9934850344956));
#51266=CARTESIAN_POINT('Ctrl Pts',(53.2164675859309,29.8933934101298,18.9941763114672));
#51267=CARTESIAN_POINT('Ctrl Pts',(53.209377067077,29.8790485690898,18.9952143813226));
#51268=CARTESIAN_POINT('Ctrl Pts',(53.2069977482108,29.8741852214916,18.9955644452487));
#51269=CARTESIAN_POINT('Ctrl Pts',(53.2027630392138,29.8654394166503,18.9961905314394));
#51270=CARTESIAN_POINT('Ctrl Pts',(53.2009003909755,29.861560604365,18.9964669914489));
#51271=CARTESIAN_POINT('Ctrl Pts',(53.1968517623983,29.8530592829174,18.9970702637217));
#51272=CARTESIAN_POINT('Ctrl Pts',(53.1946710020045,29.8484343918882,18.9973967564096));
#51273=CARTESIAN_POINT('Ctrl Pts',(53.1884972506746,29.8352097042761,18.9983256498074));
#51274=CARTESIAN_POINT('Ctrl Pts',(53.1845476939467,29.8265896162969,18.9989254686864));
#51275=CARTESIAN_POINT('Ctrl Pts',(53.1581741776796,29.7679272273677,19.0029713927468));
#51276=CARTESIAN_POINT('Ctrl Pts',(53.137758349,29.7170019555476,19.0063068100104));
#51277=CARTESIAN_POINT('Ctrl Pts',(53.0893253284311,29.5801003891777,19.0149745841698));
#51278=CARTESIAN_POINT('Ctrl Pts',(53.0650100751346,29.4929578116711,19.0201936490204));
#51279=CARTESIAN_POINT('Ctrl Pts',(53.0466869973344,29.4044698704695,19.02544331564));
#51280=CARTESIAN_POINT('Origin',(55.,29.,3.45145488139523));
#51281=CARTESIAN_POINT('',(53.0466870003186,29.404469884881,19.982208722643));
#51282=CARTESIAN_POINT('',(53.0466869979816,29.4044698735951,19.8236610414577));
#51283=CARTESIAN_POINT('',(53.0466869980082,29.4044698737233,3.45145488139523));
#51284=CARTESIAN_POINT('Ctrl Pts',(53.0466870003186,29.404469884881,19.982208722643));
#51285=CARTESIAN_POINT('Ctrl Pts',(53.0809855152632,29.5701082614707,19.9721559016089));
#51286=CARTESIAN_POINT('Ctrl Pts',(53.1362186434219,29.7307426871855,19.9626316675732));
#51287=CARTESIAN_POINT('Ctrl Pts',(53.2369797591282,29.9349931684407,19.9489879473138));
#51288=CARTESIAN_POINT('Ctrl Pts',(53.2651666453031,29.9863086988721,19.9454229282393));
#51289=CARTESIAN_POINT('Ctrl Pts',(53.3031188551555,30.0487293633254,19.9408720584243));
#51290=CARTESIAN_POINT('Ctrl Pts',(53.3108066690786,30.0610677501633,19.9399617063667));
#51291=CARTESIAN_POINT('Ctrl Pts',(53.3232804335094,30.080608071092,19.9385020991789));
#51292=CARTESIAN_POINT('Ctrl Pts',(53.3279796338778,30.0878649729846,19.9379560363604));
#51293=CARTESIAN_POINT('Ctrl Pts',(53.3369555199429,30.1015307442765,19.9369200256813));
#51294=CARTESIAN_POINT('Ctrl Pts',(53.3412224624332,30.1079458476772,19.9364304464665));
#51295=CARTESIAN_POINT('Ctrl Pts',(53.3509696889223,30.1224177204253,19.9353185355355));
#51296=CARTESIAN_POINT('Ctrl Pts',(53.3564720254768,30.1304593302738,19.9346953840858));
#51297=CARTESIAN_POINT('Ctrl Pts',(53.3708179444487,30.1510996147478,19.933082054274));
#51298=CARTESIAN_POINT('Ctrl Pts',(53.3797487038272,30.1636366308049,19.9320885943011));
#51299=CARTESIAN_POINT('Ctrl Pts',(53.4442043791538,30.2519388426516,19.924993147104));
#51300=CARTESIAN_POINT('Ctrl Pts',(53.5048668912053,30.3237912707411,19.9186918095494));
#51301=CARTESIAN_POINT('Ctrl Pts',(53.6902095118712,30.5142698031121,19.9004549542756));
#51302=CARTESIAN_POINT('Ctrl Pts',(53.8254705912628,30.6214323545154,19.8882053821055));
#51303=CARTESIAN_POINT('Ctrl Pts',(53.9859156762507,30.7178169434364,19.875706599145));
#51304=CARTESIAN_POINT('Ctrl Pts',(53.9991334958088,30.7255516042332,19.8746911161022));
#51305=CARTESIAN_POINT('Ctrl Pts',(54.0194651702628,30.7371368387581,19.8731521253314));
#51306=CARTESIAN_POINT('Ctrl Pts',(54.0265152481549,30.741097467672,19.8726226491175));
#51307=CARTESIAN_POINT('Ctrl Pts',(54.0395852710823,30.7483358054153,19.8716490184927));
#51308=CARTESIAN_POINT('Ctrl Pts',(54.0455983711186,30.7516255519124,19.8712041654684));
#51309=CARTESIAN_POINT('Ctrl Pts',(54.0555870247051,30.7570236030948,19.8704704413292));
#51310=CARTESIAN_POINT('Ctrl Pts',(54.059552911579,30.7591495344609,19.8701804843349));
#51311=CARTESIAN_POINT('Ctrl Pts',(54.0674227929945,30.7633339993845,19.8696078360786));
#51312=CARTESIAN_POINT('Ctrl Pts',(54.0713264726637,30.7653930215741,19.869325118415));
#51313=CARTESIAN_POINT('Ctrl Pts',(54.080973213246,30.7704404084755,19.8686296704532));
#51314=CARTESIAN_POINT('Ctrl Pts',(54.086724113237,30.7734138355636,19.868217866661));
#51315=CARTESIAN_POINT('Ctrl Pts',(54.106616961713,30.7835767398903,19.866802643581));
#51316=CARTESIAN_POINT('Ctrl Pts',(54.1208305594225,30.7906256928368,19.8658074961266));
#51317=CARTESIAN_POINT('Ctrl Pts',(54.2425621597303,30.8491970836889,19.8574076158891));
#51318=CARTESIAN_POINT('Ctrl Pts',(54.3544304914475,30.8911609295634,19.8504904324379));
#51319=CARTESIAN_POINT('Ctrl Pts',(54.5714065844679,30.9510343487714,19.8374189133662));
#51320=CARTESIAN_POINT('Ctrl Pts',(54.6754970631497,30.9710208435891,19.831285456852));
#51321=CARTESIAN_POINT('Ctrl Pts',(54.8347017216589,30.9886323575099,19.821662676116));
#51322=CARTESIAN_POINT('Ctrl Pts',(54.8889460492788,30.9923976504616,19.8183444698508));
#51323=CARTESIAN_POINT('Ctrl Pts',(54.9574737023675,30.9943472359192,19.8140718161429));
#51324=CARTESIAN_POINT('Ctrl Pts',(54.9716779375989,30.9945995156371,19.8131818853279));
#51325=CARTESIAN_POINT('Ctrl Pts',(54.9944559243433,30.9947607169895,19.8117473834205));
#51326=CARTESIAN_POINT('Ctrl Pts',(55.0030286679562,30.9947661212021,19.8112058125552));
#51327=CARTESIAN_POINT('Ctrl Pts',(55.0193193191825,30.9946713763764,19.810173368059));
#51328=CARTESIAN_POINT('Ctrl Pts',(55.0270371491961,30.9945816919003,19.8096828288425));
#51329=CARTESIAN_POINT('Ctrl Pts',(55.0446221043676,30.9942752658199,19.8085618423534));
#51330=CARTESIAN_POINT('Ctrl Pts',(55.0544884707148,30.9940300822371,19.8079305230116));
#51331=CARTESIAN_POINT('Ctrl Pts',(55.0801535500153,30.9932016719954,19.8062819479021));
#51332=CARTESIAN_POINT('Ctrl Pts',(55.0959476220709,30.9925038336013,19.8052611670606));
#51333=CARTESIAN_POINT('Ctrl Pts',(55.2277109001588,30.9851118095156,19.7966911438192));
#51334=CARTESIAN_POINT('Ctrl Pts',(55.3428802889527,30.9684882466191,19.7888304477018));
#51335=CARTESIAN_POINT('Ctrl Pts',(55.5359760102981,30.9231529866264,19.775107132445));
#51336=CARTESIAN_POINT('Ctrl Pts',(55.6147805215814,30.8994294389724,19.7693494140294));
#51337=CARTESIAN_POINT('Ctrl Pts',(55.7635030793175,30.844429399546,19.7583482866169));
#51338=CARTESIAN_POINT('Ctrl Pts',(55.833540638356,30.8138547793134,19.7531072022106));
#51339=CARTESIAN_POINT('Ctrl Pts',(55.9152415893866,30.7724537400094,19.7470489452602));
#51340=CARTESIAN_POINT('Ctrl Pts',(55.9287455633322,30.7654152881345,19.7460495878322));
#51341=CARTESIAN_POINT('Ctrl Pts',(55.947622953794,30.7552995755015,19.7446567488043));
#51342=CARTESIAN_POINT('Ctrl Pts',(55.9530642704512,30.7523510952891,19.7442557634354));
#51343=CARTESIAN_POINT('Ctrl Pts',(55.9623535798591,30.7472614399443,19.743572170244));
#51344=CARTESIAN_POINT('Ctrl Pts',(55.9662083420439,30.745132772437,19.7432887873472));
#51345=CARTESIAN_POINT('Ctrl Pts',(55.9741570665803,30.7407089358132,19.7427050717838));
#51346=CARTESIAN_POINT('Ctrl Pts',(55.9782500076183,30.7384120665946,19.7424048490615));
#51347=CARTESIAN_POINT('Ctrl Pts',(55.9889208990069,30.7323741747402,19.7416229208344));
#51348=CARTESIAN_POINT('Ctrl Pts',(55.9954858097408,30.7286100869687,19.7411426591838));
#51349=CARTESIAN_POINT('Ctrl Pts',(56.0222535387391,30.7130593488149,19.7391870334872));
#51350=CARTESIAN_POINT('Ctrl Pts',(56.0422706359667,30.7009546328631,19.7377306685757));
#51351=CARTESIAN_POINT('Ctrl Pts',(56.2269903972806,30.5847653917481,19.7243036199759));
#51352=CARTESIAN_POINT('Ctrl Pts',(56.3758416579623,30.4574183040491,19.7134855734595));
#51353=CARTESIAN_POINT('Ctrl Pts',(56.535378260469,30.274339204396,19.6990640616802));
#51354=CARTESIAN_POINT('Ctrl Pts',(56.5655646831117,30.2370665127549,19.696181706194));
#51355=CARTESIAN_POINT('Ctrl Pts',(56.6136016011858,30.1731755042671,19.6912939990029));
#51356=CARTESIAN_POINT('Ctrl Pts',(56.6322069473577,30.147149160133,19.6893168825357));
#51357=CARTESIAN_POINT('Ctrl Pts',(56.6567977492473,30.1109399738721,19.6865789739702));
#51358=CARTESIAN_POINT('Ctrl Pts',(56.6633311804523,30.1011338620458,19.6858387557726));
#51359=CARTESIAN_POINT('Ctrl Pts',(56.6741808027612,30.0845326154817,19.6845874213316));
#51360=CARTESIAN_POINT('Ctrl Pts',(56.6785434884909,30.0777681144629,19.6840780422092));
#51361=CARTESIAN_POINT('Ctrl Pts',(56.6870876914727,30.0643423038906,19.683067948061));
#51362=CARTESIAN_POINT('Ctrl Pts',(56.6912709926829,30.057682298701,19.6825673108078));
#51363=CARTESIAN_POINT('Ctrl Pts',(56.7004143226992,30.0429327564139,19.6814594359579));
#51364=CARTESIAN_POINT('Ctrl Pts',(56.7053562110417,30.034832252872,19.6808515510307));
#51365=CARTESIAN_POINT('Ctrl Pts',(56.7221331416946,30.0068857592873,19.6787560933355));
#51366=CARTESIAN_POINT('Ctrl Pts',(56.7336806731489,29.9868701736201,19.6772582454576));
#51367=CARTESIAN_POINT('Ctrl Pts',(56.8238865692704,29.8240431471759,19.6650920276266));
#51368=CARTESIAN_POINT('Ctrl Pts',(56.8850985591302,29.67230386812,19.6537935042898));
#51369=CARTESIAN_POINT('Ctrl Pts',(56.9545767036112,29.4122358606628,19.6350365087271));
#51370=CARTESIAN_POINT('Ctrl Pts',(56.9737539259589,29.3075855530193,19.6276613640761));
#51371=CARTESIAN_POINT('Ctrl Pts',(56.9858006598142,29.1891740677725,19.619817369963));
#51372=CARTESIAN_POINT('Ctrl Pts',(56.9869726282983,29.1764394601699,19.6189803292083));
#51373=CARTESIAN_POINT('Ctrl Pts',(56.9884954466862,29.1579452257679,19.6177750396574));
#51374=CARTESIAN_POINT('Ctrl Pts',(56.9889438765151,29.1521942637276,19.6174016903485));
#51375=CARTESIAN_POINT('Ctrl Pts',(56.9896857531418,29.1421160642841,19.6167500482779));
#51376=CARTESIAN_POINT('Ctrl Pts',(56.9899900426221,29.1377897081094,19.6164711633991));
#51377=CARTESIAN_POINT('Ctrl Pts',(56.9906066311998,29.1285947197375,19.6158802724591));
#51378=CARTESIAN_POINT('Ctrl Pts',(56.9909151814092,29.1237259220304,19.6155684748353));
#51379=CARTESIAN_POINT('Ctrl Pts',(56.9917064892622,29.110469063948,19.6147223332519));
#51380=CARTESIAN_POINT('Ctrl Pts',(56.992154125241,29.102078894279,19.6141898958572));
#51381=CARTESIAN_POINT('Ctrl Pts',(56.9940047379995,29.0627193609686,19.61170554401));
#51382=CARTESIAN_POINT('Ctrl Pts',(56.9947387391731,29.0317210075871,19.6097877921708));
#51383=CARTESIAN_POINT('Ctrl Pts',(56.9948237145519,28.7950532744245,19.5953573526225));
#51384=CARTESIAN_POINT('Ctrl Pts',(56.9630938523464,28.5906002848818,19.5839853449259));
#51385=CARTESIAN_POINT('Ctrl Pts',(56.8840039905391,28.3423009104254,19.5683356404376));
#51386=CARTESIAN_POINT('Ctrl Pts',(56.8651991233053,28.2907253414678,19.5649865024792));
#51387=CARTESIAN_POINT('Ctrl Pts',(56.8388642931578,28.2268190900567,19.5606789363534));
#51388=CARTESIAN_POINT('Ctrl Pts',(56.8332943235612,28.2137032908676,19.5597863496411));
#51389=CARTESIAN_POINT('Ctrl Pts',(56.8241452856285,28.1927855339599,19.558348582819));
#51390=CARTESIAN_POINT('Ctrl Pts',(56.8206554817723,28.1849448912794,19.5578064276401));
#51391=CARTESIAN_POINT('Ctrl Pts',(56.8139320632165,28.1700978518033,19.5567735301981));
#51392=CARTESIAN_POINT('Ctrl Pts',(56.8107081697433,28.1630872047548,19.5562831268507));
#51393=CARTESIAN_POINT('Ctrl Pts',(56.8032755155427,28.1471682181404,19.5551633742045));
#51394=CARTESIAN_POINT('Ctrl Pts',(56.7990412938667,28.1382720554921,19.5545331599245));
#51395=CARTESIAN_POINT('Ctrl Pts',(56.7878662564414,28.1152345170071,19.5528893667873));
#51396=CARTESIAN_POINT('Ctrl Pts',(56.7808236282824,28.1011435641362,19.5518722963646));
#51397=CARTESIAN_POINT('Ctrl Pts',(56.7134837752296,27.9703078501442,19.5423173556185));
#51398=CARTESIAN_POINT('Ctrl Pts',(56.6419676893934,27.8597268044612,19.5333744583581));
#51399=CARTESIAN_POINT('Ctrl Pts',(56.5003870086894,27.6820264044872,19.517593577708));
#51400=CARTESIAN_POINT('Ctrl Pts',(56.4353301739288,27.6114599644888,19.510869076918));
#51401=CARTESIAN_POINT('Ctrl Pts',(56.3244383129585,27.5073326322989,19.5004343766566));
#51402=CARTESIAN_POINT('Ctrl Pts',(56.2818102664538,27.4705699028715,19.4966327867027));
#51403=CARTESIAN_POINT('Ctrl Pts',(56.230199956324,27.4297367655303,19.4923199277571));
#51404=CARTESIAN_POINT('Ctrl Pts',(56.2226765135045,27.42387160737,19.4916981193046));
#51405=CARTESIAN_POINT('Ctrl Pts',(56.2110463573182,27.4149383124835,19.4907478052342));
#51406=CARTESIAN_POINT('Ctrl Pts',(56.2069695324575,27.411831752632,19.4904167207292));
#51407=CARTESIAN_POINT('Ctrl Pts',(56.1994488248153,27.4061466230073,19.489809760966));
#51408=CARTESIAN_POINT('Ctrl Pts',(56.1960085859419,27.4035634889783,19.4895335772083));
#51409=CARTESIAN_POINT('Ctrl Pts',(56.1882319667504,27.3977635924435,19.4889125339968));
#51410=CARTESIAN_POINT('Ctrl Pts',(56.1838908745714,27.3945532985316,19.4885681204272));
#51411=CARTESIAN_POINT('Ctrl Pts',(56.1710556528962,27.3851418569298,19.4875562892174));
#51412=CARTESIAN_POINT('Ctrl Pts',(56.1625253008029,27.3789900985121,19.4868921486032));
#51413=CARTESIAN_POINT('Ctrl Pts',(56.0899237891398,27.3275005991908,19.4813060466464));
#51414=CARTESIAN_POINT('Ctrl Pts',(56.0232687995311,27.2859077966735,19.476610700372));
#51415=CARTESIAN_POINT('Ctrl Pts',(55.8421042918325,27.1872064651714,19.4644809402379));
#51416=CARTESIAN_POINT('Ctrl Pts',(55.7242655217244,27.1369915904744,19.4571901841058));
#51417=CARTESIAN_POINT('Ctrl Pts',(55.5530467115627,27.0827492319694,19.4465574078655));
#51418=CARTESIAN_POINT('Ctrl Pts',(55.5030744296854,27.0690347720489,19.4434526049287));
#51419=CARTESIAN_POINT('Ctrl Pts',(55.4305024857964,27.0521264765659,19.4389038030478));
#51420=CARTESIAN_POINT('Ctrl Pts',(55.4082916699949,27.0473501327574,19.4375064648245));
#51421=CARTESIAN_POINT('Ctrl Pts',(55.3683579969855,27.0394736747881,19.4349819348445));
#51422=CARTESIAN_POINT('Ctrl Pts',(55.350665422506,27.0362319856017,19.4338591958836));
#51423=CARTESIAN_POINT('Ctrl Pts',(55.3236797041584,27.0316638836034,19.4321392608121));
#51424=CARTESIAN_POINT('Ctrl Pts',(55.3144167333096,27.0301630191847,19.4315475544084));
#51425=CARTESIAN_POINT('Ctrl Pts',(55.298289723885,27.0276666344277,19.430514930585));
#51426=CARTESIAN_POINT('Ctrl Pts',(55.2914303899745,27.0266414440981,19.4300749535121));
#51427=CARTESIAN_POINT('Ctrl Pts',(55.2760183492369,27.0244200820794,19.4290845915252));
#51428=CARTESIAN_POINT('Ctrl Pts',(55.2674629817585,27.0232436440592,19.4285335968298));
#51429=CARTESIAN_POINT('Ctrl Pts',(55.2445295003389,27.0202416950568,19.4270531654654));
#51430=CARTESIAN_POINT('Ctrl Pts',(55.2301388951744,27.0185172992992,19.4261205896033));
#51431=CARTESIAN_POINT('Ctrl Pts',(55.1649688744876,27.0114276149592,19.4218801157838));
#51432=CARTESIAN_POINT('Ctrl Pts',(55.1140175347032,27.0078569115449,19.4185170710026));
#51433=CARTESIAN_POINT('Ctrl Pts',(54.8789311883801,27.0004298061275,19.4027710055126));
#51434=CARTESIAN_POINT('Ctrl Pts',(54.694963403131,27.0201332395865,19.3896932137029));
#51435=CARTESIAN_POINT('Ctrl Pts',(54.4640230463797,27.0778485192307,19.3733859283527));
#51436=CARTESIAN_POINT('Ctrl Pts',(54.4122345519854,27.0930467956845,19.3697456423188));
#51437=CARTESIAN_POINT('Ctrl Pts',(54.3521747163503,27.1133524026632,19.3655915170578));
#51438=CARTESIAN_POINT('Ctrl Pts',(54.3432494279742,27.1164407497424,19.3649759860419));
#51439=CARTESIAN_POINT('Ctrl Pts',(54.3295336419076,27.1212960615824,19.3640332199847));
#51440=CARTESIAN_POINT('Ctrl Pts',(54.3247275740477,27.1230181733128,19.363703468125));
#51441=CARTESIAN_POINT('Ctrl Pts',(54.3158824854726,27.1262259185069,19.3630977641005));
#51442=CARTESIAN_POINT('Ctrl Pts',(54.3118416777655,27.1277061645309,19.3628215127369));
#51443=CARTESIAN_POINT('Ctrl Pts',(54.3027186368942,27.131081681143,19.362198830599));
#51444=CARTESIAN_POINT('Ctrl Pts',(54.2976393317177,27.132984607667,19.3618528564744));
#51445=CARTESIAN_POINT('Ctrl Pts',(54.282625649235,27.138679320949,19.3608321282679));
#51446=CARTESIAN_POINT('Ctrl Pts',(54.2727135738986,27.1425299207035,19.3601607377418));
#51447=CARTESIAN_POINT('Ctrl Pts',(54.1784857909409,27.180005047721,19.3537978312573));
#51448=CARTESIAN_POINT('Ctrl Pts',(54.0965154595727,27.2192733896552,19.3484104391332));
#51449=CARTESIAN_POINT('Ctrl Pts',(53.9148739286312,27.3220746107217,19.336202371856));
#51450=CARTESIAN_POINT('Ctrl Pts',(53.8176058788225,27.3891380697575,19.329448738821));
#51451=CARTESIAN_POINT('Ctrl Pts',(53.6881860802265,27.4964402887968,19.3194833405899));
#51452=CARTESIAN_POINT('Ctrl Pts',(53.6507669388669,27.529926132263,19.3164710132448));
#51453=CARTESIAN_POINT('Ctrl Pts',(53.5986578340375,27.5802247087775,19.3120468714056));
#51454=CARTESIAN_POINT('Ctrl Pts',(53.5829230052124,27.5959293192739,19.3106787747584));
#51455=CARTESIAN_POINT('Ctrl Pts',(53.5551516093398,27.6245897875243,19.3082026259016));
#51456=CARTESIAN_POINT('Ctrl Pts',(53.5430185078242,27.6374490744267,19.3070987776576));
#51457=CARTESIAN_POINT('Ctrl Pts',(53.5247527680116,27.6573310043498,19.3054018993267));
#51458=CARTESIAN_POINT('Ctrl Pts',(53.5184955729439,27.664238398794,19.3048141320337));
#51459=CARTESIAN_POINT('Ctrl Pts',(53.507671304719,27.6763570575715,19.3037858427187));
#51460=CARTESIAN_POINT('Ctrl Pts',(53.5030825168778,27.6815487796074,19.3033462353837));
#51461=CARTESIAN_POINT('Ctrl Pts',(53.4928062546393,27.6932980735253,19.30235336441));
#51462=CARTESIAN_POINT('Ctrl Pts',(53.4871343759873,27.6998690410253,19.3017994709368));
#51463=CARTESIAN_POINT('Ctrl Pts',(53.4719759445861,27.7176638447469,19.3003030478218));
#51464=CARTESIAN_POINT('Ctrl Pts',(53.4625703858617,27.7289556689449,19.299357259908));
#51465=CARTESIAN_POINT('Ctrl Pts',(53.4196913534228,27.7816063319796,19.2949637216228));
#51466=CARTESIAN_POINT('Ctrl Pts',(53.3877590479423,27.8241867561021,19.2914558178671));
#51467=CARTESIAN_POINT('Ctrl Pts',(53.254387391879,28.0176953151499,19.2756981544922));
#51468=CARTESIAN_POINT('Ctrl Pts',(53.1721650204346,28.1808006519824,19.2627870578473));
#51469=CARTESIAN_POINT('Ctrl Pts',(53.101464500245,28.3868973773681,19.2478623208375));
#51470=CARTESIAN_POINT('Ctrl Pts',(53.0906748889082,28.4213724860796,19.2454132675873));
#51471=CARTESIAN_POINT('Ctrl Pts',(53.0748413187565,28.47724429338,19.2415390980684));
#51472=CARTESIAN_POINT('Ctrl Pts',(53.069204631899,28.4984635416484,19.2400894000607));
#51473=CARTESIAN_POINT('Ctrl Pts',(53.0622027444243,28.5266922907014,19.2381931939999));
#51474=CARTESIAN_POINT('Ctrl Pts',(53.0605234414366,28.5336213192122,19.237730319033));
#51475=CARTESIAN_POINT('Ctrl Pts',(53.057822571403,28.5450323884993,19.2369724185095));
#51476=CARTESIAN_POINT('Ctrl Pts',(53.0567793003946,28.5495091506689,19.2366761876684));
#51477=CARTESIAN_POINT('Ctrl Pts',(53.054765453687,28.558287909771,19.2360975111195));
#51478=CARTESIAN_POINT('Ctrl Pts',(53.0537936571418,28.5625895721285,19.2358150007262));
#51479=CARTESIAN_POINT('Ctrl Pts',(53.0514341970133,28.5731972763926,19.2351208403134));
#51480=CARTESIAN_POINT('Ctrl Pts',(53.0500628552959,28.5795069704419,19.2347101089625));
#51481=CARTESIAN_POINT('Ctrl Pts',(53.0454495209873,28.6012414074214,19.2333024118755));
#51482=CARTESIAN_POINT('Ctrl Pts',(53.0423596243331,28.6166983094784,19.2323136008385));
#51483=CARTESIAN_POINT('Ctrl Pts',(53.0168140555292,28.7528647790546,19.2236976874981));
#51484=CARTESIAN_POINT('Ctrl Pts',(53.0053615296379,28.8753886883317,19.2165886790864));
#51485=CARTESIAN_POINT('Ctrl Pts',(53.0051277480755,29.1347064779513,19.2015306109203));
#51486=CARTESIAN_POINT('Ctrl Pts',(53.0190159974418,29.2708378576247,19.193601623165));
#51487=CARTESIAN_POINT('Ctrl Pts',(53.0466869987623,29.4044698773653,19.1852189598335));
#51488=CARTESIAN_POINT('',(53.0052500460737,29.0004287317334,19.0496800917662));
#51489=CARTESIAN_POINT('Ctrl Pts',(53.0466869973344,29.4044698704695,19.02544331564));
#51490=CARTESIAN_POINT('Ctrl Pts',(53.0455062711038,29.3987677698503,19.0257816004602));
#51491=CARTESIAN_POINT('Ctrl Pts',(53.0443504267425,29.3930600816379,19.0261199936269));
#51492=CARTESIAN_POINT('Ctrl Pts',(53.017991194005,29.2598997968382,19.0340108203298));
#51493=CARTESIAN_POINT('Ctrl Pts',(53.0052779626167,29.1303153687274,19.0416346866029));
#51494=CARTESIAN_POINT('Ctrl Pts',(53.0052500460737,29.0004287317334,19.0496800917662));
#51495=CARTESIAN_POINT('Ctrl Pts',(53.0052500457895,29.0004274077679,19.0496801737749));
#51496=CARTESIAN_POINT('Ctrl Pts',(53.0052478063791,28.9899758804868,19.0503275598346));
#51497=CARTESIAN_POINT('Ctrl Pts',(53.0053277084281,28.9795246123797,19.0509773538252));
#51498=CARTESIAN_POINT('Ctrl Pts',(53.005646711531,28.9589507726378,19.0522615537449));
#51499=CARTESIAN_POINT('Ctrl Pts',(53.0058807590315,28.9488284732444,19.0528957849875));
#51500=CARTESIAN_POINT('Ctrl Pts',(53.0064225229065,28.9312049216504,19.0540044101039));
#51501=CARTESIAN_POINT('Ctrl Pts',(53.0066955457967,28.9237027499559,19.0544777265378));
#51502=CARTESIAN_POINT('Ctrl Pts',(53.0073233780377,28.9087707888847,19.0554226340525));
#51503=CARTESIAN_POINT('Ctrl Pts',(53.0076774093588,28.9013410872481,19.0558941935145));
#51504=CARTESIAN_POINT('Ctrl Pts',(53.0084668548631,28.8865180927034,19.0568378711042));
#51505=CARTESIAN_POINT('Ctrl Pts',(53.0089019062289,28.8791248990796,19.0573099705662));
#51506=CARTESIAN_POINT('Ctrl Pts',(53.0101904368998,28.8591275111539,19.0585908677934));
#51507=CARTESIAN_POINT('Ctrl Pts',(53.0111224870436,28.8465288891049,19.0594020958668));
#51508=CARTESIAN_POINT('Ctrl Pts',(53.0151158014306,28.7987267486747,19.0624967101783));
#51509=CARTESIAN_POINT('Ctrl Pts',(53.0189924724166,28.7635996678762,19.064805201475));
#51510=CARTESIAN_POINT('Ctrl Pts',(53.0512359465118,28.5288222854712,19.0804753273298));
#51511=CARTESIAN_POINT('Ctrl Pts',(53.1088074172142,28.3343803605279,19.0947959733641));
#51512=CARTESIAN_POINT('Ctrl Pts',(53.2182450193238,28.1013929809828,19.1124492188469));
#51513=CARTESIAN_POINT('Ctrl Pts',(53.2440984053558,28.0518669834042,19.1162213608639));
#51514=CARTESIAN_POINT('Ctrl Pts',(53.2767556003028,27.9952378513681,19.1205052967201));
#51515=CARTESIAN_POINT('Ctrl Pts',(53.2815717483618,27.9870229079583,19.1211259900399));
#51516=CARTESIAN_POINT('Ctrl Pts',(53.2890686482566,27.9744427341258,19.1220749635518));
#51517=CARTESIAN_POINT('Ctrl Pts',(53.2917076163545,27.9700529482718,19.1224058115589));
#51518=CARTESIAN_POINT('Ctrl Pts',(53.2965943633647,27.9619945522091,19.1230125472206));
#51519=CARTESIAN_POINT('Ctrl Pts',(53.2988370946657,27.9583230622015,19.1232887417282));
#51520=CARTESIAN_POINT('Ctrl Pts',(53.3039234013095,27.9500567011087,19.1239100703869));
#51521=CARTESIAN_POINT('Ctrl Pts',(53.3067737738283,27.9454661180584,19.124254756769));
#51522=CARTESIAN_POINT('Ctrl Pts',(53.3152374736723,27.9319579490454,19.1252681414036));
#51523=CARTESIAN_POINT('Ctrl Pts',(53.3209029494058,27.9230730299676,19.1259335475991));
#51524=CARTESIAN_POINT('Ctrl Pts',(53.3701650094872,27.8471513641234,19.1316133711269));
#51525=CARTESIAN_POINT('Ctrl Pts',(53.4176913566518,27.7827389007307,19.1363924645113));
#51526=CARTESIAN_POINT('Ctrl Pts',(53.5493389577999,27.6251062556018,19.1484590061293));
#51527=CARTESIAN_POINT('Ctrl Pts',(53.6386096689264,27.5366588463793,19.1556175144074));
#51528=CARTESIAN_POINT('Ctrl Pts',(53.7760896828648,27.423988437114,19.1661359464649));
#51529=CARTESIAN_POINT('Ctrl Pts',(53.8178739184378,27.3924098024809,19.1692726681336));
#51530=CARTESIAN_POINT('Ctrl Pts',(53.8796357045458,27.3494439987075,19.1738644386051));
#51531=CARTESIAN_POINT('Ctrl Pts',(53.8986445545685,27.3366998503861,19.1752717878577));
#51532=CARTESIAN_POINT('Ctrl Pts',(53.9286244627288,27.3173396137033,19.1774849767904));
#51533=CARTESIAN_POINT('Ctrl Pts',(53.939447466235,27.3104971651932,19.178282676217));
#51534=CARTESIAN_POINT('Ctrl Pts',(53.9577414396238,27.2991765203366,19.179629298302));
#51535=CARTESIAN_POINT('Ctrl Pts',(53.9651773153871,27.2946421421735,19.1801761831571));
#51536=CARTESIAN_POINT('Ctrl Pts',(53.9797793797204,27.2858685082583,19.1812493362727));
#51537=CARTESIAN_POINT('Ctrl Pts',(53.9869428935655,27.2816251338136,19.1817754421767));
#51538=CARTESIAN_POINT('Ctrl Pts',(54.0006142827687,27.2736419586889,19.1827789156502));
#51539=CARTESIAN_POINT('Ctrl Pts',(54.007117125688,27.2698937911232,19.1832559713337));
#51540=CARTESIAN_POINT('Ctrl Pts',(54.0222097419011,27.2613076861743,19.1843626873562));
#51541=CARTESIAN_POINT('Ctrl Pts',(54.0308144788745,27.2564965813347,19.1849932907758));
#51542=CARTESIAN_POINT('Ctrl Pts',(54.053277963919,27.2441544129441,19.1866387681824));
#51543=CARTESIAN_POINT('Ctrl Pts',(54.0671907849444,27.2367237074331,19.1876571455239));
#51544=CARTESIAN_POINT('Ctrl Pts',(54.1976894877986,27.1690023063201,19.1972042738253));
#51545=CARTESIAN_POINT('Ctrl Pts',(54.3198496013681,27.1202025461571,19.20613706764));
#51546=CARTESIAN_POINT('Ctrl Pts',(54.5360915628439,27.0576734373542,19.2217713993886));
#51547=CARTESIAN_POINT('Ctrl Pts',(54.6280191536068,27.0379922921636,19.2283569245646));
#51548=CARTESIAN_POINT('Ctrl Pts',(54.7786178314443,27.0167187546396,19.2388011500169));
#51549=CARTESIAN_POINT('Ctrl Pts',(54.8365784782753,27.0111034844638,19.2427380750565));
#51550=CARTESIAN_POINT('Ctrl Pts',(54.9043078099967,27.0075234009131,19.2471835425869));
#51551=CARTESIAN_POINT('Ctrl Pts',(54.9139122676135,27.0070853243724,19.2478103027406));
#51552=CARTESIAN_POINT('Ctrl Pts',(54.9286573415978,27.0065195708625,19.2487665663839));
#51553=CARTESIAN_POINT('Ctrl Pts',(54.9337957516041,27.006342307418,19.2490986981816));
#51554=CARTESIAN_POINT('Ctrl Pts',(54.9432340627601,27.006053237581,19.2497066542654));
#51555=CARTESIAN_POINT('Ctrl Pts',(54.9475336287227,27.0059354715635,19.2499827943348));
#51556=CARTESIAN_POINT('Ctrl Pts',(54.9572121466435,27.0057017006123,19.2506025922383));
#51557=CARTESIAN_POINT('Ctrl Pts',(54.9625911975236,27.0055935493339,19.2509458124359));
#51558=CARTESIAN_POINT('Ctrl Pts',(54.9764053822487,27.0053717091144,19.2518242021446));
#51559=CARTESIAN_POINT('Ctrl Pts',(54.9848410181764,27.0052897614051,19.2523576717401));
#51560=CARTESIAN_POINT('Ctrl Pts',(55.0365749669107,27.0051154014859,19.2556128088198));
#51561=CARTESIAN_POINT('Ctrl Pts',(55.0798697677149,27.0063792411834,19.2582660652183));
#51562=CARTESIAN_POINT('Ctrl Pts',(55.1294713727338,27.0094459134535,19.2612590704408));
#51563=CARTESIAN_POINT('Ctrl Pts',(55.1358483534701,27.0098709503743,19.2616429725774));
#51564=CARTESIAN_POINT('Ctrl Pts',(55.1570280403962,27.0113848891505,19.2629153711276));
#51565=CARTESIAN_POINT('Ctrl Pts',(55.171820842013,27.012608373066,19.2637997756829));
#51566=CARTESIAN_POINT('Ctrl Pts',(55.30926044153,27.0255217837657,19.2719876816518));
#51567=CARTESIAN_POINT('Ctrl Pts',(55.4305939170739,27.048385905668,19.2790167449683));
#51568=CARTESIAN_POINT('Ctrl Pts',(55.6428903483604,27.1091673467042,19.2919737450275));
#51569=CARTESIAN_POINT('Ctrl Pts',(55.7346238256166,27.1428838728818,19.297806546523));
#51570=CARTESIAN_POINT('Ctrl Pts',(55.8386134151468,27.1900193571786,19.3049001245724));
#51571=CARTESIAN_POINT('Ctrl Pts',(55.8536262954095,27.1970511628516,19.305936209793));
#51572=CARTESIAN_POINT('Ctrl Pts',(55.8767308645133,27.2082262563654,19.307550196967));
#51573=CARTESIAN_POINT('Ctrl Pts',(55.8848850365041,27.2122392148411,19.3081236134962));
#51574=CARTESIAN_POINT('Ctrl Pts',(55.8991906174989,27.2194013508477,19.3091364483572));
#51575=CARTESIAN_POINT('Ctrl Pts',(55.9053536589434,27.2225270561144,19.3095750456032));
#51576=CARTESIAN_POINT('Ctrl Pts',(55.9193854779955,27.2297354743785,19.3105788534202));
#51577=CARTESIAN_POINT('Ctrl Pts',(55.9272434869398,27.2338387220894,19.3111447752997));
#51578=CARTESIAN_POINT('Ctrl Pts',(55.9484446365664,27.2450898988362,19.3126820498467));
#51579=CARTESIAN_POINT('Ctrl Pts',(55.9617339759139,27.2523374380213,19.3136568901226));
#51580=CARTESIAN_POINT('Ctrl Pts',(56.0276775557568,27.2892806607301,19.3185516916453));
#51581=CARTESIAN_POINT('Ctrl Pts',(56.0790404227824,27.3212051021236,19.3225504592779));
#51582=CARTESIAN_POINT('Ctrl Pts',(56.2724337871031,27.4539530841267,19.3383555247969));
#51583=CARTESIAN_POINT('Ctrl Pts',(56.4024699620655,27.5708697809595,19.3507155619692));
#51584=CARTESIAN_POINT('Ctrl Pts',(56.5388225049768,27.7302271729996,19.3650757897771));
#51585=CARTESIAN_POINT('Ctrl Pts',(56.5612644131866,27.7579245328783,19.3674916203489));
#51586=CARTESIAN_POINT('Ctrl Pts',(56.5961853514039,27.8034663573516,19.3713193255936));
#51587=CARTESIAN_POINT('Ctrl Pts',(56.6091349880337,27.8209388830386,19.3727551082474));
#51588=CARTESIAN_POINT('Ctrl Pts',(56.6259332256596,27.8443966162524,19.3746360710949));
#51589=CARTESIAN_POINT('Ctrl Pts',(56.6300387172647,27.8501948779358,19.3750972970341));
#51590=CARTESIAN_POINT('Ctrl Pts',(56.6367462392396,27.8597761668842,19.3758531977741));
#51591=CARTESIAN_POINT('Ctrl Pts',(56.6393663007456,27.8635464046931,19.3761490657136));
#51592=CARTESIAN_POINT('Ctrl Pts',(56.6444796981123,27.8709590053242,19.376727623174));
#51593=CARTESIAN_POINT('Ctrl Pts',(56.6469739934054,27.874600643861,19.3770103741043));
#51594=CARTESIAN_POINT('Ctrl Pts',(56.6530983886751,27.8836061502658,19.3777060290041));
#51595=CARTESIAN_POINT('Ctrl Pts',(56.6567145316131,27.8889795348928,19.378118005205));
#51596=CARTESIAN_POINT('Ctrl Pts',(56.6691067907516,27.9075887743114,19.379534438761));
#51597=CARTESIAN_POINT('Ctrl Pts',(56.6777512406203,27.9209121553058,19.380530605369));
#51598=CARTESIAN_POINT('Ctrl Pts',(56.7496226740914,28.0346369361543,19.388895596884));
#51599=CARTESIAN_POINT('Ctrl Pts',(56.8039431155786,28.1404057897559,19.3957817210386));
#51600=CARTESIAN_POINT('Ctrl Pts',(56.9064822507263,28.3932675341782,19.4116281495014));
#51601=CARTESIAN_POINT('Ctrl Pts',(56.9476544124801,28.5423608936478,19.4205717857586));
#51602=CARTESIAN_POINT('Ctrl Pts',(56.9739988982319,28.7124605494592,19.4312478597554));
#51603=CARTESIAN_POINT('Ctrl Pts',(56.976509438149,28.7302575414514,19.4323697442541));
#51604=CARTESIAN_POINT('Ctrl Pts',(56.9799637947506,28.7573913943248,19.434088636665));
#51605=CARTESIAN_POINT('Ctrl Pts',(56.9810828221314,28.7667053127298,19.4346801652282));
#51606=CARTESIAN_POINT('Ctrl Pts',(56.9829147939246,28.7829180338033,19.4357125923112));
#51607=CARTESIAN_POINT('Ctrl Pts',(56.9836575393697,28.7898133578423,19.4361525516411));
#51608=CARTESIAN_POINT('Ctrl Pts',(56.985244598104,28.8053052119858,19.4371430218139));
#51609=CARTESIAN_POINT('Ctrl Pts',(56.9860690567932,28.8139035933078,19.4376941433216));
#51610=CARTESIAN_POINT('Ctrl Pts',(56.9881280499444,28.8369517354825,19.4391752750005));
#51611=CARTESIAN_POINT('Ctrl Pts',(56.989260874199,28.8514098401416,19.4401084295451));
#51612=CARTESIAN_POINT('Ctrl Pts',(56.9936758689586,28.9169242766799,19.4443559737099));
#51613=CARTESIAN_POINT('Ctrl Pts',(56.9951504502837,28.9680790735397,19.4477257384473));
#51614=CARTESIAN_POINT('Ctrl Pts',(56.9928830431827,29.2032638859485,19.4634723888697));
#51615=CARTESIAN_POINT('Ctrl Pts',(56.9656455395308,29.3861577437401,19.476542492339));
#51616=CARTESIAN_POINT('Ctrl Pts',(56.898531365494,29.6144227532047,19.4928417381771));
#51617=CARTESIAN_POINT('Ctrl Pts',(56.8812230855057,29.6655355009283,19.4964814148573));
#51618=CARTESIAN_POINT('Ctrl Pts',(56.858473142986,29.7247029214556,19.5006349386809));
#51619=CARTESIAN_POINT('Ctrl Pts',(56.8550212640473,29.7334936031845,19.5012504448394));
#51620=CARTESIAN_POINT('Ctrl Pts',(56.8496073561582,29.7469981611493,19.5021931808433));
#51621=CARTESIAN_POINT('Ctrl Pts',(56.8476894991173,29.751729433355,19.5025229272637));
#51622=CARTESIAN_POINT('Ctrl Pts',(56.8441215103822,29.7604353602534,19.503128625961));
#51623=CARTESIAN_POINT('Ctrl Pts',(56.8424766876577,29.7644120212646,19.5034048774));
#51624=CARTESIAN_POINT('Ctrl Pts',(56.8387295949393,29.7733889445849,19.5040275655343));
#51625=CARTESIAN_POINT('Ctrl Pts',(56.8366197949205,29.7783859669098,19.5043735455382));
#51626=CARTESIAN_POINT('Ctrl Pts',(56.8303135453714,29.7931538089394,19.5053943080593));
#51627=CARTESIAN_POINT('Ctrl Pts',(56.8260592416577,29.8028999294047,19.5060657266824));
#51628=CARTESIAN_POINT('Ctrl Pts',(56.7844338864745,29.8962163643188,19.5124771292406));
#51629=CARTESIAN_POINT('Ctrl Pts',(56.7414243466232,29.9771661884607,19.5179077140421));
#51630=CARTESIAN_POINT('Ctrl Pts',(56.6806591299543,30.0746892586491,19.5246268651176));
#51631=CARTESIAN_POINT('Ctrl Pts',(56.6679718336253,30.0942769747882,19.5259857752489));
#51632=CARTESIAN_POINT('Ctrl Pts',(56.5914688947928,30.2079656979871,19.5339527979515));
#51633=CARTESIAN_POINT('Ctrl Pts',(56.5200497700436,30.2966885727577,19.5405108062158));
#51634=CARTESIAN_POINT('Ctrl Pts',(56.4012679012639,30.4208650354141,19.5508075993651));
#51635=CARTESIAN_POINT('Ctrl Pts',(56.3592563488577,30.4611058819626,19.5543506200421));
#51636=CARTESIAN_POINT('Ctrl Pts',(56.3046436064739,30.5090205872882,19.5588767232874));
#51637=CARTESIAN_POINT('Ctrl Pts',(56.2936333847748,30.5184698617707,19.5597853243805));
#51638=CARTESIAN_POINT('Ctrl Pts',(56.2759043600714,30.5333526222113,19.5612427786714));
#51639=CARTESIAN_POINT('Ctrl Pts',(56.2692515036537,30.5388641320096,19.5617884562186));
#51640=CARTESIAN_POINT('Ctrl Pts',(56.2565974323395,30.5492094218162,19.5628241532649));
#51641=CARTESIAN_POINT('Ctrl Pts',(56.2506035860601,30.5540519963713,19.5633138070197));
#51642=CARTESIAN_POINT('Ctrl Pts',(56.2369591711558,30.5649455951951,19.5644264591327));
#51643=CARTESIAN_POINT('Ctrl Pts',(56.229292019185,30.5709754399873,19.5650502815214));
#51644=CARTESIAN_POINT('Ctrl Pts',(56.2093855131378,30.5863959862849,19.5666664987351));
#51645=CARTESIAN_POINT('Ctrl Pts',(56.1970810753765,30.5957012319404,19.5676621948154));
#51646=CARTESIAN_POINT('Ctrl Pts',(56.1081788587082,30.6613266680748,19.5748342900133));
#51647=CARTESIAN_POINT('Ctrl Pts',(56.0277600635917,30.7122415821892,19.5812151325597));
#51648=CARTESIAN_POINT('Ctrl Pts',(55.7930011073831,30.8383604519086,19.599510613008));
#51649=CARTESIAN_POINT('Ctrl Pts',(55.6321523185078,30.8996846582156,19.6117288699982));
#51650=CARTESIAN_POINT('Ctrl Pts',(55.4438911774468,30.9448597902957,19.6246481001136));
#51651=CARTESIAN_POINT('Ctrl Pts',(55.4222493014826,30.949672948775,19.6261122879272));
#51652=CARTESIAN_POINT('Ctrl Pts',(55.3935210755427,30.9555612809892,19.6280243476571));
#51653=CARTESIAN_POINT('Ctrl Pts',(55.3865037078211,30.9569603082822,19.6284889240765));
#51654=CARTESIAN_POINT('Ctrl Pts',(55.374960575581,30.9591971086414,19.6292488880222));
#51655=CARTESIAN_POINT('Ctrl Pts',(55.3704392422043,30.960057017698,19.6295454934098));
#51656=CARTESIAN_POINT('Ctrl Pts',(55.361583596545,30.9617095296753,19.6301242978393));
#51657=CARTESIAN_POINT('Ctrl Pts',(55.3572495821939,30.9625034299789,19.6304065649286));
#51658=CARTESIAN_POINT('Ctrl Pts',(55.3465778161003,30.9644217496476,19.6310992073881));
#51659=CARTESIAN_POINT('Ctrl Pts',(55.3402371140098,30.9655298781963,19.6315086733137));
#51660=CARTESIAN_POINT('Ctrl Pts',(55.3184714623735,30.9692252556808,19.6329074843549));
#51661=CARTESIAN_POINT('Ctrl Pts',(55.3030210531202,30.9716618515259,19.6338888121188));
#51662=CARTESIAN_POINT('Ctrl Pts',(55.163667429994,30.991961677723,19.6426483055549));
#51663=CARTESIAN_POINT('Ctrl Pts',(55.0383501666605,30.9983083678952,19.6498868154105));
#51664=CARTESIAN_POINT('Ctrl Pts',(54.7647391119377,30.9863980947121,19.6657897114707));
#51665=CARTESIAN_POINT('Ctrl Pts',(54.6174369152007,30.9633550387138,19.6744421469481));
#51666=CARTESIAN_POINT('Ctrl Pts',(54.4571249606752,30.9195371323278,19.6847551310954));
#51667=CARTESIAN_POINT('Ctrl Pts',(54.4402433051979,30.9146823555533,19.6858519775186));
#51668=CARTESIAN_POINT('Ctrl Pts',(54.4145287672803,30.9069183048982,19.6875403037169));
#51669=CARTESIAN_POINT('Ctrl Pts',(54.4056481769327,30.9041690816794,19.6881266036671));
#51670=CARTESIAN_POINT('Ctrl Pts',(54.3901848252909,30.8992632768257,19.6891532873395));
#51671=CARTESIAN_POINT('Ctrl Pts',(54.3835934271708,30.8971342801739,19.6895927659308));
#51672=CARTESIAN_POINT('Ctrl Pts',(54.3687508736513,30.8922546735312,19.6905866200501));
#51673=CARTESIAN_POINT('Ctrl Pts',(54.3605063923939,30.8894843558286,19.6911416331092));
#51674=CARTESIAN_POINT('Ctrl Pts',(54.3383068928586,30.8818629247589,19.6926442405079));
#51675=CARTESIAN_POINT('Ctrl Pts',(54.3243874363688,30.8769106212394,19.6935951396701));
#51676=CARTESIAN_POINT('Ctrl Pts',(54.2598228529578,30.8531283837888,19.6980475884345));
#51677=CARTESIAN_POINT('Ctrl Pts',(54.2099052973631,30.8324018280796,19.701611272545));
#51678=CARTESIAN_POINT('Ctrl Pts',(53.9967550176066,30.7335688856311,19.7173734418554));
#51679=CARTESIAN_POINT('Ctrl Pts',(53.8437413303386,30.6354847500644,19.73022054465));
#51680=CARTESIAN_POINT('Ctrl Pts',(53.6786330371633,30.4947633314687,19.7450798477257));
#51681=CARTESIAN_POINT('Ctrl Pts',(53.6518244489224,30.4706294774457,19.7475252213904));
#51682=CARTESIAN_POINT('Ctrl Pts',(53.6097890063487,30.4306718236124,19.751394249132));
#51683=CARTESIAN_POINT('Ctrl Pts',(53.5941439532769,30.4153011499753,19.7528424099391));
#51684=CARTESIAN_POINT('Ctrl Pts',(53.5737541727934,30.3945971434197,19.7547369327676));
#51685=CARTESIAN_POINT('Ctrl Pts',(53.5687806851537,30.389492579533,19.7551996260815));
#51686=CARTESIAN_POINT('Ctrl Pts',(53.560644908272,30.3810523545494,19.7559573061627));
#51687=CARTESIAN_POINT('Ctrl Pts',(53.5574666513218,30.3777322762714,19.7562534968753));
#51688=CARTESIAN_POINT('Ctrl Pts',(53.5512610207255,30.3712047201151,19.7568321596495));
#51689=CARTESIAN_POINT('Ctrl Pts',(53.5482327719927,30.3679981472172,19.757114696037));
#51690=CARTESIAN_POINT('Ctrl Pts',(53.540795985085,30.3600709261856,19.7578090190553));
#51691=CARTESIAN_POINT('Ctrl Pts',(53.5363996437534,30.3553388068496,19.7582198860257));
#51692=CARTESIAN_POINT('Ctrl Pts',(53.5213457806812,30.3389765122593,19.7596285362708));
#51693=CARTESIAN_POINT('Ctrl Pts',(53.5108029584606,30.3272409760407,19.7606181500471));
#51694=CARTESIAN_POINT('Ctrl Pts',(53.4200400313021,30.2237667285734,19.7691778105887));
#51695=CARTESIAN_POINT('Ctrl Pts',(53.3482329652704,30.1249676973428,19.7762376092627));
#51696=CARTESIAN_POINT('Ctrl Pts',(53.2327174921941,29.9308854704085,19.7893529279146));
#51697=CARTESIAN_POINT('Ctrl Pts',(53.1866143829717,29.8375355534069,19.7953840508298));
#51698=CARTESIAN_POINT('Ctrl Pts',(53.1347953712536,29.7080271062106,19.8037674016661));
#51699=CARTESIAN_POINT('Ctrl Pts',(53.1224773587453,29.6746845234481,19.8059259747632));
#51700=CARTESIAN_POINT('Ctrl Pts',(53.10285333501,29.6168579904176,19.809682730715));
#51701=CARTESIAN_POINT('Ctrl Pts',(53.0951147381528,29.5925295742279,19.8112671094947));
#51702=CARTESIAN_POINT('Ctrl Pts',(53.0847723662567,29.557715984457,19.8135427581142));
#51703=CARTESIAN_POINT('Ctrl Pts',(53.081783366705,29.5473471922249,19.8142215772134));
#51704=CARTESIAN_POINT('Ctrl Pts',(53.0767635230396,29.5293871547827,19.8153993997752));
#51705=CARTESIAN_POINT('Ctrl Pts',(53.0746931147149,29.5218071488323,19.8158971170494));
#51706=CARTESIAN_POINT('Ctrl Pts',(53.0708062509204,29.5072387760593,19.816854972627));
#51707=CARTESIAN_POINT('Ctrl Pts',(53.0689828450676,29.5002523788463,19.8173148786383));
#51708=CARTESIAN_POINT('Ctrl Pts',(53.0647792960958,29.4837809620813,19.8184005529486));
#51709=CARTESIAN_POINT('Ctrl Pts',(53.0624309089407,29.4742881021688,19.8190273272267));
#51710=CARTESIAN_POINT('Ctrl Pts',(53.0553526387268,29.4447455022966,19.8209814332942));
#51711=CARTESIAN_POINT('Ctrl Pts',(53.0508636462377,29.4246402295994,19.8223163538649));
#51712=CARTESIAN_POINT('Ctrl Pts',(53.0466869979816,29.4044698735951,19.8236610414577));
#51713=CARTESIAN_POINT('Origin',(55.,29.,3.45145488139523));
#51714=CARTESIAN_POINT('',(53.0466870286012,29.4044700214667,20.7832412988479));
#51715=CARTESIAN_POINT('',(53.0466869978243,29.4044698728352,20.6265291208673));
#51716=CARTESIAN_POINT('',(53.0466869980082,29.4044698737233,3.45145488139523));
#51717=CARTESIAN_POINT('',(53.0052502012793,29.0008961046522,20.0080399322459));
#51718=CARTESIAN_POINT('Ctrl Pts',(53.0466870286012,29.4044700214667,20.7832412988479));
#51719=CARTESIAN_POINT('Ctrl Pts',(53.0553314951071,29.4462168695904,20.7802703107498));
#51720=CARTESIAN_POINT('Ctrl Pts',(53.0653153162778,29.4876915346209,20.7773015864245));
#51721=CARTESIAN_POINT('Ctrl Pts',(53.0950104017614,29.5956936661242,20.7695663386943));
#51722=CARTESIAN_POINT('Ctrl Pts',(53.1168708710286,29.6615611137937,20.7648434349152));
#51723=CARTESIAN_POINT('Ctrl Pts',(53.1458993127313,29.7358301089969,20.7596082951248));
#51724=CARTESIAN_POINT('Ctrl Pts',(53.1497535331037,29.7454685309452,20.7589307160286));
#51725=CARTESIAN_POINT('Ctrl Pts',(53.1557155242807,29.7600468202737,20.7579091115319));
#51726=CARTESIAN_POINT('Ctrl Pts',(53.1577682242515,29.7650088119996,20.7575619638558));
#51727=CARTESIAN_POINT('Ctrl Pts',(53.1615010351062,29.7739299807685,20.7569389415378));
#51728=CARTESIAN_POINT('Ctrl Pts',(53.1631739260645,29.7778920453244,20.7566626487112));
#51729=CARTESIAN_POINT('Ctrl Pts',(53.1668783023558,29.7865868855655,20.7560572070357));
#51730=CARTESIAN_POINT('Ctrl Pts',(53.1689153040983,29.7913172087005,20.7557283945056));
#51731=CARTESIAN_POINT('Ctrl Pts',(53.1748238748398,29.8048931020259,20.754786207604));
#51732=CARTESIAN_POINT('Ctrl Pts',(53.1787414423642,29.8137186667577,20.7541755322148));
#51733=CARTESIAN_POINT('Ctrl Pts',(53.2071827159566,29.8765571935635,20.7498381965224));
#51734=CARTESIAN_POINT('Ctrl Pts',(53.2340434615237,29.9294865745365,20.7462412908334));
#51735=CARTESIAN_POINT('Ctrl Pts',(53.3090388818845,30.062239715722,20.7371702423419));
#51736=CARTESIAN_POINT('Ctrl Pts',(53.3604769902493,30.1400301279895,20.7318021602038));
#51737=CARTESIAN_POINT('Ctrl Pts',(53.496775687192,30.3177469759902,20.7187799579456));
#51738=CARTESIAN_POINT('Ctrl Pts',(53.5863923204465,30.4134522449883,20.7110942110001));
#51739=CARTESIAN_POINT('Ctrl Pts',(53.6965754071445,30.510086221292,20.7019991799708));
#51740=CARTESIAN_POINT('Ctrl Pts',(53.7085495855829,30.5203393930225,20.7010153871055));
#51741=CARTESIAN_POINT('Ctrl Pts',(53.7282055338175,30.5367704888667,20.6994071440083));
#51742=CARTESIAN_POINT('Ctrl Pts',(53.7358139323089,30.5430354112414,20.6987862199059));
#51743=CARTESIAN_POINT('Ctrl Pts',(53.7494616737045,30.5541045672664,20.6976750756369));
#51744=CARTESIAN_POINT('Ctrl Pts',(53.7554830965794,30.558930654621,20.6971857424836));
#51745=CARTESIAN_POINT('Ctrl Pts',(53.7682585937351,30.569048849743,20.6961493584569));
#51746=CARTESIAN_POINT('Ctrl Pts',(53.7750190987135,30.5743325482571,20.6956019887293));
#51747=CARTESIAN_POINT('Ctrl Pts',(53.7930901959422,30.5882692114758,20.6941415276353));
#51748=CARTESIAN_POINT('Ctrl Pts',(53.8044595544307,30.5968448230567,20.6932254432017));
#51749=CARTESIAN_POINT('Ctrl Pts',(53.8599992043105,30.6378113127696,20.6887627472052));
#51750=CARTESIAN_POINT('Ctrl Pts',(53.9053954309941,30.6684926105381,20.6851517100277));
#51751=CARTESIAN_POINT('Ctrl Pts',(54.1259058107122,30.8046507258535,20.6677680425098));
#51752=CARTESIAN_POINT('Ctrl Pts',(54.3152498351048,30.8846483702919,20.6531283277326));
#51753=CARTESIAN_POINT('Ctrl Pts',(54.5446692825354,30.9423542430837,20.6371711979269));
#51754=CARTESIAN_POINT('Ctrl Pts',(54.5761097422814,30.9494572059151,20.635024938875));
#51755=CARTESIAN_POINT('Ctrl Pts',(54.6159642829957,30.957451147703,20.632366481615));
#51756=CARTESIAN_POINT('Ctrl Pts',(54.6242286029815,30.9590544379303,20.6318185684144));
#51757=CARTESIAN_POINT('Ctrl Pts',(54.6373491715042,30.9615137648302,20.6309542625789));
#51758=CARTESIAN_POINT('Ctrl Pts',(54.6421987592813,30.9624041750971,20.6306360038038));
#51759=CARTESIAN_POINT('Ctrl Pts',(54.6508822938563,30.9639652587919,20.6300683513419));
#51760=CARTESIAN_POINT('Ctrl Pts',(54.6547148745724,30.9646426883762,20.6298185869035));
#51761=CARTESIAN_POINT('Ctrl Pts',(54.6639064328017,30.9662396190081,20.6292214166979));
#51762=CARTESIAN_POINT('Ctrl Pts',(54.6692672084739,30.9671484304837,20.6288746148961));
#51763=CARTESIAN_POINT('Ctrl Pts',(54.6855359201763,30.9698380788148,20.627826468042));
#51764=CARTESIAN_POINT('Ctrl Pts',(54.6964552180826,30.9715502257612,20.6271288450403));
#51765=CARTESIAN_POINT('Ctrl Pts',(54.7217669673691,30.9753038322458,20.6255241146606));
#51766=CARTESIAN_POINT('Ctrl Pts',(54.7361687893421,30.9772789304423,20.6246203189618));
#51767=CARTESIAN_POINT('Ctrl Pts',(54.7856186606282,30.983510675758,20.6215448180797));
#51768=CARTESIAN_POINT('Ctrl Pts',(54.8207590562504,30.9869944471541,20.6194069284775));
#51769=CARTESIAN_POINT('Ctrl Pts',(55.0246767137982,31.001756207901,20.6071822595322));
#51770=CARTESIAN_POINT('Ctrl Pts',(55.1942504915554,30.9924634424106,20.5976747691155));
#51771=CARTESIAN_POINT('Ctrl Pts',(55.4248483668661,30.9500757014966,20.5836991240699));
#51772=CARTESIAN_POINT('Ctrl Pts',(55.488446111065,30.9351254394238,20.5797381323352));
#51773=CARTESIAN_POINT('Ctrl Pts',(55.5660636393772,30.9128091818571,20.5747145329519));
#51774=CARTESIAN_POINT('Ctrl Pts',(55.5808846553037,30.9083605545498,20.5737466626839));
#51775=CARTESIAN_POINT('Ctrl Pts',(55.604185975882,30.9010699160559,20.5722106995769));
#51776=CARTESIAN_POINT('Ctrl Pts',(55.6127016920449,30.8983424747837,20.5716463302622));
#51777=CARTESIAN_POINT('Ctrl Pts',(55.6284904987294,30.8931682800392,20.5705941664712));
#51778=CARTESIAN_POINT('Ctrl Pts',(55.6357683914033,30.8907366271787,20.5701068735415));
#51779=CARTESIAN_POINT('Ctrl Pts',(55.651862591564,30.8852558836661,20.5690241029813));
#51780=CARTESIAN_POINT('Ctrl Pts',(55.6606718628811,30.8821868318323,20.5684279787952));
#51781=CARTESIAN_POINT('Ctrl Pts',(55.6861515672887,30.8731090713802,20.5666935295342));
#51782=CARTESIAN_POINT('Ctrl Pts',(55.7027635244819,30.8669399995253,20.5655499462101));
#51783=CARTESIAN_POINT('Ctrl Pts',(55.7400854344698,30.8525113130348,20.5629509862148));
#51784=CARTESIAN_POINT('Ctrl Pts',(55.7607432495935,30.8441242522601,20.5614915257487));
#51785=CARTESIAN_POINT('Ctrl Pts',(55.8276393450442,30.8156491832557,20.5566956562784));
#51786=CARTESIAN_POINT('Ctrl Pts',(55.8732546281813,30.7941556523979,20.5533147857872));
#51787=CARTESIAN_POINT('Ctrl Pts',(56.0255327576674,30.7152199304328,20.5416547324534));
#51788=CARTESIAN_POINT('Ctrl Pts',(56.1277551988651,30.6498062428275,20.5331628660581));
#51789=CARTESIAN_POINT('Ctrl Pts',(56.2923311389045,30.5220129383272,20.5186911413622));
#51790=CARTESIAN_POINT('Ctrl Pts',(56.357680462187,30.4640186122098,20.5126937591709));
#51791=CARTESIAN_POINT('Ctrl Pts',(56.4264891700111,30.3943704480612,20.5062632836647));
#51792=CARTESIAN_POINT('Ctrl Pts',(56.4338911495428,30.3867575424905,20.5055699673716));
#51793=CARTESIAN_POINT('Ctrl Pts',(56.4449797860629,30.3751692127862,20.5045294486039));
#51794=CARTESIAN_POINT('Ctrl Pts',(56.4487114662739,30.3712374101826,20.5041789526781));
#51795=CARTESIAN_POINT('Ctrl Pts',(56.4553767472369,30.3641571038,20.5035524092397));
#51796=CARTESIAN_POINT('Ctrl Pts',(56.4583162184178,30.3610142866377,20.5032759210915));
#51797=CARTESIAN_POINT('Ctrl Pts',(56.4647225991806,30.3541201424562,20.502672955222));
#51798=CARTESIAN_POINT('Ctrl Pts',(56.4681852738671,30.3503650083425,20.5023467946637));
#51799=CARTESIAN_POINT('Ctrl Pts',(56.4780174229222,30.3396199042582,20.5014197993077));
#51800=CARTESIAN_POINT('Ctrl Pts',(56.4843517692538,30.3325977726942,20.5008215298104));
#51801=CARTESIAN_POINT('Ctrl Pts',(56.5266792026148,30.2849981209674,20.4968144667943));
#51802=CARTESIAN_POINT('Ctrl Pts',(56.5610577346746,30.2430082293071,20.4935139387138));
#51803=CARTESIAN_POINT('Ctrl Pts',(56.7066642949965,30.0495784551256,20.4790562548759));
#51804=CARTESIAN_POINT('Ctrl Pts',(56.7978781162392,29.8842852165941,20.4685519342679));
#51805=CARTESIAN_POINT('Ctrl Pts',(56.8815651996263,29.6640886648209,20.454341185917));
#51806=CARTESIAN_POINT('Ctrl Pts',(56.8969008286751,29.6189249159408,20.4514222693561));
#51807=CARTESIAN_POINT('Ctrl Pts',(56.9146688118634,29.5597062413393,20.4475686562545));
#51808=CARTESIAN_POINT('Ctrl Pts',(56.9185904085718,29.5461122262323,20.4466823114557));
#51809=CARTESIAN_POINT('Ctrl Pts',(56.9246519853572,29.5242285484562,20.4452522177104));
#51810=CARTESIAN_POINT('Ctrl Pts',(56.926883830507,29.5159646652715,20.4447114357689));
#51811=CARTESIAN_POINT('Ctrl Pts',(56.9310275000814,29.5002199236002,20.4436795973319));
#51812=CARTESIAN_POINT('Ctrl Pts',(56.9329492186225,29.4927418122427,20.4431888691491));
#51813=CARTESIAN_POINT('Ctrl Pts',(56.9372339952756,29.4756573086641,20.4420661899594));
#51814=CARTESIAN_POINT('Ctrl Pts',(56.9395690882497,29.4660441758567,20.4414333571717));
#51815=CARTESIAN_POINT('Ctrl Pts',(56.9465312990696,29.4364231710655,20.4394797481006));
#51816=CARTESIAN_POINT('Ctrl Pts',(56.9509209130551,29.4163614073564,20.4381514737828));
#51817=CARTESIAN_POINT('Ctrl Pts',(56.9603362306117,29.3699069145034,20.4350629378972));
#51818=CARTESIAN_POINT('Ctrl Pts',(56.9651399245771,29.3434737626215,20.4332960253404));
#51819=CARTESIAN_POINT('Ctrl Pts',(56.9799533083057,29.2514297393085,20.4271092710799));
#51820=CARTESIAN_POINT('Ctrl Pts',(56.9872209839308,29.1854273920682,20.4226113117506));
#51821=CARTESIAN_POINT('Ctrl Pts',(56.996697378033,29.0271161180425,20.4117070400412));
#51822=CARTESIAN_POINT('Ctrl Pts',(56.9958155750849,28.9347726036196,20.4052501342461));
#51823=CARTESIAN_POINT('Ctrl Pts',(56.9813754053983,28.7520763259508,20.3925110992425));
#51824=CARTESIAN_POINT('Ctrl Pts',(56.9679977404678,28.6619120677663,20.386243584732));
#51825=CARTESIAN_POINT('Ctrl Pts',(56.9462284939126,28.5625811111966,20.3795644616586));
#51826=CARTESIAN_POINT('Ctrl Pts',(56.9438690068451,28.5522121809567,20.3788700976218));
#51827=CARTESIAN_POINT('Ctrl Pts',(56.9401809102486,28.5365833214134,20.3778283210176));
#51828=CARTESIAN_POINT('Ctrl Pts',(56.9389136221333,28.5313093236825,20.3774776034586));
#51829=CARTESIAN_POINT('Ctrl Pts',(56.9366023132329,28.5218603109288,20.37685082523));
#51830=CARTESIAN_POINT('Ctrl Pts',(56.9355662838206,28.5176834608775,20.3765743224425));
#51831=CARTESIAN_POINT('Ctrl Pts',(56.9332716411066,28.508558867405,20.3759715127447));
#51832=CARTESIAN_POINT('Ctrl Pts',(56.9320075501746,28.5036125982868,20.3756455217654));
#51833=CARTESIAN_POINT('Ctrl Pts',(56.9283509724295,28.4895303359028,20.3747194945795));
#51834=CARTESIAN_POINT('Ctrl Pts',(56.9259125379672,28.4804062594372,20.3741220152618));
#51835=CARTESIAN_POINT('Ctrl Pts',(56.9091127571718,28.419288739278,20.3701345279476));
#51836=CARTESIAN_POINT('Ctrl Pts',(56.8927109788618,28.3678739271519,20.3668515758046));
#51837=CARTESIAN_POINT('Ctrl Pts',(56.8112374451797,28.1442398491353,20.3526351668634));
#51838=CARTESIAN_POINT('Ctrl Pts',(56.724599330744,27.9808476377776,20.3423328029556));
#51839=CARTESIAN_POINT('Ctrl Pts',(56.586838811969,27.7902136253842,20.3281798200685));
#51840=CARTESIAN_POINT('Ctrl Pts',(56.555319642321,27.7499517490247,20.3250565253297));
#51841=CARTESIAN_POINT('Ctrl Pts',(56.5129218618315,27.6998826187298,20.3209691768479));
#51842=CARTESIAN_POINT('Ctrl Pts',(56.503432538321,27.688920921385,20.3200612300968));
#51843=CARTESIAN_POINT('Ctrl Pts',(56.4881009669051,27.6715958174595,20.3186045799908));
#51844=CARTESIAN_POINT('Ctrl Pts',(56.4823353007905,27.6651650992916,20.318059046068));
#51845=CARTESIAN_POINT('Ctrl Pts',(56.4718649232624,27.6536384922174,20.3170723004125));
#51846=CARTESIAN_POINT('Ctrl Pts',(56.4671750285736,27.6485292842532,20.3166317151307));
#51847=CARTESIAN_POINT('Ctrl Pts',(56.4560781486309,27.6365660950298,20.315592439666));
#51848=CARTESIAN_POINT('Ctrl Pts',(56.4496493056796,27.629732699891,20.3149928263584));
#51849=CARTESIAN_POINT('Ctrl Pts',(56.4307609273641,27.6099374194775,20.3132381181289));
#51850=CARTESIAN_POINT('Ctrl Pts',(56.4181743272363,27.5970985951557,20.3120775743221));
#51851=CARTESIAN_POINT('Ctrl Pts',(56.3007411756435,27.4805076173041,20.301326039478));
#51852=CARTESIAN_POINT('Ctrl Pts',(56.1848825816581,27.388534254254,20.2912179121016));
#51853=CARTESIAN_POINT('Ctrl Pts',(55.9535101994514,27.2434009298712,20.2721968691635));
#51854=CARTESIAN_POINT('Ctrl Pts',(55.8409643670657,27.1868242477141,20.2633846613646));
#51855=CARTESIAN_POINT('Ctrl Pts',(55.7092712227914,27.1355413253915,20.2540274837502));
#51856=CARTESIAN_POINT('Ctrl Pts',(55.6946411449234,27.1300413018901,20.2530008733104));
#51857=CARTESIAN_POINT('Ctrl Pts',(55.6738980439167,27.1225202012563,20.2515649186153));
#51858=CARTESIAN_POINT('Ctrl Pts',(55.6678380019933,27.120356051234,20.2511477533775));
#51859=CARTESIAN_POINT('Ctrl Pts',(55.6576113325546,27.1167596256042,20.2504478331459));
#51860=CARTESIAN_POINT('Ctrl Pts',(55.6534502744929,27.1153117731264,20.2501641783316));
#51861=CARTESIAN_POINT('Ctrl Pts',(55.6449321778437,27.1123794780715,20.2495858663123));
#51862=CARTESIAN_POINT('Ctrl Pts',(55.6405747484556,27.1108963126644,20.2492912839591));
#51863=CARTESIAN_POINT('Ctrl Pts',(55.6294282065591,27.1071452963251,20.2485408302524));
#51864=CARTESIAN_POINT('Ctrl Pts',(55.6226318805277,27.1048988571841,20.2480861940411));
#51865=CARTESIAN_POINT('Ctrl Pts',(55.5947184433502,27.095838797817,20.2462303846405));
#51866=CARTESIAN_POINT('Ctrl Pts',(55.5734995279226,27.089340873188,20.2448464278422));
#51867=CARTESIAN_POINT('Ctrl Pts',(55.387447378154,27.035744593043,20.2329082187872));
#51868=CARTESIAN_POINT('Ctrl Pts',(55.2172685546736,27.0097172402152,20.2232760400318));
#51869=CARTESIAN_POINT('Ctrl Pts',(54.9508300797814,27.0035928778312,20.2076289897623));
#51870=CARTESIAN_POINT('Ctrl Pts',(54.8557978286487,27.0082014617678,20.20194730633));
#51871=CARTESIAN_POINT('Ctrl Pts',(54.746148165588,27.0214083892458,20.1950902735904));
#51872=CARTESIAN_POINT('Ctrl Pts',(54.7308553741873,27.0234305816337,20.1941272574393));
#51873=CARTESIAN_POINT('Ctrl Pts',(54.7059336231978,27.0270206114352,20.1925462964937));
#51874=CARTESIAN_POINT('Ctrl Pts',(54.6962898166136,27.0284821023465,20.1919316798763));
#51875=CARTESIAN_POINT('Ctrl Pts',(54.6790472840467,27.0312246716884,20.190827525957));
#51876=CARTESIAN_POINT('Ctrl Pts',(54.6714444822628,27.0324791720783,20.1903388330641));
#51877=CARTESIAN_POINT('Ctrl Pts',(54.6553333007128,27.0352335839746,20.1892992581965));
#51878=CARTESIAN_POINT('Ctrl Pts',(54.6468270361667,27.0367447804964,20.1887480296168));
#51879=CARTESIAN_POINT('Ctrl Pts',(54.6240616895708,27.0409419400025,20.187266308807));
#51880=CARTESIAN_POINT('Ctrl Pts',(54.6098218639321,27.0437282654283,20.1863326678506));
#51881=CARTESIAN_POINT('Ctrl Pts',(54.5386592520432,27.0584606240599,20.1816317134885));
#51882=CARTESIAN_POINT('Ctrl Pts',(54.4822528125834,27.0727358396722,20.1777913281591));
#51883=CARTESIAN_POINT('Ctrl Pts',(54.3176181343566,27.122150465332,20.166234823831));
#51884=CARTESIAN_POINT('Ctrl Pts',(54.2116883187531,27.1641015009474,20.1583305280501));
#51885=CARTESIAN_POINT('Ctrl Pts',(54.0144788372994,27.262429985131,20.1429720384443));
#51886=CARTESIAN_POINT('Ctrl Pts',(53.9229963553846,27.3176001886033,20.1355486561141));
#51887=CARTESIAN_POINT('Ctrl Pts',(53.8233015978568,27.3892030519188,20.127416773094));
#51888=CARTESIAN_POINT('Ctrl Pts',(53.8103592670076,27.3987377157222,20.1263604304975));
#51889=CARTESIAN_POINT('Ctrl Pts',(53.7923397859005,27.412351822388,20.1248903577272));
#51890=CARTESIAN_POINT('Ctrl Pts',(53.7871655911813,27.4163009666524,20.1244683128819));
#51891=CARTESIAN_POINT('Ctrl Pts',(53.7788267234149,27.4227303478538,20.1237883869248));
#51892=CARTESIAN_POINT('Ctrl Pts',(53.7756501084085,27.4251949102557,20.1235294351904));
#51893=CARTESIAN_POINT('Ctrl Pts',(53.7690110635026,27.4303780139795,20.1229883967133));
#51894=CARTESIAN_POINT('Ctrl Pts',(53.76555013977,27.4330984446766,20.1227064501391));
#51895=CARTESIAN_POINT('Ctrl Pts',(53.7572332431891,27.439680531862,20.1220290632497));
#51896=CARTESIAN_POINT('Ctrl Pts',(53.7523861809491,27.4435534652799,20.1216344121271));
#51897=CARTESIAN_POINT('Ctrl Pts',(53.7418679603286,27.4520385133603,20.1207780953088));
#51898=CARTESIAN_POINT('Ctrl Pts',(53.736203899764,27.4566593330837,20.1203170224554));
#51899=CARTESIAN_POINT('Ctrl Pts',(53.7203382421365,27.4697486710161,20.1190252448566));
#51900=CARTESIAN_POINT('Ctrl Pts',(53.7101952925552,27.4782880754162,20.1181991009269));
#51901=CARTESIAN_POINT('Ctrl Pts',(53.6766920046685,27.5070703533618,20.1154663102282));
#51902=CARTESIAN_POINT('Ctrl Pts',(53.6537161201567,27.5277558286336,20.1135857041806));
#51903=CARTESIAN_POINT('Ctrl Pts',(53.5423986913421,27.6327625124005,20.1043872997839));
#51904=CARTESIAN_POINT('Ctrl Pts',(53.461444578748,27.7245426484481,20.0974042762455));
#51905=CARTESIAN_POINT('Ctrl Pts',(53.3210266894231,27.9167165245161,20.0835254858019));
#51906=CARTESIAN_POINT('Ctrl Pts',(53.2609553638323,28.016042182112,20.0766677079713));
#51907=CARTESIAN_POINT('Ctrl Pts',(53.2028733896335,28.134197832196,20.0684975556814));
#51908=CARTESIAN_POINT('Ctrl Pts',(53.1960688057421,28.1484662827926,20.0675110735903));
#51909=CARTESIAN_POINT('Ctrl Pts',(53.1852927200342,28.1717715007861,20.0658993017305));
#51910=CARTESIAN_POINT('Ctrl Pts',(53.1812173636708,28.1807596963884,20.0652775640902));
#51911=CARTESIAN_POINT('Ctrl Pts',(53.1740739224297,28.196830594306,20.0641655130332));
#51912=CARTESIAN_POINT('Ctrl Pts',(53.1709799124847,28.2039016067456,20.0636760921307));
#51913=CARTESIAN_POINT('Ctrl Pts',(53.1645360519804,28.2188641892993,20.062640094573));
#51914=CARTESIAN_POINT('Ctrl Pts',(53.1611958910269,28.2267597370135,20.0620932025368));
#51915=CARTESIAN_POINT('Ctrl Pts',(53.1524557791894,28.247796723616,20.0606353713992));
#51916=CARTESIAN_POINT('Ctrl Pts',(53.1471452342085,28.2609745494767,20.0597214582628));
#51917=CARTESIAN_POINT('Ctrl Pts',(53.1221930727145,28.3248519350917,20.0552871525848));
#51918=CARTESIAN_POINT('Ctrl Pts',(53.1044907314344,28.3762793554329,20.051703325191));
#51919=CARTESIAN_POINT('Ctrl Pts',(53.0333349164898,28.614165836027,20.0350527207555));
#51920=CARTESIAN_POINT('Ctrl Pts',(53.0051631110213,28.8070311647972,20.0212202968295));
#51921=CARTESIAN_POINT('Ctrl Pts',(53.0052502012793,29.0008961046522,20.0080399322459));
#51922=CARTESIAN_POINT('Ctrl Pts',(53.0052502025236,29.0008988702651,20.0080397442193));
#51923=CARTESIAN_POINT('Ctrl Pts',(53.0052629847114,29.0292647731376,20.0061112226866));
#51924=CARTESIAN_POINT('Ctrl Pts',(53.0058808240606,29.0576289395148,20.0042010851021));
#51925=CARTESIAN_POINT('Ctrl Pts',(53.0077894752773,29.1018729660331,20.001259313683));
#51926=CARTESIAN_POINT('Ctrl Pts',(53.0086657422133,29.1177658134764,20.0002102331456));
#51927=CARTESIAN_POINT('Ctrl Pts',(53.0101217043145,29.1394479590473,19.9987909340733));
#51928=CARTESIAN_POINT('Ctrl Pts',(53.010536603078,29.1452472347752,19.9984124844107));
#51929=CARTESIAN_POINT('Ctrl Pts',(53.0113048449,29.1553637816291,19.9977544310216));
#51930=CARTESIAN_POINT('Ctrl Pts',(53.0116469033244,29.1596818347597,19.9974742323081));
#51931=CARTESIAN_POINT('Ctrl Pts',(53.0123411150536,29.1680970848409,19.9969295342592));
#51932=CARTESIAN_POINT('Ctrl Pts',(53.0126918790685,29.1721943859476,19.9966649600227));
#51933=CARTESIAN_POINT('Ctrl Pts',(53.0134715559545,29.1809820030418,19.9960989133663));
#51934=CARTESIAN_POINT('Ctrl Pts',(53.0139044116136,29.1856719131389,19.9957976625808));
#51935=CARTESIAN_POINT('Ctrl Pts',(53.0150831042282,29.1979668420696,19.995010027922));
#51936=CARTESIAN_POINT('Ctrl Pts',(53.0158560454696,29.2055692726816,19.9945251269722));
#51937=CARTESIAN_POINT('Ctrl Pts',(53.0192362760699,29.237019247725,19.9925272761347));
#51938=CARTESIAN_POINT('Ctrl Pts',(53.0222300849177,29.2608243407843,19.9910343636161));
#51939=CARTESIAN_POINT('Ctrl Pts',(53.0304342745286,29.3177448556571,19.9874986109912));
#51940=CARTESIAN_POINT('Ctrl Pts',(53.0360513951564,29.3507948940656,19.9854733189229));
#51941=CARTESIAN_POINT('Ctrl Pts',(53.0438584337799,29.3906247340389,19.9830495052251));
#51942=CARTESIAN_POINT('Ctrl Pts',(53.045254455155,29.3975516712013,19.9826285985524));
#51943=CARTESIAN_POINT('Ctrl Pts',(53.0466870003186,29.404469884881,19.982208722643));
#51944=CARTESIAN_POINT('Ctrl Pts',(53.0466869979816,29.4044698735951,19.8236610414577));
#51945=CARTESIAN_POINT('Ctrl Pts',(53.0459258685407,29.4007941386882,19.8239060899399));
#51946=CARTESIAN_POINT('Ctrl Pts',(53.0451751118795,29.3971162423574,19.8241514621327));
#51947=CARTESIAN_POINT('Ctrl Pts',(53.0182529607406,29.2633003408038,19.8330856262503));
#51948=CARTESIAN_POINT('Ctrl Pts',(53.0051309262974,29.1308984294748,19.8421861286945));
#51949=CARTESIAN_POINT('Ctrl Pts',(53.0053684879735,28.8679477486202,19.8604895091017));
#51950=CARTESIAN_POINT('Ctrl Pts',(53.0182430481131,28.7380122936548,19.8696375241136));
#51951=CARTESIAN_POINT('Ctrl Pts',(53.046701492835,28.5951678610035,19.8792777975915));
#51952=CARTESIAN_POINT('Ctrl Pts',(53.0498810867118,28.580118615176,19.8802878517556));
#51953=CARTESIAN_POINT('Ctrl Pts',(53.0544905052521,28.559484897967,19.8816636385968));
#51954=CARTESIAN_POINT('Ctrl Pts',(53.0557708349192,28.5538680633545,19.8820372211867));
#51955=CARTESIAN_POINT('Ctrl Pts',(53.0580033015897,28.544266338487,19.8826741605567));
#51956=CARTESIAN_POINT('Ctrl Pts',(53.0589434059971,28.5402787295693,19.882938184349));
#51957=CARTESIAN_POINT('Ctrl Pts',(53.0609228923809,28.5319967365322,19.883485467669));
#51958=CARTESIAN_POINT('Ctrl Pts',(53.0619642629959,28.5277028833428,19.8837686021172));
#51959=CARTESIAN_POINT('Ctrl Pts',(53.0645179141907,28.5173241564827,19.8844515699688));
#51960=CARTESIAN_POINT('Ctrl Pts',(53.0660446505626,28.5112428176311,19.8848505852162));
#51961=CARTESIAN_POINT('Ctrl Pts',(53.0715030205004,28.4899269604195,19.8862454168152));
#51962=CARTESIAN_POINT('Ctrl Pts',(53.075586315137,28.4747313912378,19.8872329926328));
#51963=CARTESIAN_POINT('Ctrl Pts',(53.1019674911502,28.3809962898027,19.8932919810013));
#51964=CARTESIAN_POINT('Ctrl Pts',(53.1288924652618,28.3038300292542,19.8981377023729));
#51965=CARTESIAN_POINT('Ctrl Pts',(53.1691801757111,28.2077671066386,19.9042347667852));
#51966=CARTESIAN_POINT('Ctrl Pts',(53.1782361297719,28.1871589276696,19.9055465772683));
#51967=CARTESIAN_POINT('Ctrl Pts',(53.2546931575205,28.0208693526359,19.9161933621505));
#51968=CARTESIAN_POINT('Ctrl Pts',(53.3390956026355,27.8836741638707,19.9254257294014));
#51969=CARTESIAN_POINT('Ctrl Pts',(53.4537358026589,27.7395821108431,19.9367752997941));
#51970=CARTESIAN_POINT('Ctrl Pts',(53.4687785380385,27.7213495456193,19.9382441909977));
#51971=CARTESIAN_POINT('Ctrl Pts',(53.4902642633129,27.6962307326188,19.9403166454428));
#51972=CARTESIAN_POINT('Ctrl Pts',(53.4964378593553,27.6891158779021,19.9409092840253));
#51973=CARTESIAN_POINT('Ctrl Pts',(53.5078462153795,27.6761547587684,19.9419994121569));
#51974=CARTESIAN_POINT('Ctrl Pts',(53.5130655476693,27.6702951187148,19.942496259432));
#51975=CARTESIAN_POINT('Ctrl Pts',(53.5237233945691,27.6584709851919,19.9435071042012));
#51976=CARTESIAN_POINT('Ctrl Pts',(53.5291638048277,27.6525084055346,19.9440211758571));
#51977=CARTESIAN_POINT('Ctrl Pts',(53.5427083815469,27.6378435824265,19.9452963961772));
#51978=CARTESIAN_POINT('Ctrl Pts',(53.5508543778261,27.6291805652089,19.9460593098843));
#51979=CARTESIAN_POINT('Ctrl Pts',(53.5817358081406,27.5969219974693,19.9489369371594));
#51980=CARTESIAN_POINT('Ctrl Pts',(53.6049729793758,27.5738160703316,19.9510731690277));
#51981=CARTESIAN_POINT('Ctrl Pts',(53.6647472130576,27.5172384302366,19.9565002863236));
#51982=CARTESIAN_POINT('Ctrl Pts',(53.7019804112189,27.4845375734769,19.9598207362227));
#51983=CARTESIAN_POINT('Ctrl Pts',(53.8216524980202,27.387080959678,19.9703048514465));
#51984=CARTESIAN_POINT('Ctrl Pts',(53.9079986269628,27.3274150563049,19.9776170202001));
#51985=CARTESIAN_POINT('Ctrl Pts',(54.0461432857822,27.2472296471289,19.9887431184047));
#51986=CARTESIAN_POINT('Ctrl Pts',(54.0947847259439,27.2216208724008,19.9925596269708));
#51987=CARTESIAN_POINT('Ctrl Pts',(54.1909277319891,27.1759715288244,19.9998434906164));
#51988=CARTESIAN_POINT('Ctrl Pts',(54.2382742689395,27.1556972309014,20.0033149411549));
#51989=CARTESIAN_POINT('Ctrl Pts',(54.294648297656,27.1340993097724,20.00727360884));
#51990=CARTESIAN_POINT('Ctrl Pts',(54.3029614886335,27.1309778678669,20.0078529987519));
#51991=CARTESIAN_POINT('Ctrl Pts',(54.316470739234,27.1260080787655,20.0087871394955));
#51992=CARTESIAN_POINT('Ctrl Pts',(54.3216539990172,27.12412562364,20.0091437990098));
#51993=CARTESIAN_POINT('Ctrl Pts',(54.3309019296265,27.120810305489,20.0097769442371));
#51994=CARTESIAN_POINT('Ctrl Pts',(54.3349634970455,27.1193690987681,20.010053911679));
#51995=CARTESIAN_POINT('Ctrl Pts',(54.3437819027651,27.1162721165611,20.0106528607775));
#51996=CARTESIAN_POINT('Ctrl Pts',(54.3485403462966,27.1146211916633,20.0109745580367));
#51997=CARTESIAN_POINT('Ctrl Pts',(54.3619372683264,27.1100299526725,20.0118761935313));
#51998=CARTESIAN_POINT('Ctrl Pts',(54.3705898746535,27.1071308204293,20.0124537825494));
#51999=CARTESIAN_POINT('Ctrl Pts',(54.4240486134709,27.0896260988569,20.0159948954767));
#52000=CARTESIAN_POINT('Ctrl Pts',(54.4693446541612,27.076551499702,20.0188770098322));
#52001=CARTESIAN_POINT('Ctrl Pts',(54.6310908631257,27.0360139632071,20.0288921244463));
#52002=CARTESIAN_POINT('Ctrl Pts',(54.7495045370738,27.0174281459756,20.0357375576361));
#52003=CARTESIAN_POINT('Ctrl Pts',(54.9859774136273,27.0018501061328,20.0495517046744));
#52004=CARTESIAN_POINT('Ctrl Pts',(55.1035142356001,27.0044852616821,20.0564920526417));
#52005=CARTESIAN_POINT('Ctrl Pts',(55.2358494954615,27.0191787683284,20.0647544914739));
#52006=CARTESIAN_POINT('Ctrl Pts',(55.2515480954056,27.0211111022326,20.0657415345642));
#52007=CARTESIAN_POINT('Ctrl Pts',(55.2770044300003,27.0245523143743,20.0673540422416));
#52008=CARTESIAN_POINT('Ctrl Pts',(55.2867770511817,27.0259473334792,20.0679759492637));
#52009=CARTESIAN_POINT('Ctrl Pts',(55.3041716460096,27.0285622633218,20.0690881889367));
#52010=CARTESIAN_POINT('Ctrl Pts',(55.3117977024553,27.0297539925529,20.0695776279258));
#52011=CARTESIAN_POINT('Ctrl Pts',(55.3278774565582,27.0323624809046,20.070613544683));
#52012=CARTESIAN_POINT('Ctrl Pts',(55.3363293039312,27.0337895258566,20.0711603371094));
#52013=CARTESIAN_POINT('Ctrl Pts',(55.3587584929024,27.0377254106278,20.0726176210716));
#52014=CARTESIAN_POINT('Ctrl Pts',(55.3727184849025,27.0403290750367,20.0735310826924));
#52015=CARTESIAN_POINT('Ctrl Pts',(55.4399073690834,27.0536042974031,20.0779595184352));
#52016=CARTESIAN_POINT('Ctrl Pts',(55.4927090899632,27.066295900276,20.0815377236312));
#52017=CARTESIAN_POINT('Ctrl Pts',(55.6465079757681,27.1099718054639,20.0922583970074));
#52018=CARTESIAN_POINT('Ctrl Pts',(55.7456303249572,27.1468378458137,20.099565152123));
#52019=CARTESIAN_POINT('Ctrl Pts',(55.9497623905248,27.2417982525519,20.1152520962225));
#52020=CARTESIAN_POINT('Ctrl Pts',(56.0534226525224,27.3018751965146,20.1236163459108));
#52021=CARTESIAN_POINT('Ctrl Pts',(56.1640324977419,27.3800286282452,20.1325862624167));
#52022=CARTESIAN_POINT('Ctrl Pts',(56.1768712097706,27.3893314759745,20.1336278908278));
#52023=CARTESIAN_POINT('Ctrl Pts',(56.1947934239375,27.4026465244753,20.1350810788089));
#52024=CARTESIAN_POINT('Ctrl Pts',(56.1999700056604,27.4065316319514,20.1355007071317));
#52025=CARTESIAN_POINT('Ctrl Pts',(56.208644253358,27.4131080358804,20.1362035613062));
#52026=CARTESIAN_POINT('Ctrl Pts',(56.2121520325748,27.4157858452376,20.1364877037132));
#52027=CARTESIAN_POINT('Ctrl Pts',(56.2192920134908,27.4212740457829,20.1370658454745));
#52028=CARTESIAN_POINT('Ctrl Pts',(56.222923440658,27.4240853728696,20.1373597765682));
#52029=CARTESIAN_POINT('Ctrl Pts',(56.2321522811287,27.4312811368237,20.1381065678778));
#52030=CARTESIAN_POINT('Ctrl Pts',(56.237736077697,27.4356830496389,20.1385582165152));
#52031=CARTESIAN_POINT('Ctrl Pts',(56.2603378735922,27.4536976635929,20.1403861572467));
#52032=CARTESIAN_POINT('Ctrl Pts',(56.2771565260448,27.467559537541,20.1417458755702));
#52033=CARTESIAN_POINT('Ctrl Pts',(56.3209540927002,27.5048793766787,20.1452956277409));
#52034=CARTESIAN_POINT('Ctrl Pts',(56.3475362550277,27.528792423374,20.1474593213889));
#52035=CARTESIAN_POINT('Ctrl Pts',(56.5009307203715,27.6744324124099,20.1601003662825));
#52036=CARTESIAN_POINT('Ctrl Pts',(56.6118467369842,27.8117744695597,20.1699611155816));
#52037=CARTESIAN_POINT('Ctrl Pts',(56.7339688655553,28.012151320056,20.1840059464739));
#52038=CARTESIAN_POINT('Ctrl Pts',(56.762362635997,28.0637468323247,20.1875884597438));
#52039=CARTESIAN_POINT('Ctrl Pts',(56.7950785964096,28.1299737882219,20.1921860363399));
#52040=CARTESIAN_POINT('Ctrl Pts',(56.8015731052074,28.1435030042143,20.1931251338487));
#52041=CARTESIAN_POINT('Ctrl Pts',(56.8116475298905,28.1651114754298,20.1946254377782));
#52042=CARTESIAN_POINT('Ctrl Pts',(56.8153275635434,28.1731436315659,20.1951832072608));
#52043=CARTESIAN_POINT('Ctrl Pts',(56.8221068186365,28.1882036604399,20.1962292909067));
#52044=CARTESIAN_POINT('Ctrl Pts',(56.8252190537049,28.1952255230493,20.196717150463));
#52045=CARTESIAN_POINT('Ctrl Pts',(56.8320750937027,28.2109385546904,20.1978091884106));
#52046=CARTESIAN_POINT('Ctrl Pts',(56.8357977416376,28.2196386989535,20.1984140696041));
#52047=CARTESIAN_POINT('Ctrl Pts',(56.8465656443678,28.2453077068345,20.2001995772363));
#52048=CARTESIAN_POINT('Ctrl Pts',(56.8534383696564,28.2623474334278,20.201385948705));
#52049=CARTESIAN_POINT('Ctrl Pts',(56.9118076517027,28.4130317956587,20.2118898116477));
#52050=CARTESIAN_POINT('Ctrl Pts',(56.9489971670341,28.551741808585,20.2216916776208));
#52051=CARTESIAN_POINT('Ctrl Pts',(56.9909458957835,28.821246522897,20.2406786473538));
#52052=CARTESIAN_POINT('Ctrl Pts',(56.9983533526711,28.9509313242624,20.249777392004));
#52053=CARTESIAN_POINT('Ctrl Pts',(56.9925059845408,29.0958407620512,20.2593769543132));
#52054=CARTESIAN_POINT('Ctrl Pts',(56.9917051713398,29.1112479001567,20.2603901055058));
#52055=CARTESIAN_POINT('Ctrl Pts',(56.9903595130661,29.1324002694528,20.2617693568444));
#52056=CARTESIAN_POINT('Ctrl Pts',(56.9899683978047,29.1381542627691,20.2621433580583));
#52057=CARTESIAN_POINT('Ctrl Pts',(56.989256645171,29.1479944609557,20.2627808265858));
#52058=CARTESIAN_POINT('Ctrl Pts',(56.9889483614221,29.1520814819885,20.2630449632698));
#52059=CARTESIAN_POINT('Ctrl Pts',(56.9882816754148,29.160571017478,20.2635922786538));
#52060=CARTESIAN_POINT('Ctrl Pts',(56.9879212452285,29.1649733178663,20.2638753332722));
#52061=CARTESIAN_POINT('Ctrl Pts',(56.9870144060123,29.1756147409497,20.2645577807351));
#52062=CARTESIAN_POINT('Ctrl Pts',(56.9864532241826,29.1818526260368,20.2649563585303));
#52063=CARTESIAN_POINT('Ctrl Pts',(56.9843832755523,29.2037074847165,20.2663479884683));
#52064=CARTESIAN_POINT('Ctrl Pts',(56.9827196030883,29.2193096784319,20.2673328503376));
#52065=CARTESIAN_POINT('Ctrl Pts',(56.9713135097276,29.315498945145,20.2733602891634));
#52066=CARTESIAN_POINT('Ctrl Pts',(56.9568425362784,29.3954577358452,20.2781797016291));
#52067=CARTESIAN_POINT('Ctrl Pts',(56.9288616780554,29.5097559755924,20.2850685553799));
#52068=CARTESIAN_POINT('Ctrl Pts',(56.9192161058482,29.5449478334186,20.2871892957999));
#52069=CARTESIAN_POINT('Ctrl Pts',(56.8662496329642,29.7192883846498,20.2977720079935));
#52070=CARTESIAN_POINT('Ctrl Pts',(56.8087433972027,29.8536420547964,20.3062141603725));
#52071=CARTESIAN_POINT('Ctrl Pts',(56.7253128843831,30.0014490120412,20.3166662730501));
#52072=CARTESIAN_POINT('Ctrl Pts',(56.7131276657345,30.0221537051854,20.3181580151639));
#52073=CARTESIAN_POINT('Ctrl Pts',(56.695480112871,30.0509375084443,20.3202734883446));
#52074=CARTESIAN_POINT('Ctrl Pts',(56.6903276368519,30.0592048595698,20.3208860207876));
#52075=CARTESIAN_POINT('Ctrl Pts',(56.6812560536497,30.073525800752,20.3219558343948));
#52076=CARTESIAN_POINT('Ctrl Pts',(56.6773642613603,30.0795965428431,20.3224121088525));
#52077=CARTESIAN_POINT('Ctrl Pts',(56.6691589362793,30.0922444195437,20.3233686077197));
#52078=CARTESIAN_POINT('Ctrl Pts',(56.6648392558706,30.0988173987543,20.3238690543218));
#52079=CARTESIAN_POINT('Ctrl Pts',(56.6544773036228,30.1143831439354,20.3250623034697));
#52080=CARTESIAN_POINT('Ctrl Pts',(56.6484004684786,30.1233524948079,20.3257563892084));
#52081=CARTESIAN_POINT('Ctrl Pts',(56.6276141130209,30.1535010984437,20.3281118236163));
#52082=CARTESIAN_POINT('Ctrl Pts',(56.6125675880513,30.1744437646563,20.3297858323143));
#52083=CARTESIAN_POINT('Ctrl Pts',(56.575545901197,30.2239196757102,20.333834235261));
#52084=CARTESIAN_POINT('Ctrl Pts',(56.553196342446,30.2521601793398,20.3362224441773));
#52085=CARTESIAN_POINT('Ctrl Pts',(56.4009255932269,30.4342141485875,20.3521396694851));
#52086=CARTESIAN_POINT('Ctrl Pts',(56.2491503754633,30.5681722070565,20.3665418677768));
#52087=CARTESIAN_POINT('Ctrl Pts',(56.0504041094137,30.6961459657168,20.3825274499051));
#52088=CARTESIAN_POINT('Ctrl Pts',(56.0203897840854,30.7143701390975,20.3848701817045));
#52089=CARTESIAN_POINT('Ctrl Pts',(55.9823828814955,30.7360952065576,20.3877348110478));
#52090=CARTESIAN_POINT('Ctrl Pts',(55.9748296440348,30.74034762727,20.3882991967866));
#52091=CARTESIAN_POINT('Ctrl Pts',(55.9628863538466,30.7469694653301,20.3891836154373));
#52092=CARTESIAN_POINT('Ctrl Pts',(55.9585148278326,30.7493718213574,20.3895056588589));
#52093=CARTESIAN_POINT('Ctrl Pts',(55.9503800886817,30.7538025900046,20.3901017635972));
#52094=CARTESIAN_POINT('Ctrl Pts',(55.9466193974751,30.755835286825,20.3903760846715));
#52095=CARTESIAN_POINT('Ctrl Pts',(55.9379505793471,30.760484935931,20.3910055683735));
#52096=CARTESIAN_POINT('Ctrl Pts',(55.9330380233506,30.7630934597205,20.3913602009648));
#52097=CARTESIAN_POINT('Ctrl Pts',(55.9177672883943,30.7711203840502,20.3924563089915));
#52098=CARTESIAN_POINT('Ctrl Pts',(55.9073721250756,30.7764684214648,20.3931935458831));
#52099=CARTESIAN_POINT('Ctrl Pts',(55.8036874426749,30.8286638687452,20.4004648611885));
#52100=CARTESIAN_POINT('Ctrl Pts',(55.7068900351237,30.8682177601293,20.4066010757966));
#52101=CARTESIAN_POINT('Ctrl Pts',(55.4482520227733,30.9509035461319,20.4224142989559));
#52102=CARTESIAN_POINT('Ctrl Pts',(55.2833305211374,30.9815833485493,20.4319958236938));
#52103=CARTESIAN_POINT('Ctrl Pts',(55.0958396954895,30.9925539976236,20.4435797620111));
#52104=CARTESIAN_POINT('Ctrl Pts',(55.0751429273717,30.9934417904447,20.444866705357));
#52105=CARTESIAN_POINT('Ctrl Pts',(55.0431754482489,30.9943145069531,20.4468688402119));
#52106=CARTESIAN_POINT('Ctrl Pts',(55.0319120194958,30.9945265319651,20.4475770202546));
#52107=CARTESIAN_POINT('Ctrl Pts',(55.0127813362699,30.9947245635323,20.4487847628381));
#52108=CARTESIAN_POINT('Ctrl Pts',(55.0049147728055,30.9947594564398,20.4492827988564));
#52109=CARTESIAN_POINT('Ctrl Pts',(54.9890011602543,30.9947359084866,20.4502932396808));
#52110=CARTESIAN_POINT('Ctrl Pts',(54.9809542655453,30.9946753059029,20.4508057022784));
#52111=CARTESIAN_POINT('Ctrl Pts',(54.9611365648998,30.9944061244919,20.4520716336622));
#52112=CARTESIAN_POINT('Ctrl Pts',(54.949366936242,30.9941420308167,20.4528268113612));
#52113=CARTESIAN_POINT('Ctrl Pts',(54.9057023614303,30.9927754535424,20.45564129832));
#52114=CARTESIAN_POINT('Ctrl Pts',(54.8738343612364,30.9910118258572,20.4577209216516));
#52115=CARTESIAN_POINT('Ctrl Pts',(54.7943769146838,30.9846992887201,20.4629728670991));
#52116=CARTESIAN_POINT('Ctrl Pts',(54.7468848436522,30.9792029308532,20.466172371802));
#52117=CARTESIAN_POINT('Ctrl Pts',(54.6034165452111,30.9573509307911,20.4760160636148));
#52118=CARTESIAN_POINT('Ctrl Pts',(54.5084030589648,30.9356731844385,20.4827872068433));
#52119=CARTESIAN_POINT('Ctrl Pts',(54.3129537807286,30.8757578373116,20.4970350918243));
#52120=CARTESIAN_POINT('Ctrl Pts',(54.213232674389,30.8361649258113,20.5044918611154));
#52121=CARTESIAN_POINT('Ctrl Pts',(54.1027676650897,30.7816451675347,20.5126528816709));
#52122=CARTESIAN_POINT('Ctrl Pts',(54.0884553190085,30.7743651538878,20.513708035996));
#52123=CARTESIAN_POINT('Ctrl Pts',(54.0684690556011,30.7638934178564,20.5151767450756));
#52124=CARTESIAN_POINT('Ctrl Pts',(54.0627209109932,30.7608457632865,20.5155985945279));
#52125=CARTESIAN_POINT('Ctrl Pts',(54.0534452933166,30.7558695594842,20.516278290354));
#52126=CARTESIAN_POINT('Ctrl Pts',(54.0499086168348,30.7539584051512,20.516537205984));
#52127=CARTESIAN_POINT('Ctrl Pts',(54.0425111560367,30.7499320145241,20.5170782145469));
#52128=CARTESIAN_POINT('Ctrl Pts',(54.0386515500382,30.7478146641589,20.5173601671325));
#52129=CARTESIAN_POINT('Ctrl Pts',(54.0291831062738,30.7425794961207,20.5180511547974));
#52130=CARTESIAN_POINT('Ctrl Pts',(54.0235821879486,30.7394473261514,20.5184592898812));
#52131=CARTESIAN_POINT('Ctrl Pts',(54.0115154156832,30.7326226444023,20.5193374840467));
#52132=CARTESIAN_POINT('Ctrl Pts',(54.0050548985863,30.7289208340657,20.5198069774494));
#52133=CARTESIAN_POINT('Ctrl Pts',(53.9868414760145,30.7183488269894,20.5211290514063));
#52134=CARTESIAN_POINT('Ctrl Pts',(53.9751377245541,30.7113942340231,20.5219768037957));
#52135=CARTESIAN_POINT('Ctrl Pts',(53.9360720882025,30.6876361934612,20.5248035944069));
#52136=CARTESIAN_POINT('Ctrl Pts',(53.9090437268382,30.6702913396737,20.5267545614378));
#52137=CARTESIAN_POINT('Ctrl Pts',(53.8253695243302,30.6136971780551,20.532817428938));
#52138=CARTESIAN_POINT('Ctrl Pts',(53.7703296525654,30.5721600672652,20.5368409028858));
#52139=CARTESIAN_POINT('Ctrl Pts',(53.5969867763769,30.42665936361,20.5500000806916));
#52140=CARTESIAN_POINT('Ctrl Pts',(53.488841491452,30.3115627843558,20.5590669790425));
#52141=CARTESIAN_POINT('Ctrl Pts',(53.3811609625366,30.1657436493565,20.5702371379898));
#52142=CARTESIAN_POINT('Ctrl Pts',(53.3673187463974,30.1462765520836,20.5717212770388));
#52143=CARTESIAN_POINT('Ctrl Pts',(53.3484874648867,30.1187597556868,20.5738116861549));
#52144=CARTESIAN_POINT('Ctrl Pts',(53.3432007384361,30.1109154992853,20.5744067736246));
#52145=CARTESIAN_POINT('Ctrl Pts',(53.3336252649365,30.0964873648291,20.5754999805151));
#52146=CARTESIAN_POINT('Ctrl Pts',(53.3293192221399,30.0899151501465,20.5759974439459));
#52147=CARTESIAN_POINT('Ctrl Pts',(53.3206756167565,30.0765510303496,20.577008064401));
#52148=CARTESIAN_POINT('Ctrl Pts',(53.3163401628376,30.0697579421131,20.5775212870127));
#52149=CARTESIAN_POINT('Ctrl Pts',(53.3057428417171,30.0529293257487,20.5787916144061));
#52150=CARTESIAN_POINT('Ctrl Pts',(53.2995289149833,30.0428641150754,20.5795504546087));
#52151=CARTESIAN_POINT('Ctrl Pts',(53.2766744528706,30.0050974510196,20.5823946803126));
#52152=CARTESIAN_POINT('Ctrl Pts',(53.260619076799,29.9770494513216,20.5845009424396));
#52153=CARTESIAN_POINT('Ctrl Pts',(53.2221335836362,29.9058597807356,20.5898350888148));
#52154=CARTESIAN_POINT('Ctrl Pts',(53.2005871599024,29.862266630887,20.5930912590761));
#52155=CARTESIAN_POINT('Ctrl Pts',(53.1210421906139,29.6853331690329,20.6062589913965));
#52156=CARTESIAN_POINT('Ctrl Pts',(53.0761357395278,29.5466871649761,20.6165112064369));
#52157=CARTESIAN_POINT('Ctrl Pts',(53.0466869978243,29.4044698728352,20.6265291208673));
#52158=CARTESIAN_POINT('Origin',(55.,29.,3.45145488139523));
#52159=CARTESIAN_POINT('',(53.0466869980088,29.4044698737264,21.5853976382171));
#52160=CARTESIAN_POINT('',(53.0466869889941,29.4044698301913,21.4261018347979));
#52161=CARTESIAN_POINT('',(53.0466869980082,29.4044698737233,3.45145488139523));
#52162=CARTESIAN_POINT('Ctrl Pts',(53.0466869980088,29.4044698737264,21.5853976382171));
#52163=CARTESIAN_POINT('Ctrl Pts',(53.0475866729437,29.4088146886609,21.5851174197649));
#52164=CARTESIAN_POINT('Ctrl Pts',(53.0485008375208,29.4131564689104,21.5848367448388));
#52165=CARTESIAN_POINT('Ctrl Pts',(53.0510413850145,29.4250261089356,21.5840676230934));
#52166=CARTESIAN_POINT('Ctrl Pts',(53.0526968760825,29.4325475893758,21.583578258594));
#52167=CARTESIAN_POINT('Ctrl Pts',(53.0565387818416,29.4495335484862,21.5824685170729));
#52168=CARTESIAN_POINT('Ctrl Pts',(53.0587508439812,29.458991967766,21.5818473329122));
#52169=CARTESIAN_POINT('Ctrl Pts',(53.0646230954277,29.4832987330159,21.5802424594353));
#52170=CARTESIAN_POINT('Ctrl Pts',(53.0683850609454,29.498121605463,21.5792555457274));
#52171=CARTESIAN_POINT('Ctrl Pts',(53.0956441761513,29.6005723596881,21.5723758036104));
#52172=CARTESIAN_POINT('Ctrl Pts',(53.1249218596305,29.6865392346039,21.5662975730865));
#52173=CARTESIAN_POINT('Ctrl Pts',(53.1882623848679,29.8378626369893,21.5550572670715));
#52174=CARTESIAN_POINT('Ctrl Pts',(53.2202905530021,29.9039028044674,21.5499526866739));
#52175=CARTESIAN_POINT('Ctrl Pts',(53.2883615924447,30.0265482942105,21.5401760873784));
#52176=CARTESIAN_POINT('Ctrl Pts',(53.3237688596617,30.0834007853545,21.5355117692802));
#52177=CARTESIAN_POINT('Ctrl Pts',(53.3924546143605,30.1822348132552,21.527268869493));
#52178=CARTESIAN_POINT('Ctrl Pts',(53.4246937558834,30.2248643451385,21.5236648751646));
#52179=CARTESIAN_POINT('Ctrl Pts',(53.4646133103848,30.2734617263761,21.5195439456683));
#52180=CARTESIAN_POINT('Ctrl Pts',(53.4706700751721,30.2807291066709,21.5189273642788));
#52181=CARTESIAN_POINT('Ctrl Pts',(53.4800769303661,30.2918542962245,21.5179833345641));
#52182=CARTESIAN_POINT('Ctrl Pts',(53.4833904253468,30.2957426672599,21.5176533590854));
#52183=CARTESIAN_POINT('Ctrl Pts',(53.4895224920075,30.3028828719338,21.5170474451264));
#52184=CARTESIAN_POINT('Ctrl Pts',(53.4923366364015,30.3061383015728,21.5167712058849));
#52185=CARTESIAN_POINT('Ctrl Pts',(53.4987189830961,30.3134733512336,21.5161488023784));
#52186=CARTESIAN_POINT('Ctrl Pts',(53.5022932850605,30.3175475451772,21.5158030929373));
#52187=CARTESIAN_POINT('Ctrl Pts',(53.5129160831282,30.3295569309571,21.5147838764607));
#52188=CARTESIAN_POINT('Ctrl Pts',(53.5200114849164,30.3374506403257,21.5141137181987));
#52189=CARTESIAN_POINT('Ctrl Pts',(53.5856367652806,30.4092976588884,21.5080077977972));
#52190=CARTESIAN_POINT('Ctrl Pts',(53.6482224551423,30.4694368291067,21.5028491131765));
#52191=CARTESIAN_POINT('Ctrl Pts',(53.8361286121852,30.6277956045964,21.4884533435434));
#52192=CARTESIAN_POINT('Ctrl Pts',(53.9695358952056,30.7153593442868,21.4794101365334));
#52193=CARTESIAN_POINT('Ctrl Pts',(54.1378952152832,30.7990675759546,21.4680253646136));
#52194=CARTESIAN_POINT('Ctrl Pts',(54.1641438568256,30.8114119320441,21.4662529701945));
#52195=CARTESIAN_POINT('Ctrl Pts',(54.210432358446,30.8319603976711,21.4631253405386));
#52196=CARTESIAN_POINT('Ctrl Pts',(54.2303543107103,30.8404188152807,21.4617786124758));
#52197=CARTESIAN_POINT('Ctrl Pts',(54.2597368819936,30.8523334978606,21.4597896198253));
#52198=CARTESIAN_POINT('Ctrl Pts',(54.2690927592634,30.8560451154775,21.4591558974024));
#52199=CARTESIAN_POINT('Ctrl Pts',(54.2857219773621,30.8624969458554,21.4580286338037));
#52200=CARTESIAN_POINT('Ctrl Pts',(54.2929840471148,30.8652657737004,21.4575360567882));
#52201=CARTESIAN_POINT('Ctrl Pts',(54.308108179015,30.8709311775209,21.456509508502));
#52202=CARTESIAN_POINT('Ctrl Pts',(54.3159726680144,30.8738207941411,21.4559753180964));
#52203=CARTESIAN_POINT('Ctrl Pts',(54.3363891202137,30.8811766689238,21.4545874194387));
#52204=CARTESIAN_POINT('Ctrl Pts',(54.3489678786778,30.8855668172432,21.4537312256197));
#52205=CARTESIAN_POINT('Ctrl Pts',(54.3999095468147,30.9027756086774,21.4502587846134));
#52206=CARTESIAN_POINT('Ctrl Pts',(54.4386120410212,30.9145513149261,21.4476089489539));
#52207=CARTESIAN_POINT('Ctrl Pts',(54.6669542790494,30.9765083331097,21.4318971128434));
#52208=CARTESIAN_POINT('Ctrl Pts',(54.8627945184981,30.999663148227,21.4179627900108));
#52209=CARTESIAN_POINT('Ctrl Pts',(55.1136080505873,30.992266951694,21.4007642780754));
#52210=CARTESIAN_POINT('Ctrl Pts',(55.1683345292068,30.9883910749464,21.3970620342585));
#52211=CARTESIAN_POINT('Ctrl Pts',(55.2322586958507,30.9812050266889,21.3928468493298));
#52212=CARTESIAN_POINT('Ctrl Pts',(55.2416733086971,30.9800786549909,21.3922288572349));
#52213=CARTESIAN_POINT('Ctrl Pts',(55.2561522353545,30.9782415775427,21.3912831313436));
#52214=CARTESIAN_POINT('Ctrl Pts',(55.261222293697,30.9775784741657,21.3909528564705));
#52215=CARTESIAN_POINT('Ctrl Pts',(55.2705541975896,30.9763214575533,21.3903466613938));
#52216=CARTESIAN_POINT('Ctrl Pts',(55.2748166546953,30.9757332523321,21.3900704383363));
#52217=CARTESIAN_POINT('Ctrl Pts',(55.2844381566664,30.9743737766701,21.3894484073221));
#52218=CARTESIAN_POINT('Ctrl Pts',(55.2897959767613,30.973594479238,21.3891030517513));
#52219=CARTESIAN_POINT('Ctrl Pts',(55.305621128299,30.9712268701544,21.3880858542176));
#52220=CARTESIAN_POINT('Ctrl Pts',(55.3160792560108,30.9695770010663,21.3874173413406));
#52221=CARTESIAN_POINT('Ctrl Pts',(55.4093491075843,30.9541007497376,21.3814844312317));
#52222=CARTESIAN_POINT('Ctrl Pts',(55.4912349431084,30.9351403653771,21.3764797168246));
#52223=CARTESIAN_POINT('Ctrl Pts',(55.7195727714648,30.8668338603714,21.3625016573911));
#52224=CARTESIAN_POINT('Ctrl Pts',(55.8618131388206,30.8055833633758,21.3537264356013));
#52225=CARTESIAN_POINT('Ctrl Pts',(56.024175401637,30.7120695261921,21.3424343371581));
#52226=CARTESIAN_POINT('Ctrl Pts',(56.0523667046824,30.694886857151,21.3404247528584));
#52227=CARTESIAN_POINT('Ctrl Pts',(56.1003930862474,30.6639544007427,21.3369053769586));
#52228=CARTESIAN_POINT('Ctrl Pts',(56.1204293606411,30.6505293581636,21.3354071073224));
#52229=CARTESIAN_POINT('Ctrl Pts',(56.1488730299327,30.6307144511484,21.3332340089243));
#52230=CARTESIAN_POINT('Ctrl Pts',(56.1574812796662,30.6246156285403,21.3325701232361));
#52231=CARTESIAN_POINT('Ctrl Pts',(56.1723823672207,30.6138798720346,21.3314098356442));
#52232=CARTESIAN_POINT('Ctrl Pts',(56.1786971340212,30.6092736621721,21.3309146150367));
#52233=CARTESIAN_POINT('Ctrl Pts',(56.1916371949081,30.5997177097605,21.3298924691774));
#52234=CARTESIAN_POINT('Ctrl Pts',(56.198259096259,30.5947636470875,21.329365383029));
#52235=CARTESIAN_POINT('Ctrl Pts',(56.2150709093343,30.5820223515973,21.3280168008159));
#52236=CARTESIAN_POINT('Ctrl Pts',(56.2252167556231,30.574177856771,21.3271930794357));
#52237=CARTESIAN_POINT('Ctrl Pts',(56.2640187489987,30.5435748347311,21.3240040339419));
#52238=CARTESIAN_POINT('Ctrl Pts',(56.2921207259121,30.5201284180012,21.32161163995));
#52239=CARTESIAN_POINT('Ctrl Pts',(56.4701012857083,30.3631310161828,21.305901274376));
#52240=CARTESIAN_POINT('Ctrl Pts',(56.5997206967542,30.2083822667965,21.2916410916346));
#52241=CARTESIAN_POINT('Ctrl Pts',(56.7326947913602,29.9898664933802,21.2741056128495));
#52242=CARTESIAN_POINT('Ctrl Pts',(56.7593922637672,29.9415980980176,21.2703827649737));
#52243=CARTESIAN_POINT('Ctrl Pts',(56.7883043616662,29.8837902469877,21.2661472993053));
#52244=CARTESIAN_POINT('Ctrl Pts',(56.792490413267,29.8752689972314,21.2655285026119));
#52245=CARTESIAN_POINT('Ctrl Pts',(56.798838356384,29.8621103763271,21.2645818091744));
#52246=CARTESIAN_POINT('Ctrl Pts',(56.8010434431125,29.8574941695458,21.2642513634029));
#52247=CARTESIAN_POINT('Ctrl Pts',(56.8050704371073,29.8489798543156,21.2636450072715));
#52248=CARTESIAN_POINT('Ctrl Pts',(56.8068974844995,29.845084349113,21.2633687928649));
#52249=CARTESIAN_POINT('Ctrl Pts',(56.8109937399303,29.8362765776634,21.2627469720233));
#52250=CARTESIAN_POINT('Ctrl Pts',(56.8132555705126,29.8313609794026,21.262401816593));
#52251=CARTESIAN_POINT('Ctrl Pts',(56.8198774729612,29.8168141249134,21.2613857605827));
#52252=CARTESIAN_POINT('Ctrl Pts',(56.8241810917021,29.807157164007,21.2607181779785));
#52253=CARTESIAN_POINT('Ctrl Pts',(56.8684164559205,29.7057355777539,21.2537745422634));
#52254=CARTESIAN_POINT('Ctrl Pts',(56.9014710342913,29.6111106577518,21.2478694496601));
#52255=CARTESIAN_POINT('Ctrl Pts',(56.9311218502605,29.5000173279117,21.2411634803102));
#52256=CARTESIAN_POINT('Ctrl Pts',(56.9347976548042,29.4855995968175,21.2402975415681));
#52257=CARTESIAN_POINT('Ctrl Pts',(56.9651722033418,29.3606365404419,21.2328206320292));
#52258=CARTESIAN_POINT('Ctrl Pts',(56.9825320292906,29.2480432304664,21.2262611585592));
#52259=CARTESIAN_POINT('Ctrl Pts',(56.994128524497,29.0765604276137,21.2159623428842));
#52260=CARTESIAN_POINT('Ctrl Pts',(56.9955126541715,29.0183945161383,21.2124188690831));
#52261=CARTESIAN_POINT('Ctrl Pts',(56.994064904118,28.9457482884481,21.2078922551418));
#52262=CARTESIAN_POINT('Ctrl Pts',(56.9936175388369,28.9312454989239,21.2069836173327));
#52263=CARTESIAN_POINT('Ctrl Pts',(56.9926514408767,28.9081172616422,21.2055261175926));
#52264=CARTESIAN_POINT('Ctrl Pts',(56.9922348042019,28.8994878933492,21.2049804316586));
#52265=CARTESIAN_POINT('Ctrl Pts',(56.9913405308366,28.8831675147011,21.2039447272672));
#52266=CARTESIAN_POINT('Ctrl Pts',(56.9908743591029,28.8754760146559,21.2034550746141));
#52267=CARTESIAN_POINT('Ctrl Pts',(56.9897171415978,28.8580549419975,21.2023424367542));
#52268=CARTESIAN_POINT('Ctrl Pts',(56.9889992764816,28.8483274063523,21.2017186276038));
#52269=CARTESIAN_POINT('Ctrl Pts',(56.986961998098,28.8232302583095,21.2001024683209));
#52270=CARTESIAN_POINT('Ctrl Pts',(56.9855356070042,28.807870213824,21.1991068173323));
#52271=CARTESIAN_POINT('Ctrl Pts',(56.9740451350478,28.6979933490655,21.1919362989337));
#52272=CARTESIAN_POINT('Ctrl Pts',(56.9574163504813,28.6042996718033,21.1855570936841));
#52273=CARTESIAN_POINT('Ctrl Pts',(56.8922463236282,28.3459155112234,21.1672628605141));
#52274=CARTESIAN_POINT('Ctrl Pts',(56.8290616118007,28.1857796816078,21.1550440028991));
#52275=CARTESIAN_POINT('Ctrl Pts',(56.7354585648006,28.0162809621643,21.1421231446964));
#52276=CARTESIAN_POINT('Ctrl Pts',(56.7244119724049,27.9970428605373,21.1406580555409));
#52277=CARTESIAN_POINT('Ctrl Pts',(56.7093794110298,27.9718459197623,21.1387450099526));
#52278=CARTESIAN_POINT('Ctrl Pts',(56.7056794685354,27.9657194104438,21.1382803279182));
#52279=CARTESIAN_POINT('Ctrl Pts',(56.6995459877783,27.9556857836644,21.1375202356841));
#52280=CARTESIAN_POINT('Ctrl Pts',(56.6971317957851,27.9517670030988,21.1372236068421));
#52281=CARTESIAN_POINT('Ctrl Pts',(56.6923801381624,27.9441134331864,21.1366447937774));
#52282=CARTESIAN_POINT('Ctrl Pts',(56.6900438349191,27.9403779869113,21.1363625413001));
#52283=CARTESIAN_POINT('Ctrl Pts',(56.6842645950846,27.9312054682969,21.1356699911688));
#52284=CARTESIAN_POINT('Ctrl Pts',(56.6808076483625,27.9257771976033,21.1352606023971));
#52285=CARTESIAN_POINT('Ctrl Pts',(56.6688633535334,27.9072204910524,21.1338623344909));
#52286=CARTESIAN_POINT('Ctrl Pts',(56.6602477292406,27.8941747602424,21.1328814643415));
#52287=CARTESIAN_POINT('Ctrl Pts',(56.5808963407455,27.7770395874117,21.1240809376007));
#52288=CARTESIAN_POINT('Ctrl Pts',(56.5006012768501,27.6797462186289,21.1168067781436));
#52289=CARTESIAN_POINT('Ctrl Pts',(56.3071510762284,27.4859773917615,21.1009075841975));
#52290=CARTESIAN_POINT('Ctrl Pts',(56.1913370186391,27.3932588928929,21.0922946927273));
#52291=CARTESIAN_POINT('Ctrl Pts',(56.0514643828032,27.3047831039346,21.0820248406906));
#52292=CARTESIAN_POINT('Ctrl Pts',(56.0364582368483,27.295566966588,21.0809252634917));
#52293=CARTESIAN_POINT('Ctrl Pts',(56.0133390183227,27.2817863368983,21.0792336013539));
#52294=CARTESIAN_POINT('Ctrl Pts',(56.0053125018352,27.277077794248,21.0786467285246));
#52295=CARTESIAN_POINT('Ctrl Pts',(55.9912537081761,27.2689622648976,21.0776194184293));
#52296=CARTESIAN_POINT('Ctrl Pts',(55.9852360367152,27.2655301950416,21.0771798900242));
#52297=CARTESIAN_POINT('Ctrl Pts',(55.971629084303,27.2578633766516,21.0761864224438));
#52298=CARTESIAN_POINT('Ctrl Pts',(55.9640297986444,27.2536467610235,21.0756318487557));
#52299=CARTESIAN_POINT('Ctrl Pts',(55.9434650841826,27.2424111506515,21.0741316694769));
#52300=CARTESIAN_POINT('Ctrl Pts',(55.9304491942491,27.2354861275397,21.0731827773761));
#52301=CARTESIAN_POINT('Ctrl Pts',(55.8696675157905,27.2040071265859,21.0687535379843));
#52302=CARTESIAN_POINT('Ctrl Pts',(55.8210031216531,27.1812463161389,21.0652118407498));
#52303=CARTESIAN_POINT('Ctrl Pts',(55.6043126855331,27.0903677757737,21.0494514633099));
#52304=CARTESIAN_POINT('Ctrl Pts',(55.4283711448534,27.0433779294654,21.0365791649457));
#52305=CARTESIAN_POINT('Ctrl Pts',(55.2127517289641,27.016299853377,21.0216940953161));
#52306=CARTESIAN_POINT('Ctrl Pts',(55.1768319924736,27.0127757233648,21.0192472671285));
#52307=CARTESIAN_POINT('Ctrl Pts',(55.1189504424811,27.0086789152652,21.0153762066015));
#52308=CARTESIAN_POINT('Ctrl Pts',(55.0970412904931,27.0074910404696,21.013927437896));
#52309=CARTESIAN_POINT('Ctrl Pts',(55.0679932290472,27.0063964063919,21.0120322492798));
#52310=CARTESIAN_POINT('Ctrl Pts',(55.0608689936922,27.0061661711769,21.0115694839951));
#52311=CARTESIAN_POINT('Ctrl Pts',(55.049148934728,27.0058502888386,21.0108117164979));
#52312=CARTESIAN_POINT('Ctrl Pts',(55.0445538500787,27.0057423326479,21.0105155098098));
#52313=CARTESIAN_POINT('Ctrl Pts',(55.0355489803478,27.0055619129486,21.0099368413561));
#52314=CARTESIAN_POINT('Ctrl Pts',(55.0311392735246,27.0054881902333,21.0096543151223));
#52315=CARTESIAN_POINT('Ctrl Pts',(55.0202717386222,27.0053425539706,21.008960056072));
#52316=CARTESIAN_POINT('Ctrl Pts',(55.013813665148,27.005287375134,21.0085492425247));
#52317=CARTESIAN_POINT('Ctrl Pts',(54.9915859702474,27.0052054133999,21.0071409683663));
#52318=CARTESIAN_POINT('Ctrl Pts',(54.9758158972198,27.0053342625682,21.00615167141));
#52319=CARTESIAN_POINT('Ctrl Pts',(54.8379178685051,27.0080966871332,20.9975741894971));
#52320=CARTESIAN_POINT('Ctrl Pts',(54.7162526165712,27.0217570817255,20.9904987464281));
#52321=CARTESIAN_POINT('Ctrl Pts',(54.4949827445759,27.0674500854174,20.9773788164561));
#52322=CARTESIAN_POINT('Ctrl Pts',(54.3951730042513,27.0963262137655,20.9713592013312));
#52323=CARTESIAN_POINT('Ctrl Pts',(54.2648390214939,27.14532318027,20.9629905732852));
#52324=CARTESIAN_POINT('Ctrl Pts',(54.2319510402049,27.1586992775821,20.9608344175842));
#52325=CARTESIAN_POINT('Ctrl Pts',(54.1760774994199,27.1831814054556,20.9570814995931));
#52326=CARTESIAN_POINT('Ctrl Pts',(54.1529155582769,27.1938643601365,20.955498502523));
#52327=CARTESIAN_POINT('Ctrl Pts',(54.1202585254526,27.2096930809307,20.9532244954146));
#52328=CARTESIAN_POINT('Ctrl Pts',(54.1105899355263,27.2144766435468,20.9525459111537));
#52329=CARTESIAN_POINT('Ctrl Pts',(54.0939469993248,27.2228795045259,20.9513683654091));
#52330=CARTESIAN_POINT('Ctrl Pts',(54.0869542957043,27.226462057222,20.9508706884499));
#52331=CARTESIAN_POINT('Ctrl Pts',(54.0735756660803,27.2334163866106,20.9499128182821));
#52332=CARTESIAN_POINT('Ctrl Pts',(54.0671865152667,27.2367817179849,20.9494528568374));
#52333=CARTESIAN_POINT('Ctrl Pts',(54.0521855716578,27.2447874581097,20.948366909629));
#52334=CARTESIAN_POINT('Ctrl Pts',(54.043589423659,27.2494566381734,20.9477399166424));
#52335=CARTESIAN_POINT('Ctrl Pts',(54.0137138783033,27.2659699139842,20.9455441382238));
#52336=CARTESIAN_POINT('Ctrl Pts',(53.992618021504,27.2781399255592,20.9439638454979));
#52337=CARTESIAN_POINT('Ctrl Pts',(53.8593808753254,27.3582899138892,20.9337866924179));
#52338=CARTESIAN_POINT('Ctrl Pts',(53.7539694850766,27.436791456716,20.9248018826938));
#52339=CARTESIAN_POINT('Ctrl Pts',(53.5828300923145,27.5926162860125,20.9086945810757));
#52340=CARTESIAN_POINT('Ctrl Pts',(53.51382534887,27.6656889549421,20.9016609362184));
#52341=CARTESIAN_POINT('Ctrl Pts',(53.4329748277004,27.7653973162296,20.8929369266958));
#52342=CARTESIAN_POINT('Ctrl Pts',(53.4157973145792,27.7875175505144,20.8910519734023));
#52343=CARTESIAN_POINT('Ctrl Pts',(53.3882058932978,27.8246361380822,20.8879803380853));
#52344=CARTESIAN_POINT('Ctrl Pts',(53.3775223010567,27.839428320528,20.8867793823382));
#52345=CARTESIAN_POINT('Ctrl Pts',(53.3632259115094,27.8598060200889,20.8851584586557));
#52346=CARTESIAN_POINT('Ctrl Pts',(53.3594362349707,27.8652655533219,20.8847274131131));
#52347=CARTESIAN_POINT('Ctrl Pts',(53.3531304752003,27.874447462333,20.8840080044845));
#52348=CARTESIAN_POINT('Ctrl Pts',(53.3505995825922,27.8781595429862,20.8837186629159));
#52349=CARTESIAN_POINT('Ctrl Pts',(53.3458278299211,27.8852093670303,20.8831720464143));
#52350=CARTESIAN_POINT('Ctrl Pts',(53.3435844888756,27.8885453770744,20.8829146011717));
#52351=CARTESIAN_POINT('Ctrl Pts',(53.3377367195202,27.8972984607662,20.8822422261263));
#52352=CARTESIAN_POINT('Ctrl Pts',(53.3341486476719,27.9027264821275,20.8818283776927));
#52353=CARTESIAN_POINT('Ctrl Pts',(53.3217966418752,27.9216127886908,20.8803988197069));
#52354=CARTESIAN_POINT('Ctrl Pts',(53.3131684579371,27.9351596947544,20.879391607141));
#52355=CARTESIAN_POINT('Ctrl Pts',(53.2472355815369,28.0414922220892,20.8716142837777));
#52356=CARTESIAN_POINT('Ctrl Pts',(53.1974560591343,28.1387440574427,20.8652499193493));
#52357=CARTESIAN_POINT('Ctrl Pts',(53.1302656413683,28.3016923803078,20.8550055780894));
#52358=CARTESIAN_POINT('Ctrl Pts',(53.1078116434887,28.3650487307882,20.8511184608071));
#52359=CARTESIAN_POINT('Ctrl Pts',(53.06295064399,28.5153288405849,20.8419195531604));
#52360=CARTESIAN_POINT('Ctrl Pts',(53.043128424588,28.6028637249946,20.8365739464099));
#52361=CARTESIAN_POINT('Ctrl Pts',(53.0258366984816,28.7132999664281,20.8296731230831));
#52362=CARTESIAN_POINT('Ctrl Pts',(53.0227765874294,28.7352261972321,20.8282958260924));
#52363=CARTESIAN_POINT('Ctrl Pts',(53.0188411939818,28.767317205628,20.8262676273844));
#52364=CARTESIAN_POINT('Ctrl Pts',(53.0176778847017,28.7774454617425,20.8256257140402));
#52365=CARTESIAN_POINT('Ctrl Pts',(53.0157658242641,28.7952989213614,20.8244908480397));
#52366=CARTESIAN_POINT('Ctrl Pts',(53.0149844189756,28.8030204678559,20.8239989250313));
#52367=CARTESIAN_POINT('Ctrl Pts',(53.0134500878188,28.8191194970896,20.8229709179553));
#52368=CARTESIAN_POINT('Ctrl Pts',(53.0127050508937,28.8274975605128,20.8224345980065));
#52369=CARTESIAN_POINT('Ctrl Pts',(53.0109046605308,28.8493057019706,20.8210349589545));
#52370=CARTESIAN_POINT('Ctrl Pts',(53.0099323441504,28.8627420260075,20.8201690746088));
#52371=CARTESIAN_POINT('Ctrl Pts',(53.0065097342746,28.9177772930961,20.8166072788937));
#52372=CARTESIAN_POINT('Ctrl Pts',(53.0052272996647,28.9594357326713,20.8138755641965));
#52373=CARTESIAN_POINT('Ctrl Pts',(53.0052897809569,29.0726028522538,20.8063530938477));
#52374=CARTESIAN_POINT('Ctrl Pts',(53.0091736191226,29.1440436529404,20.801492171297));
#52375=CARTESIAN_POINT('Ctrl Pts',(53.0237803554166,29.278700715536,20.7921524527072));
#52376=CARTESIAN_POINT('Ctrl Pts',(53.0337289129306,29.3418912045436,20.7876948307582));
#52377=CARTESIAN_POINT('Ctrl Pts',(53.0466870286012,29.4044700214667,20.7832412988479));
#52378=CARTESIAN_POINT('',(53.0052497878256,29.0009911092822,20.6530359722443));
#52379=CARTESIAN_POINT('Ctrl Pts',(53.0466869978243,29.4044698728352,20.6265291208673));
#52380=CARTESIAN_POINT('Ctrl Pts',(53.0423917803693,29.3837269086108,20.6279902739909));
#52381=CARTESIAN_POINT('Ctrl Pts',(53.0384253997232,29.3629079073144,20.6294455367161));
#52382=CARTESIAN_POINT('Ctrl Pts',(53.0291254426595,29.3094714389379,20.6331463186058));
#52383=CARTESIAN_POINT('Ctrl Pts',(53.02426986673,29.2767847291785,20.6353774910218));
#52384=CARTESIAN_POINT('Ctrl Pts',(53.0179376162708,29.2254040379901,20.638819347937));
#52385=CARTESIAN_POINT('Ctrl Pts',(53.0159087212894,29.2067852307779,20.6400532000872));
#52386=CARTESIAN_POINT('Ctrl Pts',(53.0134887093812,29.1812414667323,20.6417252052073));
#52387=CARTESIAN_POINT('Ctrl Pts',(53.0128710972373,29.1743396232666,20.6421749038912));
#52388=CARTESIAN_POINT('Ctrl Pts',(53.0119452901785,29.1633488443142,20.6428875777845));
#52389=CARTESIAN_POINT('Ctrl Pts',(53.0116137230563,29.1592620123635,20.6431518224063));
#52390=CARTESIAN_POINT('Ctrl Pts',(53.0109763952033,29.1510940455679,20.6436783913493));
#52391=CARTESIAN_POINT('Ctrl Pts',(53.0106705909434,29.1470129708689,20.6439407100236));
#52392=CARTESIAN_POINT('Ctrl Pts',(53.0100651935259,29.1385857382147,20.6444808278499));
#52393=CARTESIAN_POINT('Ctrl Pts',(53.0097672726809,29.1342394607415,20.6447585350891));
#52394=CARTESIAN_POINT('Ctrl Pts',(53.0091005646849,29.1240225787607,20.6454094130717));
#52395=CARTESIAN_POINT('Ctrl Pts',(53.0087434985907,29.1181512132631,20.6457819551888));
#52396=CARTESIAN_POINT('Ctrl Pts',(53.0076145848768,29.0981265854036,20.6470476796835));
#52397=CARTESIAN_POINT('Ctrl Pts',(53.0069675999165,29.0839663452612,20.6479344661133));
#52398=CARTESIAN_POINT('Ctrl Pts',(53.0056688480167,29.0468732193099,20.6502386092127));
#52399=CARTESIAN_POINT('Ctrl Pts',(53.0052616459177,29.0239335306591,20.6516447617078));
#52400=CARTESIAN_POINT('Ctrl Pts',(53.0052502462445,29.0009911570512,20.6530367634788));
#52401=CARTESIAN_POINT('Ctrl Pts',(53.0052502449332,29.0009885144422,20.653036923816));
#52402=CARTESIAN_POINT('Ctrl Pts',(53.0051989849948,28.8975497125354,20.6593129475683));
#52403=CARTESIAN_POINT('Ctrl Pts',(53.0131936139981,28.794251182285,20.6652955731722));
#52404=CARTESIAN_POINT('Ctrl Pts',(53.0514847436693,28.5492109164505,20.6796977461016));
#52405=CARTESIAN_POINT('Ctrl Pts',(53.0892555137733,28.4092625251289,20.6881242733579));
#52406=CARTESIAN_POINT('Ctrl Pts',(53.1484359598757,28.2576590340402,20.6982154482694));
#52407=CARTESIAN_POINT('Ctrl Pts',(53.1552932332696,28.2407790736154,20.6993524755353));
#52408=CARTESIAN_POINT('Ctrl Pts',(53.1660497119535,28.2153071562461,20.7010898339193));
#52409=CARTESIAN_POINT('Ctrl Pts',(53.1697803591026,28.2066447332736,20.701684500728));
#52410=CARTESIAN_POINT('Ctrl Pts',(53.1766594771817,28.1909784533875,20.7027670936905));
#52411=CARTESIAN_POINT('Ctrl Pts',(53.1797872425967,28.1839656624003,20.7032543100944));
#52412=CARTESIAN_POINT('Ctrl Pts',(53.1866106031195,28.1689013654378,20.7043066248604));
#52413=CARTESIAN_POINT('Ctrl Pts',(53.1903194900122,28.1608560953517,20.7048721690013));
#52414=CARTESIAN_POINT('Ctrl Pts',(53.2004996920883,28.1391547363046,20.7064074270979));
#52415=CARTESIAN_POINT('Ctrl Pts',(53.2070726964551,28.1255472627527,20.7073806133059));
#52416=CARTESIAN_POINT('Ctrl Pts',(53.2405537686634,28.0581993005751,20.7122509336185));
#52417=CARTESIAN_POINT('Ctrl Pts',(53.2697238921021,28.0056243481379,20.7162259181694));
#52418=CARTESIAN_POINT('Ctrl Pts',(53.3721458578102,27.8392119879154,20.7293891472845));
#52419=CARTESIAN_POINT('Ctrl Pts',(53.4546078327571,27.7314996108954,20.7388688884355));
#52420=CARTESIAN_POINT('Ctrl Pts',(53.5902251982648,27.5873847271806,20.7526213803075));
#52421=CARTESIAN_POINT('Ctrl Pts',(53.6352544108055,27.5438346798413,20.7569421839769));
#52422=CARTESIAN_POINT('Ctrl Pts',(53.6982097756871,27.4884375186073,20.7625937797129));
#52423=CARTESIAN_POINT('Ctrl Pts',(53.7143832161155,27.4746579120183,20.7640135131849));
#52424=CARTESIAN_POINT('Ctrl Pts',(53.7386347278624,27.4546556927652,20.7660916254736));
#52425=CARTESIAN_POINT('Ctrl Pts',(53.7465448144534,27.4482327863435,20.7667616588283));
#52426=CARTESIAN_POINT('Ctrl Pts',(53.7592680630799,27.4380624140574,20.7678265685715));
#52427=CARTESIAN_POINT('Ctrl Pts',(53.7640496859873,27.4342760188215,20.7682239229845));
#52428=CARTESIAN_POINT('Ctrl Pts',(53.7731685390955,27.4271229313564,20.7689761719254));
#52429=CARTESIAN_POINT('Ctrl Pts',(53.7775024396143,27.4237521060715,20.7693313419399));
#52430=CARTESIAN_POINT('Ctrl Pts',(53.7851797162008,27.4178315771225,20.7699562882723));
#52431=CARTESIAN_POINT('Ctrl Pts',(53.7885172983543,27.415274501652,20.7702265743523));
#52432=CARTESIAN_POINT('Ctrl Pts',(53.7957885449339,27.40974006183,20.770812364423));
#52433=CARTESIAN_POINT('Ctrl Pts',(53.7997251763587,27.40676673131,20.7711275894078));
#52434=CARTESIAN_POINT('Ctrl Pts',(53.8104183069469,27.3987523555781,20.7719787755734));
#52435=CARTESIAN_POINT('Ctrl Pts',(53.8171958861225,27.3937394179745,20.7725128357389));
#52436=CARTESIAN_POINT('Ctrl Pts',(53.8501385958939,27.3696953995737,20.7750835354035));
#52437=CARTESIAN_POINT('Ctrl Pts',(53.876733956542,27.351258658223,20.777082801111));
#52438=CARTESIAN_POINT('Ctrl Pts',(54.0743707090325,27.2212540717832,20.7914853567128));
#52439=CARTESIAN_POINT('Ctrl Pts',(54.2612048450082,27.1358840933454,20.8027859059759));
#52440=CARTESIAN_POINT('Ctrl Pts',(54.5104654921247,27.0654761840217,20.81834212755));
#52441=CARTESIAN_POINT('Ctrl Pts',(54.563751897701,27.0527678081384,20.8216843951475));
#52442=CARTESIAN_POINT('Ctrl Pts',(54.63146587729,27.0395375705888,20.8259842075171));
#52443=CARTESIAN_POINT('Ctrl Pts',(54.6454700426122,27.0369567428291,20.8268762063524));
#52444=CARTESIAN_POINT('Ctrl Pts',(54.6679545680287,27.0330615128253,20.8283132502221));
#52445=CARTESIAN_POINT('Ctrl Pts',(54.6764180295075,27.0316514826152,20.8288552757992));
#52446=CARTESIAN_POINT('Ctrl Pts',(54.6925101639894,27.0290770910995,20.8298880720088));
#52447=CARTESIAN_POINT('Ctrl Pts',(54.700137029478,27.0279023076273,20.8303785047201));
#52448=CARTESIAN_POINT('Ctrl Pts',(54.7175202640017,27.0253278992801,20.8314985278464));
#52449=CARTESIAN_POINT('Ctrl Pts',(54.7272805155149,27.0239562799208,20.8321289848006));
#52450=CARTESIAN_POINT('Ctrl Pts',(54.7526779736182,27.0205788932182,20.8337738285262));
#52451=CARTESIAN_POINT('Ctrl Pts',(54.7683292622009,27.0186861055289,20.8347917142158));
#52452=CARTESIAN_POINT('Ctrl Pts',(54.9138070400975,27.0028400510913,20.8442942080277));
#52453=CARTESIAN_POINT('Ctrl Pts',(55.0446634812681,27.0014828624549,20.8531784177598));
#52454=CARTESIAN_POINT('Ctrl Pts',(55.2684251834071,27.0211545405083,20.8687773625685));
#52455=CARTESIAN_POINT('Ctrl Pts',(55.3614586451128,27.0360169228024,20.8753775001902));
#52456=CARTESIAN_POINT('Ctrl Pts',(55.510221269787,27.0707144866618,20.8858697444773));
#52457=CARTESIAN_POINT('Ctrl Pts',(55.5667367503657,27.0865530578495,20.8898388362679));
#52458=CARTESIAN_POINT('Ctrl Pts',(55.6316273930924,27.107867034147,20.8943157484908));
#52459=CARTESIAN_POINT('Ctrl Pts',(55.6407560571719,27.1109388553363,20.8949436454975));
#52460=CARTESIAN_POINT('Ctrl Pts',(55.6547266615384,27.1157529269056,20.8959012745984));
#52461=CARTESIAN_POINT('Ctrl Pts',(55.659584555704,27.1174479425236,20.8962336464041));
#52462=CARTESIAN_POINT('Ctrl Pts',(55.6684913226914,27.1205943990513,20.89684183203));
#52463=CARTESIAN_POINT('Ctrl Pts',(55.6725420494519,27.122040135198,20.8971179632994));
#52464=CARTESIAN_POINT('Ctrl Pts',(55.6816452636787,27.1253223755439,20.8977374812206));
#52465=CARTESIAN_POINT('Ctrl Pts',(55.6866950131695,27.1271662055478,20.8980804320996));
#52466=CARTESIAN_POINT('Ctrl Pts',(55.7014995162723,27.1326397458753,20.8990839580816));
#52467=CARTESIAN_POINT('Ctrl Pts',(55.711233564339,27.1363254796112,20.8997413359285));
#52468=CARTESIAN_POINT('Ctrl Pts',(55.7882970131251,27.166196780996,20.9049296114878));
#52469=CARTESIAN_POINT('Ctrl Pts',(55.85419552537,27.1959493195657,20.9092689068439));
#52470=CARTESIAN_POINT('Ctrl Pts',(56.0085333695467,27.2759899920151,20.9195238182742));
#52471=CARTESIAN_POINT('Ctrl Pts',(56.0950222611976,27.3295876336119,20.9253539733489));
#52472=CARTESIAN_POINT('Ctrl Pts',(56.235903304666,27.432554949113,20.9355516547217));
#52473=CARTESIAN_POINT('Ctrl Pts',(56.2923476820771,27.4787580170933,20.9398573874958));
#52474=CARTESIAN_POINT('Ctrl Pts',(56.3778833095861,27.5569767433172,20.9468793420569));
#52475=CARTESIAN_POINT('Ctrl Pts',(56.4086831805226,27.587028019372,20.9495215011912));
#52476=CARTESIAN_POINT('Ctrl Pts',(56.4475872885617,27.6275237004495,20.9530267201318));
#52477=CARTESIAN_POINT('Ctrl Pts',(56.4565947282819,27.637086967064,20.9538506423045));
#52478=CARTESIAN_POINT('Ctrl Pts',(56.4711634773622,27.6528641094489,20.9552040773903));
#52479=CARTESIAN_POINT('Ctrl Pts',(56.476781538925,27.6590252173804,20.9557311777323));
#52480=CARTESIAN_POINT('Ctrl Pts',(56.487571456292,27.6710081399447,20.9567537102882));
#52481=CARTESIAN_POINT('Ctrl Pts',(56.4927481803061,27.6768253822508,20.9572489256947));
#52482=CARTESIAN_POINT('Ctrl Pts',(56.5046204741856,27.6903249873051,20.9583955019549));
#52483=CARTESIAN_POINT('Ctrl Pts',(56.5112914543566,27.6980285932985,20.9590478598907));
#52484=CARTESIAN_POINT('Ctrl Pts',(56.5326460480436,27.7230740057945,20.9611627735162));
#52485=CARTESIAN_POINT('Ctrl Pts',(56.5470920213188,27.7406151857018,20.962634875113));
#52486=CARTESIAN_POINT('Ctrl Pts',(56.6668547161944,27.8912091663019,20.9752016806785));
#52487=CARTESIAN_POINT('Ctrl Pts',(56.7550772698159,28.0369305422543,20.98698673135));
#52488=CARTESIAN_POINT('Ctrl Pts',(56.8532753195288,28.2585828905094,21.0038712842703));
#52489=CARTESIAN_POINT('Ctrl Pts',(56.8791022980351,28.3267209644896,21.0089216946339));
#52490=CARTESIAN_POINT('Ctrl Pts',(56.9082063151757,28.4183471899178,21.0154188183984));
#52491=CARTESIAN_POINT('Ctrl Pts',(56.9148757924548,28.4406949567341,21.0169808305956));
#52492=CARTESIAN_POINT('Ctrl Pts',(56.9254345576521,28.4784805634041,21.0195783612159));
#52493=CARTESIAN_POINT('Ctrl Pts',(56.929533607894,28.4938568851945,21.0206234023165));
#52494=CARTESIAN_POINT('Ctrl Pts',(56.9349977397196,28.5153857450806,21.0220683676396));
#52495=CARTESIAN_POINT('Ctrl Pts',(56.9365182146849,28.5214977162313,21.0224765487398));
#52496=CARTESIAN_POINT('Ctrl Pts',(56.9390572898854,28.5319145840581,21.0231686396929));
#52497=CARTESIAN_POINT('Ctrl Pts',(56.9400905576879,28.5362158266049,21.0234533727512));
#52498=CARTESIAN_POINT('Ctrl Pts',(56.942051661859,28.5445006760501,21.0239997708041));
#52499=CARTESIAN_POINT('Ctrl Pts',(56.9429815608248,28.5484837251296,21.024261557326));
#52500=CARTESIAN_POINT('Ctrl Pts',(56.9451859851918,28.5580588942474,21.024888784609));
#52501=CARTESIAN_POINT('Ctrl Pts',(56.9464486649457,28.5636537446015,21.0252535592312));
#52502=CARTESIAN_POINT('Ctrl Pts',(56.9509670883086,28.5840845236042,21.0265796028233));
#52503=CARTESIAN_POINT('Ctrl Pts',(56.9540775835192,28.5989525048917,21.0275330598609));
#52504=CARTESIAN_POINT('Ctrl Pts',(56.9830896585188,28.7459883773731,21.0368616299607));
#52505=CARTESIAN_POINT('Ctrl Pts',(56.9957161398604,28.8804422194785,21.04460795487));
#52506=CARTESIAN_POINT('Ctrl Pts',(56.9936358400592,29.1541944385792,21.0605099228372));
#52507=CARTESIAN_POINT('Ctrl Pts',(56.9780465592986,29.2927193188917,21.068640455057));
#52508=CARTESIAN_POINT('Ctrl Pts',(56.9443190271023,29.4460661045214,21.0783787188003));
#52509=CARTESIAN_POINT('Ctrl Pts',(56.9402155630594,29.46358924134,21.0795020776734));
#52510=CARTESIAN_POINT('Ctrl Pts',(56.9336121687649,29.4901628686293,21.0812227687045));
#52511=CARTESIAN_POINT('Ctrl Pts',(56.9312844431495,29.4992554975174,21.0818146036314));
#52512=CARTESIAN_POINT('Ctrl Pts',(56.9271251929072,29.5150380162726,21.082847369183));
#52513=CARTESIAN_POINT('Ctrl Pts',(56.9253227712924,29.5217354614298,21.083287358622));
#52514=CARTESIAN_POINT('Ctrl Pts',(56.9211981428157,29.5367493015338,21.08427764088));
#52515=CARTESIAN_POINT('Ctrl Pts',(56.9188568040183,29.5450602521618,21.0848285428376));
#52516=CARTESIAN_POINT('Ctrl Pts',(56.9124428303823,29.5672740573276,21.0863084641226));
#52517=CARTESIAN_POINT('Ctrl Pts',(56.9082726347894,29.5811479748371,21.087240618879));
#52518=CARTESIAN_POINT('Ctrl Pts',(56.8887435186629,29.6436421955234,21.0914758811401));
#52519=CARTESIAN_POINT('Ctrl Pts',(56.8716761341378,29.691704438567,21.0948339672078));
#52520=CARTESIAN_POINT('Ctrl Pts',(56.784530840852,29.9101744233413,21.1105795940926));
#52521=CARTESIAN_POINT('Ctrl Pts',(56.6928979618292,30.0710020284877,21.1236630514197));
#52522=CARTESIAN_POINT('Ctrl Pts',(56.5476231286222,30.259682878865,21.13997625934));
#52523=CARTESIAN_POINT('Ctrl Pts',(56.5129850168429,30.301082540889,21.1436169928867));
#52524=CARTESIAN_POINT('Ctrl Pts',(56.4703582781784,30.3480219929654,21.1477715592361));
#52525=CARTESIAN_POINT('Ctrl Pts',(56.4639592534428,30.3549686610402,21.1483871079318));
#52526=CARTESIAN_POINT('Ctrl Pts',(56.4540254875256,30.3656000540955,21.1493298951057));
#52527=CARTESIAN_POINT('Ctrl Pts',(56.4505256375328,30.3693169838959,21.1496596505769));
#52528=CARTESIAN_POINT('Ctrl Pts',(56.4440493781061,30.3761422439869,21.150265357755));
#52529=CARTESIAN_POINT('Ctrl Pts',(56.4410771928575,30.3792543663,21.1505416086872));
#52530=CARTESIAN_POINT('Ctrl Pts',(56.4343361275596,30.3862672376662,21.1511642854768));
#52531=CARTESIAN_POINT('Ctrl Pts',(56.4305614008705,30.3901622427088,21.151510254717));
#52532=CARTESIAN_POINT('Ctrl Pts',(56.4193398945117,30.4016472044408,21.1525309557542));
#52533=CARTESIAN_POINT('Ctrl Pts',(56.4118481249087,30.4091932109312,21.1532023242584));
#52534=CARTESIAN_POINT('Ctrl Pts',(56.3384606989584,30.4819391693019,21.1596861158934));
#52535=CARTESIAN_POINT('Ctrl Pts',(56.2681468515568,30.5425397558459,21.1651811678491));
#52536=CARTESIAN_POINT('Ctrl Pts',(56.1050740192947,30.6643685420558,21.1770795042808));
#52537=CARTESIAN_POINT('Ctrl Pts',(56.0109124953292,30.7231851296029,21.1834364628123));
#52538=CARTESIAN_POINT('Ctrl Pts',(55.8648789916884,30.7982941746864,21.1931463494728));
#52539=CARTESIAN_POINT('Ctrl Pts',(55.8164463283188,30.8207944358888,21.1963422083825));
#52540=CARTESIAN_POINT('Ctrl Pts',(55.7457636213967,30.8502437852368,21.2010135106738));
#52541=CARTESIAN_POINT('Ctrl Pts',(55.7242019409201,30.8587891023694,21.2024392984853));
#52542=CARTESIAN_POINT('Ctrl Pts',(55.685383805207,30.8733955591535,21.2050108168111));
#52543=CARTESIAN_POINT('Ctrl Pts',(55.6681835368932,30.879599055123,21.206151844966));
#52544=CARTESIAN_POINT('Ctrl Pts',(55.6419728613992,30.8886470329995,21.2078940796743));
#52545=CARTESIAN_POINT('Ctrl Pts',(55.6330232181185,30.8916655017306,21.2084895725686));
#52546=CARTESIAN_POINT('Ctrl Pts',(55.6167585579605,30.8970227776174,21.2095730390657));
#52547=CARTESIAN_POINT('Ctrl Pts',(55.6094507895989,30.8993831288064,21.2100602973306));
#52548=CARTESIAN_POINT('Ctrl Pts',(55.5936936120888,30.9043722742563,21.2111119919665));
#52549=CARTESIAN_POINT('Ctrl Pts',(55.5852400019251,30.9069871525526,21.2116768696042));
#52550=CARTESIAN_POINT('Ctrl Pts',(55.5623458925904,30.9139022117629,21.2132085711775));
#52551=CARTESIAN_POINT('Ctrl Pts',(55.5478738423156,30.918095099694,21.2141788403523));
#52552=CARTESIAN_POINT('Ctrl Pts',(55.4758598560546,30.9380777339457,21.2190180343386));
#52553=CARTESIAN_POINT('Ctrl Pts',(55.4176823693218,30.9514425735709,21.2229636508999));
#52554=CARTESIAN_POINT('Ctrl Pts',(55.2027368528984,30.9907687649775,21.2376791721169));
#52555=CARTESIAN_POINT('Ctrl Pts',(55.0436290404494,31.0005868376054,21.248892807459));
#52556=CARTESIAN_POINT('Ctrl Pts',(54.8387742540884,30.9887645837924,21.2630521102782));
#52557=CARTESIAN_POINT('Ctrl Pts',(54.7925792096729,30.9844786449024,21.2662215441081));
#52558=CARTESIAN_POINT('Ctrl Pts',(54.7292267383726,30.9763641429337,21.2705020917353));
#52559=CARTESIAN_POINT('Ctrl Pts',(54.7119099900578,30.973914277789,21.2716652488485));
#52560=CARTESIAN_POINT('Ctrl Pts',(54.682011235717,30.9692825311097,21.273659112919));
#52561=CARTESIAN_POINT('Ctrl Pts',(54.6694140520212,30.967207028434,21.2744947322004));
#52562=CARTESIAN_POINT('Ctrl Pts',(54.6511588324566,30.964018999523,21.2756983619489));
#52563=CARTESIAN_POINT('Ctrl Pts',(54.645484624748,30.9630027104846,21.2760714537769));
#52564=CARTESIAN_POINT('Ctrl Pts',(54.6355496212595,30.9611788008642,21.2767228046752));
#52565=CARTESIAN_POINT('Ctrl Pts',(54.6312869485221,30.9603818644855,21.2770016541657));
#52566=CARTESIAN_POINT('Ctrl Pts',(54.6222322648156,30.9586584492949,21.2775926429705));
#52567=CARTESIAN_POINT('Ctrl Pts',(54.6174410431473,30.9577282826023,21.2779045727925));
#52568=CARTESIAN_POINT('Ctrl Pts',(54.6044019053851,30.9551471714728,21.278751450841));
#52569=CARTESIAN_POINT('Ctrl Pts',(54.5961608295053,30.9534616056857,21.2792844868916));
#52570=CARTESIAN_POINT('Ctrl Pts',(54.5575005197377,30.9452992141314,21.2817756936754));
#52571=CARTESIAN_POINT('Ctrl Pts',(54.5272229866976,30.9381632972807,21.2836994738747));
#52572=CARTESIAN_POINT('Ctrl Pts',(54.2982074118985,30.8785013771913,21.2981278033037));
#52573=CARTESIAN_POINT('Ctrl Pts',(54.1084812608212,30.7962447791321,21.3094945107392));
#52574=CARTESIAN_POINT('Ctrl Pts',(53.8882665777907,30.6571321600984,21.3251372814889));
#52575=CARTESIAN_POINT('Ctrl Pts',(53.8431104881462,30.6259286693526,21.3284859164819));
#52576=CARTESIAN_POINT('Ctrl Pts',(53.7879223535345,30.5843289958351,21.3327929145874));
#52577=CARTESIAN_POINT('Ctrl Pts',(53.7766365262738,30.575630788828,21.3336854578911));
#52578=CARTESIAN_POINT('Ctrl Pts',(53.7587041306838,30.5615011301157,21.3351231710755));
#52579=CARTESIAN_POINT('Ctrl Pts',(53.7519976172571,30.5561462860208,21.3356653164279));
#52580=CARTESIAN_POINT('Ctrl Pts',(53.7393270762424,30.5458948493462,21.3366982057311));
#52581=CARTESIAN_POINT('Ctrl Pts',(53.7333564849006,30.5410065894931,21.3371886108393));
#52582=CARTESIAN_POINT('Ctrl Pts',(53.7198272671223,30.5297981606379,21.338308382274));
#52583=CARTESIAN_POINT('Ctrl Pts',(53.7122868492832,30.5234564234145,21.3389386136935));
#52584=CARTESIAN_POINT('Ctrl Pts',(53.692812799206,30.5068302362748,21.3405824818258));
#52585=CARTESIAN_POINT('Ctrl Pts',(53.6809536552743,30.4964599746932,21.3415996106325));
#52586=CARTESIAN_POINT('Ctrl Pts',(53.5713651742345,30.3983152004726,21.3511522218678));
#52587=CARTESIAN_POINT('Ctrl Pts',(53.4824253743957,30.3012449470915,21.3600924861554));
#52588=CARTESIAN_POINT('Ctrl Pts',(53.3462509420951,30.119515165601,21.3758650957462));
#52589=CARTESIAN_POINT('Ctrl Pts',(53.2944138081073,30.0388341798271,21.3825839074236));
#52590=CARTESIAN_POINT('Ctrl Pts',(53.2215933760939,29.9052484691171,21.3930211451163));
#52591=CARTESIAN_POINT('Ctrl Pts',(53.1967212984401,29.8546298071825,21.3968302890198));
#52592=CARTESIAN_POINT('Ctrl Pts',(53.1701829852911,29.7942847931287,21.4011505628708));
#52593=CARTESIAN_POINT('Ctrl Pts',(53.1664037569904,29.7855211430696,21.4017726547652));
#52594=CARTESIAN_POINT('Ctrl Pts',(53.1606913386702,29.7720087373195,21.4027233093546));
#52595=CARTESIAN_POINT('Ctrl Pts',(53.1587133781316,29.7672792318912,21.4030544537562));
#52596=CARTESIAN_POINT('Ctrl Pts',(53.1551090783361,29.7585667784494,21.403661470089));
#52597=CARTESIAN_POINT('Ctrl Pts',(53.1534773963189,29.7545862077781,21.4039376509376));
#52598=CARTESIAN_POINT('Ctrl Pts',(53.1498273654406,29.7455990362546,21.4045586212454));
#52599=CARTESIAN_POINT('Ctrl Pts',(53.1478164566483,29.7405895110753,21.4049029652995));
#52600=CARTESIAN_POINT('Ctrl Pts',(53.1419496953011,29.7258010202053,21.4059144015996));
#52601=CARTESIAN_POINT('Ctrl Pts',(53.1381507049136,29.7159994898052,21.4065782206326));
#52602=CARTESIAN_POINT('Ctrl Pts',(53.1067720770863,29.6331027315131,21.4121411816274));
#52603=CARTESIAN_POINT('Ctrl Pts',(53.0834276957116,29.5584663008516,21.4168158330767));
#52604=CARTESIAN_POINT('Ctrl Pts',(53.0580509838884,29.4567017169179,21.4229833679291));
#52605=CARTESIAN_POINT('Ctrl Pts',(53.0521056353475,29.4306381909294,21.4245451343344));
#52606=CARTESIAN_POINT('Ctrl Pts',(53.0466869889941,29.4044698301913,21.4261018347978));
#52607=CARTESIAN_POINT('Origin',(55.,29.,3.45145488139523));
#52608=CARTESIAN_POINT('',(53.0466870263011,29.4044700103589,22.3827843708292));
#52609=CARTESIAN_POINT('',(53.0466869980082,29.4044698737232,22.2235966764224));
#52610=CARTESIAN_POINT('',(53.0466869980082,29.4044698737233,3.45145488139523));
#52611=CARTESIAN_POINT('',(53.0052507292241,28.9982943508983,21.6101045922788));
#52612=CARTESIAN_POINT('Ctrl Pts',(53.0466870263011,29.4044700103589,22.3827843708292));
#52613=CARTESIAN_POINT('Ctrl Pts',(53.0598329847647,29.467955981039,22.3790005439717));
#52614=CARTESIAN_POINT('Ctrl Pts',(53.0760731107924,29.5307966436041,22.3752521208703));
#52615=CARTESIAN_POINT('Ctrl Pts',(53.130699039501,29.7063173768748,22.364540696809));
#52616=CARTESIAN_POINT('Ctrl Pts',(53.1761169485835,29.8164652051821,22.3575129973853));
#52617=CARTESIAN_POINT('Ctrl Pts',(53.2383853048394,29.9359443700092,22.3491524672674));
#52618=CARTESIAN_POINT('Ctrl Pts',(53.2458687742928,29.9498956882499,22.3481645272101));
#52619=CARTESIAN_POINT('Ctrl Pts',(53.2582890630588,29.9724032684934,22.3465508262489));
#52620=CARTESIAN_POINT('Ctrl Pts',(53.2631248606693,29.981014703867,22.3459286313328));
#52621=CARTESIAN_POINT('Ctrl Pts',(53.2718539702567,29.9962923533435,22.3448160484956));
#52622=CARTESIAN_POINT('Ctrl Pts',(53.275722431704,30.0029725909519,22.3443265560172));
#52623=CARTESIAN_POINT('Ctrl Pts',(53.2839670109837,30.0170210333699,22.3432907044636));
#52624=CARTESIAN_POINT('Ctrl Pts',(53.2883520209901,30.0243838118137,22.3427440317953));
#52625=CARTESIAN_POINT('Ctrl Pts',(53.3001241268624,30.0438634796229,22.341287487662));
#52626=CARTESIAN_POINT('Ctrl Pts',(53.3075932079485,30.0559300077317,22.3403746518494));
#52627=CARTESIAN_POINT('Ctrl Pts',(53.344189427374,30.1136664708123,22.3359546852019));
#52628=CARTESIAN_POINT('Ctrl Pts',(53.3750375524976,30.1582131837948,22.332384621682));
#52629=CARTESIAN_POINT('Ctrl Pts',(53.4710172058588,30.2854202573017,22.3217001467797));
#52630=CARTESIAN_POINT('Ctrl Pts',(53.5409134440939,30.3642417298118,22.3144228628248));
#52631=CARTESIAN_POINT('Ctrl Pts',(53.7032292166296,30.520473820879,22.2987262026748));
#52632=CARTESIAN_POINT('Ctrl Pts',(53.7971238529569,30.5957911056109,22.2903214106043));
#52633=CARTESIAN_POINT('Ctrl Pts',(53.9104264742239,30.6709601448555,22.2813162909636));
#52634=CARTESIAN_POINT('Ctrl Pts',(53.923724942976,30.6795565822045,22.2802759860643));
#52635=CARTESIAN_POINT('Ctrl Pts',(53.9425991770478,30.6914410756005,22.2788242979449));
#52636=CARTESIAN_POINT('Ctrl Pts',(53.9480903320249,30.6948614886845,22.2784048687356));
#52637=CARTESIAN_POINT('Ctrl Pts',(53.9573548542675,30.7005699437952,22.2777022379552));
#52638=CARTESIAN_POINT('Ctrl Pts',(53.9611193167372,30.7028722679239,22.2774181213302));
#52639=CARTESIAN_POINT('Ctrl Pts',(53.9688180553954,30.7075457415525,22.2768399390771));
#52640=CARTESIAN_POINT('Ctrl Pts',(53.9727529292902,30.7099158222335,22.2765459422578));
#52641=CARTESIAN_POINT('Ctrl Pts',(53.9828031578799,30.7159221326631,22.2757987951736));
#52642=CARTESIAN_POINT('Ctrl Pts',(53.9889299056617,30.7195393130044,22.2753468587109));
#52643=CARTESIAN_POINT('Ctrl Pts',(54.0139331669215,30.7341211899004,22.273516286604));
#52644=CARTESIAN_POINT('Ctrl Pts',(54.0329705240681,30.7448089252109,22.2721542844037));
#52645=CARTESIAN_POINT('Ctrl Pts',(54.0837093534366,30.7722085016365,22.2685971189489));
#52646=CARTESIAN_POINT('Ctrl Pts',(54.1156932339018,30.7883828914282,22.2664284319025));
#52647=CARTESIAN_POINT('Ctrl Pts',(54.3082560096138,30.879332532698,22.2537025173719));
#52648=CARTESIAN_POINT('Ctrl Pts',(54.4777784629726,30.9333113102216,22.2437695716354));
#52649=CARTESIAN_POINT('Ctrl Pts',(54.7088976602232,30.9742343312022,22.2297093038134));
#52650=CARTESIAN_POINT('Ctrl Pts',(54.7659883876497,30.981812151576,22.2262035533025));
#52651=CARTESIAN_POINT('Ctrl Pts',(54.838171971324,30.9882307411456,22.2216924231182));
#52652=CARTESIAN_POINT('Ctrl Pts',(54.853034718526,30.9893845726872,22.2207594768401));
#52653=CARTESIAN_POINT('Ctrl Pts',(54.8767015203862,30.9909552234435,22.2192667992507));
#52654=CARTESIAN_POINT('Ctrl Pts',(54.8854980024805,30.9914804807956,22.2187104448917));
#52655=CARTESIAN_POINT('Ctrl Pts',(54.9019695441293,30.9923545410491,22.2176656307446));
#52656=CARTESIAN_POINT('Ctrl Pts',(54.9096437231439,30.9927173226681,22.2171776153755));
#52657=CARTESIAN_POINT('Ctrl Pts',(54.9268055593143,30.9934292744804,22.2160834257242));
#52658=CARTESIAN_POINT('Ctrl Pts',(54.9362939495634,30.9937550583067,22.2154765357684));
#52659=CARTESIAN_POINT('Ctrl Pts',(54.964301834862,30.9945165732256,22.2136792152674));
#52660=CARTESIAN_POINT('Ctrl Pts',(54.982825076913,30.9947620669439,22.2124829240611));
#52661=CARTESIAN_POINT('Ctrl Pts',(55.1281424834146,30.994663825164,22.203035420841));
#52662=CARTESIAN_POINT('Ctrl Pts',(55.2546163816618,30.9824894065802,22.1944119596635));
#52663=CARTESIAN_POINT('Ctrl Pts',(55.5191926350764,30.9312792723567,22.1757062655652));
#52664=CARTESIAN_POINT('Ctrl Pts',(55.6560162689696,30.8891923875666,22.1656282796835));
#52665=CARTESIAN_POINT('Ctrl Pts',(55.8033839513498,30.8259005291532,22.1549802122286));
#52666=CARTESIAN_POINT('Ctrl Pts',(55.8194943662817,30.8187269037097,22.1538195818));
#52667=CARTESIAN_POINT('Ctrl Pts',(55.8416510031535,30.8085068189757,22.1522302229855));
#52668=CARTESIAN_POINT('Ctrl Pts',(55.8477794842616,30.8056420671445,22.1517913435245));
#52669=CARTESIAN_POINT('Ctrl Pts',(55.8575701313108,30.8010046040626,22.1510915223317));
#52670=CARTESIAN_POINT('Ctrl Pts',(55.8612415875257,30.7992518007796,22.1508293902107));
#52671=CARTESIAN_POINT('Ctrl Pts',(55.8689102892833,30.7955618067127,22.1502825300579));
#52672=CARTESIAN_POINT('Ctrl Pts',(55.8729064588538,30.7936224817755,22.1499979443256));
#52673=CARTESIAN_POINT('Ctrl Pts',(55.8826389460832,30.7888591149401,22.1493057096109));
#52674=CARTESIAN_POINT('Ctrl Pts',(55.8883682921963,30.7860207788114,22.1488989343593));
#52675=CARTESIAN_POINT('Ctrl Pts',(55.9088601551993,30.7757460424047,22.1474463174213));
#52676=CARTESIAN_POINT('Ctrl Pts',(55.9235442290236,30.7681535248846,22.146409651711));
#52677=CARTESIAN_POINT('Ctrl Pts',(55.9597788134409,30.7488435637173,22.143857977051));
#52678=CARTESIAN_POINT('Ctrl Pts',(55.9812112508956,30.7369092587347,22.1423543996137));
#52679=CARTESIAN_POINT('Ctrl Pts',(56.0709394941548,30.6847544206982,22.1360607951342));
#52680=CARTESIAN_POINT('Ctrl Pts',(56.1370309272559,30.6408752159367,22.1314262586001));
#52681=CARTESIAN_POINT('Ctrl Pts',(56.3278848816975,30.4970809228322,22.1175273258594));
#52682=CARTESIAN_POINT('Ctrl Pts',(56.4434140708205,30.3860300646697,22.1083386247208));
#52683=CARTESIAN_POINT('Ctrl Pts',(56.5594680228495,30.2440454127757,22.0970362813726));
#52684=CARTESIAN_POINT('Ctrl Pts',(56.5741412891131,30.2254258979602,22.0955631581706));
#52685=CARTESIAN_POINT('Ctrl Pts',(56.594183169545,30.1990398348524,22.0934857231678));
#52686=CARTESIAN_POINT('Ctrl Pts',(56.5998341341592,30.1914895055922,22.0928924074817));
#52687=CARTESIAN_POINT('Ctrl Pts',(56.610090211931,30.1775817135092,22.0918014329077));
#52688=CARTESIAN_POINT('Ctrl Pts',(56.6147117661703,30.1712365652968,22.0913044201152));
#52689=CARTESIAN_POINT('Ctrl Pts',(56.6240070450825,30.1583150566358,22.0902936535355));
#52690=CARTESIAN_POINT('Ctrl Pts',(56.6286785607081,30.1517372945556,22.0897798279951));
#52691=CARTESIAN_POINT('Ctrl Pts',(56.6401262896793,30.1354093087656,22.0885060036167));
#52692=CARTESIAN_POINT('Ctrl Pts',(56.6468555246192,30.1256266767992,22.0877442481267));
#52693=CARTESIAN_POINT('Ctrl Pts',(56.6717534052805,30.0887301610368,22.0848761133982));
#52694=CARTESIAN_POINT('Ctrl Pts',(56.689342205288,30.0612330177196,22.0827483988628));
#52695=CARTESIAN_POINT('Ctrl Pts',(56.7317742321882,29.9911679014684,22.0773477467103));
#52696=CARTESIAN_POINT('Ctrl Pts',(56.7557282234358,29.9480894243627,22.0740456113054));
#52697=CARTESIAN_POINT('Ctrl Pts',(56.8247812581386,29.8122959517584,22.0636991339926));
#52698=CARTESIAN_POINT('Ctrl Pts',(56.864306594491,29.7169442821764,22.0565118771273));
#52699=CARTESIAN_POINT('Ctrl Pts',(56.9145299129415,29.5630806498938,22.0452357551412));
#52700=CARTESIAN_POINT('Ctrl Pts',(56.9302951920905,29.5064046284258,22.0411498066037));
#52701=CARTESIAN_POINT('Ctrl Pts',(56.9547852154069,29.40042415409,22.0337127819011));
#52702=CARTESIAN_POINT('Ctrl Pts',(56.9642037359643,29.3513251287401,22.0303462325659));
#52703=CARTESIAN_POINT('Ctrl Pts',(56.9730978000059,29.2932400739027,22.026493773977));
#52704=CARTESIAN_POINT('Ctrl Pts',(56.9743695761721,29.2845513182708,22.0259209056333));
#52705=CARTESIAN_POINT('Ctrl Pts',(56.9763424442228,29.270422239856,22.0249951836858));
#52706=CARTESIAN_POINT('Ctrl Pts',(56.9770785309122,29.2649870354986,22.0246404756779));
#52707=CARTESIAN_POINT('Ctrl Pts',(56.978352657116,29.2552780443603,22.0240094375561));
#52708=CARTESIAN_POINT('Ctrl Pts',(56.978899279649,29.2510054939982,22.0237326386927));
#52709=CARTESIAN_POINT('Ctrl Pts',(56.9800577335877,29.241711646977,22.0231324914836));
#52710=CARTESIAN_POINT('Ctrl Pts',(56.9806643062082,29.2366897887507,22.0228094375814));
#52711=CARTESIAN_POINT('Ctrl Pts',(56.9823231906738,29.2225026688582,22.0219001235922));
#52712=CARTESIAN_POINT('Ctrl Pts',(56.9833310495227,29.2133321956124,22.0213162771984));
#52713=CARTESIAN_POINT('Ctrl Pts',(56.9893033866144,29.1552842938777,22.0176435710284));
#52714=CARTESIAN_POINT('Ctrl Pts',(56.9925248057147,29.1062400867935,22.0146432965894));
#52715=CARTESIAN_POINT('Ctrl Pts',(56.9979573651124,28.9166105992374,22.0032684818477));
#52716=CARTESIAN_POINT('Ctrl Pts',(56.9871193359043,28.7760591004324,21.9952902217953));
#52717=CARTESIAN_POINT('Ctrl Pts',(56.9443482811274,28.5444162561162,21.9814599410495));
#52718=CARTESIAN_POINT('Ctrl Pts',(56.9204592460025,28.4523872896624,21.9757819451573));
#52719=CARTESIAN_POINT('Ctrl Pts',(56.8851797956597,28.3478017195607,21.9689290241223));
#52720=CARTESIAN_POINT('Ctrl Pts',(56.8800806145646,28.333244931807,21.9679661213253));
#52721=CARTESIAN_POINT('Ctrl Pts',(56.8714822425185,28.309582077704,21.9663853069995));
#52722=CARTESIAN_POINT('Ctrl Pts',(56.8680840988328,28.3004397911743,21.9657707225438));
#52723=CARTESIAN_POINT('Ctrl Pts',(56.8618815063645,28.2841199853164,21.9646666009084));
#52724=CARTESIAN_POINT('Ctrl Pts',(56.8591022379137,28.2769330560418,21.9641779078969));
#52725=CARTESIAN_POINT('Ctrl Pts',(56.8531185358715,28.2617223405605,21.9631383056347));
#52726=CARTESIAN_POINT('Ctrl Pts',(56.8499034810511,28.2537029295486,21.96258704961));
#52727=CARTESIAN_POINT('Ctrl Pts',(56.8411490887477,28.2322707644579,21.9611051889312));
#52728=CARTESIAN_POINT('Ctrl Pts',(56.8355153987317,28.2188973506798,21.9601714345742));
#52729=CARTESIAN_POINT('Ctrl Pts',(56.8065643980926,28.1522157981566,21.9554689429363));
#52730=CARTESIAN_POINT('Ctrl Pts',(56.7810705427922,28.0998891415957,21.9516270768162));
#52731=CARTESIAN_POINT('Ctrl Pts',(56.6990530758438,27.9487150136528,21.9400637408719));
#52732=CARTESIAN_POINT('Ctrl Pts',(56.6363204513971,27.8535133798241,21.9321538107858));
#52733=CARTESIAN_POINT('Ctrl Pts',(56.4998455899081,27.6805940728614,21.9168006916445));
#52734=CARTESIAN_POINT('Ctrl Pts',(56.4272732596328,27.6024076848864,21.9093883189934));
#52735=CARTESIAN_POINT('Ctrl Pts',(56.3369298733133,27.5194914413605,21.9012638662573));
#52736=CARTESIAN_POINT('Ctrl Pts',(56.3249293585527,27.508742372175,21.9002051567743));
#52737=CARTESIAN_POINT('Ctrl Pts',(56.3078944002621,27.4938518519565,21.8987323655551));
#52738=CARTESIAN_POINT('Ctrl Pts',(56.3029682492781,27.4895882182928,21.8983099294069));
#52739=CARTESIAN_POINT('Ctrl Pts',(56.2949675216596,27.482731779217,21.8976295410589));
#52740=CARTESIAN_POINT('Ctrl Pts',(56.2919058874237,27.4801240462822,21.8973705155157));
#52741=CARTESIAN_POINT('Ctrl Pts',(56.2854087202918,27.4746239308153,21.896823695741));
#52742=CARTESIAN_POINT('Ctrl Pts',(56.2819712651923,27.4717338560896,21.8965360750329));
#52743=CARTESIAN_POINT('Ctrl Pts',(56.2734295870199,27.4646014527571,21.8958254507801));
#52744=CARTESIAN_POINT('Ctrl Pts',(56.2683138424793,27.4603728984157,21.8954034326054));
#52745=CARTESIAN_POINT('Ctrl Pts',(56.249104242892,27.4446554148857,21.8938316995477));
#52746=CARTESIAN_POINT('Ctrl Pts',(56.2348741166123,27.4333334244437,21.8926932577358));
#52747=CARTESIAN_POINT('Ctrl Pts',(56.1984435689165,27.4051528302748,21.8898378276753));
#52748=CARTESIAN_POINT('Ctrl Pts',(56.1760403984157,27.3885616301051,21.8881360860405));
#52749=CARTESIAN_POINT('Ctrl Pts',(56.0721190181157,27.3149222997963,21.8804494352355));
#52750=CARTESIAN_POINT('Ctrl Pts',(55.9867461779164,27.2635492924463,21.8746983888214));
#52751=CARTESIAN_POINT('Ctrl Pts',(55.7798689253882,27.1592663222408,21.8612439595537));
#52752=CARTESIAN_POINT('Ctrl Pts',(55.6562419831442,27.1116576282914,21.8535363897701));
#52753=CARTESIAN_POINT('Ctrl Pts',(55.5053468750363,27.0701697235569,21.8439024252603));
#52754=CARTESIAN_POINT('Ctrl Pts',(55.4817552474219,27.0641456248202,21.8423908980651));
#52755=CARTESIAN_POINT('Ctrl Pts',(55.4485251495608,27.0563053923958,21.8402518899577));
#52756=CARTESIAN_POINT('Ctrl Pts',(55.438973958947,27.0541260587233,21.8396359462226));
#52757=CARTESIAN_POINT('Ctrl Pts',(55.422351766823,27.0504619146785,21.8385618624199));
#52758=CARTESIAN_POINT('Ctrl Pts',(55.415287976312,27.0489449890971,21.838104749518));
#52759=CARTESIAN_POINT('Ctrl Pts',(55.4005282244063,27.0458591678138,21.837148148686));
#52760=CARTESIAN_POINT('Ctrl Pts',(55.3928309390589,27.0442972871621,21.8366484473059));
#52761=CARTESIAN_POINT('Ctrl Pts',(55.3745563030294,27.0407013616197,21.8354600157491));
#52762=CARTESIAN_POINT('Ctrl Pts',(55.3639713914206,27.0387074677042,21.834770029925));
#52763=CARTESIAN_POINT('Ctrl Pts',(55.3283634708023,27.032298134205,21.8324431422806));
#52764=CARTESIAN_POINT('Ctrl Pts',(55.3032732046244,27.0282752558391,21.8307939936068));
#52765=CARTESIAN_POINT('Ctrl Pts',(55.2431334100836,27.0198076868543,21.8268165612725));
#52766=CARTESIAN_POINT('Ctrl Pts',(55.2080301959714,27.0158128521791,21.8244750945022));
#52767=CARTESIAN_POINT('Ctrl Pts',(55.0703578944151,27.0038387858167,21.8152139911706));
#52768=CARTESIAN_POINT('Ctrl Pts',(54.9673496283287,27.0028671916453,21.8081052102771));
#52769=CARTESIAN_POINT('Ctrl Pts',(54.7416239791641,27.0182088185041,21.7923455960044));
#52770=CARTESIAN_POINT('Ctrl Pts',(54.61954221925,27.0379827645893,21.7837003415978));
#52771=CARTESIAN_POINT('Ctrl Pts',(54.4848223885558,27.0728603010286,21.7744850170074));
#52772=CARTESIAN_POINT('Ctrl Pts',(54.4696289384813,27.0769862287012,21.7734508041158));
#52773=CARTESIAN_POINT('Ctrl Pts',(54.4482777182078,27.0830566684888,21.772006126021));
#52774=CARTESIAN_POINT('Ctrl Pts',(54.4420785588406,27.0848517340103,21.7715877147889));
#52775=CARTESIAN_POINT('Ctrl Pts',(54.4316587535354,27.0879238423909,21.7708863113902));
#52776=CARTESIAN_POINT('Ctrl Pts',(54.4274334686279,27.0891848406086,21.7706024109387));
#52777=CARTESIAN_POINT('Ctrl Pts',(54.4188112020043,27.0917892462421,21.7700241894135));
#52778=CARTESIAN_POINT('Ctrl Pts',(54.4144146315422,27.0931338597171,21.7697299398412));
#52779=CARTESIAN_POINT('Ctrl Pts',(54.4032083999987,27.0966035004131,21.7689813552683));
#52780=CARTESIAN_POINT('Ctrl Pts',(54.3964053478848,27.0987498985961,21.7685282433718));
#52781=CARTESIAN_POINT('Ctrl Pts',(54.369571621524,27.1073746251021,21.7667457564929));
#52782=CARTESIAN_POINT('Ctrl Pts',(54.3496316992131,27.1141336456549,21.7654316957567));
#52783=CARTESIAN_POINT('Ctrl Pts',(54.2973124034251,27.1327968594876,21.7620023921236));
#52784=CARTESIAN_POINT('Ctrl Pts',(54.2651273887918,27.1452277918205,21.759911788675));
#52785=CARTESIAN_POINT('Ctrl Pts',(54.0871224263905,27.2193408557184,21.7483720451434));
#52786=CARTESIAN_POINT('Ctrl Pts',(53.9487243055471,27.2973790158574,21.7394425326835));
#52787=CARTESIAN_POINT('Ctrl Pts',(53.7596366433212,27.4359303293865,21.7255568693647));
#52788=CARTESIAN_POINT('Ctrl Pts',(53.7008995385378,27.484364414519,21.7209668128009));
#52789=CARTESIAN_POINT('Ctrl Pts',(53.6342533272438,27.5460464131429,21.7153234193134));
#52790=CARTESIAN_POINT('Ctrl Pts',(53.6235427051677,27.5561820391053,21.7144021865132));
#52791=CARTESIAN_POINT('Ctrl Pts',(53.6060844113694,27.5730739183128,21.7128761905145));
#52792=CARTESIAN_POINT('Ctrl Pts',(53.5992710086468,27.5797616402398,21.7122743729387));
#52793=CARTESIAN_POINT('Ctrl Pts',(53.5870590847981,27.5919216576817,21.7111841593285));
#52794=CARTESIAN_POINT('Ctrl Pts',(53.5816436576878,27.5973767678048,21.7106965213601));
#52795=CARTESIAN_POINT('Ctrl Pts',(53.571197290975,27.6080220448201,21.709747636686));
#52796=CARTESIAN_POINT('Ctrl Pts',(53.566162760002,27.6132085319105,21.7092865574761));
#52797=CARTESIAN_POINT('Ctrl Pts',(53.5524946308395,27.6274431974088,21.7080243475205));
#52798=CARTESIAN_POINT('Ctrl Pts',(53.5439178745069,27.6365452694837,21.7072207993786));
#52799=CARTESIAN_POINT('Ctrl Pts',(53.5076950252474,27.6757183165869,21.7037769947041));
#52800=CARTESIAN_POINT('Ctrl Pts',(53.4808922020602,27.7065522005325,21.7011018837599));
#52801=CARTESIAN_POINT('Ctrl Pts',(53.4121394175042,27.7907319018335,21.6938856302979));
#52802=CARTESIAN_POINT('Ctrl Pts',(53.3719353200296,27.8454289052491,21.6892832737757));
#52803=CARTESIAN_POINT('Ctrl Pts',(53.3004259960457,27.9538975417717,21.6803428151126));
#52804=CARTESIAN_POINT('Ctrl Pts',(53.2686931772748,28.0072974703124,21.6760205067402));
#52805=CARTESIAN_POINT('Ctrl Pts',(53.2065816110673,28.1238832709777,21.6668134307857));
#52806=CARTESIAN_POINT('Ctrl Pts',(53.1769351165128,28.1873714011938,21.6619332178443));
#52807=CARTESIAN_POINT('Ctrl Pts',(53.1317504450598,28.2991265983257,21.6536885513824));
#52808=CARTESIAN_POINT('Ctrl Pts',(53.1145976000471,28.3466710915223,21.6502838892133));
#52809=CARTESIAN_POINT('Ctrl Pts',(53.096595283424,28.4032122476348,21.646393462868));
#52810=CARTESIAN_POINT('Ctrl Pts',(53.0939787288689,28.4116225214854,21.6458188371866));
#52811=CARTESIAN_POINT('Ctrl Pts',(53.089820956718,28.4253055112258,21.6448908444411));
#52812=CARTESIAN_POINT('Ctrl Pts',(53.0882456951202,28.4305676402481,21.6445356084347));
#52813=CARTESIAN_POINT('Ctrl Pts',(53.0854737665576,28.4399683735514,21.6439040006906));
#52814=CARTESIAN_POINT('Ctrl Pts',(53.0842687534931,28.4441044041449,21.6436271566926));
#52815=CARTESIAN_POINT('Ctrl Pts',(53.0816796105856,28.4530996686802,21.6430273374766));
#52816=CARTESIAN_POINT('Ctrl Pts',(53.0803005409883,28.4579602622801,21.6427046539598));
#52817=CARTESIAN_POINT('Ctrl Pts',(53.0764629770322,28.4716842927374,21.6417974368092));
#52818=CARTESIAN_POINT('Ctrl Pts',(53.0740472608403,28.4805597055689,21.6412152991928));
#52819=CARTESIAN_POINT('Ctrl Pts',(53.0687452361623,28.5005851011892,21.6399114381129));
#52820=CARTESIAN_POINT('Ctrl Pts',(53.0658939032587,28.5117440996214,21.6391915435963));
#52821=CARTESIAN_POINT('Ctrl Pts',(53.0248278849474,28.6784674989925,21.6285265107986));
#52822=CARTESIAN_POINT('Ctrl Pts',(53.0053877304754,28.8380719780943,21.6194559710624));
#52823=CARTESIAN_POINT('Ctrl Pts',(53.0052507292241,28.9982943508983,21.6101045922788));
#52824=CARTESIAN_POINT('Ctrl Pts',(53.0052507279944,28.9982957896247,21.6101045083075));
#52825=CARTESIAN_POINT('Ctrl Pts',(53.0051543369249,29.111119897792,21.6035195283877));
#52826=CARTESIAN_POINT('Ctrl Pts',(53.0146297098485,29.2237376212089,21.5968303826914));
#52827=CARTESIAN_POINT('Ctrl Pts',(53.0356382363993,29.3470761145801,21.5890638196957));
#52828=CARTESIAN_POINT('Ctrl Pts',(53.0378165173038,29.3591864938383,21.5882966432258));
#52829=CARTESIAN_POINT('Ctrl Pts',(53.0416896620939,29.3796320814841,21.5869932937447));
#52830=CARTESIAN_POINT('Ctrl Pts',(53.043326067099,29.387978109682,21.5864589521394));
#52831=CARTESIAN_POINT('Ctrl Pts',(53.0455671781555,29.3990333444643,21.5857480115283));
#52832=CARTESIAN_POINT('Ctrl Pts',(53.0461242535664,29.401752202751,21.5855729141647));
#52833=CARTESIAN_POINT('Ctrl Pts',(53.0466869980088,29.4044698737264,21.5853976382171));
#52834=CARTESIAN_POINT('Ctrl Pts',(53.0466869889941,29.4044698301913,21.4261018347978));
#52835=CARTESIAN_POINT('Ctrl Pts',(53.0326898260591,29.3368730938287,21.4301230217525));
#52836=CARTESIAN_POINT('Ctrl Pts',(53.0222071592501,29.2685769241553,21.4341119456716));
#52837=CARTESIAN_POINT('Ctrl Pts',(53.0053974029733,29.101643606587,21.4439176190189));
#52838=CARTESIAN_POINT('Ctrl Pts',(53.0028121123142,29.0028444611566,21.4497733469691));
#52839=CARTESIAN_POINT('Ctrl Pts',(53.0086640626487,28.881050474017,21.4572921980709));
#52840=CARTESIAN_POINT('Ctrl Pts',(53.0101852158744,28.8578561986267,21.4587370814236));
#52841=CARTESIAN_POINT('Ctrl Pts',(53.0129727323458,28.8243347891428,21.4608463566309));
#52842=CARTESIAN_POINT('Ctrl Pts',(53.0139151663532,28.8139821090879,21.4615006914772));
#52843=CARTESIAN_POINT('Ctrl Pts',(53.0157054367892,28.7958839713239,21.4626498665838));
#52844=CARTESIAN_POINT('Ctrl Pts',(53.0165178200337,28.788135171123,21.4631435918216));
#52845=CARTESIAN_POINT('Ctrl Pts',(53.0182923695322,28.7721145532399,21.46416797403));
#52846=CARTESIAN_POINT('Ctrl Pts',(53.0192609792212,28.7638436161743,21.4646988232406));
#52847=CARTESIAN_POINT('Ctrl Pts',(53.0218851739499,28.7425886129283,21.4660682668944));
#52848=CARTESIAN_POINT('Ctrl Pts',(53.0236167993391,28.7296145012734,21.4669092235009));
#52849=CARTESIAN_POINT('Ctrl Pts',(53.030957964626,28.6784560454844,21.4702457186156));
#52850=CARTESIAN_POINT('Ctrl Pts',(53.037547178178,28.6404229796717,21.4727716231307));
#52851=CARTESIAN_POINT('Ctrl Pts',(53.0806777163801,28.4282650601508,21.487126918388));
#52852=CARTESIAN_POINT('Ctrl Pts',(53.1392826006906,28.2594675373326,21.4996600711593));
#52853=CARTESIAN_POINT('Ctrl Pts',(53.2500330016433,28.0401866019628,21.5166520829093));
#52854=CARTESIAN_POINT('Ctrl Pts',(53.2836751641037,27.9812472549074,21.5212854254095));
#52855=CARTESIAN_POINT('Ctrl Pts',(53.3280019545623,27.9120403227734,21.5267146822501));
#52856=CARTESIAN_POINT('Ctrl Pts',(53.3358766949517,27.9000330108804,21.527656162949));
#52857=CARTESIAN_POINT('Ctrl Pts',(53.3472499933094,27.8830928796436,21.5289825604316));
#52858=CARTESIAN_POINT('Ctrl Pts',(53.3506421653916,27.8780896489335,21.5293740750825));
#52859=CARTESIAN_POINT('Ctrl Pts',(53.356530579013,27.8694890557082,21.5300465801928));
#52860=CARTESIAN_POINT('Ctrl Pts',(53.3590160020726,27.8658843740917,21.5303282827753));
#52861=CARTESIAN_POINT('Ctrl Pts',(53.3638848491774,27.8588724591405,21.5308759132449));
#52862=CARTESIAN_POINT('Ctrl Pts',(53.3662670632256,27.8554644857747,21.5311419225735));
#52863=CARTESIAN_POINT('Ctrl Pts',(53.3728165779378,27.846156924004,21.5318680775835));
#52864=CARTESIAN_POINT('Ctrl Pts',(53.377005342635,27.8402724117119,21.5323267910038));
#52865=CARTESIAN_POINT('Ctrl Pts',(53.3933614059699,27.817557061976,21.5340965727038));
#52866=CARTESIAN_POINT('Ctrl Pts',(53.4057597841301,27.8008932127253,21.5353928621875));
#52867=CARTESIAN_POINT('Ctrl Pts',(53.5035691672887,27.6736335033382,21.5453027078332));
#52868=CARTESIAN_POINT('Ctrl Pts',(53.6001387647533,27.5720812053738,21.5532912755637));
#52869=CARTESIAN_POINT('Ctrl Pts',(53.8037562360298,27.3986458058006,21.5688512959098));
#52870=CARTESIAN_POINT('Ctrl Pts',(53.9086817374746,27.3253798759876,21.5763673221513));
#52871=CARTESIAN_POINT('Ctrl Pts',(54.0349432554034,27.2541500260347,21.5853661824784));
#52872=CARTESIAN_POINT('Ctrl Pts',(54.050115343245,27.2458489912622,21.5864463430546));
#52873=CARTESIAN_POINT('Ctrl Pts',(54.0735558311548,27.2334173848938,21.5881142769111));
#52874=CARTESIAN_POINT('Ctrl Pts',(54.0817484454076,27.2291451183499,21.588697065626));
#52875=CARTESIAN_POINT('Ctrl Pts',(54.0967313600687,27.2214637893646,21.5897627265298));
#52876=CARTESIAN_POINT('Ctrl Pts',(54.1035120547547,27.2180362938999,21.5902449439673));
#52877=CARTESIAN_POINT('Ctrl Pts',(54.1183588435381,27.2106377495471,21.5913007431632));
#52878=CARTESIAN_POINT('Ctrl Pts',(54.1264325046708,27.2066823430086,21.5918748543908));
#52879=CARTESIAN_POINT('Ctrl Pts',(54.1486670559882,27.1959750844159,21.5934559993439));
#52880=CARTESIAN_POINT('Ctrl Pts',(54.1628810508908,27.1893356137982,21.5944668621273));
#52881=CARTESIAN_POINT('Ctrl Pts',(54.2394653392656,27.1546570023187,21.5999149482736));
#52882=CARTESIAN_POINT('Ctrl Pts',(54.3031615134258,27.1296743463669,21.6044541979121));
#52883=CARTESIAN_POINT('Ctrl Pts',(54.5254893990466,27.0554088775765,21.6203265488493));
#52884=CARTESIAN_POINT('Ctrl Pts',(54.6888980684427,27.0226784634631,21.6321034574298));
#52885=CARTESIAN_POINT('Ctrl Pts',(54.8894471260371,27.0080069514659,21.6458650583217));
#52886=CARTESIAN_POINT('Ctrl Pts',(54.9244982428272,27.006370642205,21.6482419143026));
#52887=CARTESIAN_POINT('Ctrl Pts',(54.9740456268257,27.0053663536532,21.6515463258986));
#52888=CARTESIAN_POINT('Ctrl Pts',(54.9885182770832,27.005230537293,21.6525048464667));
#52889=CARTESIAN_POINT('Ctrl Pts',(55.0140059888009,27.0052687618697,21.6541796672458));
#52890=CARTESIAN_POINT('Ctrl Pts',(55.0250203785965,27.0053765082341,21.6548990831112));
#52891=CARTESIAN_POINT('Ctrl Pts',(55.0414623546451,27.0056735681967,21.6559659579855));
#52892=CARTESIAN_POINT('Ctrl Pts',(55.046890758797,27.0057938166122,21.6563170447705));
#52893=CARTESIAN_POINT('Ctrl Pts',(55.0562084738759,27.0060382875121,21.6569176286165));
#52894=CARTESIAN_POINT('Ctrl Pts',(55.0600979741194,27.006151726476,21.6571677149568));
#52895=CARTESIAN_POINT('Ctrl Pts',(55.0689203370409,27.006434874318,21.6577335643256));
#52896=CARTESIAN_POINT('Ctrl Pts',(55.0738529119217,27.0066115100507,21.6580489398408));
#52897=CARTESIAN_POINT('Ctrl Pts',(55.087218429008,27.0071398080612,21.6589009331939));
#52898=CARTESIAN_POINT('Ctrl Pts',(55.095649990006,27.0075266916801,21.6594356439555));
#52899=CARTESIAN_POINT('Ctrl Pts',(55.136504050019,27.0096612198826,21.6620142101926));
#52900=CARTESIAN_POINT('Ctrl Pts',(55.168885068367,27.0121469044711,21.6640204171014));
#52901=CARTESIAN_POINT('Ctrl Pts',(55.404232352239,27.0360060032627,21.6784206717914));
#52902=CARTESIAN_POINT('Ctrl Pts',(55.6029251026515,27.0876252512724,21.6897151636601));
#52903=CARTESIAN_POINT('Ctrl Pts',(55.8406180259541,27.1901970622447,21.7052634624077));
#52904=CARTESIAN_POINT('Ctrl Pts',(55.8899706301136,27.2139493837507,21.7086051396365));
#52905=CARTESIAN_POINT('Ctrl Pts',(55.9508463435213,27.246397552357,21.7129042856659));
#52906=CARTESIAN_POINT('Ctrl Pts',(55.9633394991137,27.2532294637553,21.7137962338686));
#52907=CARTESIAN_POINT('Ctrl Pts',(55.9832415624452,27.2643914012693,21.7152332154343));
#52908=CARTESIAN_POINT('Ctrl Pts',(55.9906976796374,27.2686365829308,21.7157752298101));
#52909=CARTESIAN_POINT('Ctrl Pts',(56.004807414227,27.2767910245874,21.716808017208));
#52910=CARTESIAN_POINT('Ctrl Pts',(56.0114662027884,27.2806910601878,21.7172984523943));
#52911=CARTESIAN_POINT('Ctrl Pts',(56.0265781343705,27.2896602539413,21.7184184986742));
#52912=CARTESIAN_POINT('Ctrl Pts',(56.035016619846,27.2947535943949,21.7190489764413));
#52913=CARTESIAN_POINT('Ctrl Pts',(56.0568541695821,27.3081562126981,21.7206939104042));
#52914=CARTESIAN_POINT('Ctrl Pts',(56.0701928740682,27.316562051885,21.7217118661511));
#52915=CARTESIAN_POINT('Ctrl Pts',(56.193079677447,27.396054116401,21.7312155434476));
#52916=CARTESIAN_POINT('Ctrl Pts',(56.2954785588323,27.4775659943593,21.7401009757547));
#52917=CARTESIAN_POINT('Ctrl Pts',(56.4555243147278,27.6328763654893,21.7555882373448));
#52918=CARTESIAN_POINT('Ctrl Pts',(56.5173263503175,27.7018092581273,21.76207309058));
#52919=CARTESIAN_POINT('Ctrl Pts',(56.611082256705,27.8222640172783,21.7725658297789));
#52920=CARTESIAN_POINT('Ctrl Pts',(56.6458770911098,27.8713998997048,21.7766407568717));
#52921=CARTESIAN_POINT('Ctrl Pts',(56.6836345385913,27.9301887422015,21.7812209328473));
#52922=CARTESIAN_POINT('Ctrl Pts',(56.6888096997353,27.9383770942622,21.7818524659045));
#52923=CARTESIAN_POINT('Ctrl Pts',(56.6966482951519,27.9509820228463,21.7828144609058));
#52924=CARTESIAN_POINT('Ctrl Pts',(56.6993545047949,27.9553716343531,21.7831475991763));
#52925=CARTESIAN_POINT('Ctrl Pts',(56.7042863298049,27.9634411918571,21.7837565209236));
#52926=CARTESIAN_POINT('Ctrl Pts',(56.7065170632049,27.9671178332437,21.7840326271597));
#52927=CARTESIAN_POINT('Ctrl Pts',(56.7115025998036,27.9753951169,21.7846512645056));
#52928=CARTESIAN_POINT('Ctrl Pts',(56.7142507477354,27.9799996612229,21.7849933657298));
#52929=CARTESIAN_POINT('Ctrl Pts',(56.7212446230271,27.9918260618727,21.7858669626214));
#52930=CARTESIAN_POINT('Ctrl Pts',(56.7254635340341,27.9990637681063,21.7863967895636));
#52931=CARTESIAN_POINT('Ctrl Pts',(56.7506730196657,28.042944700352,21.7895814181753));
#52932=CARTESIAN_POINT('Ctrl Pts',(56.7705428915108,28.0802232244211,21.7921711936333));
#52933=CARTESIAN_POINT('Ctrl Pts',(56.8014196790028,28.1428671715307,21.7963814635769));
#52934=CARTESIAN_POINT('Ctrl Pts',(56.8131087773977,28.1678784872796,21.7980264448393));
#52935=CARTESIAN_POINT('Ctrl Pts',(56.8437140475889,28.2370744009187,21.8025003474452));
#52936=CARTESIAN_POINT('Ctrl Pts',(56.8615587982408,28.2817130944537,21.805302308808));
#52937=CARTESIAN_POINT('Ctrl Pts',(56.9159862333013,28.433563677902,21.8146800581273));
#52938=CARTESIAN_POINT('Ctrl Pts',(56.9450476328063,28.5432273704115,21.8212138781943));
#52939=CARTESIAN_POINT('Ctrl Pts',(56.9746896007058,28.7119107011216,21.8314772757107));
#52940=CARTESIAN_POINT('Ctrl Pts',(56.9822330190645,28.7694663422195,21.8350128058286));
#52941=CARTESIAN_POINT('Ctrl Pts',(56.9885125258223,28.8417099940911,21.8395304752656));
#52942=CARTESIAN_POINT('Ctrl Pts',(56.9896105291314,28.8561677495695,21.8404384778559));
#52943=CARTESIAN_POINT('Ctrl Pts',(56.9911109417793,28.8792548929383,21.8418951966982));
#52944=CARTESIAN_POINT('Ctrl Pts',(56.9916150896518,28.8878773250058,21.8424407429929));
#52945=CARTESIAN_POINT('Ctrl Pts',(56.9924630437307,28.9041983047796,21.8434763342679));
#52946=CARTESIAN_POINT('Ctrl Pts',(56.9928182679779,28.9118961207521,21.8439660144987));
#52947=CARTESIAN_POINT('Ctrl Pts',(56.9935221909096,28.9293455529221,21.8450789234196));
#52948=CARTESIAN_POINT('Ctrl Pts',(56.9938439551319,28.9390980003042,21.845702977621));
#52949=CARTESIAN_POINT('Ctrl Pts',(56.9944900081758,28.9642856427506,21.8473201914177));
#52950=CARTESIAN_POINT('Ctrl Pts',(56.9947066745876,28.9797227150708,21.8483166590519));
#52951=CARTESIAN_POINT('Ctrl Pts',(56.9949757611202,29.0906323886909,21.8555154645358));
#52952=CARTESIAN_POINT('Ctrl Pts',(56.9883530580062,29.1859835505098,21.8619240371279));
#52953=CARTESIAN_POINT('Ctrl Pts',(56.9552288061438,29.41921775728,21.8780997667597));
#52954=CARTESIAN_POINT('Ctrl Pts',(56.9209633799058,29.5554822622232,21.888008849744));
#52955=CARTESIAN_POINT('Ctrl Pts',(56.8558056995437,29.7330893207081,21.9009298231738));
#52956=CARTESIAN_POINT('Ctrl Pts',(56.837212222332,29.7785158201695,21.9042311120878));
#52957=CARTESIAN_POINT('Ctrl Pts',(56.813154748049,29.8316143759536,21.9080490748728));
#52958=CARTESIAN_POINT('Ctrl Pts',(56.8092905560906,29.8399882750129,21.9086499398049));
#52959=CARTESIAN_POINT('Ctrl Pts',(56.8032174362263,29.8529126679774,21.9095750484779));
#52960=CARTESIAN_POINT('Ctrl Pts',(56.8010491032363,29.8574819360236,21.9099016665574));
#52961=CARTESIAN_POINT('Ctrl Pts',(56.7970018776368,29.8659274616107,21.9105044754199));
#52962=CARTESIAN_POINT('Ctrl Pts',(56.7951278198106,29.8698058565635,21.9107809433718));
#52963=CARTESIAN_POINT('Ctrl Pts',(56.7908384823345,29.8786098027946,21.9114077393708));
#52964=CARTESIAN_POINT('Ctrl Pts',(56.7884154408008,29.8835314755013,21.9117575841526));
#52965=CARTESIAN_POINT('Ctrl Pts',(56.7820596900496,29.8963079748639,21.9126644892759));
#52966=CARTESIAN_POINT('Ctrl Pts',(56.7780952955702,29.9041470296405,21.9132196587441));
#52967=CARTESIAN_POINT('Ctrl Pts',(56.7512034424082,29.9564610416247,21.9169177992159));
#52968=CARTESIAN_POINT('Ctrl Pts',(56.7266592536226,30.0000899763826,21.9199691089865));
#52969=CARTESIAN_POINT('Ctrl Pts',(56.6698072448161,30.092802913023,21.9264812092313));
#52970=CARTESIAN_POINT('Ctrl Pts',(56.6369203194908,30.1414758019681,21.9299184786696));
#52971=CARTESIAN_POINT('Ctrl Pts',(56.5405308079826,30.2713813356631,21.9393362646317));
#52972=CARTESIAN_POINT('Ctrl Pts',(56.472811461787,30.3492484060225,21.9452702183037));
#52973=CARTESIAN_POINT('Ctrl Pts',(56.3642486454867,30.4561193619647,21.9543070540327));
#52974=CARTESIAN_POINT('Ctrl Pts',(56.3278483059836,30.4893879037489,21.9572673837152));
#52975=CARTESIAN_POINT('Ctrl Pts',(56.2735121908096,30.5354726392185,21.9616213179429));
#52976=CARTESIAN_POINT('Ctrl Pts',(56.256536716552,30.5493950270616,21.9629728157528));
#52977=CARTESIAN_POINT('Ctrl Pts',(56.2256194625723,30.5739094309909,21.9654214623042));
#52978=CARTESIAN_POINT('Ctrl Pts',(56.2117613254909,30.5846035541081,21.9665145448715));
#52979=CARTESIAN_POINT('Ctrl Pts',(56.1903408615432,30.6006880963543,21.9681982721597));
#52980=CARTESIAN_POINT('Ctrl Pts',(56.182878421693,30.6062105662989,21.9687837813924));
#52981=CARTESIAN_POINT('Ctrl Pts',(56.1692377802098,30.6161585091717,21.9698522503255));
#52982=CARTESIAN_POINT('Ctrl Pts',(56.163072288097,30.6206011734851,21.9703345368431));
#52983=CARTESIAN_POINT('Ctrl Pts',(56.1495888541343,30.6302003463717,21.97138791928));
#52984=CARTESIAN_POINT('Ctrl Pts',(56.1422613110252,30.6353430208707,21.9719595280313));
#52985=CARTESIAN_POINT('Ctrl Pts',(56.1221368617105,30.6492656765441,21.9735272362233));
#52986=CARTESIAN_POINT('Ctrl Pts',(56.1092719287055,30.6579457693105,21.9745270586532));
#52987=CARTESIAN_POINT('Ctrl Pts',(56.0412036294163,30.702725192572,21.9798059464523));
#52988=CARTESIAN_POINT('Ctrl Pts',(55.9843417605355,30.7362165005147,21.9841796263484));
#52989=CARTESIAN_POINT('Ctrl Pts',(55.7766837935421,30.8450425765089,22.000031335567));
#52990=CARTESIAN_POINT('Ctrl Pts',(55.6181520175082,30.9040212223296,22.0119854499516));
#52991=CARTESIAN_POINT('Ctrl Pts',(55.4197768690426,30.950399451454,22.0259298360871));
#52992=CARTESIAN_POINT('Ctrl Pts',(55.3852364749688,30.9575146973316,22.0283189908872));
#52993=CARTESIAN_POINT('Ctrl Pts',(55.329281000868,30.9675027867316,22.0321093197401));
#52994=CARTESIAN_POINT('Ctrl Pts',(55.3079770997849,30.9709498701211,22.0335338666503));
#52995=CARTESIAN_POINT('Ctrl Pts',(55.2796099601323,30.9750686103723,22.0354025085003));
#52996=CARTESIAN_POINT('Ctrl Pts',(55.2725939745955,30.9760491578249,22.0358623920578));
#52997=CARTESIAN_POINT('Ctrl Pts',(55.2610269212721,30.9776029800429,22.0366166649311));
#52998=CARTESIAN_POINT('Ctrl Pts',(55.2564789058193,30.9781979608235,22.0369122375321));
#52999=CARTESIAN_POINT('Ctrl Pts',(55.2475470559683,30.9793351228833,22.0374907014316));
#53000=CARTESIAN_POINT('Ctrl Pts',(55.2431634162335,30.9798784374832,22.0377736514599));
#53001=CARTESIAN_POINT('Ctrl Pts',(55.2323315595517,30.9811844359558,22.0384705395914));
#53002=CARTESIAN_POINT('Ctrl Pts',(55.2258812838997,30.9819302135095,22.0388835424001));
#53003=CARTESIAN_POINT('Ctrl Pts',(55.2035451186552,30.984402248269,22.0403071781012));
#53004=CARTESIAN_POINT('Ctrl Pts',(55.1876417267717,30.9859691634881,22.0413094073121));
#53005=CARTESIAN_POINT('Ctrl Pts',(55.0575696636511,30.9972083091225,22.0494260045621));
#53006=CARTESIAN_POINT('Ctrl Pts',(54.9427650930077,30.9972196809258,22.0560912670462));
#53007=CARTESIAN_POINT('Ctrl Pts',(54.7210883157731,30.9780992741398,22.0690161452696));
#53008=CARTESIAN_POINT('Ctrl Pts',(54.6145308213104,30.9601224604578,22.0752581106597));
#53009=CARTESIAN_POINT('Ctrl Pts',(54.4738224377186,30.9244620008916,22.0839660105202));
#53010=CARTESIAN_POINT('Ctrl Pts',(54.4379574464821,30.9142948421327,22.0862263253102));
#53011=CARTESIAN_POINT('Ctrl Pts',(54.3771407039134,30.8951978241047,22.0901442301412));
#53012=CARTESIAN_POINT('Ctrl Pts',(54.3520429829838,30.8867644520071,22.0917863258965));
#53013=CARTESIAN_POINT('Ctrl Pts',(54.3168154391487,30.87414147518,22.0941304510988));
#53014=CARTESIAN_POINT('Ctrl Pts',(54.3065402083608,30.870363847745,22.0948189646843));
#53015=CARTESIAN_POINT('Ctrl Pts',(54.2889178145575,30.8637199028417,22.0960082596749));
#53016=CARTESIAN_POINT('Ctrl Pts',(54.2815555243378,30.8608942160159,22.096507685885));
#53017=CARTESIAN_POINT('Ctrl Pts',(54.2675152332534,30.8554097369493,22.0974651112245));
#53018=CARTESIAN_POINT('Ctrl Pts',(54.2608344558986,30.8527583549089,22.0979228566811));
#53019=CARTESIAN_POINT('Ctrl Pts',(54.2435299184012,30.8457822581777,22.0991142418413));
#53020=CARTESIAN_POINT('Ctrl Pts',(54.2329289887807,30.8414019614572,22.0998497347644));
#53021=CARTESIAN_POINT('Ctrl Pts',(54.2025837339469,30.8285558125094,22.1019716358125));
#53022=CARTESIAN_POINT('Ctrl Pts',(54.1829381086179,30.8198623209147,22.1033656560979));
#53023=CARTESIAN_POINT('Ctrl Pts',(54.0201399059574,30.7446541950829,22.1150918315081));
#53024=CARTESIAN_POINT('Ctrl Pts',(53.8852323302802,30.6616915009662,22.1260115949719));
#53025=CARTESIAN_POINT('Ctrl Pts',(53.6727900266267,30.4934381365881,22.1448987434276));
#53026=CARTESIAN_POINT('Ctrl Pts',(53.5901777376367,30.415715615389,22.1527751135213));
#53027=CARTESIAN_POINT('Ctrl Pts',(53.5071420683006,30.3230750550441,22.1609522652364));
#53028=CARTESIAN_POINT('Ctrl Pts',(53.4997542731274,30.3146920469187,22.1616822072969));
#53029=CARTESIAN_POINT('Ctrl Pts',(53.4888608886134,30.3021197998366,22.1627615601897));
#53030=CARTESIAN_POINT('Ctrl Pts',(53.4853015829056,30.2979776939723,22.1631147213075));
#53031=CARTESIAN_POINT('Ctrl Pts',(53.4789665206678,30.2905437833259,22.1637441026496));
#53032=CARTESIAN_POINT('Ctrl Pts',(53.4761843765348,30.2872575689229,22.1640207812985));
#53033=CARTESIAN_POINT('Ctrl Pts',(53.4701454677765,30.2800775131251,22.1646219337992));
#53034=CARTESIAN_POINT('Ctrl Pts',(53.4668929222065,30.2761802454073,22.1649461050142));
#53035=CARTESIAN_POINT('Ctrl Pts',(53.4578809613239,30.2652977496979,22.1658455313301));
#53036=CARTESIAN_POINT('Ctrl Pts',(53.4521540844598,30.258285561355,22.1664185085655));
#53037=CARTESIAN_POINT('Ctrl Pts',(53.4212013058256,30.2198547828103,22.1695246459531));
#53038=CARTESIAN_POINT('Ctrl Pts',(53.3968821353645,30.1877140351431,22.171999200276));
#53039=CARTESIAN_POINT('Ctrl Pts',(53.3017090756875,30.0536765006612,22.1819273843312));
#53040=CARTESIAN_POINT('Ctrl Pts',(53.2394590326199,29.9460057261593,22.1890262323963));
#53041=CARTESIAN_POINT('Ctrl Pts',(53.1441913718116,29.7387886607047,22.2023135761678));
#53042=CARTESIAN_POINT('Ctrl Pts',(53.1082217751973,29.6410974848849,22.2084411469301));
#53043=CARTESIAN_POINT('Ctrl Pts',(53.0724242703148,29.5140676355583,22.2165405869007));
#53044=CARTESIAN_POINT('Ctrl Pts',(53.0653892506668,29.4869238705244,22.2182778564859));
#53045=CARTESIAN_POINT('Ctrl Pts',(53.0563487391451,29.4487457204341,22.2207344690498));
#53046=CARTESIAN_POINT('Ctrl Pts',(53.0538603934951,29.437828241775,22.2214384438084));
#53047=CARTESIAN_POINT('Ctrl Pts',(53.0498288077357,29.4194261264137,22.2226277635318));
#53048=CARTESIAN_POINT('Ctrl Pts',(53.0482364028276,29.4119524398565,22.2231115367065));
#53049=CARTESIAN_POINT('Ctrl Pts',(53.0466869980082,29.4044698737232,22.2235966764224));
#53050=CARTESIAN_POINT('Origin',(55.,29.,3.45145488139523));
#53051=CARTESIAN_POINT('',(53.0466869980276,29.4044698738173,23.182578193545));
#53052=CARTESIAN_POINT('',(53.0466869607994,29.4044696940301,23.0258937941419));
#53053=CARTESIAN_POINT('',(53.0466869980082,29.4044698737233,3.45145488139523));
#53054=CARTESIAN_POINT('Ctrl Pts',(53.0466869980277,29.4044698738173,23.182578193545));
#53055=CARTESIAN_POINT('Ctrl Pts',(53.0538997031978,29.4393023093092,23.1801157224449));
#53056=CARTESIAN_POINT('Ctrl Pts',(53.0620477325019,29.4739592596979,23.1776673773361));
#53057=CARTESIAN_POINT('Ctrl Pts',(53.0781797018133,29.5351636908076,23.1733655989426));
#53058=CARTESIAN_POINT('Ctrl Pts',(53.0857896001927,29.5617758786925,23.1715027165459));
#53059=CARTESIAN_POINT('Ctrl Pts',(53.0992777680491,29.6054823173301,23.1684649597213));
#53060=CARTESIAN_POINT('Ctrl Pts',(53.104838748457,29.6226698367687,23.1672760126887));
#53061=CARTESIAN_POINT('Ctrl Pts',(53.1127462437541,29.6460218635402,23.1656705992356));
#53062=CARTESIAN_POINT('Ctrl Pts',(53.1148907733692,29.6522531680889,23.165243183718));
#53063=CARTESIAN_POINT('Ctrl Pts',(53.1185386463897,29.6626844154669,23.1645294627576));
#53064=CARTESIAN_POINT('Ctrl Pts',(53.1200252559022,29.6668901129382,23.1642421899611));
#53065=CARTESIAN_POINT('Ctrl Pts',(53.1228785943496,29.6748769925741,23.163697609728));
#53066=CARTESIAN_POINT('Ctrl Pts',(53.124242652323,29.6786590454626,23.1634401420789));
#53067=CARTESIAN_POINT('Ctrl Pts',(53.1278446089525,29.6885521817349,23.1627676640657));
#53068=CARTESIAN_POINT('Ctrl Pts',(53.1301010176534,29.6946565437952,23.1623537353227));
#53069=CARTESIAN_POINT('Ctrl Pts',(53.138030009091,29.7157885997186,23.1609239495184));
#53070=CARTESIAN_POINT('Ctrl Pts',(53.1438543705644,29.7307591991237,23.1599165893653));
#53071=CARTESIAN_POINT('Ctrl Pts',(53.1887640577894,29.8421899182108,23.1524485231488));
#53072=CARTESIAN_POINT('Ctrl Pts',(53.2351694282081,29.9355415919484,23.1463566052155));
#53073=CARTESIAN_POINT('Ctrl Pts',(53.3343985266328,30.1012385421766,23.1351231307564));
#53074=CARTESIAN_POINT('Ctrl Pts',(53.3852041377663,30.1744736506369,23.1299839114327));
#53075=CARTESIAN_POINT('Ctrl Pts',(53.4749864673935,30.2870036031922,23.1214813156407));
#53076=CARTESIAN_POINT('Ctrl Pts',(53.5109994945791,30.3285034342905,23.1181967461995));
#53077=CARTESIAN_POINT('Ctrl Pts',(53.5649115754111,30.3856798973613,23.1134054420972));
#53078=CARTESIAN_POINT('Ctrl Pts',(53.5814506510131,30.4026065875893,23.111951307643));
#53079=CARTESIAN_POINT('Ctrl Pts',(53.6113725186843,30.4321590586585,23.1093446147938));
#53080=CARTESIAN_POINT('Ctrl Pts',(53.6246363705457,30.4449016239568,23.1081971590598));
#53081=CARTESIAN_POINT('Ctrl Pts',(53.6449817403593,30.4639134048103,23.1064480068358));
#53082=CARTESIAN_POINT('Ctrl Pts',(53.6519349881482,30.4703188972623,23.1058520998634));
#53083=CARTESIAN_POINT('Ctrl Pts',(53.6590269554757,30.4767595851479,23.1052461177814));
#53084=CARTESIAN_POINT('Ctrl Pts',(53.6591205060713,30.4768445284554,23.1052381245507));
#53085=CARTESIAN_POINT('Ctrl Pts',(53.659311035933,30.4770174952526,23.1052218457807));
#53086=CARTESIAN_POINT('Ctrl Pts',(53.6594080157387,30.4771055180275,23.1052135602188));
#53087=CARTESIAN_POINT('Ctrl Pts',(53.6596056274981,30.4772848429224,23.105196677765));
#53088=CARTESIAN_POINT('Ctrl Pts',(53.6597062602118,30.4773761444017,23.1051880808341));
#53089=CARTESIAN_POINT('Ctrl Pts',(53.6599114211406,30.4775622434345,23.1051705549317));
#53090=CARTESIAN_POINT('Ctrl Pts',(53.6600159500464,30.4776570401425,23.1051616259301));
#53091=CARTESIAN_POINT('Ctrl Pts',(53.6602291679991,30.4778503651388,23.1051434133678));
#53092=CARTESIAN_POINT('Ctrl Pts',(53.6603378578581,30.4779488925307,23.1051341297696));
#53093=CARTESIAN_POINT('Ctrl Pts',(53.6605596862744,30.4781499354858,23.1051151834644));
#53094=CARTESIAN_POINT('Ctrl Pts',(53.6606728257552,30.4782524500704,23.105105520714));
#53095=CARTESIAN_POINT('Ctrl Pts',(53.6609038687936,30.4784617476255,23.1050857892767));
#53096=CARTESIAN_POINT('Ctrl Pts',(53.6610217732926,30.4785685294255,23.105075720549));
#53097=CARTESIAN_POINT('Ctrl Pts',(53.6612626912722,30.4787866675936,23.1050551478234));
#53098=CARTESIAN_POINT('Ctrl Pts',(53.6613857058697,30.4788980227123,23.1050446437742));
#53099=CARTESIAN_POINT('Ctrl Pts',(53.6616372219687,30.479125642706,23.1050231682693));
#53100=CARTESIAN_POINT('Ctrl Pts',(53.6617657248338,30.479241906282,23.1050121967465));
#53101=CARTESIAN_POINT('Ctrl Pts',(53.6619655359365,30.4794226389776,23.1049951378772));
#53102=CARTESIAN_POINT('Ctrl Pts',(53.6620368336565,30.4794871196632,23.1049890510182));
#53103=CARTESIAN_POINT('Ctrl Pts',(53.6621962401624,30.4796312637863,23.1049754425064));
#53104=CARTESIAN_POINT('Ctrl Pts',(53.6622843514159,30.4797109245196,23.1049679207391));
#53105=CARTESIAN_POINT('Ctrl Pts',(53.6624817405421,30.4798893505303,23.1049510709034));
#53106=CARTESIAN_POINT('Ctrl Pts',(53.6625910222643,30.4799881115969,23.1049417426559));
#53107=CARTESIAN_POINT('Ctrl Pts',(53.6628364429752,30.4802098560419,23.1049207945949));
#53108=CARTESIAN_POINT('Ctrl Pts',(53.6629725879568,30.4803328327115,23.1049091745054));
#53109=CARTESIAN_POINT('Ctrl Pts',(53.6632792815313,30.4806097852277,23.1048829994416));
#53110=CARTESIAN_POINT('Ctrl Pts',(53.6634498397601,30.4807637503863,23.1048684440216));
#53111=CARTESIAN_POINT('Ctrl Pts',(53.6638355491008,30.4811118143535,23.1048355299769));
#53112=CARTESIAN_POINT('Ctrl Pts',(53.6640507157838,30.4813058956429,23.1048171706361));
#53113=CARTESIAN_POINT('Ctrl Pts',(53.6700012291259,30.4866709336535,23.1043094819185));
#53114=CARTESIAN_POINT('Ctrl Pts',(53.675766446143,30.4918085291384,23.103818772236));
#53115=CARTESIAN_POINT('Ctrl Pts',(53.688893197399,30.5033702052665,23.1027040309015));
#53116=CARTESIAN_POINT('Ctrl Pts',(53.6962723473708,30.5097738983413,23.1020791757001));
#53117=CARTESIAN_POINT('Ctrl Pts',(53.7154361783318,30.5261591845363,23.1004608349454));
#53118=CARTESIAN_POINT('Ctrl Pts',(53.7272900939902,30.536058443408,23.0994640513898));
#53119=CARTESIAN_POINT('Ctrl Pts',(53.8114114508847,30.6046663344822,23.0924185568241));
#53120=CARTESIAN_POINT('Ctrl Pts',(53.8875864830662,30.6583813032988,23.0861747656923));
#53121=CARTESIAN_POINT('Ctrl Pts',(54.1147510317692,30.7958554966519,23.0679656339418));
#53122=CARTESIAN_POINT('Ctrl Pts',(54.2732232102207,30.8656248933099,23.055680124614));
#53123=CARTESIAN_POINT('Ctrl Pts',(54.4599100713233,30.92036962702,23.0427010891681));
#53124=CARTESIAN_POINT('Ctrl Pts',(54.4812345446595,30.9262396359463,23.0412406487318));
#53125=CARTESIAN_POINT('Ctrl Pts',(54.5095921058613,30.9335405345991,23.0393315634974));
#53126=CARTESIAN_POINT('Ctrl Pts',(54.5165406562702,30.9352896342105,23.0388663814523));
#53127=CARTESIAN_POINT('Ctrl Pts',(54.5279807889037,30.9381039013883,23.0381049542647));
#53128=CARTESIAN_POINT('Ctrl Pts',(54.5324668404817,30.9391909689403,23.037807495589));
#53129=CARTESIAN_POINT('Ctrl Pts',(54.5412519120285,30.9412875248254,23.0372272276282));
#53130=CARTESIAN_POINT('Ctrl Pts',(54.5455505535809,30.9422983198658,23.0369443508637));
#53131=CARTESIAN_POINT('Ctrl Pts',(54.5561471963361,30.9447529405661,23.0362495496678));
#53132=CARTESIAN_POINT('Ctrl Pts',(54.5624489963716,30.9461804729115,23.0358385423359));
#53133=CARTESIAN_POINT('Ctrl Pts',(54.5841456636752,30.9509846569421,23.0344306452576));
#53134=CARTESIAN_POINT('Ctrl Pts',(54.5995740052117,30.9542095638736,23.0334418948166));
#53135=CARTESIAN_POINT('Ctrl Pts',(54.7355571940909,30.9809553136539,23.0248229898514));
#53136=CARTESIAN_POINT('Ctrl Pts',(54.8580240203191,30.9934806403364,23.0177105924691));
#53137=CARTESIAN_POINT('Ctrl Pts',(55.0840258055236,30.995647141275,23.0045846162774));
#53138=CARTESIAN_POINT('Ctrl Pts',(55.1870894825611,30.9886335408157,22.9985971347068));
#53139=CARTESIAN_POINT('Ctrl Pts',(55.3241485259237,30.9685545562316,22.9902700116087));
#53140=CARTESIAN_POINT('Ctrl Pts',(55.3590106242435,30.9624959787507,22.9881207634184));
#53141=CARTESIAN_POINT('Ctrl Pts',(55.4186318350391,30.9504928009747,22.9843787845915));
#53142=CARTESIAN_POINT('Ctrl Pts',(55.4434726324289,30.9449952991038,22.9827996954215));
#53143=CARTESIAN_POINT('Ctrl Pts',(55.4786787819389,30.9364943528188,22.9805301464296));
#53144=CARTESIAN_POINT('Ctrl Pts',(55.4891360556734,30.9338794343386,22.9798520324048));
#53145=CARTESIAN_POINT('Ctrl Pts',(55.5071794290482,30.9292118452308,22.9786748555919));
#53146=CARTESIAN_POINT('Ctrl Pts',(55.5147756107562,30.9271988441098,22.9781770722162));
#53147=CARTESIAN_POINT('Ctrl Pts',(55.5293349519768,30.9232483741408,22.9772186804588));
#53148=CARTESIAN_POINT('Ctrl Pts',(55.5362998772211,30.9213178392616,22.9767583021505));
#53149=CARTESIAN_POINT('Ctrl Pts',(55.5526822332216,30.9166809653052,22.9756708806159));
#53150=CARTESIAN_POINT('Ctrl Pts',(55.5620904516329,30.9139430222001,22.9750428253226));
#53151=CARTESIAN_POINT('Ctrl Pts',(55.5948004045686,30.904161918882,22.97284658496));
#53152=CARTESIAN_POINT('Ctrl Pts',(55.6179923185565,30.8967618570668,22.9712669157421));
#53153=CARTESIAN_POINT('Ctrl Pts',(55.766219297105,30.8464586331983,22.9610211012216));
#53154=CARTESIAN_POINT('Ctrl Pts',(55.8868422687238,30.7916475759597,22.9519602324581));
#53155=CARTESIAN_POINT('Ctrl Pts',(56.087363590916,30.6752927204214,22.9358227548717));
#53156=CARTESIAN_POINT('Ctrl Pts',(56.1697184137742,30.6188655666442,22.9288370616602));
#53157=CARTESIAN_POINT('Ctrl Pts',(56.2692875145394,30.5390632008799,22.920165677334));
#53158=CARTESIAN_POINT('Ctrl Pts',(56.2906955797649,30.5211546309681,22.9182872735512));
#53159=CARTESIAN_POINT('Ctrl Pts',(56.32543303876,30.4908340109624,22.9152251094162));
#53160=CARTESIAN_POINT('Ctrl Pts',(56.3389803978116,30.4786785786073,22.9140271755895));
#53161=CARTESIAN_POINT('Ctrl Pts',(56.3572404087538,30.4618379227196,22.9124096502127));
#53162=CARTESIAN_POINT('Ctrl Pts',(56.3620983495171,30.4573125020788,22.9119790366044));
#53163=CARTESIAN_POINT('Ctrl Pts',(56.3702044316858,30.449685326789,22.9112601648336));
#53164=CARTESIAN_POINT('Ctrl Pts',(56.3734648183057,30.4465967390132,22.9109709310116));
#53165=CARTESIAN_POINT('Ctrl Pts',(56.3796225754742,30.4407238659447,22.9104245387317));
#53166=CARTESIAN_POINT('Ctrl Pts',(56.3825220040547,30.4379417991214,22.9101672100938));
#53167=CARTESIAN_POINT('Ctrl Pts',(56.3900946069374,30.4306316393876,22.9094949203922));
#53168=CARTESIAN_POINT('Ctrl Pts',(56.3947541128942,30.426089362992,22.9090810424584));
#53169=CARTESIAN_POINT('Ctrl Pts',(56.4108500515556,30.4102440355237,22.907650235004));
#53170=CARTESIAN_POINT('Ctrl Pts',(56.4221723330464,30.3988252218292,22.9066418338055));
#53171=CARTESIAN_POINT('Ctrl Pts',(56.5047858959526,30.3134672204676,22.899257962477));
#53172=CARTESIAN_POINT('Ctrl Pts',(56.570418759547,30.2342475435585,22.8932417548336));
#53173=CARTESIAN_POINT('Ctrl Pts',(56.6796015345761,30.0795672201732,22.882227719001));
#53174=CARTESIAN_POINT('Ctrl Pts',(56.724879290495,30.0056429173181,22.8772298975857));
#53175=CARTESIAN_POINT('Ctrl Pts',(56.8018831294644,29.8593285826721,22.8674810397443));
#53176=CARTESIAN_POINT('Ctrl Pts',(56.8343951249771,29.7875410575784,22.8627577505855));
#53177=CARTESIAN_POINT('Ctrl Pts',(56.869987797857,29.6946954369629,22.8566098673597));
#53178=CARTESIAN_POINT('Ctrl Pts',(56.8770963627109,29.6752520341767,22.8553205676457));
#53179=CARTESIAN_POINT('Ctrl Pts',(56.8871615723847,29.6463336307355,22.853398716248));
#53180=CARTESIAN_POINT('Ctrl Pts',(56.890352332517,29.6369411399545,22.8527738583601));
#53181=CARTESIAN_POINT('Ctrl Pts',(56.895901132691,29.6201983866708,22.8516586739924));
#53182=CARTESIAN_POINT('Ctrl Pts',(56.8982868292375,29.6128574507927,22.8511692638996));
#53183=CARTESIAN_POINT('Ctrl Pts',(56.903220233472,29.5973718524534,22.850135824718));
#53184=CARTESIAN_POINT('Ctrl Pts',(56.9057583966007,29.5892243352719,22.8495914958556));
#53185=CARTESIAN_POINT('Ctrl Pts',(56.9123367436444,29.5676205881953,22.848146456147));
#53186=CARTESIAN_POINT('Ctrl Pts',(56.9162871188425,29.5541377218099,22.8472428568503));
#53187=CARTESIAN_POINT('Ctrl Pts',(56.9327872710219,29.4955343134574,22.8433070453543));
#53188=CARTESIAN_POINT('Ctrl Pts',(56.9438874042038,29.4500244964851,22.8402288658391));
#53189=CARTESIAN_POINT('Ctrl Pts',(56.9916628136589,29.2191229417368,22.824492232927));
#53190=CARTESIAN_POINT('Ctrl Pts',(57.0034566568534,29.0295845494409,22.8110686740147));
#53191=CARTESIAN_POINT('Ctrl Pts',(56.9841024379244,28.7871241464056,22.7944012858426));
#53192=CARTESIAN_POINT('Ctrl Pts',(56.9775691187795,28.7331664349957,22.7907344992934));
#53193=CARTESIAN_POINT('Ctrl Pts',(56.9673213353977,28.6702065685746,22.7865547430236));
#53194=CARTESIAN_POINT('Ctrl Pts',(56.9657361380247,28.6608858772697,22.7859385424139));
#53195=CARTESIAN_POINT('Ctrl Pts',(56.9631930925143,28.6465505695968,22.7849951581774));
#53196=CARTESIAN_POINT('Ctrl Pts',(56.9622821887394,28.641527920877,22.7846654476872));
#53197=CARTESIAN_POINT('Ctrl Pts',(56.9605681296859,28.6322790786566,22.7840598951356));
#53198=CARTESIAN_POINT('Ctrl Pts',(56.959770588306,28.6280520077412,22.7837837535927));
#53199=CARTESIAN_POINT('Ctrl Pts',(56.9579374055326,28.618505510358,22.7831614852482));
#53200=CARTESIAN_POINT('Ctrl Pts',(56.9568937591502,28.6131877113254,22.7828158136982));
#53201=CARTESIAN_POINT('Ctrl Pts',(56.9537428811031,28.5974718971388,22.781796901337));
#53202=CARTESIAN_POINT('Ctrl Pts',(56.951574313855,28.587086173454,22.7811270056566));
#53203=CARTESIAN_POINT('Ctrl Pts',(56.9310516115129,28.4925738331424,22.7750581991181));
#53204=CARTESIAN_POINT('Ctrl Pts',(56.9073487212173,28.4096896541196,22.7699325448912));
#53205=CARTESIAN_POINT('Ctrl Pts',(56.8251953968689,28.1798554681987,22.755630579849));
#53206=CARTESIAN_POINT('Ctrl Pts',(56.7545587792672,28.0379720580763,22.7466489723096));
#53207=CARTESIAN_POINT('Ctrl Pts',(56.6431918198514,27.8681952105304,22.7343677748723));
#53208=CARTESIAN_POINT('Ctrl Pts',(56.6171857394711,27.8313378373637,22.7316012495629));
#53209=CARTESIAN_POINT('Ctrl Pts',(56.5818883782659,27.7847489439689,22.7279539382438));
#53210=CARTESIAN_POINT('Ctrl Pts',(56.5737157154849,27.7741840253791,22.7271164414022));
#53211=CARTESIAN_POINT('Ctrl Pts',(56.5602390914297,27.7571195160947,22.725746236237));
#53212=CARTESIAN_POINT('Ctrl Pts',(56.5549990583862,27.7505697920041,22.7252160557743));
#53213=CARTESIAN_POINT('Ctrl Pts',(56.5448241973342,27.7380149870812,22.7241914157125));
#53214=CARTESIAN_POINT('Ctrl Pts',(56.5398952660091,27.73200530741,22.7236971976861));
#53215=CARTESIAN_POINT('Ctrl Pts',(56.5284909807001,27.7182650135866,22.7225584974618));
#53216=CARTESIAN_POINT('Ctrl Pts',(56.5219919173525,27.7105544405231,22.721913063356));
#53217=CARTESIAN_POINT('Ctrl Pts',(56.5010493940144,27.6860868812332,22.7198440281444));
#53218=CARTESIAN_POINT('Ctrl Pts',(56.4863859309555,27.6695212266667,22.718411456505));
#53219=CARTESIAN_POINT('Ctrl Pts',(56.3535810177888,27.5244244454763,22.7055727411746));
#53220=CARTESIAN_POINT('Ctrl Pts',(56.2193363922665,27.4116993904971,22.6934296479604));
#53221=CARTESIAN_POINT('Ctrl Pts',(56.0634871035524,27.3123599166396,22.6805649733658));
#53222=CARTESIAN_POINT('Ctrl Pts',(56.0547497063202,27.306885435272,22.6798477890294));
#53223=CARTESIAN_POINT('Ctrl Pts',(55.9762115955583,27.2585206984383,22.6734391786604));
#53224=CARTESIAN_POINT('Ctrl Pts',(55.9038651631222,27.2198961354828,22.6677991412972));
#53225=CARTESIAN_POINT('Ctrl Pts',(55.8150059943801,27.1792745287799,22.6613318743826));
#53226=CARTESIAN_POINT('Ctrl Pts',(55.8005928923439,27.1728910623025,22.6602968448215));
#53227=CARTESIAN_POINT('Ctrl Pts',(55.780336580407,27.1642054096953,22.6588631462726));
#53228=CARTESIAN_POINT('Ctrl Pts',(55.7745563139171,27.1617591355744,22.6584563940354));
#53229=CARTESIAN_POINT('Ctrl Pts',(55.7646850208706,27.1576363207665,22.6577658972735));
#53230=CARTESIAN_POINT('Ctrl Pts',(55.7605998172617,27.1559460346482,22.6574813400384));
#53231=CARTESIAN_POINT('Ctrl Pts',(55.7527182105534,27.1527156034691,22.656934698963));
#53232=CARTESIAN_POINT('Ctrl Pts',(55.7489226580933,27.1511735616632,22.6566724968923));
#53233=CARTESIAN_POINT('Ctrl Pts',(55.7397800984469,27.1474919336289,22.6560433633041));
#53234=CARTESIAN_POINT('Ctrl Pts',(55.7344284863538,27.1453637741024,22.6556771065823));
#53235=CARTESIAN_POINT('Ctrl Pts',(55.7147671599753,27.1376435613859,22.6543386006907));
#53236=CARTESIAN_POINT('Ctrl Pts',(55.7004017598008,27.1321935309153,22.6533743586092));
#53237=CARTESIAN_POINT('Ctrl Pts',(55.5634354234915,27.0820328976609,22.6442976507526));
#53238=CARTESIAN_POINT('Ctrl Pts',(55.4367702701057,27.0492825186422,22.6367740082767));
#53239=CARTESIAN_POINT('Ctrl Pts',(55.1670533116677,27.0071595280791,22.6209203324711));
#53240=CARTESIAN_POINT('Ctrl Pts',(55.024378691819,27.0003203985089,22.6126076976001));
#53241=CARTESIAN_POINT('Ctrl Pts',(54.8639226821456,27.0098126247242,22.6026420906276));
#53242=CARTESIAN_POINT('Ctrl Pts',(54.8456607065585,27.0111455123618,22.6014994741977));
#53243=CARTESIAN_POINT('Ctrl Pts',(54.8180051514018,27.0135471946582,22.5997552934014));
#53244=CARTESIAN_POINT('Ctrl Pts',(54.8085962379358,27.0144317015751,22.5991594619777));
#53245=CARTESIAN_POINT('Ctrl Pts',(54.7915530404021,27.0161561525795,22.5980756230096));
#53246=CARTESIAN_POINT('Ctrl Pts',(54.7839166050162,27.0169733966369,22.5975883329859));
#53247=CARTESIAN_POINT('Ctrl Pts',(54.767495841239,27.0188267074952,22.5965368437857));
#53248=CARTESIAN_POINT('Ctrl Pts',(54.7587133308977,27.0198771406912,22.5959722050662));
#53249=CARTESIAN_POINT('Ctrl Pts',(54.7350066153004,27.0228726442627,22.5944418240503));
#53250=CARTESIAN_POINT('Ctrl Pts',(54.7200971987941,27.0249282351914,22.5934726467313));
#53251=CARTESIAN_POINT('Ctrl Pts',(54.6464264048459,27.0359362856412,22.5886494973666));
#53252=CARTESIAN_POINT('Ctrl Pts',(54.5880676461809,27.0473425582163,22.5847194519114));
#53253=CARTESIAN_POINT('Ctrl Pts',(54.3600011951108,27.1025974036752,22.5689185555687));
#53254=CARTESIAN_POINT('Ctrl Pts',(54.1958782146237,27.1661218475954,22.5564789473656));
#53255=CARTESIAN_POINT('Ctrl Pts',(54.0108737930314,27.2673914721722,22.5420370302211));
#53256=CARTESIAN_POINT('Ctrl Pts',(53.9800114809717,27.2853785588183,22.5396160631595));
#53257=CARTESIAN_POINT('Ctrl Pts',(53.9311331567388,27.3156527985473,22.5357811743812));
#53258=CARTESIAN_POINT('Ctrl Pts',(53.912807324986,27.3274229450696,22.5343432382754));
#53259=CARTESIAN_POINT('Ctrl Pts',(53.8887600434674,27.3434300963437,22.5324599310119));
#53260=CARTESIAN_POINT('Ctrl Pts',(53.8828640192392,27.3474004444923,22.531998463147));
#53261=CARTESIAN_POINT('Ctrl Pts',(53.8731942655931,27.3539873985975,22.5312422793703));
#53262=CARTESIAN_POINT('Ctrl Pts',(53.8694081842772,27.3565856291473,22.5309463683965));
#53263=CARTESIAN_POINT('Ctrl Pts',(53.8620012466177,27.3617064143402,22.5303678363168));
#53264=CARTESIAN_POINT('Ctrl Pts',(53.8583797433621,27.3642279420008,22.5300851532358));
#53265=CARTESIAN_POINT('Ctrl Pts',(53.8494669585984,27.3704776224028,22.5293898187092));
#53266=CARTESIAN_POINT('Ctrl Pts',(53.8441853403444,27.3742195923964,22.5289780934057));
#53267=CARTESIAN_POINT('Ctrl Pts',(53.8260262482276,27.387218333381,22.527563276225));
#53268=CARTESIAN_POINT('Ctrl Pts',(53.813240624408,27.3966032009004,22.5265684514128));
#53269=CARTESIAN_POINT('Ctrl Pts',(53.705188553773,27.4779159396128,22.5181598109004));
#53270=CARTESIAN_POINT('Ctrl Pts',(53.6164310181734,27.5581188741702,22.5112348402623));
#53271=CARTESIAN_POINT('Ctrl Pts',(53.4635918929388,27.7234199871026,22.4981608545747));
#53272=CARTESIAN_POINT('Ctrl Pts',(53.3981018789543,27.8066321664326,22.4920328761045));
#53273=CARTESIAN_POINT('Ctrl Pts',(53.3196341083094,27.9245067909746,22.4835257171264));
#53274=CARTESIAN_POINT('Ctrl Pts',(53.3005604218475,27.9549066685323,22.4813470044653));
#53275=CARTESIAN_POINT('Ctrl Pts',(53.269242735418,28.007947490989,22.4775583167706));
#53276=CARTESIAN_POINT('Ctrl Pts',(53.2565976683357,28.0303417582436,22.4759624738757));
#53277=CARTESIAN_POINT('Ctrl Pts',(53.2392517338491,28.0624978842584,22.4736732484704));
#53278=CARTESIAN_POINT('Ctrl Pts',(53.2341916578246,28.0720638140863,22.4729925263917));
#53279=CARTESIAN_POINT('Ctrl Pts',(53.2255900336217,28.0886500926603,22.47181249678));
#53280=CARTESIAN_POINT('Ctrl Pts',(53.2220116614762,28.0956511471796,22.4713144892854));
#53281=CARTESIAN_POINT('Ctrl Pts',(53.2152301948318,28.1091148620658,22.4703568454649));
#53282=CARTESIAN_POINT('Ctrl Pts',(53.212020573306,28.1155741105571,22.4698974458219));
#53283=CARTESIAN_POINT('Ctrl Pts',(53.2037352365732,28.1324774908103,22.4686952366882));
#53284=CARTESIAN_POINT('Ctrl Pts',(53.198715621955,28.1429486688055,22.4679505060558));
#53285=CARTESIAN_POINT('Ctrl Pts',(53.1816520502392,28.1793563244686,22.465360776941));
#53286=CARTESIAN_POINT('Ctrl Pts',(53.1700750521043,28.2055065425248,22.4635000086074));
#53287=CARTESIAN_POINT('Ctrl Pts',(53.0946356819842,28.3863139775897,22.4506234384185));
#53288=CARTESIAN_POINT('Ctrl Pts',(53.0499022741434,28.5482012936273,22.4389579101157));
#53289=CARTESIAN_POINT('Ctrl Pts',(53.0121406845093,28.8086022671649,22.420648066318));
#53290=CARTESIAN_POINT('Ctrl Pts',(53.0052383308774,28.9043553628939,22.4140288393459));
#53291=CARTESIAN_POINT('Ctrl Pts',(53.0052514115234,29.0117056221172,22.4069693451081));
#53292=CARTESIAN_POINT('Ctrl Pts',(53.00535161038,29.0231682838032,22.4062202334303));
#53293=CARTESIAN_POINT('Ctrl Pts',(53.0056464057258,29.0401465810844,22.405118227178));
#53294=CARTESIAN_POINT('Ctrl Pts',(53.00576508561,29.0456630589919,22.4047613539211));
#53295=CARTESIAN_POINT('Ctrl Pts',(53.0060172294825,29.0554873599829,22.4041279903023));
#53296=CARTESIAN_POINT('Ctrl Pts',(53.0061417656245,29.0597953062303,22.4038510167415));
#53297=CARTESIAN_POINT('Ctrl Pts',(53.0064420368293,29.0691342941143,22.4032522296248));
#53298=CARTESIAN_POINT('Ctrl Pts',(53.006622854182,29.074165079496,22.4029306993279));
#53299=CARTESIAN_POINT('Ctrl Pts',(53.0071844967961,29.088300448807,22.4020300268339));
#53300=CARTESIAN_POINT('Ctrl Pts',(53.0076086732183,29.0974033239466,22.4014532257062));
#53301=CARTESIAN_POINT('Ctrl Pts',(53.0105982048108,29.1533158558037,22.3979283418912));
#53302=CARTESIAN_POINT('Ctrl Pts',(53.0147508877728,29.2000299805981,22.3950608033523));
#53303=CARTESIAN_POINT('Ctrl Pts',(53.0271467672353,29.2995483206916,22.3890361504842));
#53304=CARTESIAN_POINT('Ctrl Pts',(53.0358692663766,29.3522276431481,22.3858980677615));
#53305=CARTESIAN_POINT('Ctrl Pts',(53.0466870263011,29.4044700103589,22.3827843708292));
#53306=CARTESIAN_POINT('Ctrl Pts',(53.0466869980082,29.4044698737232,22.2235966764224));
#53307=CARTESIAN_POINT('Ctrl Pts',(53.0466279142296,29.4041845394613,22.2236151763568));
#53308=CARTESIAN_POINT('Ctrl Pts',(53.0465688929793,29.4038991922872,22.2236336782779));
#53309=CARTESIAN_POINT('Ctrl Pts',(53.0448752433889,29.3957019319717,22.2241652220084));
#53310=CARTESIAN_POINT('Ctrl Pts',(53.0432886540183,29.3877802705747,22.2246797803914));
#53311=CARTESIAN_POINT('Ctrl Pts',(53.0394790740625,29.3681406152766,22.2259577851166));
#53312=CARTESIAN_POINT('Ctrl Pts',(53.037312997492,29.3564120279491,22.226723013369));
#53313=CARTESIAN_POINT('Ctrl Pts',(53.0295460413525,29.3121368254177,22.2296197496557));
#53314=CARTESIAN_POINT('Ctrl Pts',(53.0246487884617,29.2794737509575,22.2317731475286));
#53315=CARTESIAN_POINT('Ctrl Pts',(53.0143716279036,29.1970152869603,22.2372537451535));
#53316=CARTESIAN_POINT('Ctrl Pts',(53.0100522244178,29.1471129740373,22.2406112592087));
#53317=CARTESIAN_POINT('Ctrl Pts',(53.0019573640592,28.9810226014101,22.2519123805226));
#53318=CARTESIAN_POINT('Ctrl Pts',(53.0064559700848,28.8646758132676,22.2600486505167));
#53319=CARTESIAN_POINT('Ctrl Pts',(53.0326987454006,28.65744554289,22.2745732287844));
#53320=CARTESIAN_POINT('Ctrl Pts',(53.0507385803354,28.5664083035089,22.2809593160895));
#53321=CARTESIAN_POINT('Ctrl Pts',(53.077835422851,28.4666858705796,22.2877467968102));
#53322=CARTESIAN_POINT('Ctrl Pts',(53.0807056153905,28.456447151284,22.2884411217788));
#53323=CARTESIAN_POINT('Ctrl Pts',(53.0851633623117,28.4410209018282,22.2894828520759));
#53324=CARTESIAN_POINT('Ctrl Pts',(53.0866903758059,28.4358162844709,22.2898335619525));
#53325=CARTESIAN_POINT('Ctrl Pts',(53.089466982211,28.4264935313206,22.2904603308994));
#53326=CARTESIAN_POINT('Ctrl Pts',(53.0907086852651,28.4223731669599,22.2907368320506));
#53327=CARTESIAN_POINT('Ctrl Pts',(53.0934526153654,28.4133734615281,22.2913396423756));
#53328=CARTESIAN_POINT('Ctrl Pts',(53.0949602406917,28.4084958644702,22.2916656355923));
#53329=CARTESIAN_POINT('Ctrl Pts',(53.0993101894195,28.3946116935405,22.2925916876043));
#53330=CARTESIAN_POINT('Ctrl Pts',(53.1021978181974,28.3856192998748,22.2931891892226));
#53331=CARTESIAN_POINT('Ctrl Pts',(53.1220086131748,28.3253989557272,22.2971773536682));
#53332=CARTESIAN_POINT('Ctrl Pts',(53.1409418338569,28.274850300297,22.3004609169913));
#53333=CARTESIAN_POINT('Ctrl Pts',(53.2334537947233,28.0554002353968,22.3146855580666));
#53334=CARTESIAN_POINT('Ctrl Pts',(53.3281663945419,27.8963993089427,22.3249947921508));
#53335=CARTESIAN_POINT('Ctrl Pts',(53.4752481410213,27.7128480765358,22.3391495801228));
#53336=CARTESIAN_POINT('Ctrl Pts',(53.5086499464523,27.6742916384692,22.3422657754461));
#53337=CARTESIAN_POINT('Ctrl Pts',(53.5533891754133,27.6264809506489,22.3463450880223));
#53338=CARTESIAN_POINT('Ctrl Pts',(53.5634028561744,27.6160108072289,22.3472523780619));
#53339=CARTESIAN_POINT('Ctrl Pts',(53.5795651396772,27.5994761959036,22.3487082161511));
#53340=CARTESIAN_POINT('Ctrl Pts',(53.5856407347501,27.5933408432425,22.3492536009295));
#53341=CARTESIAN_POINT('Ctrl Pts',(53.5966679733433,27.582348812778,22.3502402155453));
#53342=CARTESIAN_POINT('Ctrl Pts',(53.601605502494,27.5774781221229,22.3506808199816));
#53343=CARTESIAN_POINT('Ctrl Pts',(53.6132841481262,27.5660771306427,22.3517203246385));
#53344=CARTESIAN_POINT('Ctrl Pts',(53.6200461051383,27.559568504851,22.3523201493295));
#53345=CARTESIAN_POINT('Ctrl Pts',(53.6399064426672,27.5407204161777,22.3540761120386));
#53346=CARTESIAN_POINT('Ctrl Pts',(53.6531258984516,27.5285104458243,22.3552377110104));
#53347=CARTESIAN_POINT('Ctrl Pts',(53.6834137892194,27.5012855454956,22.3578837408916));
#53348=CARTESIAN_POINT('Ctrl Pts',(53.7005771017622,27.4863803884188,22.359372472571));
#53349=CARTESIAN_POINT('Ctrl Pts',(53.757713618036,27.4384493522052,22.3642949249135));
#53350=CARTESIAN_POINT('Ctrl Pts',(53.798717505439,27.4066903938278,22.3677757680215));
#53351=CARTESIAN_POINT('Ctrl Pts',(53.9450015653188,27.3022472252632,22.3800090735154));
#53352=CARTESIAN_POINT('Ctrl Pts',(54.0559960423527,27.2381152103718,22.3889986724976));
#53353=CARTESIAN_POINT('Ctrl Pts',(54.2436196051254,27.1525553690392,22.4032852939445));
#53354=CARTESIAN_POINT('Ctrl Pts',(54.3167490057629,27.1242777764996,22.4086446039783));
#53355=CARTESIAN_POINT('Ctrl Pts',(54.4013726971017,27.0971643615563,22.4144799606055));
#53356=CARTESIAN_POINT('Ctrl Pts',(54.4114111556857,27.0940353364946,22.4151664339282));
#53357=CARTESIAN_POINT('Ctrl Pts',(54.4266406341925,27.0894200503009,22.416198730247));
#53358=CARTESIAN_POINT('Ctrl Pts',(54.4318135332571,27.0878753055267,22.4165477718197));
#53359=CARTESIAN_POINT('Ctrl Pts',(54.4411198032717,27.0851373429404,22.417172776062));
#53360=CARTESIAN_POINT('Ctrl Pts',(54.4452508016077,27.083936483924,22.417449169654));
#53361=CARTESIAN_POINT('Ctrl Pts',(54.4543124010385,27.0813340884088,22.418053170844));
#53362=CARTESIAN_POINT('Ctrl Pts',(54.4592445236492,27.0799381905332,22.4183804531221));
#53363=CARTESIAN_POINT('Ctrl Pts',(54.4733722042709,27.0759985045899,22.4193138752085));
#53364=CARTESIAN_POINT('Ctrl Pts',(54.4825808544397,27.0735016153837,22.4199173934789));
#53365=CARTESIAN_POINT('Ctrl Pts',(54.5462527776601,27.0567267081257,22.4240588303713));
#53366=CARTESIAN_POINT('Ctrl Pts',(54.601286804014,27.0446926872494,22.4274799850179));
#53367=CARTESIAN_POINT('Ctrl Pts',(54.751152958943,27.0185146183934,22.4365507507374));
#53368=CARTESIAN_POINT('Ctrl Pts',(54.8466146534227,27.0088485625662,22.4420720743799));
#53369=CARTESIAN_POINT('Ctrl Pts',(55.0737294666312,27.0022883360107,22.4552818637473));
#53370=CARTESIAN_POINT('Ctrl Pts',(55.2050880312969,27.0114778669021,22.4629985723785));
#53371=CARTESIAN_POINT('Ctrl Pts',(55.3501099195795,27.0361520582397,22.4721279260015));
#53372=CARTESIAN_POINT('Ctrl Pts',(55.3656067510442,27.0389779767527,22.4731109963521));
#53373=CARTESIAN_POINT('Ctrl Pts',(55.3907389808102,27.0438692071489,22.4747182908607));
#53374=CARTESIAN_POINT('Ctrl Pts',(55.4003955910327,27.0458229366361,22.4753389958397));
#53375=CARTESIAN_POINT('Ctrl Pts',(55.4175887938356,27.0494342604448,22.4764498953761));
#53376=CARTESIAN_POINT('Ctrl Pts',(55.4251310375242,27.0510642126325,22.4769392043954));
#53377=CARTESIAN_POINT('Ctrl Pts',(55.4410415352649,27.0545993773658,22.4779756912345));
#53378=CARTESIAN_POINT('Ctrl Pts',(55.4494073112564,27.0565149130512,22.4785231888429));
#53379=CARTESIAN_POINT('Ctrl Pts',(55.4716298279579,27.0617544212893,22.479984356558));
#53380=CARTESIAN_POINT('Ctrl Pts',(55.4854635515009,27.065172942921,22.4809010248597));
#53381=CARTESIAN_POINT('Ctrl Pts',(55.5523950236962,27.0824757087335,22.4853714076687));
#53382=CARTESIAN_POINT('Ctrl Pts',(55.6049366126394,27.0983979379471,22.4889898173175));
#53383=CARTESIAN_POINT('Ctrl Pts',(55.8510569401975,27.1842151705142,22.5064749305106));
#53384=CARTESIAN_POINT('Ctrl Pts',(56.0336676877004,27.2816052054567,22.5212221655983));
#53385=CARTESIAN_POINT('Ctrl Pts',(56.2228850928981,27.4237585604516,22.5371671109658));
#53386=CARTESIAN_POINT('Ctrl Pts',(56.247190184982,27.4429187821038,22.5392260244135));
#53387=CARTESIAN_POINT('Ctrl Pts',(56.2775122347541,27.4679880707784,22.5417984767466));
#53388=CARTESIAN_POINT('Ctrl Pts',(56.2839496314808,27.4733790873239,22.5423448336399));
#53389=CARTESIAN_POINT('Ctrl Pts',(56.2940723561193,27.4819657158504,22.5432040661044));
#53390=CARTESIAN_POINT('Ctrl Pts',(56.2977802456266,27.4851344000146,22.5435188174282));
#53391=CARTESIAN_POINT('Ctrl Pts',(56.3047637130131,27.491146782908,22.5441115984268));
#53392=CARTESIAN_POINT('Ctrl Pts',(56.3080416021934,27.4939875349767,22.5443898191192));
#53393=CARTESIAN_POINT('Ctrl Pts',(56.3156591333626,27.5006328292874,22.5450363851539));
#53394=CARTESIAN_POINT('Ctrl Pts',(56.3199915572768,27.5044455347532,22.545404125019));
#53395=CARTESIAN_POINT('Ctrl Pts',(56.3338807290319,27.5167759298904,22.5465833130639));
#53396=CARTESIAN_POINT('Ctrl Pts',(56.3433722770605,27.5253670332411,22.5473895477711));
#53397=CARTESIAN_POINT('Ctrl Pts',(56.4212574875305,27.5972395759938,22.5540152090296));
#53398=CARTESIAN_POINT('Ctrl Pts',(56.4852317859414,27.6651589344583,22.5595240989389));
#53399=CARTESIAN_POINT('Ctrl Pts',(56.6488314091771,27.8652361081725,22.5746135335527));
#53400=CARTESIAN_POINT('Ctrl Pts',(56.7371240184743,28.0056506229502,22.5840433937638));
#53401=CARTESIAN_POINT('Ctrl Pts',(56.8200288006433,28.1830200895703,22.5960242153697));
#53402=CARTESIAN_POINT('Ctrl Pts',(56.8323277368797,28.2109905452035,22.5979131173461));
#53403=CARTESIAN_POINT('Ctrl Pts',(56.8485283290613,28.250258133462,22.6005695971389));
#53404=CARTESIAN_POINT('Ctrl Pts',(56.8529785754591,28.2613253497816,22.6013187958591));
#53405=CARTESIAN_POINT('Ctrl Pts',(56.8599815679416,28.279202518492,22.602530073859));
#53406=CARTESIAN_POINT('Ctrl Pts',(56.8625968440385,28.2859877894969,22.6029900612316));
#53407=CARTESIAN_POINT('Ctrl Pts',(56.8679476696764,28.3000998431279,22.6039473317306));
#53408=CARTESIAN_POINT('Ctrl Pts',(56.8706773441114,28.3074287057457,22.6044448001278));
#53409=CARTESIAN_POINT('Ctrl Pts',(56.8769964100254,28.3247046091197,22.6056183099861));
#53410=CARTESIAN_POINT('Ctrl Pts',(56.880549912397,28.3346644394788,22.6062955218131));
#53411=CARTESIAN_POINT('Ctrl Pts',(56.8919939276747,28.3675642058324,22.608534973175));
#53412=CARTESIAN_POINT('Ctrl Pts',(56.8995449214612,28.3906191158875,22.6101082377976));
#53413=CARTESIAN_POINT('Ctrl Pts',(56.916448161428,28.4455990578515,22.6138709086531));
#53414=CARTESIAN_POINT('Ctrl Pts',(56.9254257155978,28.4776308183483,22.6160716873626));
#53415=CARTESIAN_POINT('Ctrl Pts',(56.971463482644,28.6592533101598,22.6285999238263));
#53416=CARTESIAN_POINT('Ctrl Pts',(56.9918860331995,28.8125061357827,22.6394163157833));
#53417=CARTESIAN_POINT('Ctrl Pts',(56.9958743096145,29.0503126074673,22.655920493156));
#53418=CARTESIAN_POINT('Ctrl Pts',(56.992001173939,29.1340903230906,22.6616679390425));
#53419=CARTESIAN_POINT('Ctrl Pts',(56.9817159759096,29.2279065481281,22.6678663740218));
#53420=CARTESIAN_POINT('Ctrl Pts',(56.9804786816828,29.2384193929931,22.6685575199026));
#53421=CARTESIAN_POINT('Ctrl Pts',(56.9784821590729,29.2542935648063,22.6695954364631));
#53422=CARTESIAN_POINT('Ctrl Pts',(56.9777847144697,29.2596622724775,22.6699454766677));
#53423=CARTESIAN_POINT('Ctrl Pts',(56.9764937448485,29.2692926886636,22.6705715274912));
#53424=CARTESIAN_POINT('Ctrl Pts',(56.9759082826968,29.2735553601114,22.6708479758256));
#53425=CARTESIAN_POINT('Ctrl Pts',(56.9745969132792,29.2828793646414,22.6714512228779));
#53426=CARTESIAN_POINT('Ctrl Pts',(56.9738653384883,29.2879398058453,22.6717777020297));
#53427=CARTESIAN_POINT('Ctrl Pts',(56.9717215338075,29.3023766951074,22.6727066197861));
#53428=CARTESIAN_POINT('Ctrl Pts',(56.9702618714004,29.3117461132499,22.6733064757201));
#53429=CARTESIAN_POINT('Ctrl Pts',(56.9599029988237,29.375257675986,22.6773544293194));
#53430=CARTESIAN_POINT('Ctrl Pts',(56.9488391216017,29.4290283824883,22.6806916942969));
#53431=CARTESIAN_POINT('Ctrl Pts',(56.8880316166375,29.6730720773779,22.6957032092314));
#53432=CARTESIAN_POINT('Ctrl Pts',(56.8125469833334,29.8557871002795,22.7066737363523));
#53433=CARTESIAN_POINT('Ctrl Pts',(56.6909887663972,30.0588610640438,22.7210374346837));
#53434=CARTESIAN_POINT('Ctrl Pts',(56.6694024867358,30.0925771200705,22.7234980399389));
#53435=CARTESIAN_POINT('Ctrl Pts',(56.6393295851477,30.1365747515199,22.7268239351601));
#53436=CARTESIAN_POINT('Ctrl Pts',(56.631732476269,30.1474549084826,22.7276560499901));
#53437=CARTESIAN_POINT('Ctrl Pts',(56.6191695210474,30.1650697926875,22.729019496458));
#53438=CARTESIAN_POINT('Ctrl Pts',(56.6142687782571,30.171850616686,22.7295483447846));
#53439=CARTESIAN_POINT('Ctrl Pts',(56.6047315743875,30.1848732383603,22.7305718425194));
#53440=CARTESIAN_POINT('Ctrl Pts',(56.6001009833363,30.1911191616094,22.7310662596901));
#53441=CARTESIAN_POINT('Ctrl Pts',(56.5892541401297,30.2055724121651,22.7322186757651));
#53442=CARTESIAN_POINT('Ctrl Pts',(56.5830106701347,30.2137589441886,22.73287772627));
#53443=CARTESIAN_POINT('Ctrl Pts',(56.5628038377754,30.2398333240396,22.7349973895402));
#53444=CARTESIAN_POINT('Ctrl Pts',(56.5485989129713,30.2575308518829,22.7364674663212));
#53445=CARTESIAN_POINT('Ctrl Pts',(56.4739250625041,30.3473806400944,22.7440976738615));
#53446=CARTESIAN_POINT('Ctrl Pts',(56.4087134840878,30.4154192244916,22.7504489683036));
#53447=CARTESIAN_POINT('Ctrl Pts',(56.2456792579482,30.5630561175936,22.7655957844854));
#53448=CARTESIAN_POINT('Ctrl Pts',(56.1446287702448,30.6385008105236,22.774469699348));
#53449=CARTESIAN_POINT('Ctrl Pts',(55.9905072924911,30.7323117683897,22.7868405394336));
#53450=CARTESIAN_POINT('Ctrl Pts',(55.9427167919945,30.7587765546672,22.7905290403572));
#53451=CARTESIAN_POINT('Ctrl Pts',(55.8858514754668,30.787281652349,22.7947012156162));
#53452=CARTESIAN_POINT('Ctrl Pts',(55.8777794056537,30.7912598537439,22.7952884994628));
#53453=CARTESIAN_POINT('Ctrl Pts',(55.8646859020451,30.7976030301898,22.7962327987375));
#53454=CARTESIAN_POINT('Ctrl Pts',(55.8596811421078,30.8000018608431,22.7965917897665));
#53455=CARTESIAN_POINT('Ctrl Pts',(55.8507698817116,30.8042274710534,22.7972274486804));
#53456=CARTESIAN_POINT('Ctrl Pts',(55.8468674062139,30.8060625007061,22.7975046139053));
#53457=CARTESIAN_POINT('Ctrl Pts',(55.8384173360632,30.8100024980625,22.7981021438577));
#53458=CARTESIAN_POINT('Ctrl Pts',(55.8338677553347,30.8121029883375,22.7984222359931));
#53459=CARTESIAN_POINT('Ctrl Pts',(55.821118096166,30.817931178514,22.799314857448));
#53460=CARTESIAN_POINT('Ctrl Pts',(55.8129004904925,30.8216205690145,22.7998851119913));
#53461=CARTESIAN_POINT('Ctrl Pts',(55.7635508701782,30.843376204672,22.8032810638749));
#53462=CARTESIAN_POINT('Ctrl Pts',(55.7218396850365,30.8601058905158,22.8060328915489));
#53463=CARTESIAN_POINT('Ctrl Pts',(55.5776517173704,30.912355432801,22.8152617051967));
#53464=CARTESIAN_POINT('Ctrl Pts',(55.4728580581662,30.940925938301,22.8214987688217));
#53465=CARTESIAN_POINT('Ctrl Pts',(55.2373693298085,30.9849116985918,22.8354270744988));
#53466=CARTESIAN_POINT('Ctrl Pts',(55.1064426962563,30.9962169393929,22.843129300215));
#53467=CARTESIAN_POINT('Ctrl Pts',(54.9596091462491,30.9944032585414,22.852242432457));
#53468=CARTESIAN_POINT('Ctrl Pts',(54.9438586895901,30.9940220434908,22.8532256701733));
#53469=CARTESIAN_POINT('Ctrl Pts',(54.918267910712,30.993099223391,22.8548331944138));
#53470=CARTESIAN_POINT('Ctrl Pts',(54.9084239884708,30.9926711914521,22.8554539602591));
#53471=CARTESIAN_POINT('Ctrl Pts',(54.8908770814694,30.9917779239375,22.856564940424));
#53472=CARTESIAN_POINT('Ctrl Pts',(54.8831728132156,30.9913408837629,22.8570542688876));
#53473=CARTESIAN_POINT('Ctrl Pts',(54.8669059379484,30.990323387462,22.8580907673206));
#53474=CARTESIAN_POINT('Ctrl Pts',(54.8583441728841,30.9897323535854,22.8586382569076));
#53475=CARTESIAN_POINT('Ctrl Pts',(54.83557861582,30.9880131259394,22.8600993331932));
#53476=CARTESIAN_POINT('Ctrl Pts',(54.8213828528857,30.9867879801013,22.8610159171576));
#53477=CARTESIAN_POINT('Ctrl Pts',(54.7525948384834,30.9801081486227,22.865484990311));
#53478=CARTESIAN_POINT('Ctrl Pts',(54.6982348175648,30.9725552990531,22.8691021241113));
#53479=CARTESIAN_POINT('Ctrl Pts',(54.4419864452696,30.9261118108534,22.886571589375));
#53480=CARTESIAN_POINT('Ctrl Pts',(54.2466400690703,30.8584164759875,22.9013022891682));
#53481=CARTESIAN_POINT('Ctrl Pts',(54.0376039193733,30.7475096544542,22.9172477620295));
#53482=CARTESIAN_POINT('Ctrl Pts',(54.0104541132185,30.732280404806,22.9193189215391));
#53483=CARTESIAN_POINT('Ctrl Pts',(53.976429916474,30.712133945314,22.9219044130911));
#53484=CARTESIAN_POINT('Ctrl Pts',(53.9692167319578,30.7078009904327,22.9224519498709));
#53485=CARTESIAN_POINT('Ctrl Pts',(53.9578623286614,30.7008822613596,22.9233126360267));
#53486=CARTESIAN_POINT('Ctrl Pts',(53.9537029121571,30.6983267642705,22.9236276710994));
#53487=CARTESIAN_POINT('Ctrl Pts',(53.9458647766519,30.6934713799886,22.9242207848029));
#53488=CARTESIAN_POINT('Ctrl Pts',(53.9421842188321,30.6911747861774,22.9244990559264));
#53489=CARTESIAN_POINT('Ctrl Pts',(53.9336282908388,30.6857972002675,22.925145425672));
#53490=CARTESIAN_POINT('Ctrl Pts',(53.9287587599139,30.6827070541403,22.9255129211782));
#53491=CARTESIAN_POINT('Ctrl Pts',(53.9131488998003,30.6727059993634,22.9266899783752));
#53492=CARTESIAN_POINT('Ctrl Pts',(53.9024612615716,30.6657128839652,22.9274943573537));
#53493=CARTESIAN_POINT('Ctrl Pts',(53.8772942793409,30.6488982690352,22.9293867216191));
#53494=CARTESIAN_POINT('Ctrl Pts',(53.8628753195279,30.638987840701,22.9304695100193));
#53495=CARTESIAN_POINT('Ctrl Pts',(53.8106999113317,30.6021066296465,22.934389737978));
#53496=CARTESIAN_POINT('Ctrl Pts',(53.7737550762776,30.5740089947114,22.9371698941071));
#53497=CARTESIAN_POINT('Ctrl Pts',(53.6148456686757,30.4441592129391,22.9493078032797));
#53498=CARTESIAN_POINT('Ctrl Pts',(53.5043107729896,30.3293475010938,22.9582876740802));
#53499=CARTESIAN_POINT('Ctrl Pts',(53.3726615447035,30.1551372828438,22.9713516382022));
#53500=CARTESIAN_POINT('Ctrl Pts',(53.338912400064,30.106055856973,22.9749738815175));
#53501=CARTESIAN_POINT('Ctrl Pts',(53.2994412992652,30.0427629085061,22.9796163039157));
#53502=CARTESIAN_POINT('Ctrl Pts',(53.2916170958747,30.0298942719655,22.9805586935427));
#53503=CARTESIAN_POINT('Ctrl Pts',(53.2794281756914,30.0093257486017,22.9820631939168));
#53504=CARTESIAN_POINT('Ctrl Pts',(53.274967596055,30.0016831188956,22.9826218376749));
#53505=CARTESIAN_POINT('Ctrl Pts',(53.2667298270567,29.9873505402908,22.9836689005801));
#53506=CARTESIAN_POINT('Ctrl Pts',(53.2629401348411,29.9806679376805,22.9841568600963));
#53507=CARTESIAN_POINT('Ctrl Pts',(53.2545741703182,29.9657150582695,22.9852482701948));
#53508=CARTESIAN_POINT('Ctrl Pts',(53.2500179106197,29.9574338528013,22.9858524177522));
#53509=CARTESIAN_POINT('Ctrl Pts',(53.2368092785104,29.9330172836346,22.9876330169227));
#53510=CARTESIAN_POINT('Ctrl Pts',(53.2283201846487,29.9167951608448,22.9888151619028));
#53511=CARTESIAN_POINT('Ctrl Pts',(53.1557643431617,29.773373461889,22.9992620178185));
#53512=CARTESIAN_POINT('Ctrl Pts',(53.1052803448653,29.639792556273,23.0090052571375));
#53513=CARTESIAN_POINT('Ctrl Pts',(53.0610441144254,29.4696738527281,23.0212400442453));
#53514=CARTESIAN_POINT('Ctrl Pts',(53.0534544604073,29.4371521061416,23.023569125178));
#53515=CARTESIAN_POINT('Ctrl Pts',(53.0466869607994,29.4044696940301,23.0258937941419));
#53516=CARTESIAN_POINT('Origin',(55.,29.,14.365));
#53517=CARTESIAN_POINT('',(52.5495005484666,29.0016395226469,5.18832749621205));
#53518=CARTESIAN_POINT('',(56.0772398577513,31.2053700969644,4.93052640483872));
#53519=CARTESIAN_POINT('Ctrl Pts',(52.5467359272522,29.0016413723348,5.18832749621205));
#53520=CARTESIAN_POINT('Ctrl Pts',(52.5460824238429,29.0920814519017,5.18361297623425));
#53521=CARTESIAN_POINT('Ctrl Pts',(52.5915758653443,29.9920162182401,5.13666417946793));
#53522=CARTESIAN_POINT('Ctrl Pts',(53.6625878394777,31.5282585313447,5.05073048234352));
#53523=CARTESIAN_POINT('Ctrl Pts',(55.4037421823906,31.5296428126932,4.96951130519688));
#53524=CARTESIAN_POINT('Ctrl Pts',(56.0772398577513,31.2053700969644,4.93052640483872));
#53525=CARTESIAN_POINT('',(53.9249115396487,31.2020751695661,4.9305));
#53526=CARTESIAN_POINT('Origin',(55.,29.,4.9305));
#53527=CARTESIAN_POINT('',(52.5493359835256,29.0024358842253,5.07267250378794));
#53528=CARTESIAN_POINT('Ctrl Pts',(53.9249115396487,31.2020751695661,4.9305));
#53529=CARTESIAN_POINT('Ctrl Pts',(53.1944672756053,30.8454605498401,4.97273427678848));
#53530=CARTESIAN_POINT('Ctrl Pts',(52.5965917064306,30.0088392096125,5.02012511138446));
#53531=CARTESIAN_POINT('Ctrl Pts',(52.5465875494899,29.1013071020944,5.06751594598044));
#53532=CARTESIAN_POINT('Ctrl Pts',(52.5473557780223,29.0024378524883,5.07267250378794));
#53533=CARTESIAN_POINT('',(52.5495001447487,29.0008422667624,5.87267250374925));
#53534=CARTESIAN_POINT('Ctrl Pts',(52.5495012105149,29.0024357199948,5.07267250378794));
#53535=CARTESIAN_POINT('Ctrl Pts',(52.5494224648678,28.9232122816583,5.0768080814921));
#53536=CARTESIAN_POINT('Ctrl Pts',(52.5531897391159,28.8438158281259,5.08094365919625));
#53537=CARTESIAN_POINT('Ctrl Pts',(52.5608267508401,28.764661710334,5.0850792369004));
#53538=CARTESIAN_POINT('Ctrl Pts',(52.5684526154381,28.6856231273839,5.08920877823741));
#53539=CARTESIAN_POINT('Ctrl Pts',(52.5799369575232,28.606826657945,5.09333831957442));
#53540=CARTESIAN_POINT('Ctrl Pts',(52.5952514853866,28.5286881802196,5.09746786091143));
#53541=CARTESIAN_POINT('Ctrl Pts',(52.6105535814955,28.4506131323553,5.10159405004295));
#53542=CARTESIAN_POINT('Ctrl Pts',(52.6296796078446,28.3731954926565,5.10572023917448));
#53543=CARTESIAN_POINT('Ctrl Pts',(52.652549558233,28.296845199513,5.10984642830601));
#53544=CARTESIAN_POINT('Ctrl Pts',(52.6754086101304,28.2205312904879,5.11397065113528));
#53545=CARTESIAN_POINT('Ctrl Pts',(52.702007908902,28.1452841847404,5.11809487396455));
#53546=CARTESIAN_POINT('Ctrl Pts',(52.7322169248663,28.0715011178591,5.12221909679382));
#53547=CARTESIAN_POINT('Ctrl Pts',(52.7624216675123,27.9977284882103,5.12634273621725));
#53548=CARTESIAN_POINT('Ctrl Pts',(52.7962349286359,27.9254199362223,5.13046637564066));
#53549=CARTESIAN_POINT('Ctrl Pts',(52.8334777514998,27.8549534521455,5.13459001506409));
#53550=CARTESIAN_POINT('Ctrl Pts',(52.8707535168953,27.7844246380892,5.13871730198553));
#53551=CARTESIAN_POINT('Ctrl Pts',(52.9114646769339,27.7157415784887,5.14284458890697));
#53552=CARTESIAN_POINT('Ctrl Pts',(52.9553863302534,27.6492575406521,5.14697187582841));
#53553=CARTESIAN_POINT('Ctrl Pts',(52.9993258736485,27.5827464226767,5.15110084386769));
#53554=CARTESIAN_POINT('Ctrl Pts',(53.0464782241391,27.5184365014121,5.15522981190697));
#53555=CARTESIAN_POINT('Ctrl Pts',(53.0965767764186,27.4566496567756,5.15935877994625));
#53556=CARTESIAN_POINT('Ctrl Pts',(53.1467657495005,27.3947512956217,5.16349520018898));
#53557=CARTESIAN_POINT('Ctrl Pts',(53.1999112198573,27.3353854695021,5.1676316204317));
#53558=CARTESIAN_POINT('Ctrl Pts',(53.2557084502778,27.2788384039935,5.17176804067443));
#53559=CARTESIAN_POINT('Ctrl Pts',(53.3102842705368,27.2235291626545,5.17581391402659));
#53560=CARTESIAN_POINT('Ctrl Pts',(53.3673965452187,27.1709167338838,5.17985978737875));
#53561=CARTESIAN_POINT('Ctrl Pts',(53.4267314148439,27.1212301341141,5.18390566073091));
#53562=CARTESIAN_POINT('Ctrl Pts',(53.4888727187617,27.0691934461356,5.18814289673021));
#53563=CARTESIAN_POINT('Ctrl Pts',(53.5537128604257,27.0201473329936,5.19238013272951));
#53564=CARTESIAN_POINT('Ctrl Pts',(53.6209324746831,26.9743833011607,5.19661736872881));
#53565=CARTESIAN_POINT('Ctrl Pts',(53.6880561113035,26.9286846122147,5.20084855470976));
#53566=CARTESIAN_POINT('Ctrl Pts',(53.757552092408,26.886258955162,5.20507974069071));
#53567=CARTESIAN_POINT('Ctrl Pts',(53.8290676315859,26.8473579864269,5.20931092667167));
#53568=CARTESIAN_POINT('Ctrl Pts',(53.9005001602593,26.8085021713615,5.21353720137199));
#53569=CARTESIAN_POINT('Ctrl Pts',(53.9739471826816,26.7731631330336,5.21776347607231));
#53570=CARTESIAN_POINT('Ctrl Pts',(54.049027780934,26.7415487411581,5.22198975077262));
#53571=CARTESIAN_POINT('Ctrl Pts',(54.1240604562315,26.7099545283316,5.22621332789758));
#53572=CARTESIAN_POINT('Ctrl Pts',(54.2007242114499,26.682080421538,5.23043690502253));
#53573=CARTESIAN_POINT('Ctrl Pts',(54.2786154424704,26.6580874119306,5.23466048214749));
#53574=CARTESIAN_POINT('Ctrl Pts',(54.3564806232596,26.6341024266341,5.23888264672369));
#53575=CARTESIAN_POINT('Ctrl Pts',(54.4355720220388,26.6139960968527,5.24310481129989));
#53576=CARTESIAN_POINT('Ctrl Pts',(54.5154693972406,26.5978800310997,5.24732697587609));
#53577=CARTESIAN_POINT('Ctrl Pts',(54.5953643267749,26.5817644586612,5.25154901121137));
#53578=CARTESIAN_POINT('Ctrl Pts',(54.6760647292506,26.5696389979145,5.25577104654666));
#53579=CARTESIAN_POINT('Ctrl Pts',(54.7571400476834,26.5615641707109,5.25999308188194));
#53580=CARTESIAN_POINT('Ctrl Pts',(54.8382930369531,26.5534816077549,5.26421916196258));
#53581=CARTESIAN_POINT('Ctrl Pts',(54.9198211976031,26.5494574773029,5.26844524204323));
#53582=CARTESIAN_POINT('Ctrl Pts',(55.0012892530824,26.5495003391499,5.27267132212388));
#53583=CARTESIAN_POINT('Ctrl Pts',(55.0827941835916,26.5495432203976,5.27689931506261));
#53584=CARTESIAN_POINT('Ctrl Pts',(55.164238491225,26.5536567390748,5.28112730800134));
#53585=CARTESIAN_POINT('Ctrl Pts',(55.2451897908321,26.5617973389253,5.28535530094008));
#53586=CARTESIAN_POINT('Ctrl Pts',(55.3262852922789,26.5699524399572,5.28959082537444));
#53587=CARTESIAN_POINT('Ctrl Pts',(55.4068855710543,26.5821488893415,5.29382634980881));
#53588=CARTESIAN_POINT('Ctrl Pts',(55.4865663435973,26.5982915573954,5.29806187424317));
#53589=CARTESIAN_POINT('Ctrl Pts',(55.565244056291,26.6142310137877,5.3022440798609));
#53590=CARTESIAN_POINT('Ctrl Pts',(55.6430248886805,26.6340176960711,5.30642628547863));
#53591=CARTESIAN_POINT('Ctrl Pts',(55.7195166982866,26.6575128664416,5.31060849109635));
#53592=CARTESIAN_POINT('Ctrl Pts',(55.797057875483,26.6813303598222,5.31484807110559));
#53593=CARTESIAN_POINT('Ctrl Pts',(55.8735539493563,26.7090447615575,5.31908765111483));
#53594=CARTESIAN_POINT('Ctrl Pts',(55.9485863104976,26.7405455832134,5.32332723112406));
#53595=CARTESIAN_POINT('Ctrl Pts',(56.0235143306667,26.7720025994192,5.32756091551849));
#53596=CARTESIAN_POINT('Ctrl Pts',(56.0969822579391,26.8072353987265,5.33179459991293));
#53597=CARTESIAN_POINT('Ctrl Pts',(56.1685868793458,26.8460838095644,5.33602828430736));
#53598=CARTESIAN_POINT('Ctrl Pts',(56.2401122064234,26.8848892000131,5.34025728035685));
#53599=CARTESIAN_POINT('Ctrl Pts',(56.3097779240461,26.9273020243104,5.34448627640635));
#53600=CARTESIAN_POINT('Ctrl Pts',(56.377202362273,26.9731147286169,5.34871527245585));
#53601=CARTESIAN_POINT('Ctrl Pts',(56.4445859316388,27.0188996638667,5.35294170512838));
#53602=CARTESIAN_POINT('Ctrl Pts',(56.5097305369672,27.0680801282834,5.35716813780091));
#53603=CARTESIAN_POINT('Ctrl Pts',(56.5722816165271,27.1204040944046,5.36139457047344));
#53604=CARTESIAN_POINT('Ctrl Pts',(56.6348137209451,27.1727121878233,5.36561972103925));
#53605=CARTESIAN_POINT('Ctrl Pts',(56.6947535075508,27.2281615922263,5.36984487160506));
#53606=CARTESIAN_POINT('Ctrl Pts',(56.7517788976561,27.2864595295918,5.37407002217087));
#53607=CARTESIAN_POINT('Ctrl Pts',(56.808804254942,27.3447574334055,5.37829517030501));
#53608=CARTESIAN_POINT('Ctrl Pts',(56.862914896437,27.4059035351946,5.38252031843916));
#53609=CARTESIAN_POINT('Ctrl Pts',(56.9138260782558,27.4695686907973,5.38674546657331));
#53610=CARTESIAN_POINT('Ctrl Pts',(56.9647881705314,27.5332975106489,5.39097483979543));
#53611=CARTESIAN_POINT('Ctrl Pts',(57.0125441218747,27.5995500543816,5.39520421301754));
#53612=CARTESIAN_POINT('Ctrl Pts',(57.0568502762523,27.6679650188224,5.39943358623965));
#53613=CARTESIAN_POINT('Ctrl Pts',(57.101177550683,27.7364125956102,5.40366497553804));
#53614=CARTESIAN_POINT('Ctrl Pts',(57.1420515193405,27.8070242459414,5.40789636483643));
#53615=CARTESIAN_POINT('Ctrl Pts',(57.179273880197,27.8794128302131,5.41212775413482));
#53616=CARTESIAN_POINT('Ctrl Pts',(57.2165637116688,27.9519326286852,5.4163668134045));
#53617=CARTESIAN_POINT('Ctrl Pts',(57.2501885161182,28.0262353752396,5.42060587267418));
#53618=CARTESIAN_POINT('Ctrl Pts',(57.2799977056027,28.1019127478654,5.42484493194386));
#53619=CARTESIAN_POINT('Ctrl Pts',(57.3092190448736,28.1760977297077,5.42900039511651));
#53620=CARTESIAN_POINT('Ctrl Pts',(57.3347738512411,28.2516031919899,5.43315585828916));
#53621=CARTESIAN_POINT('Ctrl Pts',(57.356567525692,28.3280329272548,5.4373113214618));
#53622=CARTESIAN_POINT('Ctrl Pts',(57.3787400345672,28.4057912230072,5.44153901809384));
#53623=CARTESIAN_POINT('Ctrl Pts',(57.3971019507572,28.4847960014073,5.44576671472587));
#53624=CARTESIAN_POINT('Ctrl Pts',(57.4115163311385,28.5646389605716,5.4499944113579));
#53625=CARTESIAN_POINT('Ctrl Pts',(57.4259098908971,28.6443665918421,5.45421600136069));
#53626=CARTESIAN_POINT('Ctrl Pts',(57.4363671567194,28.7249295450193,5.45843759136349));
#53627=CARTESIAN_POINT('Ctrl Pts',(57.4428011376394,28.8059050439926,5.46265918136628));
#53628=CARTESIAN_POINT('Ctrl Pts',(57.4492374561203,28.8869099625686,5.46688230513549));
#53629=CARTESIAN_POINT('Ctrl Pts',(57.4516474613226,28.9683272704142,5.47110542890469));
#53630=CARTESIAN_POINT('Ctrl Pts',(57.449995460337,29.0497241825289,5.4753285526739));
#53631=CARTESIAN_POINT('Ctrl Pts',(57.4483470598133,29.1309436937316,5.47954247233464));
#53632=CARTESIAN_POINT('Ctrl Pts',(57.4426543248039,29.2121424316842,5.48375639199537));
#53633=CARTESIAN_POINT('Ctrl Pts',(57.4329338161821,29.2928878558045,5.48797031165611));
#53634=CARTESIAN_POINT('Ctrl Pts',(57.4232165743765,29.3736061434363,5.49218281512536));
#53635=CARTESIAN_POINT('Ctrl Pts',(57.4094743025865,29.4538709576714,5.49639531859461));
#53636=CARTESIAN_POINT('Ctrl Pts',(57.3917754470409,29.5332545929782,5.50060782206385));
#53637=CARTESIAN_POINT('Ctrl Pts',(57.3740770926785,29.6126359803575,5.50482020624652));
#53638=CARTESIAN_POINT('Ctrl Pts',(57.35242247976,29.6911357840195,5.50903259042918));
#53639=CARTESIAN_POINT('Ctrl Pts',(57.3269309246493,29.7683376353602,5.51324497461185));
#53640=CARTESIAN_POINT('Ctrl Pts',(57.3013281380643,29.8458763541735,5.5174757393798));
#53641=CARTESIAN_POINT('Ctrl Pts',(57.2718549837999,29.9221053139697,5.52170650414775));
#53642=CARTESIAN_POINT('Ctrl Pts',(57.2386819677278,29.9966209396608,5.5259372689157));
#53643=CARTESIAN_POINT('Ctrl Pts',(57.2056054035238,30.0709199081966,5.53015573256625));
#53644=CARTESIAN_POINT('Ctrl Pts',(57.168850712839,30.1435150931823,5.53437419621681));
#53645=CARTESIAN_POINT('Ctrl Pts',(57.1286331694868,30.2140309220775,5.53859265986736));
#53646=CARTESIAN_POINT('Ctrl Pts',(57.0882397134933,30.2848551891488,5.54282957519401));
#53647=CARTESIAN_POINT('Ctrl Pts',(57.0443533024324,30.3535814727305,5.54706649052066));
#53648=CARTESIAN_POINT('Ctrl Pts',(56.9972350276436,30.4198600263243,5.55130340584731));
#53649=CARTESIAN_POINT('Ctrl Pts',(56.9501167528548,30.486138579918,5.55554032117396));
#53650=CARTESIAN_POINT('Ctrl Pts',(56.8997669543256,30.5499690741391,5.55977723650061));
#53651=CARTESIAN_POINT('Ctrl Pts',(56.8464850698016,30.6110379067544,5.56401415182726));
#53652=CARTESIAN_POINT('Ctrl Pts',(56.793245634285,30.6720580865987,5.56824769165674));
#53653=CARTESIAN_POINT('Ctrl Pts',(56.7368794524142,30.7305495121183,5.57248123148623));
#53654=CARTESIAN_POINT('Ctrl Pts',(56.6776559975179,30.7861748525809,5.57671477131572));
#53655=CARTESIAN_POINT('Ctrl Pts',(56.6185169604046,30.8417209040535,5.58094227660962));
#53656=CARTESIAN_POINT('Ctrl Pts',(56.5565290750968,30.8944086693625,5.58516978190351));
#53657=CARTESIAN_POINT('Ctrl Pts',(56.4920010549055,30.9439349531712,5.5893972871974));
#53658=CARTESIAN_POINT('Ctrl Pts',(56.4275473552574,30.9934041947786,5.59361992343613));
#53659=CARTESIAN_POINT('Ctrl Pts',(56.3605597018324,31.0397189106184,5.59784255967486));
#53660=CARTESIAN_POINT('Ctrl Pts',(56.2913814346201,31.0826147604198,5.60206519591359));
#53661=CARTESIAN_POINT('Ctrl Pts',(56.2222469102552,31.1254834862893,5.6062851620922));
#53662=CARTESIAN_POINT('Ctrl Pts',(56.1509249154057,31.1649373935957,5.6105051282708));
#53663=CARTESIAN_POINT('Ctrl Pts',(56.0777885058566,31.2007549128977,5.61472509444941));
#53664=CARTESIAN_POINT('Ctrl Pts',(56.0046760072943,31.236560722133,5.6189436809656));
#53665=CARTESIAN_POINT('Ctrl Pts',(55.9297506887809,31.2687323003632,5.62316226748179));
#53666=CARTESIAN_POINT('Ctrl Pts',(55.8534097258461,31.2970942709935,5.62738085399797));
#53667=CARTESIAN_POINT('Ctrl Pts',(55.7770704088625,31.3254556301249,5.63159934955922));
#53668=CARTESIAN_POINT('Ctrl Pts',(55.6993159437972,31.3500073843642,5.63581784512047));
#53669=CARTESIAN_POINT('Ctrl Pts',(55.6205616338611,31.3706230211866,5.64003634068171));
#53670=CARTESIAN_POINT('Ctrl Pts',(55.5417160104358,31.3912625612814,5.64425972747429));
#53671=CARTESIAN_POINT('Ctrl Pts',(55.4618686754863,31.4079567437039,5.64848311426688));
#53672=CARTESIAN_POINT('Ctrl Pts',(55.3814478996298,31.4206296184811,5.65270650105946));
#53673=CARTESIAN_POINT('Ctrl Pts',(55.3010043621856,31.4333060800771,5.65693108320223));
#53674=CARTESIAN_POINT('Ctrl Pts',(55.2199875239284,31.4419589243,5.661155665345));
#53675=CARTESIAN_POINT('Ctrl Pts',(55.1388306373433,31.4465641835306,5.66538024748776));
#53676=CARTESIAN_POINT('Ctrl Pts',(55.0575268890906,31.4511777764477,5.669612474443));
#53677=CARTESIAN_POINT('Ctrl Pts',(54.9760830516879,31.4517291433342,5.67384470139824));
#53678=CARTESIAN_POINT('Ctrl Pts',(54.8949323643657,31.4482465239314,5.67807692835348));
#53679=CARTESIAN_POINT('Ctrl Pts',(54.8141436080213,31.4447794369645,5.68229027963322));
#53680=CARTESIAN_POINT('Ctrl Pts',(54.7336458330819,31.4373144061993,5.68650363091296));
#53681=CARTESIAN_POINT('Ctrl Pts',(54.6538573734615,31.425929828353,5.69071698219271));
#53682=CARTESIAN_POINT('Ctrl Pts',(54.5736895690821,31.414491123883,5.69495036535091));
#53683=CARTESIAN_POINT('Ctrl Pts',(54.4939409450085,31.3990531095036,5.69918374850912));
#53684=CARTESIAN_POINT('Ctrl Pts',(54.4150411429032,31.3796582497292,5.70341713166733));
#53685=CARTESIAN_POINT('Ctrl Pts',(54.336253552147,31.3602909733367,5.70764449410529));
#53686=CARTESIAN_POINT('Ctrl Pts',(54.2583128328872,31.3369781384252,5.71187185654326));
#53687=CARTESIAN_POINT('Ctrl Pts',(54.1816413452542,31.3098137072506,5.71609921898122));
#53688=CARTESIAN_POINT('Ctrl Pts',(54.1050577729587,31.2826804241626,5.72032173411536));
#53689=CARTESIAN_POINT('Ctrl Pts',(54.0297409752458,31.2517044766712,5.7245442492495));
#53690=CARTESIAN_POINT('Ctrl Pts',(53.9560995623481,31.2170300237638,5.72876676438364));
#53691=CARTESIAN_POINT('Ctrl Pts',(53.882504484241,31.1823773878403,5.73298662273342));
#53692=CARTESIAN_POINT('Ctrl Pts',(53.8105831173282,31.144031063345,5.73720648108319));
#53693=CARTESIAN_POINT('Ctrl Pts',(53.7407243612159,31.102183416252,5.74142633943296));
#53694=CARTESIAN_POINT('Ctrl Pts',(53.6708882222943,31.0603493175854,5.74564483157833));
#53695=CARTESIAN_POINT('Ctrl Pts',(53.603113766025,31.0150163860036,5.74986332372369));
#53696=CARTESIAN_POINT('Ctrl Pts',(53.5377642646719,30.9664223616328,5.75408181586905));
#53697=CARTESIAN_POINT('Ctrl Pts',(53.4724159608207,30.9178292277269,5.75830023071233));
#53698=CARTESIAN_POINT('Ctrl Pts',(53.4094928954424,30.8659753978873,5.76251864555561));
#53699=CARTESIAN_POINT('Ctrl Pts',(53.3493272111909,30.8111404126365,5.76673706039889));
#53700=CARTESIAN_POINT('Ctrl Pts',(53.2890881052569,30.756238510888,5.77096062307883));
#53701=CARTESIAN_POINT('Ctrl Pts',(53.2316134514668,30.6983484949871,5.77518418575877));
#53702=CARTESIAN_POINT('Ctrl Pts',(53.1772000794838,30.6377883562189,5.77940774843871));
#53703=CARTESIAN_POINT('Ctrl Pts',(53.122774167702,30.5772142611027,5.78363228445708));
#53704=CARTESIAN_POINT('Ctrl Pts',(53.0714112291474,30.5139691845898,5.78785682047545));
#53705=CARTESIAN_POINT('Ctrl Pts',(53.0233671420721,30.4484035331909,5.79208135649382));
#53706=CARTESIAN_POINT('Ctrl Pts',(52.9752358696952,30.3827189002181,5.79631355875104));
#53707=CARTESIAN_POINT('Ctrl Pts',(52.9304357411302,30.3147056654596,5.80054576100826));
#53708=CARTESIAN_POINT('Ctrl Pts',(52.8891788279744,30.2447426359406,5.80477796326547));
#53709=CARTESIAN_POINT('Ctrl Pts',(52.848099846182,30.1750813405138,5.8089919130297));
#53710=CARTESIAN_POINT('Ctrl Pts',(52.8105337072027,30.103487477362,5.81320586279394));
#53711=CARTESIAN_POINT('Ctrl Pts',(52.7766423574683,30.0303548143216,5.81741981255817));
#53712=CARTESIAN_POINT('Ctrl Pts',(52.7396108236006,29.9504460851199,5.82202420349075));
#53713=CARTESIAN_POINT('Ctrl Pts',(52.7068454862175,29.8684405297593,5.82662859442335));
#53714=CARTESIAN_POINT('Ctrl Pts',(52.6785676497307,29.7847942998794,5.83123298535594));
#53715=CARTESIAN_POINT('Ctrl Pts',(52.6504458222707,29.70160954685,5.83581197383071));
#53716=CARTESIAN_POINT('Ctrl Pts',(52.626762269592,29.6168024762131,5.84039096230549));
#53717=CARTESIAN_POINT('Ctrl Pts',(52.6076887509001,29.5308456813709,5.84496995078027));
#53718=CARTESIAN_POINT('Ctrl Pts',(52.5884565134465,29.4441736039286,5.84958704294176));
#53719=CARTESIAN_POINT('Ctrl Pts',(52.573911597095,29.356332870434,5.85420413510326));
#53720=CARTESIAN_POINT('Ctrl Pts',(52.5641801417191,29.2678280567907,5.85882122726475));
#53721=CARTESIAN_POINT('Ctrl Pts',(52.5544486863431,29.1793232431473,5.86343831942625));
#53722=CARTESIAN_POINT('Ctrl Pts',(52.5495308425188,29.0901546848532,5.86805541158775));
#53723=CARTESIAN_POINT('Ctrl Pts',(52.5495001447487,29.0008422667624,5.87267250374924));
#53724=CARTESIAN_POINT('',(52.5495009959581,28.9977906585885,6.67267250383498));
#53725=CARTESIAN_POINT('Ctrl Pts',(52.5495001447484,29.0008422660139,5.87267250378794));
#53726=CARTESIAN_POINT('Ctrl Pts',(52.5494714453592,28.9173438843335,5.87698903369265));
#53727=CARTESIAN_POINT('Ctrl Pts',(52.5537147778818,28.8338772411954,5.88130556359736));
#53728=CARTESIAN_POINT('Ctrl Pts',(52.5621942075986,28.7508952659337,5.88562209350207));
#53729=CARTESIAN_POINT('Ctrl Pts',(52.5706794363711,28.6678565395561,5.88994157546822));
#53730=CARTESIAN_POINT('Ctrl Pts',(52.5834064823908,28.5853035711796,5.89426105743437));
#53731=CARTESIAN_POINT('Ctrl Pts',(52.6002878479079,28.5036817179453,5.89858053940052));
#53732=CARTESIAN_POINT('Ctrl Pts',(52.6171986312631,28.4219176286784,5.90290754859073));
#53733=CARTESIAN_POINT('Ctrl Pts',(52.6382781014815,28.34108831937,5.90723455778094));
#53734=CARTESIAN_POINT('Ctrl Pts',(52.6633881422363,28.2616266011304,5.91156156697115));
#53735=CARTESIAN_POINT('Ctrl Pts',(52.6885222735803,28.1820886472676,5.91589272749675));
#53736=CARTESIAN_POINT('Ctrl Pts',(52.7176945279371,28.1039213037629,5.92022388802234));
#53737=CARTESIAN_POINT('Ctrl Pts',(52.7507185128329,28.0275376400666,5.92455504854794));
#53738=CARTESIAN_POINT('Ctrl Pts',(52.7838107128232,27.9509961965367,5.92889515561726));
#53739=CARTESIAN_POINT('Ctrl Pts',(52.8207703437845,27.8762461804629,5.93323526268658));
#53740=CARTESIAN_POINT('Ctrl Pts',(52.8613649006829,27.8036763974706,5.9375753697559));
#53741=CARTESIAN_POINT('Ctrl Pts',(52.8817778881116,27.7671846561854,5.93975779414514));
#53742=CARTESIAN_POINT('Ctrl Pts',(52.9031093113642,27.7312437481034,5.94194021853437));
#53743=CARTESIAN_POINT('Ctrl Pts',(52.9253256277235,27.695900119232,5.9441226429236));
#53744=CARTESIAN_POINT('Ctrl Pts',(52.9684138980889,27.6273515888692,5.94835542799088));
#53745=CARTESIAN_POINT('Ctrl Pts',(53.014983225727,27.5608134483899,5.95258821305815));
#53746=CARTESIAN_POINT('Ctrl Pts',(53.0648200520184,27.4966607771598,5.95682099812542));
#53747=CARTESIAN_POINT('Ctrl Pts',(53.1145858079948,27.4325995915015,5.96104774698633));
#53748=CARTESIAN_POINT('Ctrl Pts',(53.1676095253359,27.3709174823951,5.96527449584723));
#53749=CARTESIAN_POINT('Ctrl Pts',(53.2236335657583,27.3119619254,5.96950124470814));
#53750=CARTESIAN_POINT('Ctrl Pts',(53.2795930839848,27.2530742667923,5.97372312567455));
#53751=CARTESIAN_POINT('Ctrl Pts',(53.3385457393656,27.1969072543506,5.97794500664097));
#53752=CARTESIAN_POINT('Ctrl Pts',(53.4001936366458,27.1437753773394,5.98216688760738));
#53753=CARTESIAN_POINT('Ctrl Pts',(53.4618025611284,27.0906770894364,5.98638609956934));
#53754=CARTESIAN_POINT('Ctrl Pts',(53.5261029941909,27.0406104304442,5.99060531153131));
#53755=CARTESIAN_POINT('Ctrl Pts',(53.5927610265866,26.9938522682249,5.99482452349327));
#53756=CARTESIAN_POINT('Ctrl Pts',(53.6593972956249,26.9471093722017,5.99904235791355));
#53757=CARTESIAN_POINT('Ctrl Pts',(53.7283892553533,26.9036730942794,6.00326019233383));
#53758=CARTESIAN_POINT('Ctrl Pts',(53.7993719794597,26.8637784276219,6.00747802675412));
#53759=CARTESIAN_POINT('Ctrl Pts',(53.8703532265075,26.8238845911209,6.01169577340672));
#53760=CARTESIAN_POINT('Ctrl Pts',(53.9433247500623,26.787532445918,6.01591352005932));
#53761=CARTESIAN_POINT('Ctrl Pts',(54.0178961121557,26.7549115377159,6.02013126671192));
#53762=CARTESIAN_POINT('Ctrl Pts',(54.0925871803587,26.7222382646126,6.02435578392668));
#53763=CARTESIAN_POINT('Ctrl Pts',(54.1688827970325,26.6933083977567,6.02858030114144));
#53764=CARTESIAN_POINT('Ctrl Pts',(54.2463712968226,26.6682637310907,6.03280481835621));
#53765=CARTESIAN_POINT('Ctrl Pts',(54.3238475441992,26.6432230244653,6.03702866759402));
#53766=CARTESIAN_POINT('Ctrl Pts',(54.4025158421119,26.6220663907872,6.04125251683184));
#53767=CARTESIAN_POINT('Ctrl Pts',(54.4819520641742,26.6048848490758,6.04547636606966));
#53768=CARTESIAN_POINT('Ctrl Pts',(54.5615323588867,26.5876721453808,6.04970787605894));
#53769=CARTESIAN_POINT('Ctrl Pts',(54.641882901495,26.5744490174182,6.05393938604822));
#53770=CARTESIAN_POINT('Ctrl Pts',(54.7225714615492,26.5652549094303,6.0581708960375));
#53771=CARTESIAN_POINT('Ctrl Pts',(54.8030060754429,26.5560897374952,6.06238908845469));
#53772=CARTESIAN_POINT('Ctrl Pts',(54.8837761231954,26.5509282062687,6.06660728087188));
#53773=CARTESIAN_POINT('Ctrl Pts',(54.9644546244757,26.5497578127298,6.07082547328907));
#53774=CARTESIAN_POINT('Ctrl Pts',(55.0454104707045,26.5485833957803,6.07505816640148));
#53775=CARTESIAN_POINT('Ctrl Pts',(55.1265750617058,26.5514232685202,6.0792908595139));
#53776=CARTESIAN_POINT('Ctrl Pts',(55.2075175257847,26.558302490788,6.08352355262632));
#53777=CARTESIAN_POINT('Ctrl Pts',(55.2883445720611,26.5651719038076,6.08775021024003));
#53778=CARTESIAN_POINT('Ctrl Pts',(55.3689496614782,26.5760691876122,6.09197686785374));
#53779=CARTESIAN_POINT('Ctrl Pts',(55.4489010794414,26.5909673993745,6.09620352546745));
#53780=CARTESIAN_POINT('Ctrl Pts',(55.5287618547007,26.6058487207023,6.10042539122524));
#53781=CARTESIAN_POINT('Ctrl Pts',(55.6079699768964,26.62472187115,6.10464725698304));
#53782=CARTESIAN_POINT('Ctrl Pts',(55.6860994621945,26.6475081768524,6.10886912274083));
#53783=CARTESIAN_POINT('Ctrl Pts',(55.7641781934191,26.6702796802323,6.11308824591196));
#53784=CARTESIAN_POINT('Ctrl Pts',(55.8411792342355,26.6969591618318,6.11730736908308));
#53785=CARTESIAN_POINT('Ctrl Pts',(55.9166885752473,26.7274172609097,6.12152649225421));
#53786=CARTESIAN_POINT('Ctrl Pts',(55.9921732824894,26.7578654234978,6.12574423900082));
#53787=CARTESIAN_POINT('Ctrl Pts',(56.0661668259025,26.7920895818231,6.12996198574742));
#53788=CARTESIAN_POINT('Ctrl Pts',(56.1382734362833,26.8299115607304,6.13417973249403));
#53789=CARTESIAN_POINT('Ctrl Pts',(56.2103785674707,26.8677327637584,6.13839739271786));
#53790=CARTESIAN_POINT('Ctrl Pts',(56.2805964317636,26.9091514238056,6.1426150529417));
#53791=CARTESIAN_POINT('Ctrl Pts',(56.3485554944774,26.9539432245622,6.14683271316554));
#53792=CARTESIAN_POINT('Ctrl Pts',(56.4166269019741,26.9988090717364,6.15105734570629));
#53793=CARTESIAN_POINT('Ctrl Pts',(56.4824316475184,27.0470589586799,6.15528197824704));
#53794=CARTESIAN_POINT('Ctrl Pts',(56.5456266484317,27.0984247283745,6.15950661078779));
#53795=CARTESIAN_POINT('Ctrl Pts',(56.6088086988259,27.1497799717082,6.16373037757675));
#53796=CARTESIAN_POINT('Ctrl Pts',(56.6693817414734,27.2042494936698,6.16795414436571));
#53797=CARTESIAN_POINT('Ctrl Pts',(56.7270385517084,27.2615270807652,6.17217791115468));
#53798=CARTESIAN_POINT('Ctrl Pts',(56.7847999776588,27.3189085954924,6.17640934178044));
#53799=CARTESIAN_POINT('Ctrl Pts',(56.8396342828474,27.3791080133401,6.18064077240621));
#53800=CARTESIAN_POINT('Ctrl Pts',(56.8912730940144,27.441784246692,6.18487220303197));
#53801=CARTESIAN_POINT('Ctrl Pts',(56.942756547875,27.5042719162376,6.18909090323949));
#53802=CARTESIAN_POINT('Ctrl Pts',(56.9910635043335,27.5692211037456,6.193309603447));
#53803=CARTESIAN_POINT('Ctrl Pts',(57.0359719347866,27.6362666936819,6.19752830365451));
#53804=CARTESIAN_POINT('Ctrl Pts',(57.0810275402198,27.7035320070256,6.20176082948703));
#53805=CARTESIAN_POINT('Ctrl Pts',(57.1228298786424,27.7731577113981,6.20599335531954));
#53806=CARTESIAN_POINT('Ctrl Pts',(57.1611233504387,27.8447960724666,6.21022588115206));
#53807=CARTESIAN_POINT('Ctrl Pts',(57.1993621864955,27.9163322225145,6.21445236816991));
#53808=CARTESIAN_POINT('Ctrl Pts',(57.2341018819306,27.9898749196236,6.21867885518777));
#53809=CARTESIAN_POINT('Ctrl Pts',(57.2651299963173,28.0650474077348,6.22290534220562));
#53810=CARTESIAN_POINT('Ctrl Pts',(57.2961244944811,28.1401384530909,6.22712725019789));
#53811=CARTESIAN_POINT('Ctrl Pts',(57.3234152239855,28.2168553542244,6.23134915819015));
#53812=CARTESIAN_POINT('Ctrl Pts',(57.3468362310893,28.2947979336057,6.23557106618242));
#53813=CARTESIAN_POINT('Ctrl Pts',(57.3702408052715,28.3726858260007,6.23979001195009));
#53814=CARTESIAN_POINT('Ctrl Pts',(57.3897809176813,28.451797244378,6.24400895771777));
#53815=CARTESIAN_POINT('Ctrl Pts',(57.4053396763186,28.5317145192005,6.24822790348545));
#53816=CARTESIAN_POINT('Ctrl Pts',(57.4208933509156,28.6116056799446,6.25244547065406));
#53817=CARTESIAN_POINT('Ctrl Pts',(57.4324681666575,28.6923017185284,6.25666303782267));
#53818=CARTESIAN_POINT('Ctrl Pts',(57.4399981075099,28.7733736878736,6.26088060499129));
#53819=CARTESIAN_POINT('Ctrl Pts',(57.4475278904343,28.8544439568688,6.26509808370343));
#53820=CARTESIAN_POINT('Ctrl Pts',(57.4510129253457,28.9358896782611,6.26931556241557));
#53821=CARTESIAN_POINT('Ctrl Pts',(57.4504390935952,29.0172771114578,6.27353304112771));
#53822=CARTESIAN_POINT('Ctrl Pts',(57.4498642601189,29.0988066209528,6.27775788220206));
#53823=CARTESIAN_POINT('Ctrl Pts',(57.4452163859456,29.1802771715604,6.28198272327642));
#53824=CARTESIAN_POINT('Ctrl Pts',(57.4365336294594,29.2612548995014,6.28620756435077));
#53825=CARTESIAN_POINT('Ctrl Pts',(57.4278534598131,29.3422085018761,6.29043114672491));
#53826=CARTESIAN_POINT('Ctrl Pts',(57.4151409058698,29.4226691180841,6.29465472909906));
#53827=CARTESIAN_POINT('Ctrl Pts',(57.3984855618914,29.5022123648403,6.2988783114732));
#53828=CARTESIAN_POINT('Ctrl Pts',(57.3817999973935,29.5818999399418,6.30310955738485));
#53829=CARTESIAN_POINT('Ctrl Pts',(57.3611574638559,29.6606663683786,6.3073408032965));
#53830=CARTESIAN_POINT('Ctrl Pts',(57.3366979597814,29.7381008703108,6.31157204920816));
#53831=CARTESIAN_POINT('Ctrl Pts',(57.3123052282629,29.8153239820362,6.31579174414543));
#53832=CARTESIAN_POINT('Ctrl Pts',(57.284116575546,29.8912220316634,6.3200114390827));
#53833=CARTESIAN_POINT('Ctrl Pts',(57.252317547349,29.9654097140095,6.32423113401997));
#53834=CARTESIAN_POINT('Ctrl Pts',(57.2204209466352,30.0398250347235,6.32846377671943));
#53835=CARTESIAN_POINT('Ctrl Pts',(57.1847731140317,30.1127962601899,6.3326964194189));
#53836=CARTESIAN_POINT('Ctrl Pts',(57.1455266185094,30.1839196675737,6.33692906211837));
#53837=CARTESIAN_POINT('Ctrl Pts',(57.1063361015515,30.2549416293075,6.34115566766065));
#53838=CARTESIAN_POINT('Ctrl Pts',(57.063557338833,30.3241206042606,6.34538227320293));
#53839=CARTESIAN_POINT('Ctrl Pts',(57.0173907381963,30.3910732760857,6.34960887874521));
#53840=CARTESIAN_POINT('Ctrl Pts',(56.9712757696119,30.45795106902,6.35383075731355));
#53841=CARTESIAN_POINT('Ctrl Pts',(56.9217807544136,30.5226071259286,6.3580526358819));
#53842=CARTESIAN_POINT('Ctrl Pts',(56.8691510261793,30.5846844137975,6.36227451445024));
#53843=CARTESIAN_POINT('Ctrl Pts',(56.8165563413487,30.6467203676233,6.36649358188883));
#53844=CARTESIAN_POINT('Ctrl Pts',(56.7608313881616,30.7061806089203,6.37071264932742));
#53845=CARTESIAN_POINT('Ctrl Pts',(56.7022629062671,30.7627396994302,6.374931716766));
#53846=CARTESIAN_POINT('Ctrl Pts',(56.6437135491964,30.8192803212584,6.37914940651954));
#53847=CARTESIAN_POINT('Ctrl Pts',(56.5823228413088,30.8729213512001,6.38336709627308));
#53848=CARTESIAN_POINT('Ctrl Pts',(56.5184146778387,30.9233738888017,6.38758478602662));
#53849=CARTESIAN_POINT('Ctrl Pts',(56.4545078433777,30.973825377212,6.39180238807073));
#53850=CARTESIAN_POINT('Ctrl Pts',(56.388084022765,31.0210882181935,6.39601999011485));
#53851=CARTESIAN_POINT('Ctrl Pts',(56.3194993840789,31.0649144353739,6.40023759215896));
#53852=CARTESIAN_POINT('Ctrl Pts',(56.2507993594464,31.1088143852391,6.4044622898445));
#53853=CARTESIAN_POINT('Ctrl Pts',(56.1799316369248,31.1492658922123,6.40868698753004));
#53854=CARTESIAN_POINT('Ctrl Pts',(56.1072808730711,31.1860648019057,6.41291168521558));
#53855=CARTESIAN_POINT('Ctrl Pts',(56.0346471581031,31.2228550760339,6.41713539149533));
#53856=CARTESIAN_POINT('Ctrl Pts',(55.9602316729672,31.2559942966441,6.42135909777508));
#53857=CARTESIAN_POINT('Ctrl Pts',(55.884439195495,31.2853265761095,6.42558280405483));
#53858=CARTESIAN_POINT('Ctrl Pts',(55.8085092107296,31.314712071969,6.42981417323778));
#53859=CARTESIAN_POINT('Ctrl Pts',(55.7311976833491,31.340276677446,6.43404554242073));
#53860=CARTESIAN_POINT('Ctrl Pts',(55.6529254204302,31.3619141909384,6.43827691160367));
#53861=CARTESIAN_POINT('Ctrl Pts',(55.5748816383604,31.3834885433917,6.44249592919759));
#53862=CARTESIAN_POINT('Ctrl Pts',(55.4958831844018,31.4011586816502,6.44671494679151));
#53863=CARTESIAN_POINT('Ctrl Pts',(55.4163540516912,31.4148705045282,6.45093396438542));
#53864=CARTESIAN_POINT('Ctrl Pts',(55.3365684865941,31.4286265395754,6.45516658570811));
#53865=CARTESIAN_POINT('Ctrl Pts',(55.2559520888206,31.4384498229009,6.45939920703079));
#53866=CARTESIAN_POINT('Ctrl Pts',(55.1749265656419,31.4442485443655,6.46363182835347));
#53867=CARTESIAN_POINT('Ctrl Pts',(55.0940166135156,31.4500389948024,6.4678584124612));
#53868=CARTESIAN_POINT('Ctrl Pts',(55.0126991545164,31.4518162517646,6.47208499656892));
#53869=CARTESIAN_POINT('Ctrl Pts',(54.9314048223081,31.4495397428083,6.47631158067665));
#53870=CARTESIAN_POINT('Ctrl Pts',(54.8502008937526,31.447265765452,6.48053346459641));
#53871=CARTESIAN_POINT('Ctrl Pts',(54.7690205029077,31.4409469926296,6.48475534851617));
#53872=CARTESIAN_POINT('Ctrl Pts',(54.6882967024528,31.430594845773,6.48897723243593));
#53873=CARTESIAN_POINT('Ctrl Pts',(54.6076271634176,31.420249657486,6.49319627846385));
#53874=CARTESIAN_POINT('Ctrl Pts',(54.5274140648117,31.4058765386067,6.49741532449176));
#53875=CARTESIAN_POINT('Ctrl Pts',(54.4480864902674,31.387538843197,6.50163437051967));
#53876=CARTESIAN_POINT('Ctrl Pts',(54.3687848182123,31.3692071355156,6.50585203892077));
#53877=CARTESIAN_POINT('Ctrl Pts',(54.2903685482559,31.3469135267206,6.51006970732187));
#53878=CARTESIAN_POINT('Ctrl Pts',(54.2132563428266,31.3207724291489,6.51428737572297));
#53879=CARTESIAN_POINT('Ctrl Pts',(54.1361457393862,31.2946318746526,6.51850495650295));
#53880=CARTESIAN_POINT('Ctrl Pts',(54.060339586184,31.2646441405596,6.52272253728292));
#53881=CARTESIAN_POINT('Ctrl Pts',(53.9862397868842,31.2309729895952,6.5269401180629));
#53882=CARTESIAN_POINT('Ctrl Pts',(53.9120145030126,31.1972448180991,6.53116484112023));
#53883=CARTESIAN_POINT('Ctrl Pts',(53.8395017796366,31.1598209428222,6.53538956417756));
#53884=CARTESIAN_POINT('Ctrl Pts',(53.7690822829628,31.1189128872806,6.5396142872349));
#53885=CARTESIAN_POINT('Ctrl Pts',(53.698680081529,31.0780148788804,6.54383797268755));
#53886=CARTESIAN_POINT('Ctrl Pts',(53.6303704580546,31.0336346732078,6.54806165814021));
#53887=CARTESIAN_POINT('Ctrl Pts',(53.5645045325747,30.9860269416605,6.55228534359286));
#53888=CARTESIAN_POINT('Ctrl Pts',(53.4985191018522,30.9383328320131,6.55651669237904));
#53889=CARTESIAN_POINT('Ctrl Pts',(53.4349865933773,30.8873997850312,6.56074804116522));
#53890=CARTESIAN_POINT('Ctrl Pts',(53.3742251754706,30.8335229668391,6.56497938995139));
#53891=CARTESIAN_POINT('Ctrl Pts',(53.3136391463264,30.7798016649071,6.56919852488455));
#53892=CARTESIAN_POINT('Ctrl Pts',(53.2558084985499,30.7231539414781,6.57341765981771));
#53893=CARTESIAN_POINT('Ctrl Pts',(53.2010094579426,30.6639060308768,6.57763679475087));
#53894=CARTESIAN_POINT('Ctrl Pts',(53.1466819577936,30.6051679428309,6.58181962443494));
#53895=CARTESIAN_POINT('Ctrl Pts',(53.0951215203334,30.5436441968321,6.586002454119));
#53896=CARTESIAN_POINT('Ctrl Pts',(53.0466317199121,30.4796292144812,6.59018528380306));
#53897=CARTESIAN_POINT('Ctrl Pts',(52.9982051281647,30.4156976785894,6.5943626609772));
#53898=CARTESIAN_POINT('Ctrl Pts',(52.9528415189243,30.3492817231138,6.59854003815135));
#53899=CARTESIAN_POINT('Ctrl Pts',(52.9108068780089,30.2807116572536,6.6027174153255));
#53900=CARTESIAN_POINT('Ctrl Pts',(52.8688134471183,30.2122088162835,6.60689069707232));
#53901=CARTESIAN_POINT('Ctrl Pts',(52.8301427563659,30.1415564588635,6.61106397881914));
#53902=CARTESIAN_POINT('Ctrl Pts',(52.7950188390088,30.0691156764701,6.61523726056597));
#53903=CARTESIAN_POINT('Ctrl Pts',(52.7599180112606,29.9967225148847,6.61940779889889));
#53904=CARTESIAN_POINT('Ctrl Pts',(52.7283595353419,29.9225436897306,6.62357833723182));
#53905=CARTESIAN_POINT('Ctrl Pts',(52.7005218406598,29.8469654330122,6.62774887556475));
#53906=CARTESIAN_POINT('Ctrl Pts',(52.6726854079696,29.7713906025524,6.63191922483083));
#53907=CARTESIAN_POINT('Ctrl Pts',(52.6485696008035,29.6944169078521,6.63608957409691));
#53908=CARTESIAN_POINT('Ctrl Pts',(52.6283044779146,29.616449998394,6.64025992336299));
#53909=CARTESIAN_POINT('Ctrl Pts',(52.6080403381833,29.5384868714822,6.64443007030555));
#53910=CARTESIAN_POINT('Ctrl Pts',(52.5916266234608,29.4595310888085,6.64860021724811));
#53911=CARTESIAN_POINT('Ctrl Pts',(52.5791428075995,29.3800009263184,6.65277036419067));
#53912=CARTESIAN_POINT('Ctrl Pts',(52.5666493497683,29.300409338104,6.65694373197786));
#53913=CARTESIAN_POINT('Ctrl Pts',(52.5580919153856,29.2202429568221,6.66111709976505));
#53914=CARTESIAN_POINT('Ctrl Pts',(52.5534982586824,29.1399266941298,6.66529046755224));
#53915=CARTESIAN_POINT('Ctrl Pts',(52.5507897714393,29.0925710498201,6.66775114629748));
#53916=CARTESIAN_POINT('Ctrl Pts',(52.5494582852881,29.0451633717764,6.67021182504271));
#53917=CARTESIAN_POINT('Ctrl Pts',(52.5495009959572,28.9977906594942,6.67267250378794));
#53918=CARTESIAN_POINT('',(52.5495001736462,29.000922518181,7.4726725038354));
#53919=CARTESIAN_POINT('Ctrl Pts',(52.5495009959581,28.9977906585885,6.67267250383499));
#53920=CARTESIAN_POINT('Ctrl Pts',(52.5495959625876,28.8924580785088,6.67814378948657));
#53921=CARTESIAN_POINT('Ctrl Pts',(52.5564861340281,28.7874253985664,6.68361507513816));
#53922=CARTESIAN_POINT('Ctrl Pts',(52.5700336860443,28.6834341094806,6.68908636078975));
#53923=CARTESIAN_POINT('Ctrl Pts',(52.5826233164065,28.5867958467944,6.69417078223194));
#53924=CARTESIAN_POINT('Ctrl Pts',(52.6009615687309,28.4910563695803,6.69925520367413));
#53925=CARTESIAN_POINT('Ctrl Pts',(52.6249018375165,28.3967927648248,6.70433962511632));
#53926=CARTESIAN_POINT('Ctrl Pts',(52.6448313475172,28.318321321146,6.70857224375928));
#53927=CARTESIAN_POINT('Ctrl Pts',(52.6686910508689,28.2406926949251,6.71280486240224));
#53928=CARTESIAN_POINT('Ctrl Pts',(52.6963930578618,28.1643294272666,6.7170374810452));
#53929=CARTESIAN_POINT('Ctrl Pts',(52.7240555509065,28.0880750836366,6.72126406231066));
#53930=CARTESIAN_POINT('Ctrl Pts',(52.7555493052408,28.0130829468798,6.72549064357613));
#53931=CARTESIAN_POINT('Ctrl Pts',(52.7907359996734,27.9397628440482,6.7297172248416));
#53932=CARTESIAN_POINT('Ctrl Pts',(52.8258835939987,27.8665242158742,6.7339391094516));
#53933=CARTESIAN_POINT('Ctrl Pts',(52.8647157744081,27.7949543464672,6.73816099406161));
#53934=CARTESIAN_POINT('Ctrl Pts',(52.9070457472336,27.7254440985868,6.74238287867162));
#53935=CARTESIAN_POINT('Ctrl Pts',(52.949347227252,27.6559806388794,6.74660192148098));
#53936=CARTESIAN_POINT('Ctrl Pts',(52.9951415827039,27.588574443057,6.75082096429035));
#53937=CARTESIAN_POINT('Ctrl Pts',(53.0441962059324,27.5235915981305,6.75504000709972));
#53938=CARTESIAN_POINT('Ctrl Pts',(53.0932348099817,27.4586299738713,6.75925767214694));
#53939=CARTESIAN_POINT('Ctrl Pts',(53.1455312877731,27.3960904993885,6.76347533719416));
#53940=CARTESIAN_POINT('Ctrl Pts',(53.2008106434059,27.3363089502199,6.76769300224139));
#53941=CARTESIAN_POINT('Ctrl Pts',(53.2560888489012,27.2765286448609,6.77191057953624));
#53942=CARTESIAN_POINT('Ctrl Pts',(53.3143494925917,27.2195064910066,6.7761281568311));
#53943=CARTESIAN_POINT('Ctrl Pts',(53.3752793311667,27.165542860063,6.78034573412596));
#53944=CARTESIAN_POINT('Ctrl Pts',(53.4363124558048,27.11148775192,6.78457046090561));
#53945=CARTESIAN_POINT('Ctrl Pts',(53.5000234786206,27.0605018496433,6.78879518768526));
#53946=CARTESIAN_POINT('Ctrl Pts',(53.5660641828255,27.0128466787326,6.79301991446491));
#53947=CARTESIAN_POINT('Ctrl Pts',(53.6320885500798,26.9652032966146,6.79724359614437));
#53948=CARTESIAN_POINT('Ctrl Pts',(53.7004410435558,26.9208892339441,6.80146727782383));
#53949=CARTESIAN_POINT('Ctrl Pts',(53.7707460734318,26.8801214577206,6.80569095950329));
#53950=CARTESIAN_POINT('Ctrl Pts',(53.8411786604362,26.8392797149477,6.8099223043714));
#53951=CARTESIAN_POINT('Ctrl Pts',(53.9135704493358,26.8019973303931,6.81415364923951));
#53952=CARTESIAN_POINT('Ctrl Pts',(53.9875222855814,26.7684446841259,6.81838499410761));
#53953=CARTESIAN_POINT('Ctrl Pts',(54.0612610565873,26.7349887075696,6.822604147899));
#53954=CARTESIAN_POINT('Ctrl Pts',(54.1365504435938,26.7052410961928,6.82682330169039));
#53955=CARTESIAN_POINT('Ctrl Pts',(54.2129799915444,26.6793212724958,6.83104245548178));
#53956=CARTESIAN_POINT('Ctrl Pts',(54.289653381695,26.6533187537286,6.83527507013706));
#53957=CARTESIAN_POINT('Ctrl Pts',(54.3677593952038,26.6310718024977,6.83950768479234));
#53958=CARTESIAN_POINT('Ctrl Pts',(54.4468957476006,26.6127367267145,6.84374029944763));
#53959=CARTESIAN_POINT('Ctrl Pts',(54.5259192198373,26.594427804099,6.84796687669778));
#53960=CARTESIAN_POINT('Ctrl Pts',(54.6059696631954,26.5800197785084,6.85219345394793));
#53961=CARTESIAN_POINT('Ctrl Pts',(54.6866280030571,26.5696197331422,6.85642003119808));
#53962=CARTESIAN_POINT('Ctrl Pts',(54.7671968095085,26.5592312321683,6.86064191680846));
#53963=CARTESIAN_POINT('Ctrl Pts',(54.8483717132538,26.5528419303845,6.86486380241884));
#53964=CARTESIAN_POINT('Ctrl Pts',(54.9297231573378,26.5505079270621,6.86908568802922));
#53965=CARTESIAN_POINT('Ctrl Pts',(55.0110197454567,26.548175497578,6.87330472678652));
#53966=CARTESIAN_POINT('Ctrl Pts',(55.092492174327,26.5498929488533,6.87752376554382));
#53967=CARTESIAN_POINT('Ctrl Pts',(55.1737067298302,26.5556644620651,6.88174280430112));
#53968=CARTESIAN_POINT('Ctrl Pts',(55.2548947639566,26.5614340905349,6.88596046529164));
#53969=CARTESIAN_POINT('Ctrl Pts',(55.3358246289293,26.5712551188676,6.89017812628216));
#53970=CARTESIAN_POINT('Ctrl Pts',(55.4160649604304,26.5850796703199,6.89439578727268));
#53971=CARTESIAN_POINT('Ctrl Pts',(55.4963036224758,26.5989039341429,6.89861336051184));
#53972=CARTESIAN_POINT('Ctrl Pts',(55.5758523219702,26.6167314754395,6.902830933751));
#53973=CARTESIAN_POINT('Ctrl Pts',(55.6542885705336,26.6384630605326,6.90704850699016));
#53974=CARTESIAN_POINT('Ctrl Pts',(55.7328579460629,26.6602315298475,6.91127323856158));
#53975=CARTESIAN_POINT('Ctrl Pts',(55.8103106429316,26.6859171757245,6.915497970133));
#53976=CARTESIAN_POINT('Ctrl Pts',(55.8862377155446,26.7153702791161,6.91972270170442));
#53977=CARTESIAN_POINT('Ctrl Pts',(55.9621458473569,26.7448160351235,6.92394637937246));
#53978=CARTESIAN_POINT('Ctrl Pts',(56.0365286989947,26.7780271597654,6.9281700570405));
#53979=CARTESIAN_POINT('Ctrl Pts',(56.1089998023546,26.814806716014,6.93239373470853));
#53980=CARTESIAN_POINT('Ctrl Pts',(56.1816023939653,26.851653003405,6.93662507562389));
#53981=CARTESIAN_POINT('Ctrl Pts',(56.252285901021,26.8920804299587,6.94085641653923));
#53982=CARTESIAN_POINT('Ctrl Pts',(56.3206901050759,26.9358469300087,6.94508775745459));
#53983=CARTESIAN_POINT('Ctrl Pts',(56.3888976522279,26.9794876046877,6.94930693358547));
#53984=CARTESIAN_POINT('Ctrl Pts',(56.4548386619489,27.0264478475014,6.95352610971635));
#53985=CARTESIAN_POINT('Ctrl Pts',(56.5181895023843,27.0764483669914,6.95774528584723));
#53986=CARTESIAN_POINT('Ctrl Pts',(56.5817420932002,27.1266081207356,6.9619778985858));
#53987=CARTESIAN_POINT('Ctrl Pts',(56.6429243445553,27.1800141267647,6.96621051132437));
#53988=CARTESIAN_POINT('Ctrl Pts',(56.7013861374598,27.2364140334933,6.97044312406294));
#53989=CARTESIAN_POINT('Ctrl Pts',(56.7597645397355,27.2927334906931,6.97466969935003));
#53990=CARTESIAN_POINT('Ctrl Pts',(56.8154298591745,27.3520380468987,6.97889627463712));
#53991=CARTESIAN_POINT('Ctrl Pts',(56.868064127092,27.4140344685107,6.98312284992422));
#53992=CARTESIAN_POINT('Ctrl Pts',(56.9206399996994,27.4759621079319,6.98734473601957));
#53993=CARTESIAN_POINT('Ctrl Pts',(56.9701912035291,27.5405753262528,6.99156662211492));
#53994=CARTESIAN_POINT('Ctrl Pts',(57.0164368293783,27.6075443406963,6.99578850821027));
#53995=CARTESIAN_POINT('Ctrl Pts',(57.0626512435225,27.6744681569815,7.00000754490613));
#53996=CARTESIAN_POINT('Ctrl Pts',(57.1055642473226,27.7437442303109,7.00422658160198));
#53997=CARTESIAN_POINT('Ctrl Pts',(57.1449362190998,27.8150110270581,7.00844561829784));
#53998=CARTESIAN_POINT('Ctrl Pts',(57.1842953332791,27.886254550401,7.01266327719433));
#53999=CARTESIAN_POINT('Ctrl Pts',(57.2201154874759,27.9594870997823,7.01688093609082));
#54000=CARTESIAN_POINT('Ctrl Pts',(57.2522020067175,28.0343207722346,7.02109859498731));
#54001=CARTESIAN_POINT('Ctrl Pts',(57.2842878581498,28.1091528871909,7.02531616610263));
#54002=CARTESIAN_POINT('Ctrl Pts',(57.3126400471418,28.1855856315427,7.02953373721796));
#54003=CARTESIAN_POINT('Ctrl Pts',(57.3371118102645,28.2632105888913,7.03375130833328));
#54004=CARTESIAN_POINT('Ctrl Pts',(57.3616251347899,28.3409673799001,7.03797604232323));
#54005=CARTESIAN_POINT('Ctrl Pts',(57.3822447073948,28.4199199896435,7.04220077631318));
#54006=CARTESIAN_POINT('Ctrl Pts',(57.398873485459,28.4996438760623,7.04642551030313));
#54007=CARTESIAN_POINT('Ctrl Pts',(57.4154980972208,28.5793477878437,7.05064918579564));
#54008=CARTESIAN_POINT('Ctrl Pts',(57.4281338626529,28.6598221260562,7.05487286128815));
#54009=CARTESIAN_POINT('Ctrl Pts',(57.4367355838727,28.7406354991745,7.05909653678066));
#54010=CARTESIAN_POINT('Ctrl Pts',(57.4453529116408,28.8215954961812,7.06332787550637));
#54011=CARTESIAN_POINT('Ctrl Pts',(57.4499215419352,28.9028952922429,7.06755921423208));
#54012=CARTESIAN_POINT('Ctrl Pts',(57.4504484222488,28.9841009466281,7.07179055295779));
#54013=CARTESIAN_POINT('Ctrl Pts',(57.4509737895403,29.0650734058319,7.07600974070942));
#54014=CARTESIAN_POINT('Ctrl Pts',(57.4474806916846,29.1459518120799,7.08022892846104));
#54015=CARTESIAN_POINT('Ctrl Pts',(57.4400272205332,29.2263126444922,7.08444811621268));
#54016=CARTESIAN_POINT('Ctrl Pts',(57.4325500295491,29.3069292162051,7.08868073105426));
#54017=CARTESIAN_POINT('Ctrl Pts',(57.4210593812124,29.3873247478163,7.09291334589584));
#54018=CARTESIAN_POINT('Ctrl Pts',(57.4055763497897,29.4670681698986,7.09714596073742));
#54019=CARTESIAN_POINT('Ctrl Pts',(57.3901154034242,29.5466978456486,7.10137253816046));
#54020=CARTESIAN_POINT('Ctrl Pts',(57.3706734722897,29.6256768070676,7.10559911558351));
#54021=CARTESIAN_POINT('Ctrl Pts',(57.3473234261653,29.7035786970735,7.10982569300656));
#54022=CARTESIAN_POINT('Ctrl Pts',(57.3239993005622,29.7813941094085,7.11404757857204));
#54023=CARTESIAN_POINT('Ctrl Pts',(57.2967758129541,29.858134383322,7.11826946413752));
#54024=CARTESIAN_POINT('Ctrl Pts',(57.2657766664408,29.9333843516004,7.122491349703));
#54025=CARTESIAN_POINT('Ctrl Pts',(57.2347984215653,30.0085835814629,7.12671038859903));
#54026=CARTESIAN_POINT('Ctrl Pts',(57.2000497504312,30.0822940730062,7.13092942749507));
#54027=CARTESIAN_POINT('Ctrl Pts',(57.1617034667217,30.1541180060824,7.1351484663911));
#54028=CARTESIAN_POINT('Ctrl Pts',(57.1233697054719,30.2259184841526,7.13936612750708));
#54029=CARTESIAN_POINT('Ctrl Pts',(57.0814408834396,30.2958332177653,7.14358378862307));
#54030=CARTESIAN_POINT('Ctrl Pts',(57.0361364025847,30.3634877337436,7.14780144973905));
#54031=CARTESIAN_POINT('Ctrl Pts',(56.990832864466,30.4311408419062,7.15201902309015));
#54032=CARTESIAN_POINT('Ctrl Pts',(56.9421540666431,30.4965334406053,7.15623659644126));
#54033=CARTESIAN_POINT('Ctrl Pts',(56.8903627013274,30.5593200785695,7.16045416979237));
#54034=CARTESIAN_POINT('Ctrl Pts',(56.838483435925,30.6222132777509,7.16467890119119));
#54035=CARTESIAN_POINT('Ctrl Pts',(56.7834813308738,30.6824913069132,7.16890363259));
#54036=CARTESIAN_POINT('Ctrl Pts',(56.7256596719692,30.7398416440985,7.17312836398881));
#54037=CARTESIAN_POINT('Ctrl Pts',(56.667852433859,30.7971776780375,7.1773520417343));
#54038=CARTESIAN_POINT('Ctrl Pts',(56.6072274092363,30.8515871846148,7.18157571947978));
#54039=CARTESIAN_POINT('Ctrl Pts',(56.5441218547341,30.9027974006007,7.18579939722527));
#54040=CARTESIAN_POINT('Ctrl Pts',(56.480901804728,30.954100529794,7.19003073819652));
#54041=CARTESIAN_POINT('Ctrl Pts',(56.4151926066136,31.0021924928793,7.19426207916778));
#54042=CARTESIAN_POINT('Ctrl Pts',(56.3473620433452,31.0468428796937,7.19849342013903));
#54043=CARTESIAN_POINT('Ctrl Pts',(56.2797264991382,31.09136489257,7.20271259561873));
#54044=CARTESIAN_POINT('Ctrl Pts',(56.2099822061629,31.1324649329676,7.20693177109843));
#54045=CARTESIAN_POINT('Ctrl Pts',(56.1385160459505,31.1699611662685,7.21115094657812));
#54046=CARTESIAN_POINT('Ctrl Pts',(56.0668222555387,31.2075768305705,7.21538356075038));
#54047=CARTESIAN_POINT('Ctrl Pts',(55.993128950007,31.2417055725833,7.21961617492265));
#54048=CARTESIAN_POINT('Ctrl Pts',(55.9178091939508,31.2721303953558,7.22384878909491));
#54049=CARTESIAN_POINT('Ctrl Pts',(55.8425968744201,31.3025118199891,7.22807536584239));
#54050=CARTESIAN_POINT('Ctrl Pts',(55.7657631392959,31.3291996461331,7.23230194258988));
#54051=CARTESIAN_POINT('Ctrl Pts',(55.6877052978712,31.3520228896165,7.23652851933737));
#54052=CARTESIAN_POINT('Ctrl Pts',(55.6097340916694,31.3748208019255,7.24075040507096));
#54053=CARTESIAN_POINT('Ctrl Pts',(55.5305419223693,31.393762524576,7.24497229080455));
#54054=CARTESIAN_POINT('Ctrl Pts',(55.4505443868852,31.4087258053681,7.24919417653814));
#54055=CARTESIAN_POINT('Ctrl Pts',(55.3706008071098,31.4236789939191,7.25341321474855));
#54056=CARTESIAN_POINT('Ctrl Pts',(55.2898533954299,31.4346589847455,7.25763225295896));
#54057=CARTESIAN_POINT('Ctrl Pts',(55.2087299332046,31.4415941646769,7.26185129116937));
#54058=CARTESIAN_POINT('Ctrl Pts',(55.1276329629106,31.4485270798344,7.26606895159749));
#54059=CARTESIAN_POINT('Ctrl Pts',(55.0461606484581,31.4514177677565,7.2702866120256));
#54060=CARTESIAN_POINT('Ctrl Pts',(54.9647465498802,31.4502464048039,7.27450427245371));
#54061=CARTESIAN_POINT('Ctrl Pts',(54.883334145465,31.4490750662265,7.27872184511566));
#54062=CARTESIAN_POINT('Ctrl Pts',(54.8019804189986,31.4438418526952,7.28293941777761));
#54063=CARTESIAN_POINT('Ctrl Pts',(54.7211181534601,31.4345790530748,7.28715699043955));
#54064=CARTESIAN_POINT('Ctrl Pts',(54.640118620063,31.4253005293751,7.29138172264822));
#54065=CARTESIAN_POINT('Ctrl Pts',(54.5596126807539,31.4119787866303,7.29560645485689));
#54066=CARTESIAN_POINT('Ctrl Pts',(54.4800275962078,31.394698091471,7.29983118706556));
#54067=CARTESIAN_POINT('Ctrl Pts',(54.400462388443,31.3774217122534,7.30405486412579));
#54068=CARTESIAN_POINT('Ctrl Pts',(54.3218180200224,31.3561884999339,7.30827854118603));
#54069=CARTESIAN_POINT('Ctrl Pts',(54.2445068942906,31.3311328613414,7.31250221824626));
#54070=CARTESIAN_POINT('Ctrl Pts',(54.1670554990246,31.3060317630207,7.31673355854006));
#54071=CARTESIAN_POINT('Ctrl Pts',(54.0909426161636,31.2770945441863,7.32096489883387));
#54072=CARTESIAN_POINT('Ctrl Pts',(54.0165617407828,31.2445042749587,7.32519623912767));
#54073=CARTESIAN_POINT('Ctrl Pts',(53.9423946386715,31.2120076713187,7.32941541839964));
#54074=CARTESIAN_POINT('Ctrl Pts',(53.8699499719123,31.1758792648432,7.33363459767161));
#54075=CARTESIAN_POINT('Ctrl Pts',(53.7995908876004,31.1363445913213,7.33785377694359));
#54076=CARTESIAN_POINT('Ctrl Pts',(53.729007765659,31.096684031361,7.34208639094018));
#54077=CARTESIAN_POINT('Ctrl Pts',(53.6602610241045,31.0534479446395,7.34631900493677));
#54078=CARTESIAN_POINT('Ctrl Pts',(53.593735782111,31.0068311337741,7.35055161893336));
#54079=CARTESIAN_POINT('Ctrl Pts',(53.5273054321829,30.9602808174503,7.35477819550006));
#54080=CARTESIAN_POINT('Ctrl Pts',(53.4630906655255,30.9103596190429,7.35900477206677));
#54081=CARTESIAN_POINT('Ctrl Pts',(53.4014512034721,30.8573077276314,7.36323134863347));
#54082=CARTESIAN_POINT('Ctrl Pts',(53.3398801508463,30.8043147148895,7.36745323441162));
#54083=CARTESIAN_POINT('Ctrl Pts',(53.2808790739997,30.7481982145639,7.37167512018977));
#54084=CARTESIAN_POINT('Ctrl Pts',(53.2247767725121,30.6892402856277,7.37589700596792));
#54085=CARTESIAN_POINT('Ctrl Pts',(53.1687123133251,30.6303221251788,7.38011604398642));
#54086=CARTESIAN_POINT('Ctrl Pts',(53.115543065524,30.5685666783409,7.38433508200491));
#54087=CARTESIAN_POINT('Ctrl Pts',(53.0655619845638,30.5042937925935,7.38855412002341));
#54088=CARTESIAN_POINT('Ctrl Pts',(53.0155972256271,30.4400418960589,7.39277178025584));
#54089=CARTESIAN_POINT('Ctrl Pts',(52.9688188508445,30.3732745597009,7.39698944048826));
#54090=CARTESIAN_POINT('Ctrl Pts',(52.9254795192243,30.3043446725625,7.40120710072068));
#54091=CARTESIAN_POINT('Ctrl Pts',(52.8821410894974,30.235416219858,7.40542467318341));
#54092=CARTESIAN_POINT('Ctrl Pts',(52.8422418069139,30.1643256997478,7.40964224564614));
#54093=CARTESIAN_POINT('Ctrl Pts',(52.8059901941722,30.0914537195554,7.41385981810887));
#54094=CARTESIAN_POINT('Ctrl Pts',(52.7696770388051,30.0184580280952,7.41808455054222));
#54095=CARTESIAN_POINT('Ctrl Pts',(52.7370241509763,29.9436752437499,7.42230928297556));
#54096=CARTESIAN_POINT('Ctrl Pts',(52.7081934468242,29.8675096384598,7.42653401540891));
#54097=CARTESIAN_POINT('Ctrl Pts',(52.6793699462255,29.7913630636794,7.43075769226328));
#54098=CARTESIAN_POINT('Ctrl Pts',(52.654366842397,29.7138348090581,7.43498136911765));
#54099=CARTESIAN_POINT('Ctrl Pts',(52.6332959042206,29.6353439800776,7.43920504597202));
#54100=CARTESIAN_POINT('Ctrl Pts',(52.6121867359721,29.5567107412045,7.44343638605756));
#54101=CARTESIAN_POINT('Ctrl Pts',(52.5950240892831,29.4771118931882,7.4476677261431));
#54102=CARTESIAN_POINT('Ctrl Pts',(52.581868619362,29.396977173114,7.45189906622864));
#54103=CARTESIAN_POINT('Ctrl Pts',(52.5687509546984,29.317072738522,7.45611824658877));
#54104=CARTESIAN_POINT('Ctrl Pts',(52.5596174351928,29.2366359693903,7.4603374269489));
#54105=CARTESIAN_POINT('Ctrl Pts',(52.5544765733145,29.1560942648932,7.46455660730903));
#54106=CARTESIAN_POINT('Ctrl Pts',(52.5511803009539,29.1044516803041,7.46726190613533));
#54107=CARTESIAN_POINT('Ctrl Pts',(52.549519667232,29.0527035916731,7.46996720496163));
#54108=CARTESIAN_POINT('Ctrl Pts',(52.5495001736465,29.0009225190894,7.47267250378794));
#54109=CARTESIAN_POINT('',(52.5495004479559,29.0014816989085,8.27267250375952));
#54110=CARTESIAN_POINT('Ctrl Pts',(52.5495001736462,29.000922518181,7.4726725038354));
#54111=CARTESIAN_POINT('Ctrl Pts',(52.5494699637188,28.9206754040258,7.47686500918346));
#54112=CARTESIAN_POINT('Ctrl Pts',(52.553385810479,28.8402695844599,7.48105751453152));
#54113=CARTESIAN_POINT('Ctrl Pts',(52.5612682705951,28.7601296141792,7.48525001987958));
#54114=CARTESIAN_POINT('Ctrl Pts',(52.569139928792,28.6800994656379,7.48943677992691));
#54115=CARTESIAN_POINT('Ctrl Pts',(52.5809673631317,28.6003349110385,7.49362353997424));
#54116=CARTESIAN_POINT('Ctrl Pts',(52.5967191103635,28.5212608063798,7.49781030002156));
#54117=CARTESIAN_POINT('Ctrl Pts',(52.6124543520702,28.4422695598069,7.50199267295727));
#54118=CARTESIAN_POINT('Ctrl Pts',(52.6321056463101,28.3639677887937,7.50617504589298));
#54119=CARTESIAN_POINT('Ctrl Pts',(52.6555898647205,28.2867739715918,7.51035741882869));
#54120=CARTESIAN_POINT('Ctrl Pts',(52.6790611159983,28.2096227780129,7.51453748240992));
#54121=CARTESIAN_POINT('Ctrl Pts',(52.7063609543197,28.1335787769367,7.51871754599115));
#54122=CARTESIAN_POINT('Ctrl Pts',(52.737355744061,28.0590477052122,7.52289760957238));
#54123=CARTESIAN_POINT('Ctrl Pts',(52.7683433358281,27.9845339419688,7.52707670241014));
#54124=CARTESIAN_POINT('Ctrl Pts',(52.803023993077,27.9115328479399,7.5312557952479));
#54125=CARTESIAN_POINT('Ctrl Pts',(52.8412156020801,27.8404310398696,7.53543488808566));
#54126=CARTESIAN_POINT('Ctrl Pts',(52.8794105604764,27.7693229961913,7.53961434742865));
#54127=CARTESIAN_POINT('Ctrl Pts',(52.9211168554604,27.7001149856384,7.54379380677165));
#54128=CARTESIAN_POINT('Ctrl Pts',(52.9661067479375,27.6331684488517,7.54797326611464));
#54129=CARTESIAN_POINT('Ctrl Pts',(53.0111431277268,27.5661527373152,7.55215704402388));
#54130=CARTESIAN_POINT('Ctrl Pts',(53.0594696106475,27.5014035566214,7.55634082193313));
#54131=CARTESIAN_POINT('Ctrl Pts',(53.1108159391139,27.4392521555056,7.56052459984237));
#54132=CARTESIAN_POINT('Ctrl Pts',(53.162192422478,27.3770642538416,7.5647108348191));
#54133=CARTESIAN_POINT('Ctrl Pts',(53.2165919598393,27.3174775163968,7.56889706979584));
#54134=CARTESIAN_POINT('Ctrl Pts',(53.2737066682083,27.260787079564,7.57308330477257));
#54135=CARTESIAN_POINT('Ctrl Pts',(53.3309146588018,27.2040040534455,7.57727637689024));
#54136=CARTESIAN_POINT('Ctrl Pts',(53.3908463167065,27.1501270827268,7.58146944900791));
#54137=CARTESIAN_POINT('Ctrl Pts',(53.4531603921842,27.0994112812888,7.58566252112559));
#54138=CARTESIAN_POINT('Ctrl Pts',(53.4808860207514,27.0768461150342,7.58752815997522));
#54139=CARTESIAN_POINT('Ctrl Pts',(53.5090829004989,27.0549061785739,7.58939379882486));
#54140=CARTESIAN_POINT('Ctrl Pts',(53.5377192653921,27.0336111007244,7.59125943767449));
#54141=CARTESIAN_POINT('Ctrl Pts',(53.6026871897314,26.985298508966,7.59549205183763));
#54142=CARTESIAN_POINT('Ctrl Pts',(53.6701728177024,26.9401192630011,7.59972466600077));
#54143=CARTESIAN_POINT('Ctrl Pts',(53.7398413913357,26.8983457632119,7.60395728016392));
#54144=CARTESIAN_POINT('Ctrl Pts',(53.8094105892923,26.8566318493967,7.6081838569005));
#54145=CARTESIAN_POINT('Ctrl Pts',(53.8811561534627,26.8183142700959,7.61241043363708));
#54146=CARTESIAN_POINT('Ctrl Pts',(53.9547122171902,26.7836237455909,7.61663701037366));
#54147=CARTESIAN_POINT('Ctrl Pts',(54.0281866423831,26.7489717234668,7.62085889610975));
#54148=CARTESIAN_POINT('Ctrl Pts',(54.1034671563318,26.7179389544352,7.62508078184585));
#54149=CARTESIAN_POINT('Ctrl Pts',(54.1801622451278,26.6907108657238,7.62930266758195));
#54150=CARTESIAN_POINT('Ctrl Pts',(54.2568056052848,26.6635011415778,7.63352170577713));
#54151=CARTESIAN_POINT('Ctrl Pts',(54.3348612087337,26.6400911561762,7.63774074397231));
#54152=CARTESIAN_POINT('Ctrl Pts',(54.4139176264464,26.6206182102467,7.64195978216749));
#54153=CARTESIAN_POINT('Ctrl Pts',(54.4929482272182,26.6011516234706,7.64617744257876));
#54154=CARTESIAN_POINT('Ctrl Pts',(54.5729785424699,26.5856196338783,7.65039510299004));
#54155=CARTESIAN_POINT('Ctrl Pts',(54.6535833767961,26.5741092825174,7.65461276340132));
#54156=CARTESIAN_POINT('Ctrl Pts',(54.7341865337694,26.5625991706822,7.65883033604485));
#54157=CARTESIAN_POINT('Ctrl Pts',(54.8153637259979,26.5551105951925,7.66304790868838));
#54158=CARTESIAN_POINT('Ctrl Pts',(54.8966824173337,26.5516789983517,7.6672654813319));
#54159=CARTESIAN_POINT('Ctrl Pts',(54.978139152018,26.5482415761698,7.67149021355757));
#54160=CARTESIAN_POINT('Ctrl Pts',(55.0597373998212,26.5488749315336,7.67571494578324));
#54161=CARTESIAN_POINT('Ctrl Pts',(55.1410419922651,26.5535623027721,7.67993967800891));
#54162=CARTESIAN_POINT('Ctrl Pts',(55.2223262777186,26.5582485032722,7.684163355047));
#54163=CARTESIAN_POINT('Ctrl Pts',(55.3033165932996,26.5669866236706,7.68838703208508));
#54164=CARTESIAN_POINT('Ctrl Pts',(55.3835846454728,26.5797080610477,7.69261070912317));
#54165=CARTESIAN_POINT('Ctrl Pts',(55.4639983320443,26.5924525795739,7.69684204939274));
#54166=CARTESIAN_POINT('Ctrl Pts',(55.5436866803965,26.6091947624671,7.70107338966231));
#54167=CARTESIAN_POINT('Ctrl Pts',(55.6222325033254,26.6298149941818,7.70530472993188));
#54168=CARTESIAN_POINT('Ctrl Pts',(55.7005525850342,26.6503759632128,7.70952390930123));
#54169=CARTESIAN_POINT('Ctrl Pts',(55.7777362908384,26.6747925031437,7.71374308867058));
#54170=CARTESIAN_POINT('Ctrl Pts',(55.8533898045263,26.7028983279945,7.71796226803993));
#54171=CARTESIAN_POINT('Ctrl Pts',(55.9292842153978,26.7310936478828,7.7221948821908));
#54172=CARTESIAN_POINT('Ctrl Pts',(56.0039209366839,26.7631066770454,7.72642749634167));
#54173=CARTESIAN_POINT('Ctrl Pts',(56.0768892295648,26.7988049070454,7.73066011049255));
#54174=CARTESIAN_POINT('Ctrl Pts',(56.1497534400199,26.8344522168686,7.73488668721632));
#54175=CARTESIAN_POINT('Ctrl Pts',(56.2209535349518,26.8737740848049,7.73911326394009));
#54176=CARTESIAN_POINT('Ctrl Pts',(56.2900968022657,26.9165892169849,7.74333984066387));
#54177=CARTESIAN_POINT('Ctrl Pts',(56.359163328988,26.9593568295913,7.7475617264031));
#54178=CARTESIAN_POINT('Ctrl Pts',(56.4261771710985,27.0056097593228,7.75178361214233));
#54179=CARTESIAN_POINT('Ctrl Pts',(56.4907696470691,27.0551205411704,7.75600549788156));
#54180=CARTESIAN_POINT('Ctrl Pts',(56.5553185570041,27.1045979292139,7.76022453606275));
#54181=CARTESIAN_POINT('Ctrl Pts',(56.6174489766366,27.1573285233817,7.76444357424394));
#54182=CARTESIAN_POINT('Ctrl Pts',(56.6768217523575,27.2130419532567,7.76866261242513));
#54183=CARTESIAN_POINT('Ctrl Pts',(56.7361751390909,27.2687371891532,7.77288027282201));
#54184=CARTESIAN_POINT('Ctrl Pts',(56.792772331843,27.3274130086463,7.77709793321888));
#54185=CARTESIAN_POINT('Ctrl Pts',(56.846308841665,27.3887601323237,7.78131559361576));
#54186=CARTESIAN_POINT('Ctrl Pts',(56.8998442374095,27.4501059793872,7.78553316624449));
#54187=CARTESIAN_POINT('Ctrl Pts',(56.9503187722974,27.5141226693279,7.78975073887322));
#54188=CARTESIAN_POINT('Ctrl Pts',(56.9974672434017,27.5804666747353,7.79396831150194));
#54189=CARTESIAN_POINT('Ctrl Pts',(57.0446957522071,27.6469233035544,7.7981930437439));
#54190=CARTESIAN_POINT('Ctrl Pts',(57.0885866299451,27.7157147717585,7.80241777598585));
#54191=CARTESIAN_POINT('Ctrl Pts',(57.1289170306517,27.7864669239773,7.8066425082278));
#54192=CARTESIAN_POINT('Ctrl Pts',(57.1692373579566,27.857201404295,7.81086618525025));
#54193=CARTESIAN_POINT('Ctrl Pts',(57.2059987952204,27.9298951637249,7.8150898622727));
#54194=CARTESIAN_POINT('Ctrl Pts',(57.239025724956,28.0041515913629,7.81931353929515));
#54195=CARTESIAN_POINT('Ctrl Pts',(57.2721125771228,28.0785427461979,7.82354487954871));
#54196=CARTESIAN_POINT('Ctrl Pts',(57.3014512128808,28.1545018007412,7.82777621980226));
#54197=CARTESIAN_POINT('Ctrl Pts',(57.326914851716,28.2316136890446,7.83200756005582));
#54198=CARTESIAN_POINT('Ctrl Pts',(57.3523053084635,28.3085039590237,7.83622673950567));
#54199=CARTESIAN_POINT('Ctrl Pts',(57.3738429709623,28.3865399841882,7.84044591895553));
#54200=CARTESIAN_POINT('Ctrl Pts',(57.3914529302185,28.4653008953164,7.84466509840538));
#54201=CARTESIAN_POINT('Ctrl Pts',(57.4091189632073,28.5443125973866,7.84889771259049));
#54202=CARTESIAN_POINT('Ctrl Pts',(57.422897918044,28.6243476817022,7.85313032677559));
#54203=CARTESIAN_POINT('Ctrl Pts',(57.432677339609,28.7049894724712,7.8573629409607));
#54204=CARTESIAN_POINT('Ctrl Pts',(57.4424428117479,28.7855162353014,7.86158951771929));
#54205=CARTESIAN_POINT('Ctrl Pts',(57.4482200259361,28.8666475284319,7.86581609447789));
#54206=CARTESIAN_POINT('Ctrl Pts',(57.4499472632695,28.9479552385142,7.87004267123648));
#54207=CARTESIAN_POINT('Ctrl Pts',(57.4516725835626,29.0291727061224,7.87426455696708));
#54208=CARTESIAN_POINT('Ctrl Pts',(57.4493568487837,29.1105657395192,7.87848644269768));
#54209=CARTESIAN_POINT('Ctrl Pts',(57.4429901518053,29.191701247211,7.88270832842828));
#54210=CARTESIAN_POINT('Ctrl Pts',(57.4366277489401,29.2727820318571,7.88692736664547));
#54211=CARTESIAN_POINT('Ctrl Pts',(57.4262198465732,29.353605173836,7.89114640486267));
#54212=CARTESIAN_POINT('Ctrl Pts',(57.4118086027381,29.4337389926658,7.89536544307987));
#54213=CARTESIAN_POINT('Ctrl Pts',(57.3974020650894,29.5138466427139,7.89958310351311));
#54214=CARTESIAN_POINT('Ctrl Pts',(57.3789948644423,29.5932649598001,7.90380076394635));
#54215=CARTESIAN_POINT('Ctrl Pts',(57.356680668146,29.671570158946,7.90801842437959));
#54216=CARTESIAN_POINT('Ctrl Pts',(57.3343669361993,29.7498737285918,7.91223599704499));
#54217=CARTESIAN_POINT('Ctrl Pts',(57.3081464986954,29.8270637799121,7.9164535697104));
#54218=CARTESIAN_POINT('Ctrl Pts',(57.2781631384104,29.9027308373974,7.9206711423758));
#54219=CARTESIAN_POINT('Ctrl Pts',(57.2481288799168,29.9785263433832,7.92489587457538));
#54220=CARTESIAN_POINT('Ctrl Pts',(57.2143190902924,30.0527932486888,7.92912060677497));
#54221=CARTESIAN_POINT('Ctrl Pts',(57.1769263029716,30.1251409340302,7.93334533897456));
#54222=CARTESIAN_POINT('Ctrl Pts',(57.1395428546162,30.1974705503114,7.93756901603409));
#54223=CARTESIAN_POINT('Ctrl Pts',(57.0985784508561,30.2678815129337,7.94179269309362));
#54224=CARTESIAN_POINT('Ctrl Pts',(57.0542701726253,30.3360105942177,7.94601637015315));
#54225=CARTESIAN_POINT('Ctrl Pts',(57.0098815036429,30.404263285542,7.95024771044373));
#54226=CARTESIAN_POINT('Ctrl Pts',(56.9621371087501,30.4702254442061,7.95447905073432));
#54227=CARTESIAN_POINT('Ctrl Pts',(56.9113161363247,30.5335647612751,7.9587103910249));
#54228=CARTESIAN_POINT('Ctrl Pts',(56.8606412254153,30.5967220386029,7.96292957027355));
#54229=CARTESIAN_POINT('Ctrl Pts',(56.8069077621599,30.6572712452121,7.96714874952219));
#54230=CARTESIAN_POINT('Ctrl Pts',(56.7504280017128,30.7149204240488,7.97136792877084));
#54231=CARTESIAN_POINT('Ctrl Pts',(56.6937683956003,30.7727531722711,7.97560054294012));
#54232=CARTESIAN_POINT('Ctrl Pts',(56.6341342221795,30.8278824714284,7.97983315710941));
#54233=CARTESIAN_POINT('Ctrl Pts',(56.5718137789544,30.8799871526926,7.98406577127869));
#54234=CARTESIAN_POINT('Ctrl Pts',(56.5095822299898,30.9320175115214,7.98829234802129));
#54235=CARTESIAN_POINT('Ctrl Pts',(56.4446723749273,30.9810315257815,7.99251892476389));
#54236=CARTESIAN_POINT('Ctrl Pts',(56.3774097262184,31.0267443588472,7.99674550150648));
#54237=CARTESIAN_POINT('Ctrl Pts',(56.3102217312172,31.0724064559912,8.00096738724106));
#54238=CARTESIAN_POINT('Ctrl Pts',(56.2406865135504,31.1147743923521,8.00518927297563));
#54239=CARTESIAN_POINT('Ctrl Pts',(56.1691619678421,31.1536040822193,8.00941115871021));
#54240=CARTESIAN_POINT('Ctrl Pts',(56.0976856632683,31.1924075826396,8.01363019691104));
#54241=CARTESIAN_POINT('Ctrl Pts',(56.02422310268,31.2276773551747,8.01784923511188));
#54242=CARTESIAN_POINT('Ctrl Pts',(55.9491593414199,31.2592137558441,8.02206827331271));
#54243=CARTESIAN_POINT('Ctrl Pts',(55.8741200932473,31.2907398578749,8.0262859337295));
#54244=CARTESIAN_POINT('Ctrl Pts',(55.7974811107954,31.3185348294661,8.0305035941463));
#54245=CARTESIAN_POINT('Ctrl Pts',(55.7196488681722,31.3424465322689,8.03472125456309));
#54246=CARTESIAN_POINT('Ctrl Pts',(55.6418182452084,31.3663577374782,8.03893882721197));
#54247=CARTESIAN_POINT('Ctrl Pts',(55.5627948558531,31.3863856992659,8.04315639986085));
#54248=CARTESIAN_POINT('Ctrl Pts',(55.4830004539498,31.4024281074539,8.04737397250973));
#54249=CARTESIAN_POINT('Ctrl Pts',(55.4030705965005,31.4184977485442,8.05159870472861));
#54250=CARTESIAN_POINT('Ctrl Pts',(55.3223675656575,31.4305682073941,8.05582343694749));
#54251=CARTESIAN_POINT('Ctrl Pts',(55.2413238380958,31.4385883324511,8.06004816916637));
#54252=CARTESIAN_POINT('Ctrl Pts',(55.1603003521452,31.4466064543888,8.06427184620937));
#54253=CARTESIAN_POINT('Ctrl Pts',(55.0789368062758,31.4505762640251,8.06849552325237));
#54254=CARTESIAN_POINT('Ctrl Pts',(54.9976669520771,31.4504988893871,8.07271920029537));
#54255=CARTESIAN_POINT('Ctrl Pts',(54.9162496458658,31.4504213743644,8.07695054056955));
#54256=CARTESIAN_POINT('Ctrl Pts',(54.8349268363389,31.4462820239938,8.08118188084373));
#54257=CARTESIAN_POINT('Ctrl Pts',(54.7541292412137,31.438134085725,8.08541322111791));
#54258=CARTESIAN_POINT('Ctrl Pts',(54.6735638595754,31.4300095647516,8.08963240045737));
#54259=CARTESIAN_POINT('Ctrl Pts',(54.5935211151077,31.4178996169355,8.09385157979683));
#54260=CARTESIAN_POINT('Ctrl Pts',(54.5144159007389,31.4019072281303,8.09807075913629));
#54261=CARTESIAN_POINT('Ctrl Pts',(54.4350587973182,31.3858639159103,8.10230337330545));
#54262=CARTESIAN_POINT('Ctrl Pts',(54.3563500583321,31.3658537017414,8.10653598747461));
#54263=CARTESIAN_POINT('Ctrl Pts',(54.2787160376896,31.3419435722736,8.11076860164377));
#54264=CARTESIAN_POINT('Ctrl Pts',(54.2011927546892,31.3180675483609,8.11499517838617));
#54265=CARTESIAN_POINT('Ctrl Pts',(54.1247415856073,31.2903027933118,8.11922175512857));
#54266=CARTESIAN_POINT('Ctrl Pts',(54.0497786678322,31.2587672898936,8.12344833187097));
#54267=CARTESIAN_POINT('Ctrl Pts',(53.9748989501626,31.2272667872103,8.12767021760559));
#54268=CARTESIAN_POINT('Ctrl Pts',(53.9015046277485,31.1920040311541,8.13189210334021));
#54269=CARTESIAN_POINT('Ctrl Pts',(53.8299952839634,31.1531463523068,8.13611398907482));
#54270=CARTESIAN_POINT('Ctrl Pts',(53.7585341710649,31.114314881787,8.14033302727537));
#54271=CARTESIAN_POINT('Ctrl Pts',(53.6889559188865,31.0718935253044,8.14455206547593));
#54272=CARTESIAN_POINT('Ctrl Pts',(53.6216376182746,31.0260965906502,8.14877110367648));
#54273=CARTESIAN_POINT('Ctrl Pts',(53.5543413013658,30.9803146116055,8.15298876409294));
#54274=CARTESIAN_POINT('Ctrl Pts',(53.489303854164,30.9311595046703,8.15720642450941));
#54275=CARTESIAN_POINT('Ctrl Pts',(53.4268741789863,30.8788894063409,8.16142408492587));
#54276=CARTESIAN_POINT('Ctrl Pts',(53.3644458029471,30.8266203957329,8.16564165757438));
#54277=CARTESIAN_POINT('Ctrl Pts',(53.3046254464679,30.7712368217353,8.16985923022289));
#54278=CARTESIAN_POINT('Ctrl Pts',(53.2477285330397,30.7130367643681,8.1740768028714));
#54279=CARTESIAN_POINT('Ctrl Pts',(53.1907350338482,30.6547379090763,8.17830153509059));
#54280=CARTESIAN_POINT('Ctrl Pts',(53.1366752333902,30.5936133383991,8.18252626730979));
#54281=CARTESIAN_POINT('Ctrl Pts',(53.0858274795292,30.5299979777354,8.18675099952899));
#54282=CARTESIAN_POINT('Ctrl Pts',(53.0349924254941,30.4663985057579,8.19097467657151));
#54283=CARTESIAN_POINT('Ctrl Pts',(52.9873680690511,30.4003098784601,8.19519835361404));
#54284=CARTESIAN_POINT('Ctrl Pts',(52.9431895986978,30.3320965517166,8.19942203065656));
#54285=CARTESIAN_POINT('Ctrl Pts',(52.8989309731088,30.2637594620803,8.20365337093021));
#54286=CARTESIAN_POINT('Ctrl Pts',(52.8581309615497,30.1932903722078,8.20788471120387));
#54287=CARTESIAN_POINT('Ctrl Pts',(52.8209793817891,30.1210795669407,8.21211605147752));
#54288=CARTESIAN_POINT('Ctrl Pts',(52.7839345761983,30.049076296557,8.21633523081893));
#54289=CARTESIAN_POINT('Ctrl Pts',(52.750517371286,29.9753417578273,8.22055441016033));
#54290=CARTESIAN_POINT('Ctrl Pts',(52.7208672479652,29.9002800389891,8.22477358950174));
#54291=CARTESIAN_POINT('Ctrl Pts',(52.6873086607357,29.8153237232269,8.22954893888001));
#54292=CARTESIAN_POINT('Ctrl Pts',(52.6584702201738,29.7284032433861,8.23432428825828));
#54293=CARTESIAN_POINT('Ctrl Pts',(52.6345571909943,29.6400238802757,8.23909963763655));
#54294=CARTESIAN_POINT('Ctrl Pts',(52.6107313882432,29.5519668943989,8.24385756819817));
#54295=CARTESIAN_POINT('Ctrl Pts',(52.5917952654792,29.4624618606748,8.24861549875978));
#54296=CARTESIAN_POINT('Ctrl Pts',(52.5779051312006,29.3720305048458,8.2533734293214));
#54297=CARTESIAN_POINT('Ctrl Pts',(52.564101568475,29.2821627708467,8.25810170563859));
#54298=CARTESIAN_POINT('Ctrl Pts',(52.5552814037465,29.1913804539606,8.26282998195578));
#54299=CARTESIAN_POINT('Ctrl Pts',(52.5515500002522,29.1002140146641,8.26755825827297));
#54300=CARTESIAN_POINT('Ctrl Pts',(52.5502046676053,29.0673445629218,8.26926300676849));
#54301=CARTESIAN_POINT('Ctrl Pts',(52.5495203673848,29.0344253362664,8.270967755264));
#54302=CARTESIAN_POINT('Ctrl Pts',(52.5495004479559,29.0014816989085,8.27267250375952));
#54303=CARTESIAN_POINT('',(52.5495008396014,28.9979714818537,9.07267250383346));
#54304=CARTESIAN_POINT('Ctrl Pts',(52.5495004479556,29.0014816983595,8.27267250378793));
#54305=CARTESIAN_POINT('Ctrl Pts',(52.5494507665478,28.9193163462504,8.27692434941349));
#54306=CARTESIAN_POINT('Ctrl Pts',(52.5535379338215,28.837136673185,8.28117619503905));
#54307=CARTESIAN_POINT('Ctrl Pts',(52.5617397578869,28.7553834802586,8.28542804066461));
#54308=CARTESIAN_POINT('Ctrl Pts',(52.5699428094404,28.6736180521174,8.28968052262306));
#54309=CARTESIAN_POINT('Ctrl Pts',(52.582261695604,28.5922796825047,8.2939330045815));
#54310=CARTESIAN_POINT('Ctrl Pts',(52.5986224231266,28.5118033354378,8.29818548653995));
#54311=CARTESIAN_POINT('Ctrl Pts',(52.6157081009362,28.4277610497037,8.30262639765055));
#54312=CARTESIAN_POINT('Ctrl Pts',(52.6372020240865,28.3446594869578,8.30706730876115));
#54313=CARTESIAN_POINT('Ctrl Pts',(52.6629611688432,28.2629791375644,8.31150821987176));
#54314=CARTESIAN_POINT('Ctrl Pts',(52.6876730016431,28.1846197371921,8.31576857299608));
#54315=CARTESIAN_POINT('Ctrl Pts',(52.716309733793,28.1075686378834,8.32002892612039));
#54316=CARTESIAN_POINT('Ctrl Pts',(52.7486955163619,28.032230207151,8.32428927924471));
#54317=CARTESIAN_POINT('Ctrl Pts',(52.7811086573637,27.9568281330158,8.32855323137377));
#54318=CARTESIAN_POINT('Ctrl Pts',(52.8172769529868,27.8831420135458,8.33281718350283));
#54319=CARTESIAN_POINT('Ctrl Pts',(52.8569786237512,27.8115515867567,8.33708113563188));
#54320=CARTESIAN_POINT('Ctrl Pts',(52.8967483001918,27.7398385314915,8.34135239155804));
#54321=CARTESIAN_POINT('Ctrl Pts',(52.940063187104,27.6702287139669,8.3456236474842));
#54322=CARTESIAN_POINT('Ctrl Pts',(52.9866585870374,27.6030724410873,8.34989490341036));
#54323=CARTESIAN_POINT('Ctrl Pts',(52.9924095412518,27.5947837977644,8.35042207556264));
#54324=CARTESIAN_POINT('Ctrl Pts',(52.9982104195672,27.5865324869345,8.35094924771491));
#54325=CARTESIAN_POINT('Ctrl Pts',(53.0040606837377,27.5783191301145,8.35147641986719));
#54326=CARTESIAN_POINT('Ctrl Pts',(53.0510318883543,27.5123748834046,8.35570903403824));
#54327=CARTESIAN_POINT('Ctrl Pts',(53.1013620710945,27.4486383399154,8.35994164820929));
#54328=CARTESIAN_POINT('Ctrl Pts',(53.1548164171103,27.3874716140687,8.36417426238034));
#54329=CARTESIAN_POINT('Ctrl Pts',(53.2081945155205,27.3263921368131,8.3684008391247));
#54330=CARTESIAN_POINT('Ctrl Pts',(53.2646876232179,27.2678755437295,8.37262741586906));
#54331=CARTESIAN_POINT('Ctrl Pts',(53.3240185106077,27.2122538498952,8.37685399261342));
#54332=CARTESIAN_POINT('Ctrl Pts',(53.3832835475904,27.1566938896932,8.38107587834755));
#54333=CARTESIAN_POINT('Ctrl Pts',(53.4453797688037,27.1040227606304,8.38529776408169));
#54334=CARTESIAN_POINT('Ctrl Pts',(53.509991616305,27.054537261596,8.38951964981582));
#54335=CARTESIAN_POINT('Ctrl Pts',(53.5745598851104,27.0050851390024,8.39373868801841));
#54336=CARTESIAN_POINT('Ctrl Pts',(53.6416400425298,26.9588146608482,8.39795772622101));
#54337=CARTESIAN_POINT('Ctrl Pts',(53.7108827858705,26.9159829515489,8.40217676442359));
#54338=CARTESIAN_POINT('Ctrl Pts',(53.7801029170556,26.8731652295243,8.40639442484212));
#54339=CARTESIAN_POINT('Ctrl Pts',(53.8514838368787,26.8337842903864,8.41061208526065));
#54340=CARTESIAN_POINT('Ctrl Pts',(53.9246476931999,26.7980536640827,8.41482974567919));
#54341=CARTESIAN_POINT('Ctrl Pts',(53.997810027009,26.7623237813198,8.4190473183298));
#54342=CARTESIAN_POINT('Ctrl Pts',(54.0727548056031,26.7302442631621,8.42326489098041));
#54343=CARTESIAN_POINT('Ctrl Pts',(54.14908133029,26.7019817956468,8.42748246363102));
#54344=CARTESIAN_POINT('Ctrl Pts',(54.2255374235346,26.6736713510073,8.43170719584782));
#54345=CARTESIAN_POINT('Ctrl Pts',(54.3033795179171,26.6491910834525,8.43593192806462));
#54346=CARTESIAN_POINT('Ctrl Pts',(54.3821883625906,26.6286588118363,8.44015666028142));
#54347=CARTESIAN_POINT('Ctrl Pts',(54.4609775239111,26.6081316683748,8.44438033732611));
#54348=CARTESIAN_POINT('Ctrl Pts',(54.5407324919504,26.5915506230681,8.44860401437079));
#54349=CARTESIAN_POINT('Ctrl Pts',(54.6210246221457,26.5789820502565,8.45282769141548));
#54350=CARTESIAN_POINT('Ctrl Pts',(54.7014624304185,26.5663906736468,8.4570590316913));
#54351=CARTESIAN_POINT('Ctrl Pts',(54.7824388852395,26.5578263674288,8.46129037196712));
#54352=CARTESIAN_POINT('Ctrl Pts',(54.8635202295622,26.5533035492196,8.46552171224294));
#54353=CARTESIAN_POINT('Ctrl Pts',(54.9443685446839,26.548793729669,8.46974089157284));
#54354=CARTESIAN_POINT('Ctrl Pts',(55.0253206914566,26.5483021181239,8.47396007090274));
#54355=CARTESIAN_POINT('Ctrl Pts',(55.1059508059623,26.5517915373245,8.47817925023265));
#54356=CARTESIAN_POINT('Ctrl Pts',(55.1868376653727,26.5552920676417,8.48241186440388));
#54357=CARTESIAN_POINT('Ctrl Pts',(55.2677012780256,26.5628120689609,8.48664447857512));
#54358=CARTESIAN_POINT('Ctrl Pts',(55.3481100598163,26.574351708047,8.49087709274636));
#54359=CARTESIAN_POINT('Ctrl Pts',(55.4284041460295,26.5858748869214,8.49510366949089));
#54360=CARTESIAN_POINT('Ctrl Pts',(55.5082442339118,26.6014062503793,8.49933024623543));
#54361=CARTESIAN_POINT('Ctrl Pts',(55.5872008968254,26.6208940005188,8.50355682297996));
#54362=CARTESIAN_POINT('Ctrl Pts',(55.666069926992,26.6403601215137,8.50777870871405));
#54363=CARTESIAN_POINT('Ctrl Pts',(55.7440570316991,26.6637737932659,8.51200059444813));
#54364=CARTESIAN_POINT('Ctrl Pts',(55.8207414585528,26.691031895367,8.51622248018222));
#54365=CARTESIAN_POINT('Ctrl Pts',(55.8973741641327,26.7182716127214,8.52044151838499));
#54366=CARTESIAN_POINT('Ctrl Pts',(55.9727055002787,26.7493504554118,8.52466055658775));
#54367=CARTESIAN_POINT('Ctrl Pts',(56.0463296238771,26.7841153982671,8.52887959479051));
#54368=CARTESIAN_POINT('Ctrl Pts',(56.1199297045208,26.8188689881594,8.53309725520921));
#54369=CARTESIAN_POINT('Ctrl Pts',(56.1918232600546,26.857306089447,8.53731491562791));
#54370=CARTESIAN_POINT('Ctrl Pts',(56.2616254731621,26.8992259960985,8.54153257604661));
#54371=CARTESIAN_POINT('Ctrl Pts',(56.331426233712,26.9411450304126,8.54575014869739));
#54372=CARTESIAN_POINT('Ctrl Pts',(56.3991353407199,26.9865464858135,8.54996772134817));
#54373=CARTESIAN_POINT('Ctrl Pts',(56.4643948330412,27.0351849901423,8.55418529399896));
#54374=CARTESIAN_POINT('Ctrl Pts',(56.5297651070062,27.0839060610566,8.55841002621555));
#54375=CARTESIAN_POINT('Ctrl Pts',(56.5926770719442,27.1358748961834,8.56263475843215));
#54376=CARTESIAN_POINT('Ctrl Pts',(56.6528036579295,27.1908039580148,8.56685949064874));
#54377=CARTESIAN_POINT('Ctrl Pts',(56.712915226661,27.2457193007293,8.57108316769358));
#54378=CARTESIAN_POINT('Ctrl Pts',(56.7702424946668,27.3035930455017,8.57530684473841));
#54379=CARTESIAN_POINT('Ctrl Pts',(56.8244964310299,27.3641017687035,8.57953052178325));
#54380=CARTESIAN_POINT('Ctrl Pts',(56.8788488030569,27.4247202759456,8.58376186205921));
#54381=CARTESIAN_POINT('Ctrl Pts',(56.9301164064617,27.4879829538693,8.58799320233517));
#54382=CARTESIAN_POINT('Ctrl Pts',(56.9780510096974,27.5535338050839,8.59222454261113));
#54383=CARTESIAN_POINT('Ctrl Pts',(57.0258478480335,27.6188962619899,8.59644372194012));
#54384=CARTESIAN_POINT('Ctrl Pts',(57.0703306381617,27.6865333311812,8.60066290126911));
#54385=CARTESIAN_POINT('Ctrl Pts',(57.1112987246448,27.7560675479299,8.6048820805981));
#54386=CARTESIAN_POINT('Ctrl Pts',(57.15239726299,27.8258231777058,8.60911469476982));
#54387=CARTESIAN_POINT('Ctrl Pts',(57.190111512103,27.8977475107696,8.61334730894156));
#54388=CARTESIAN_POINT('Ctrl Pts',(57.224206377363,27.971478614273,8.61757992311328));
#54389=CARTESIAN_POINT('Ctrl Pts',(57.2582526094991,28.0451045472805,8.62180649985832));
#54390=CARTESIAN_POINT('Ctrl Pts',(57.2886895182319,28.1205317139537,8.62603307660336));
#54391=CARTESIAN_POINT('Ctrl Pts',(57.3153267727405,28.197371701576,8.6302596533484));
#54392=CARTESIAN_POINT('Ctrl Pts',(57.3419344629792,28.2741264057041,8.63448153908237));
#54393=CARTESIAN_POINT('Ctrl Pts',(57.364750727125,28.3522903783227,8.63870342481633));
#54394=CARTESIAN_POINT('Ctrl Pts',(57.3836330072357,28.4314545428757,8.6429253105503));
#54395=CARTESIAN_POINT('Ctrl Pts',(57.4025025518354,28.5105653136608,8.64714434875358));
#54396=CARTESIAN_POINT('Ctrl Pts',(57.417443274682,28.5906744858628,8.65136338695687));
#54397=CARTESIAN_POINT('Ctrl Pts',(57.4283625958313,28.6713583210128,8.65558242516015));
#54398=CARTESIAN_POINT('Ctrl Pts',(57.4392783511284,28.7520158077637,8.65980008557938));
#54399=CARTESIAN_POINT('Ctrl Pts',(57.4461752504949,28.8332471247745,8.66401774599861));
#54400=CARTESIAN_POINT('Ctrl Pts',(57.4490121563561,28.9146202130469,8.66823540641784));
#54401=CARTESIAN_POINT('Ctrl Pts',(57.4518490031823,28.9959916079761,8.67245297906914));
#54402=CARTESIAN_POINT('Ctrl Pts',(57.4506260094729,29.0775043039943,8.67667055172045));
#54403=CARTESIAN_POINT('Ctrl Pts',(57.4453541252492,29.158724453462,8.68088812437176));
#54404=CARTESIAN_POINT('Ctrl Pts',(57.4400732917081,29.2400824786609,8.68511285658774));
#54405=CARTESIAN_POINT('Ctrl Pts',(57.4307298461979,29.3211464976868,8.68933758880372));
#54406=CARTESIAN_POINT('Ctrl Pts',(57.4173869253028,29.401485620384,8.69356232101971));
#54407=CARTESIAN_POINT('Ctrl Pts',(57.4040473369403,29.4818046775536,8.69778599806508));
#54408=CARTESIAN_POINT('Ctrl Pts',(57.3867103907381,29.5613987494988,8.70200967511045));
#54409=CARTESIAN_POINT('Ctrl Pts',(57.3654900339305,29.6398493177111,8.70623335215583));
#54410=CARTESIAN_POINT('Ctrl Pts',(57.3442311759551,29.7184422227618,8.71046469243233));
#54411=CARTESIAN_POINT('Ctrl Pts',(57.3190749703805,29.7958870347219,8.71469603270884));
#54412=CARTESIAN_POINT('Ctrl Pts',(57.2901848993448,29.8717817254412,8.71892737298535));
#54413=CARTESIAN_POINT('Ctrl Pts',(57.261377858909,29.9474582934116,8.72314655231142));
#54414=CARTESIAN_POINT('Ctrl Pts',(57.2288586457946,30.0215932549045,8.72736573163748));
#54415=CARTESIAN_POINT('Ctrl Pts',(57.1928346499557,30.0938128029758,8.73158491096355));
#54416=CARTESIAN_POINT('Ctrl Pts',(57.1566959453605,30.1662623148349,8.73581752513496));
#54417=CARTESIAN_POINT('Ctrl Pts',(57.1168956679506,30.2370536433283,8.74005013930637));
#54418=CARTESIAN_POINT('Ctrl Pts',(57.0736094304284,30.3057925486226,8.74428275347778));
#54419=CARTESIAN_POINT('Ctrl Pts',(57.0303849366597,30.3744334043227,8.74850933022249));
#54420=CARTESIAN_POINT('Ctrl Pts',(56.9836846040812,30.4410272615588,8.7527359069672));
#54421=CARTESIAN_POINT('Ctrl Pts',(56.9337306268262,30.5052030138405,8.75696248371191));
#54422=CARTESIAN_POINT('Ctrl Pts',(56.8838320927002,30.5693075384699,8.76118436944595));
#54423=CARTESIAN_POINT('Ctrl Pts',(56.8306873731901,30.6309989261475,8.76540625518));
#54424=CARTESIAN_POINT('Ctrl Pts',(56.7745620033723,30.6899348940676,8.76962814091404));
#54425=CARTESIAN_POINT('Ctrl Pts',(56.7184744883772,30.7488311115038,8.773847179117));
#54426=CARTESIAN_POINT('Ctrl Pts',(56.6594106353566,30.8049752646763,8.77806621731995));
#54427=CARTESIAN_POINT('Ctrl Pts',(56.597675486232,30.8580590116283,8.7822852555229));
#54428=CARTESIAN_POINT('Ctrl Pts',(56.5359604975564,30.9111254233639,8.7865029159418));
#54429=CARTESIAN_POINT('Ctrl Pts',(56.471576297174,30.9611331110164,8.79072057636069));
#54430=CARTESIAN_POINT('Ctrl Pts',(56.4048629117432,31.007812354083,8.79493823677958));
#54431=CARTESIAN_POINT('Ctrl Pts',(56.3381509145928,31.0544906257723,8.79915580943055));
#54432=CARTESIAN_POINT('Ctrl Pts',(56.2691102100636,31.0978403252284,8.80337338208153));
#54433=CARTESIAN_POINT('Ctrl Pts',(56.1981106817008,31.1376344506006,8.8075909547325));
#54434=CARTESIAN_POINT('Ctrl Pts',(56.1269906276686,31.1774961287258,8.81181568694887));
#54435=CARTESIAN_POINT('Ctrl Pts',(56.0539055041992,31.2137899282438,8.81604041916525));
#54436=CARTESIAN_POINT('Ctrl Pts',(55.979251124433,31.2463342327661,8.82026515138162));
#54437=CARTESIAN_POINT('Ctrl Pts',(55.904615390384,31.2788704090057,8.82448882842666));
#54438=CARTESIAN_POINT('Ctrl Pts',(55.8284116273999,31.3076588181063,8.82871250547169));
#54439=CARTESIAN_POINT('Ctrl Pts',(55.7510529323302,31.3325672000691,8.83293618251673));
#54440=CARTESIAN_POINT('Ctrl Pts',(55.6735538814628,31.3575207745706,8.83716752279289));
#54441=CARTESIAN_POINT('Ctrl Pts',(55.594896160868,31.3785801327825,8.84139886306906));
#54442=CARTESIAN_POINT('Ctrl Pts',(55.515506001708,31.395663543197,8.84563020334522));
#54443=CARTESIAN_POINT('Ctrl Pts',(55.4363440112969,31.4126978555819,8.84984938267315));
#54444=CARTESIAN_POINT('Ctrl Pts',(55.3564542494899,31.4257790520627,8.85406856200107));
#54445=CARTESIAN_POINT('Ctrl Pts',(55.2762631782407,31.434877595763,8.858287741329));
#54446=CARTESIAN_POINT('Ctrl Pts',(55.1958167600599,31.4440051113323,8.86252035550045));
#54447=CARTESIAN_POINT('Ctrl Pts',(55.1147679047255,31.4491584908913,8.86675296967191));
#54448=CARTESIAN_POINT('Ctrl Pts',(55.0335429142519,31.4502704183219,8.87098558384337));
#54449=CARTESIAN_POINT('Ctrl Pts',(54.9524337836005,31.4513807596925,8.87521216058813));
#54450=CARTESIAN_POINT('Ctrl Pts',(54.8711494774509,31.4484610921686,8.8794387373329));
#54451=CARTESIAN_POINT('Ctrl Pts',(54.7901222519542,31.4414957671221,8.88366531407767));
#54452=CARTESIAN_POINT('Ctrl Pts',(54.7091849572946,31.4345381727798,8.8878871998117));
#54453=CARTESIAN_POINT('Ctrl Pts',(54.6285046368471,31.4235438825422,8.89210908554573));
#54454=CARTESIAN_POINT('Ctrl Pts',(54.5485129635736,31.4085492948949,8.89633097127977));
#54455=CARTESIAN_POINT('Ctrl Pts',(54.4685752422038,31.3935648206322,8.90055000948276));
#54456=CARTESIAN_POINT('Ctrl Pts',(54.389325700945,31.3745854929444,8.90476904768575));
#54457=CARTESIAN_POINT('Ctrl Pts',(54.3111890498774,31.3516993270806,8.90898808588874));
#54458=CARTESIAN_POINT('Ctrl Pts',(54.2330779153911,31.3288206350041,8.91320574630769));
#54459=CARTESIAN_POINT('Ctrl Pts',(54.1560793948241,31.3020377689536,8.91742340672663));
#54460=CARTESIAN_POINT('Ctrl Pts',(54.0806048473256,31.271489115809,8.92164106714557));
#54461=CARTESIAN_POINT('Ctrl Pts',(54.005131870424,31.2409410983705,8.92585863979659));
#54462=CARTESIAN_POINT('Ctrl Pts',(53.9311832337083,31.2066276250278,8.93007621244761));
#54463=CARTESIAN_POINT('Ctrl Pts',(53.8591507169577,31.1687353834394,8.93429378509862));
#54464=CARTESIAN_POINT('Ctrl Pts',(53.7869959209839,31.130778817653,8.93851851731494));
#54465=CARTESIAN_POINT('Ctrl Pts',(53.7167641662081,31.0892315460588,8.94274324953126));
#54466=CARTESIAN_POINT('Ctrl Pts',(53.6488232780315,31.0443267145959,8.94696798174758));
#54467=CARTESIAN_POINT('Ctrl Pts',(53.5808993588053,30.9994330985863,8.95119165879266));
#54468=CARTESIAN_POINT('Ctrl Pts',(53.5152655249853,30.9511838928963,8.95541533583774));
#54469=CARTESIAN_POINT('Ctrl Pts',(53.4522576098529,30.8998536111348,8.95963901288282));
#54470=CARTESIAN_POINT('Ctrl Pts',(53.3891353762696,30.8484301982439,8.96387035315904));
#54471=CARTESIAN_POINT('Ctrl Pts',(53.3286489288173,30.7939148494673,8.96810169343525));
#54472=CARTESIAN_POINT('Ctrl Pts',(53.2710988665349,30.7366206035583,8.97233303371146));
#54473=CARTESIAN_POINT('Ctrl Pts',(53.2137142041733,30.6794910223491,8.97655221303913));
#54474=CARTESIAN_POINT('Ctrl Pts',(53.1592493158241,30.6195988886482,8.98077139236679));
#54475=CARTESIAN_POINT('Ctrl Pts',(53.1079611439954,30.5572858496014,8.98499057169445));
#54476=CARTESIAN_POINT('Ctrl Pts',(53.0567614607749,30.4950803206081,8.98920247157944));
#54477=CARTESIAN_POINT('Ctrl Pts',(53.0085312255926,30.4302236210157,8.99341437146443));
#54478=CARTESIAN_POINT('Ctrl Pts',(52.9635585782611,30.3630321294181,8.99762627134942));
#54479=CARTESIAN_POINT('Ctrl Pts',(52.9186470371168,30.295931933666,9.00183244835266));
#54480=CARTESIAN_POINT('Ctrl Pts',(52.8769845582534,30.2265036275436,9.0060386253559));
#54481=CARTESIAN_POINT('Ctrl Pts',(52.8388195372745,30.1550970771038,9.01024480235913));
#54482=CARTESIAN_POINT('Ctrl Pts',(52.8006944219304,30.0837651898935,9.01444658135187));
#54483=CARTESIAN_POINT('Ctrl Pts',(52.7660597242993,30.0104595761678,9.0186483603446));
#54484=CARTESIAN_POINT('Ctrl Pts',(52.7351201108098,29.9355583025883,9.02285013933733));
#54485=CARTESIAN_POINT('Ctrl Pts',(52.7041994735316,29.8607029682508,9.02704934125049));
#54486=CARTESIAN_POINT('Ctrl Pts',(52.6769696037845,29.7842543477414,9.03124854316364));
#54487=CARTESIAN_POINT('Ctrl Pts',(52.6535882303907,29.7066130889241,9.0354477450768));
#54488=CARTESIAN_POINT('Ctrl Pts',(52.630216246542,29.62900300946,9.03964526066491));
#54489=CARTESIAN_POINT('Ctrl Pts',(52.6106898219177,29.5502016927393,9.04384277625303));
#54490=CARTESIAN_POINT('Ctrl Pts',(52.5951171935888,29.4706261121396,9.04804029184114));
#54491=CARTESIAN_POINT('Ctrl Pts',(52.5795387820052,29.3910209793131,9.05223936627346));
#54492=CARTESIAN_POINT('Ctrl Pts',(52.5679171975141,29.3106414678569,9.05643844070578));
#54493=CARTESIAN_POINT('Ctrl Pts',(52.5603095856078,29.2299150537103,9.0606375151381));
#54494=CARTESIAN_POINT('Ctrl Pts',(52.5530415138441,29.152791591254,9.06464917802138));
#54495=CARTESIAN_POINT('Ctrl Pts',(52.5494367842607,29.0753519218323,9.06866084090466));
#54496=CARTESIAN_POINT('Ctrl Pts',(52.5495008396007,28.9979714827317,9.07267250378794));
#54497=CARTESIAN_POINT('',(52.5495000016466,29.0000898342118,9.87267250383148));
#54498=CARTESIAN_POINT('Ctrl Pts',(52.5495008396014,28.9979714818537,9.07267250383347));
#54499=CARTESIAN_POINT('Ctrl Pts',(52.5495811640756,28.9009375672519,9.07770306915667));
#54500=CARTESIAN_POINT('Ctrl Pts',(52.5554288148724,28.8041502685366,9.08273363447987));
#54501=CARTESIAN_POINT('Ctrl Pts',(52.5669331831094,28.7082190641151,9.08776419980306));
#54502=CARTESIAN_POINT('Ctrl Pts',(52.5785831185121,28.611074022198,9.0928584179163));
#54503=CARTESIAN_POINT('Ctrl Pts',(52.5960337473273,28.5148069165952,9.09795263602954));
#54504=CARTESIAN_POINT('Ctrl Pts',(52.6191211193409,28.4200293062307,9.10304685414278));
#54505=CARTESIAN_POINT('Ctrl Pts',(52.6321833835234,28.3664064779398,9.10592903678181));
#54506=CARTESIAN_POINT('Ctrl Pts',(52.6470491004416,28.3132600501885,9.10881121942086));
#54507=CARTESIAN_POINT('Ctrl Pts',(52.6636818643731,28.2606977484539,9.1116934020599));
#54508=CARTESIAN_POINT('Ctrl Pts',(52.6881078224556,28.1835076564059,9.11592601623136));
#54509=CARTESIAN_POINT('Ctrl Pts',(52.7164087614872,28.1073858387591,9.12015863040283));
#54510=CARTESIAN_POINT('Ctrl Pts',(52.7484725483883,28.0327490580833,9.12439124457429));
#54511=CARTESIAN_POINT('Ctrl Pts',(52.7804905993079,27.9582187397671,9.12861782131907));
#54512=CARTESIAN_POINT('Ctrl Pts',(52.8162606560091,27.8851696745553,9.13284439806384));
#54513=CARTESIAN_POINT('Ctrl Pts',(52.8556209719017,27.8140030211455,9.13707097480862));
#54514=CARTESIAN_POINT('Ctrl Pts',(52.8949376024015,27.7429153544798,9.14129286054265));
#54515=CARTESIAN_POINT('Ctrl Pts',(52.9378363506593,27.6737063527297,9.14551474627668));
#54516=CARTESIAN_POINT('Ctrl Pts',(52.9841081722206,27.6067554454826,9.14973663201071));
#54517=CARTESIAN_POINT('Ctrl Pts',(53.0303487848731,27.5398496945465,9.15395567021372));
#54518=CARTESIAN_POINT('Ctrl Pts',(53.0799576889743,27.4751993944456,9.15817470841674));
#54519=CARTESIAN_POINT('Ctrl Pts',(53.1326815334158,27.4131565942559,9.16239374661975));
#54520=CARTESIAN_POINT('Ctrl Pts',(53.1853881601719,27.3511340549828,9.1666114070387));
#54521=CARTESIAN_POINT('Ctrl Pts',(53.2412074065279,27.2917176782871,9.17082906745765));
#54522=CARTESIAN_POINT('Ctrl Pts',(53.2998453534869,27.2352268055243,9.1750467278766));
#54523=CARTESIAN_POINT('Ctrl Pts',(53.3584820802124,27.1787371083153,9.17926430052763));
#54524=CARTESIAN_POINT('Ctrl Pts',(53.4199370555498,27.1251731154538,9.18348187317866));
#54525=CARTESIAN_POINT('Ctrl Pts',(53.4838802205191,27.074816615419,9.18769944582969));
#54526=CARTESIAN_POINT('Ctrl Pts',(53.5479319325845,27.0243746324112,9.19192417804599));
#54527=CARTESIAN_POINT('Ctrl Pts',(53.6144799183171,26.9771513251288,9.1961489102623));
#54528=CARTESIAN_POINT('Ctrl Pts',(53.6831614432795,26.9333876837844,9.20037364247861));
#54529=CARTESIAN_POINT('Ctrl Pts',(53.7518258143102,26.8896349728687,9.2045973195237));
#54530=CARTESIAN_POINT('Ctrl Pts',(53.8226222433147,26.8493404120462,9.2088209965688));
#54531=CARTESIAN_POINT('Ctrl Pts',(53.8951632431404,26.8126989254581,9.2130446736139));
#54532=CARTESIAN_POINT('Ctrl Pts',(53.9678358577752,26.7759909583657,9.21727601389013));
#54533=CARTESIAN_POINT('Ctrl Pts',(54.0422589430834,26.7429495003037,9.22150735416635));
#54534=CARTESIAN_POINT('Ctrl Pts',(54.1180241756887,26.7137216058996,9.22573869444258));
#54535=CARTESIAN_POINT('Ctrl Pts',(54.1935716576423,26.6845777129937,9.22995787377017));
#54536=CARTESIAN_POINT('Ctrl Pts',(54.2704531240852,26.6592255560931,9.23417705309777));
#54537=CARTESIAN_POINT('Ctrl Pts',(54.3482519025511,26.6377606667673,9.23839623242536));
#54538=CARTESIAN_POINT('Ctrl Pts',(54.4262984103412,26.6162274282639,9.24262884659684));
#54539=CARTESIAN_POINT('Ctrl Pts',(54.5055583653667,26.5985261909816,9.24686146076832));
#54540=CARTESIAN_POINT('Ctrl Pts',(54.5856211313313,26.5847897807435,9.2510940749398));
#54541=CARTESIAN_POINT('Ctrl Pts',(54.6655696952777,26.5710729642049,9.25532065168458));
#54542=CARTESIAN_POINT('Ctrl Pts',(54.7463183417245,26.5613098201536,9.25954722842937));
#54543=CARTESIAN_POINT('Ctrl Pts',(54.8274425136619,26.5555830625876,9.26377380517416));
#54544=CARTESIAN_POINT('Ctrl Pts',(54.9084766471625,26.5498626610593,9.26799569090819));
#54545=CARTESIAN_POINT('Ctrl Pts',(54.9898850169335,26.5481697769688,9.27221757664221));
#54546=CARTESIAN_POINT('Ctrl Pts',(55.0712355438955,26.5505356203272,9.27643946237624));
#54547=CARTESIAN_POINT('Ctrl Pts',(55.1525312024498,26.5528998679976,9.28065850057926));
#54548=CARTESIAN_POINT('Ctrl Pts',(55.2337686325249,26.5593173927617,9.28487753878228));
#54549=CARTESIAN_POINT('Ctrl Pts',(55.3145146019266,26.5697673331191,9.28909657698531));
#54550=CARTESIAN_POINT('Ctrl Pts',(55.3952342026387,26.580213860907,9.29331423740427));
#54551=CARTESIAN_POINT('Ctrl Pts',(55.4754622010538,26.5946901295471,9.29753189782324));
#54552=CARTESIAN_POINT('Ctrl Pts',(55.5547707158481,26.6131234420613,9.30174955824221));
#54553=CARTESIAN_POINT('Ctrl Pts',(55.6340775802621,26.6315563709852,9.30596713089325));
#54554=CARTESIAN_POINT('Ctrl Pts',(55.712464546878,26.6539460737477,9.3101847035443));
#54555=CARTESIAN_POINT('Ctrl Pts',(55.7895155600359,26.680169094425,9.31440227619534));
#54556=CARTESIAN_POINT('Ctrl Pts',(55.866697371594,26.7064366301451,9.31862700841163));
#54557=CARTESIAN_POINT('Ctrl Pts',(55.942538250152,26.7365503528518,9.32285174062792));
#54558=CARTESIAN_POINT('Ctrl Pts',(56.0166385741196,26.7703371870142,9.32707647284421));
#54559=CARTESIAN_POINT('Ctrl Pts',(56.0907203907542,26.8041155825603,9.33130014988932));
#54560=CARTESIAN_POINT('Ctrl Pts',(56.1630621179304,26.8415650218201,9.33552382693443));
#54561=CARTESIAN_POINT('Ctrl Pts',(56.2332893000427,26.8824665876543,9.33974750397954));
#54562=CARTESIAN_POINT('Ctrl Pts',(56.3036438988875,26.9234423632705,9.34397884425578));
#54563=CARTESIAN_POINT('Ctrl Pts',(56.3718758951069,26.9678825283198,9.34821018453202));
#54564=CARTESIAN_POINT('Ctrl Pts',(56.4376396439943,27.0155246275109,9.35244152480826));
#54565=CARTESIAN_POINT('Ctrl Pts',(56.5032143866743,27.0630298024444,9.35666070413577));
#54566=CARTESIAN_POINT('Ctrl Pts',(56.5663347477688,27.1137181813588,9.36087988346329));
#54567=CARTESIAN_POINT('Ctrl Pts',(56.6266937561611,27.1672922563413,9.3650990627908));
#54568=CARTESIAN_POINT('Ctrl Pts',(56.6872449616128,27.2210369235841,9.36933167696229));
#54569=CARTESIAN_POINT('Ctrl Pts',(56.745242389422,27.2778856055347,9.37356429113377));
#54570=CARTESIAN_POINT('Ctrl Pts',(56.8003510712067,27.3375661605932,9.37779690530526));
#54571=CARTESIAN_POINT('Ctrl Pts',(56.8553811456313,27.3971615869437,9.38202348205006));
#54572=CARTESIAN_POINT('Ctrl Pts',(56.9075303453909,27.4595805251693,9.38625005879485));
#54573=CARTESIAN_POINT('Ctrl Pts',(56.9564981587189,27.524511875707,9.39047663553964));
#54574=CARTESIAN_POINT('Ctrl Pts',(57.0054116234443,27.5893711599644,9.39469852127367));
#54575=CARTESIAN_POINT('Ctrl Pts',(57.0511504394666,27.6567369467867,9.39892040700769));
#54576=CARTESIAN_POINT('Ctrl Pts',(57.0934532028416,27.7262637880973,9.40314229274172));
#54577=CARTESIAN_POINT('Ctrl Pts',(57.1357274343147,27.7957437357096,9.40736133094475));
#54578=CARTESIAN_POINT('Ctrl Pts',(57.1745699750768,27.8673814471224,9.41158036914778));
#54579=CARTESIAN_POINT('Ctrl Pts',(57.2097624723251,27.9408021592243,9.41579940735081));
#54580=CARTESIAN_POINT('Ctrl Pts',(57.2449434769868,28.0141988947985,9.42001706776978));
#54581=CARTESIAN_POINT('Ctrl Pts',(57.276476604675,28.0893770561332,9.42423472818876));
#54582=CARTESIAN_POINT('Ctrl Pts',(57.304189896511,28.1659381492859,9.42845238860773));
#54583=CARTESIAN_POINT('Ctrl Pts',(57.3319026116439,28.2424976492313,9.43266996125878));
#54584=CARTESIAN_POINT('Ctrl Pts',(57.3557954919589,28.3204395865649,9.43688753390983));
#54585=CARTESIAN_POINT('Ctrl Pts',(57.3757455943626,28.3993477537987,9.44110510656089));
#54586=CARTESIAN_POINT('Ctrl Pts',(57.3957295631798,28.4783898720553,9.44532983877717));
#54587=CARTESIAN_POINT('Ctrl Pts',(57.4117572483169,28.5584010491796,9.44955457099345));
#54588=CARTESIAN_POINT('Ctrl Pts',(57.4237562755797,28.6389518500418,9.45377930320973));
#54589=CARTESIAN_POINT('Ctrl Pts',(57.4357523059595,28.719482532497,9.45800298025485));
#54590=CARTESIAN_POINT('Ctrl Pts',(57.4437216661573,28.800552103174,9.46222665729996));
#54591=CARTESIAN_POINT('Ctrl Pts',(57.4476441354587,28.8817272805974,9.46645033434508));
#54592=CARTESIAN_POINT('Ctrl Pts',(57.4515737214946,28.9630497382556,9.47068167462133));
#54593=CARTESIAN_POINT('Ctrl Pts',(57.4514417436959,29.0444777196845,9.47491301489758));
#54594=CARTESIAN_POINT('Ctrl Pts',(57.447280186925,29.1255784085121,9.47914435517382));
#54595=CARTESIAN_POINT('Ctrl Pts',(57.4431305905438,29.2064460124878,9.4833635345013));
#54596=CARTESIAN_POINT('Ctrl Pts',(57.4349746750456,29.2869877580856,9.48758271382878));
#54597=CARTESIAN_POINT('Ctrl Pts',(57.4228948822493,29.3667841866411,9.49180189315626));
#54598=CARTESIAN_POINT('Ctrl Pts',(57.4107766245956,29.4468347055032,9.49603450732774));
#54599=CARTESIAN_POINT('Ctrl Pts',(57.3946643624912,29.5264328793633,9.50026712149921));
#54600=CARTESIAN_POINT('Ctrl Pts',(57.3746040181182,29.6051495741856,9.50449973567069));
#54601=CARTESIAN_POINT('Ctrl Pts',(57.3545722879428,29.6837539870339,9.50872631241547));
#54602=CARTESIAN_POINT('Ctrl Pts',(57.3306037742864,29.7614789716775,9.51295288916026));
#54603=CARTESIAN_POINT('Ctrl Pts',(57.3027958364625,29.8379030884125,9.51717946590504));
#54604=CARTESIAN_POINT('Ctrl Pts',(57.2750187622294,29.9142423832277,9.52140135163907));
#54605=CARTESIAN_POINT('Ctrl Pts',(57.2434108890987,29.9892832446398,9.5256232373731));
#54606=CARTESIAN_POINT('Ctrl Pts',(57.2081196791139,30.0626183382145,9.52984512310713));
#54607=CARTESIAN_POINT('Ctrl Pts',(57.1728522719559,30.1359039695427,9.53406416131015));
#54608=CARTESIAN_POINT('Ctrl Pts',(57.1339066628975,30.2074857004826,9.53828319951317));
#54609=CARTESIAN_POINT('Ctrl Pts',(57.0914783412486,30.2769763498547,9.54250223771619));
#54610=CARTESIAN_POINT('Ctrl Pts',(57.0490638751426,30.3464443061142,9.54671989813515));
#54611=CARTESIAN_POINT('Ctrl Pts',(57.0031691970025,30.4138221407622,9.55093755855411));
#54612=CARTESIAN_POINT('Ctrl Pts',(56.9540349590479,30.4787486699296,9.55515521897308));
#54613=CARTESIAN_POINT('Ctrl Pts',(56.9049017435583,30.5436738480005,9.55937279162412));
#54614=CARTESIAN_POINT('Ctrl Pts',(56.8525293835573,30.6061474522904,9.56359036427516));
#54615=CARTESIAN_POINT('Ctrl Pts',(56.7972000740668,30.6658397713389,9.56780793692621));
#54616=CARTESIAN_POINT('Ctrl Pts',(56.7417768399817,30.7256334214345,9.5720326691425));
#54617=CARTESIAN_POINT('Ctrl Pts',(56.6833869308462,30.7826359974014,9.57625740135879));
#54618=CARTESIAN_POINT('Ctrl Pts',(56.6223511671111,30.8365530051086,9.58048213357508));
#54619=CARTESIAN_POINT('Ctrl Pts',(56.5613306476981,30.8904565464776,9.58470581062019));
#54620=CARTESIAN_POINT('Ctrl Pts',(56.4976659727563,30.9412757864979,9.58892948766529));
#54621=CARTESIAN_POINT('Ctrl Pts',(56.4317095815444,30.9887578847396,9.5931531647104));
#54622=CARTESIAN_POINT('Ctrl Pts',(56.3656335223123,31.0363261321564,9.59738450498664));
#54623=CARTESIAN_POINT('Ctrl Pts',(56.2972578284529,31.0805448845917,9.60161584526288));
#54624=CARTESIAN_POINT('Ctrl Pts',(56.2269629698428,31.1212053461734,9.60584718553912));
#54625=CARTESIAN_POINT('Ctrl Pts',(56.1568701399315,31.1617489488509,9.61006636486664));
#54626=CARTESIAN_POINT('Ctrl Pts',(56.0848696048905,31.1987545524203,9.61428554419417));
#54627=CARTESIAN_POINT('Ctrl Pts',(56.0113580986224,31.232062957524,9.6185047235217));
#54628=CARTESIAN_POINT('Ctrl Pts',(55.9376125146963,31.2654774243023,9.62273733769318));
#54629=CARTESIAN_POINT('Ctrl Pts',(55.8620720299263,31.2952953624052,9.62696995186467));
#54630=CARTESIAN_POINT('Ctrl Pts',(55.7851216128404,31.3213216716024,9.63120256603615));
#54631=CARTESIAN_POINT('Ctrl Pts',(55.7082809582991,31.3473108567133,9.63542914278094));
#54632=CARTESIAN_POINT('Ctrl Pts',(55.6300348022204,31.3695190071016,9.63965571952573));
#54633=CARTESIAN_POINT('Ctrl Pts',(55.5507896613485,31.3877983581014,9.64388229627053));
#54634=CARTESIAN_POINT('Ctrl Pts',(55.4716324734068,31.4060574211382,9.64810418200455));
#54635=CARTESIAN_POINT('Ctrl Pts',(55.3914789541511,31.4203962452269,9.65232606773858));
#54636=CARTESIAN_POINT('Ctrl Pts',(55.3107510644365,31.4307167720554,9.65654795347261));
#54637=CARTESIAN_POINT('Ctrl Pts',(55.23007762318,31.4410303380087,9.66076699167563));
#54638=CARTESIAN_POINT('Ctrl Pts',(55.148831040474,31.4473309306711,9.66498602987866));
#54639=CARTESIAN_POINT('Ctrl Pts',(55.0674425181974,31.4495717496614,9.66920506808168));
#54640=CARTESIAN_POINT('Ctrl Pts',(54.9860805744449,31.4518118368819,9.67342272850065));
#54641=CARTESIAN_POINT('Ctrl Pts',(54.9045772471911,31.4499947705608,9.67764038891962));
#54642=CARTESIAN_POINT('Ctrl Pts',(54.8233665178396,31.4441257870617,9.68185804933859));
#54643=CARTESIAN_POINT('Ctrl Pts',(54.7421574784526,31.4382569256938,9.68607562198964));
#54644=CARTESIAN_POINT('Ctrl Pts',(54.6612414881165,31.4283363494517,9.69029319464069));
#54645=CARTESIAN_POINT('Ctrl Pts',(54.5810487443192,31.4144212754537,9.69451076729174));
#54646=CARTESIAN_POINT('Ctrl Pts',(54.5007198688585,31.40048257984,9.69873549950803));
#54647=CARTESIAN_POINT('Ctrl Pts',(54.4211171564992,31.3825358993466,9.70296023172431));
#54648=CARTESIAN_POINT('Ctrl Pts',(54.3426622912597,31.3606900234186,9.70718496394059));
#54649=CARTESIAN_POINT('Ctrl Pts',(54.2642270209455,31.3388496037272,9.71140864098571));
#54650=CARTESIAN_POINT('Ctrl Pts',(54.1869394600097,31.3131121035319,9.71563231803082));
#54651=CARTESIAN_POINT('Ctrl Pts',(54.1112035656001,31.2836355112404,9.71985599507593));
#54652=CARTESIAN_POINT('Ctrl Pts',(54.0353302597224,31.2541054380749,9.72408733535218));
#54653=CARTESIAN_POINT('Ctrl Pts',(53.961014671789,31.2208229056018,9.72831867562842));
#54654=CARTESIAN_POINT('Ctrl Pts',(53.8886390731525,31.1839933929105,9.73255001590466));
#54655=CARTESIAN_POINT('Ctrl Pts',(53.8164714833,31.1472697289071,9.73676919523216));
#54656=CARTESIAN_POINT('Ctrl Pts',(53.7462331001432,31.1070197441476,9.74098837455966));
#54657=CARTESIAN_POINT('Ctrl Pts',(53.6782734463758,31.0634895607792,9.74520755388716));
#54658=CARTESIAN_POINT('Ctrl Pts',(53.6100973933339,31.019820767227,9.74944016805864));
#54659=CARTESIAN_POINT('Ctrl Pts',(53.5439610538095,30.9726884124556,9.75367278223012));
#54660=CARTESIAN_POINT('Ctrl Pts',(53.4802376599746,30.9223092050553,9.7579053964016));
#54661=CARTESIAN_POINT('Ctrl Pts',(53.4166051615776,30.872001858864,9.76213197314639));
#54662=CARTESIAN_POINT('Ctrl Pts',(53.3553791343214,30.8184571441745,9.76635854989118));
#54663=CARTESIAN_POINT('Ctrl Pts',(53.296904834979,30.7619356142839,9.77058512663597));
#54664=CARTESIAN_POINT('Ctrl Pts',(53.2384954353377,30.7054768167465,9.77480701237));
#54665=CARTESIAN_POINT('Ctrl Pts',(53.1828320274529,30.646048090124,9.77902889810402));
#54666=CARTESIAN_POINT('Ctrl Pts',(53.1302265809403,30.5839500028024,9.78325078383805));
#54667=CARTESIAN_POINT('Ctrl Pts',(53.07765661517,30.521893798715,9.78746982204107));
#54668=CARTESIAN_POINT('Ctrl Pts',(53.0281408139656,30.4571721632258,9.7916888602441));
#54669=CARTESIAN_POINT('Ctrl Pts',(52.9819531813185,30.3901213211836,9.79590789844712));
#54670=CARTESIAN_POINT('Ctrl Pts',(52.9357806318681,30.3230923755019,9.80012555886609));
#54671=CARTESIAN_POINT('Ctrl Pts',(52.8929343558679,30.2537361161135,9.80434321928506));
#54672=CARTESIAN_POINT('Ctrl Pts',(52.8536462207499,30.1824194282482,9.80856087970403));
#54673=CARTESIAN_POINT('Ctrl Pts',(52.8143589032031,30.1111042244562,9.81277845235508));
#54674=CARTESIAN_POINT('Ctrl Pts',(52.7786298024467,30.0378290807567,9.81699602500613));
#54675=CARTESIAN_POINT('Ctrl Pts',(52.7466451231777,29.9629860067006,9.82121359765718));
#54676=CARTESIAN_POINT('Ctrl Pts',(52.7146061481284,29.8880158823444,9.82543832987347));
#54677=CARTESIAN_POINT('Ctrl Pts',(52.6863244956853,29.8114729317168,9.82966306208975));
#54678=CARTESIAN_POINT('Ctrl Pts',(52.6619384756368,29.7337700990721,9.83388779430604));
#54679=CARTESIAN_POINT('Ctrl Pts',(52.6375585462525,29.6560866735248,9.83811147135115));
#54680=CARTESIAN_POINT('Ctrl Pts',(52.617072400219,29.5772444017894,9.84233514839625));
#54681=CARTESIAN_POINT('Ctrl Pts',(52.6005674274715,29.4976681423289,9.84655882544136));
#54682=CARTESIAN_POINT('Ctrl Pts',(52.5840325089161,29.4179475036315,9.8507901657176));
#54683=CARTESIAN_POINT('Ctrl Pts',(52.5714932707976,29.3374906761704,9.85502150599384));
#54684=CARTESIAN_POINT('Ctrl Pts',(52.5629854609046,29.2567301817819,9.85925284627008));
#54685=CARTESIAN_POINT('Ctrl Pts',(52.5545021026116,29.1762017945196,9.86347202559759));
#54686=CARTESIAN_POINT('Ctrl Pts',(52.5500269728094,29.0953719426398,9.8676912049251));
#54687=CARTESIAN_POINT('Ctrl Pts',(52.5495438984681,29.0146678036909,9.87191038425261));
#54688=CARTESIAN_POINT('Ctrl Pts',(52.5495148122119,29.0098085489954,9.87216442409772));
#54689=CARTESIAN_POINT('Ctrl Pts',(52.5495001797907,29.0049492076967,9.87241846394283));
#54690=CARTESIAN_POINT('Ctrl Pts',(52.5495000016467,29.0000898350446,9.87267250378794));
#54691=CARTESIAN_POINT('',(52.5495007823165,29.0019580941228,10.6726725037379));
#54692=CARTESIAN_POINT('Ctrl Pts',(52.5495000016466,29.0000898342118,9.87267250383148));
#54693=CARTESIAN_POINT('Ctrl Pts',(52.5494970367443,28.919213151244,9.87690060105406));
#54694=CARTESIAN_POINT('Ctrl Pts',(52.5535022747491,28.8381843604706,9.88112869827663));
#54695=CARTESIAN_POINT('Ctrl Pts',(52.5615349283419,28.7574338352052,9.88535679549921));
#54696=CARTESIAN_POINT('Ctrl Pts',(52.5695561224771,28.6767985093822,9.88957886087938));
#54697=CARTESIAN_POINT('Ctrl Pts',(52.5815932757421,28.5964411201722,9.89380092625955));
#54698=CARTESIAN_POINT('Ctrl Pts',(52.5976135911843,28.5167921847304,9.89802299163973));
#54699=CARTESIAN_POINT('Ctrl Pts',(52.6136155028604,28.4372347481349,9.9022402068093));
#54700=CARTESIAN_POINT('Ctrl Pts',(52.6335913916787,28.3583846020731,9.90645742197887));
#54701=CARTESIAN_POINT('Ctrl Pts',(52.6574568174838,28.2806658022539,9.91067463714844));
#54702=CARTESIAN_POINT('Ctrl Pts',(52.6813072384086,28.2029958664822,9.91488920083339));
#54703=CARTESIAN_POINT('Ctrl Pts',(52.7090422057637,28.1264563089838,9.91910376451835));
#54704=CARTESIAN_POINT('Ctrl Pts',(52.7405267611704,28.0514585233039,9.9233183282033));
#54705=CARTESIAN_POINT('Ctrl Pts',(52.77200120486,27.9764848242398,9.9275315383206));
#54706=CARTESIAN_POINT('Ctrl Pts',(52.8072226650356,27.9030523427262,9.9317447484379));
#54707=CARTESIAN_POINT('Ctrl Pts',(52.8460076353914,27.8315535342996,9.9359579585552));
#54708=CARTESIAN_POINT('Ctrl Pts',(52.8847920780597,27.7600556986472,9.94017111134983));
#54709=CARTESIAN_POINT('Ctrl Pts',(52.927139711311,27.6904918924786,9.94438426414447));
#54710=CARTESIAN_POINT('Ctrl Pts',(52.9728212478134,27.6232296645107,9.9485974169391));
#54711=CARTESIAN_POINT('Ctrl Pts',(53.0185477830497,27.5559011796845,9.95281471991247));
#54712=CARTESIAN_POINT('Ctrl Pts',(53.0676145196535,27.4908791881758,9.95703202288583));
#54713=CARTESIAN_POINT('Ctrl Pts',(53.1197493286007,27.4285014595289,9.9612493258592));
#54714=CARTESIAN_POINT('Ctrl Pts',(53.1719088452404,27.3660941688723,9.96546862749385));
#54715=CARTESIAN_POINT('Ctrl Pts',(53.2271390143538,27.3063339800033,9.96968792912851));
#54716=CARTESIAN_POINT('Ctrl Pts',(53.2851296666642,27.2495229250731,9.97390723076317));
#54717=CARTESIAN_POINT('Ctrl Pts',(53.3432245635654,27.1926097460083,9.97813411705768));
#54718=CARTESIAN_POINT('Ctrl Pts',(53.4040895099795,27.1386566038592,9.9823610033522));
#54719=CARTESIAN_POINT('Ctrl Pts',(53.4673801026197,27.0879261258639,9.98658788964671));
#54720=CARTESIAN_POINT('Ctrl Pts',(53.5273998501042,27.0398173888141,9.99059633130383));
#54721=CARTESIAN_POINT('Ctrl Pts',(53.5896004643821,26.9946066757912,9.99460477296094));
#54722=CARTESIAN_POINT('Ctrl Pts',(53.6536659988426,26.9524807675317,9.99861321461805));
#54723=CARTESIAN_POINT('Ctrl Pts',(53.7213144049457,26.9079989634947,10.0028458287895));
#54724=CARTESIAN_POINT('Ctrl Pts',(53.7912954463036,26.8667906133401,10.007078442961));
#54725=CARTESIAN_POINT('Ctrl Pts',(53.8632591990065,26.8291083395626,10.0113110571325));
#54726=CARTESIAN_POINT('Ctrl Pts',(53.9351203021732,26.7914798160104,10.0155376338773));
#54727=CARTESIAN_POINT('Ctrl Pts',(54.0089580914889,26.7573675930729,10.0197642106221));
#54728=CARTESIAN_POINT('Ctrl Pts',(54.0843939921836,26.7269808869148,10.0239907873669));
#54729=CARTESIAN_POINT('Ctrl Pts',(54.1597461677638,26.6966279064819,10.0282126731009));
#54730=CARTESIAN_POINT('Ctrl Pts',(54.2366925016168,26.6699923995052,10.0324345588349));
#54731=CARTESIAN_POINT('Ctrl Pts',(54.3148314290001,26.6472368841479,10.0366564445689));
#54732=CARTESIAN_POINT('Ctrl Pts',(54.3929176541002,26.6244967166801,10.040875482772));
#54733=CARTESIAN_POINT('Ctrl Pts',(54.4721944303176,26.6056314729265,10.045094520975));
#54734=CARTESIAN_POINT('Ctrl Pts',(54.5522430890643,26.5907544752124,10.049313559178));
#54735=CARTESIAN_POINT('Ctrl Pts',(54.6322656068374,26.5758823357833,10.053531219597));
#54736=CARTESIAN_POINT('Ctrl Pts',(54.7130590501692,26.5649959406935,10.057748880016));
#54737=CARTESIAN_POINT('Ctrl Pts',(54.7941939082545,26.5581576417384,10.0619665404349));
#54738=CARTESIAN_POINT('Ctrl Pts',(54.8753270779542,26.5513194850858,10.066184113086));
#54739=CARTESIAN_POINT('Ctrl Pts',(54.9568011852762,26.5485292949234,10.070401685737));
#54740=CARTESIAN_POINT('Ctrl Pts',(55.038182369416,26.5497974866012,10.0746192583881));
#54741=CARTESIAN_POINT('Ctrl Pts',(55.1197017026629,26.5510678311052,10.0788439906044));
#54742=CARTESIAN_POINT('Ctrl Pts',(55.2011273301845,26.5564103341134,10.0830687228207));
#54743=CARTESIAN_POINT('Ctrl Pts',(55.2820257766793,26.5657831420992,10.0872934550369));
#54744=CARTESIAN_POINT('Ctrl Pts',(55.3629040179388,26.5751536091279,10.0915171320821));
#54745=CARTESIAN_POINT('Ctrl Pts',(55.4432548851673,26.5885522705291,10.0957408091272));
#54746=CARTESIAN_POINT('Ctrl Pts',(55.5226547590382,26.6058859148205,10.0999644861723));
#54747=CARTESIAN_POINT('Ctrl Pts',(55.6021986921208,26.6232510084205,10.1041958264485));
#54748=CARTESIAN_POINT('Ctrl Pts',(55.6807877339682,26.6445652308838,10.1084271667248));
#54749=CARTESIAN_POINT('Ctrl Pts',(55.7580122977353,26.6696850842682,10.112658507001));
#54750=CARTESIAN_POINT('Ctrl Pts',(55.8350149167044,26.6947327427381,10.1168776863285));
#54751=CARTESIAN_POINT('Ctrl Pts',(55.9106604944123,26.7235639465777,10.121096865656));
#54752=CARTESIAN_POINT('Ctrl Pts',(55.984565470068,26.7559899543118,10.1253160449835));
#54753=CARTESIAN_POINT('Ctrl Pts',(56.0587057762799,26.7885192139631,10.129548659155));
#54754=CARTESIAN_POINT('Ctrl Pts',(56.1313701153078,26.8247872178455,10.1337812733265));
#54755=CARTESIAN_POINT('Ctrl Pts',(56.2021560821718,26.8646379688452,10.1380138874979));
#54756=CARTESIAN_POINT('Ctrl Pts',(56.2728410795005,26.9044318764905,10.1422404642427));
#54757=CARTESIAN_POINT('Ctrl Pts',(56.3416526246996,26.9477981552339,10.1464670409875));
#54758=CARTESIAN_POINT('Ctrl Pts',(56.4082091255623,26.9945331444566,10.1506936177323));
#54759=CARTESIAN_POINT('Ctrl Pts',(56.4746917564162,27.0412162632532,10.1549155034663));
#54760=CARTESIAN_POINT('Ctrl Pts',(56.5389239378018,27.0912603977723,10.1591373892003));
#54761=CARTESIAN_POINT('Ctrl Pts',(56.6005507332144,27.1444171803967,10.1633592749344));
#54762=CARTESIAN_POINT('Ctrl Pts',(56.6621359632645,27.1975381104196,10.1675783131374));
#54763=CARTESIAN_POINT('Ctrl Pts',(56.7211189465371,27.2537672163485,10.1717973513404));
#54764=CARTESIAN_POINT('Ctrl Pts',(56.7771767018898,27.312815001175,10.1760163895434));
#54765=CARTESIAN_POINT('Ctrl Pts',(56.8332161508234,27.3718435031478,10.1802340499624));
#54766=CARTESIAN_POINT('Ctrl Pts',(56.8863319493511,27.4336885193594,10.1844517103814));
#54767=CARTESIAN_POINT('Ctrl Pts',(56.936237969185,27.498023709679,10.1886693708003));
#54768=CARTESIAN_POINT('Ctrl Pts',(56.9861429504935,27.5623575612076,10.1928869434514));
#54769=CARTESIAN_POINT('Ctrl Pts',(57.0328380021068,27.6291811160359,10.1971045161025));
#54770=CARTESIAN_POINT('Ctrl Pts',(57.0760781931947,27.6981361109005,10.2013220887535));
#54771=CARTESIAN_POINT('Ctrl Pts',(57.1193917869232,27.7672081607219,10.2055468209698));
#54772=CARTESIAN_POINT('Ctrl Pts',(57.1592385378959,27.8384184941899,10.2097715531861));
#54773=CARTESIAN_POINT('Ctrl Pts',(57.1954175696032,27.9113807161924,10.2139962854024));
#54774=CARTESIAN_POINT('Ctrl Pts',(57.2315875652178,27.9843247151148,10.2182199624475));
#54775=CARTESIAN_POINT('Ctrl Pts',(57.2640915069243,28.0590192916598,10.2224436394926));
#54776=CARTESIAN_POINT('Ctrl Pts',(57.2927769641623,28.1350583588435,10.2266673165377));
#54777=CARTESIAN_POINT('Ctrl Pts',(57.321514466878,28.211235387557,10.2308986568139));
#54778=CARTESIAN_POINT('Ctrl Pts',(57.3464194971185,28.2887613383503,10.2351299970902));
#54779=CARTESIAN_POINT('Ctrl Pts',(57.3673894451691,28.3672145190494,10.2393613373664));
#54780=CARTESIAN_POINT('Ctrl Pts',(57.3882991252086,28.4454422238839,10.2435805166939));
#54781=CARTESIAN_POINT('Ctrl Pts',(57.405296297586,28.5245913734237,10.2477996960215));
#54782=CARTESIAN_POINT('Ctrl Pts',(57.4183304726086,28.6042374761897,10.252018875349));
#54783=CARTESIAN_POINT('Ctrl Pts',(57.4314061514626,28.6841371905896,10.2562514895205));
#54784=CARTESIAN_POINT('Ctrl Pts',(57.4405421596118,28.7648342018545,10.2604841036919));
#54785=CARTESIAN_POINT('Ctrl Pts',(57.445650281775,28.8459060375812,10.2647167178634));
#54786=CARTESIAN_POINT('Ctrl Pts',(57.4507511176815,28.9268622319465,10.2689432946082));
#54787=CARTESIAN_POINT('Ctrl Pts',(57.4518354497394,29.0081917291093,10.273169871353));
#54788=CARTESIAN_POINT('Ctrl Pts',(57.4488663745085,29.0894635668948,10.2773964480978));
#54789=CARTESIAN_POINT('Ctrl Pts',(57.4459005946073,29.1706452023514,10.2816183338318));
#54790=CARTESIAN_POINT('Ctrl Pts',(57.4388903634232,29.2517688436901,10.2858402195658));
#54791=CARTESIAN_POINT('Ctrl Pts',(57.4278507902601,29.3324015496857,10.2900621052999));
#54792=CARTESIAN_POINT('Ctrl Pts',(57.4168186629467,29.4129798714216,10.2942811435029));
#54793=CARTESIAN_POINT('Ctrl Pts',(57.4017626540284,29.4930674563818,10.2985001817059));
#54794=CARTESIAN_POINT('Ctrl Pts',(57.3827497697047,29.5722357774313,10.3027192199089));
#54795=CARTESIAN_POINT('Ctrl Pts',(57.3637430942958,29.6513782449936,10.3069368803279));
#54796=CARTESIAN_POINT('Ctrl Pts',(57.3407822180518,29.7296015934616,10.3111545407469));
#54797=CARTESIAN_POINT('Ctrl Pts',(57.3139851148365,29.8064881513791,10.3153722011658));
#54798=CARTESIAN_POINT('Ctrl Pts',(57.2871885692589,29.8833731093163,10.3195897738169));
#54799=CARTESIAN_POINT('Ctrl Pts',(57.2565561094307,29.9589208937306,10.3238073464679));
#54800=CARTESIAN_POINT('Ctrl Pts',(57.2222549150737,30.0327310116534,10.328024919119));
#54801=CARTESIAN_POINT('Ctrl Pts',(57.1878954925227,30.1066664263757,10.3322496513352));
#54802=CARTESIAN_POINT('Ctrl Pts',(57.1498550717141,30.1788578492762,10.3364743835515));
#54803=CARTESIAN_POINT('Ctrl Pts',(57.1083484132819,30.2489264262605,10.3406991157678));
#54804=CARTESIAN_POINT('Ctrl Pts',(57.0668521215728,30.318977502883,10.3449227928129));
#54805=CARTESIAN_POINT('Ctrl Pts',(57.0218915984879,30.3869064168714,10.349146469858));
#54806=CARTESIAN_POINT('Ctrl Pts',(56.973724496714,30.4523642315449,10.3533701469032));
#54807=CARTESIAN_POINT('Ctrl Pts',(56.9254700029283,30.5179408096461,10.3576014871794));
#54808=CARTESIAN_POINT('Ctrl Pts',(56.873997598167,30.5810369674196,10.3618328274556));
#54809=CARTESIAN_POINT('Ctrl Pts',(56.8196051476521,30.6413370636886,10.3660641677319));
#54810=CARTESIAN_POINT('Ctrl Pts',(56.765369022027,30.7014638563867,10.3702833470594));
#54811=CARTESIAN_POINT('Ctrl Pts',(56.7082299930118,30.7588103741959,10.3745025263869));
#54812=CARTESIAN_POINT('Ctrl Pts',(56.6485166481383,30.8131031715848,10.3787217057144));
#54813=CARTESIAN_POINT('Ctrl Pts',(56.5886131621475,30.8675688498126,10.3829543198859));
#54814=CARTESIAN_POINT('Ctrl Pts',(56.5258961235245,30.9191638819218,10.3871869340573));
#54815=CARTESIAN_POINT('Ctrl Pts',(56.4606718883087,30.9675842763919,10.3914195482288));
#54816=CARTESIAN_POINT('Ctrl Pts',(56.3955406893402,31.0159356037158,10.3956461249736));
#54817=CARTESIAN_POINT('Ctrl Pts',(56.3279097666342,31.0611210126294,10.3998727017184));
#54818=CARTESIAN_POINT('Ctrl Pts',(56.2581205318722,31.1028749314407,10.4040992784632));
#54819=CARTESIAN_POINT('Ctrl Pts',(56.1884087550794,31.1445825082371,10.4083211641972));
#54820=CARTESIAN_POINT('Ctrl Pts',(56.1165438226765,31.1828659252219,10.4125430499313));
#54821=CARTESIAN_POINT('Ctrl Pts',(56.0428971222023,31.2175021629081,10.4167649356653));
#54822=CARTESIAN_POINT('Ctrl Pts',(55.9693000941437,31.2521150395261,10.4209839738683));
#54823=CARTESIAN_POINT('Ctrl Pts',(55.8939241040826,31.2830854252455,10.4252030120713));
#54824=CARTESIAN_POINT('Ctrl Pts',(55.8171650896194,31.3102362360389,10.4294220502744));
#54825=CARTESIAN_POINT('Ctrl Pts',(55.7404311418517,31.3373781803675,10.4336397106933));
#54826=CARTESIAN_POINT('Ctrl Pts',(55.6623155042445,31.3607028721054,10.4378573711123));
#54827=CARTESIAN_POINT('Ctrl Pts',(55.5832327552187,31.3800818900282,10.4420750315313));
#54828=CARTESIAN_POINT('Ctrl Pts',(55.5041516518751,31.3994605046809,10.4462926041823));
#54829=CARTESIAN_POINT('Ctrl Pts',(55.4241039286052,31.414893499346,10.4505101768334));
#54830=CARTESIAN_POINT('Ctrl Pts',(55.3435165417897,31.4263030798968,10.4547277494844));
#54831=CARTESIAN_POINT('Ctrl Pts',(55.2627923533821,31.4377320288482,10.4589524817007));
#54832=CARTESIAN_POINT('Ctrl Pts',(55.1815271308917,31.4451238330451,10.463177213917));
#54833=CARTESIAN_POINT('Ctrl Pts',(55.1001555825528,31.4484523906508,10.4674019461333));
#54834=CARTESIAN_POINT('Ctrl Pts',(55.0188043576112,31.4517801169143,10.4716256231784));
#54835=CARTESIAN_POINT('Ctrl Pts',(54.9373473258697,31.4510466514572,10.4758493002235));
#54836=CARTESIAN_POINT('Ctrl Pts',(54.8562174505492,31.4462781584426,10.4800729772686));
#54837=CARTESIAN_POINT('Ctrl Pts',(54.7749403771879,31.4415010137097,10.4843043175449));
#54838=CARTESIAN_POINT('Ctrl Pts',(54.6939921096424,31.4326742612446,10.4885356578211));
#54839=CARTESIAN_POINT('Ctrl Pts',(54.6137995737617,31.4198759225988,10.4927669980974));
#54840=CARTESIAN_POINT('Ctrl Pts',(54.5338375126845,31.4071143666105,10.4969861774249));
#54841=CARTESIAN_POINT('Ctrl Pts',(54.4546272733771,31.3904041981347,10.5012053567524));
#54842=CARTESIAN_POINT('Ctrl Pts',(54.3765771121669,31.3698721807148,10.5054245360799));
#54843=CARTESIAN_POINT('Ctrl Pts',(54.2982784211698,31.3492747845969,10.5096571502514));
#54844=CARTESIAN_POINT('Ctrl Pts',(54.2208560002347,31.324754527491,10.5138897644229));
#54845=CARTESIAN_POINT('Ctrl Pts',(54.1447316255925,31.2964028953427,10.5181223785943));
#54846=CARTESIAN_POINT('Ctrl Pts',(54.0687158352229,31.2680917041356,10.5223489553391));
#54847=CARTESIAN_POINT('Ctrl Pts',(53.9939948454657,31.2359601530607,10.5265755320839));
#54848=CARTESIAN_POINT('Ctrl Pts',(53.9209772893505,31.2001500494063,10.5308021088287));
#54849=CARTESIAN_POINT('Ctrl Pts',(53.8480407742675,31.1643796908203,10.5350239945627));
#54850=CARTESIAN_POINT('Ctrl Pts',(53.7768043511669,31.1249390956278,10.5392458802968));
#54851=CARTESIAN_POINT('Ctrl Pts',(53.7076572780962,31.082018381077,10.5434677660308));
#54852=CARTESIAN_POINT('Ctrl Pts',(53.6385568425821,31.0391266152171,10.5476868042338));
#54853=CARTESIAN_POINT('Ctrl Pts',(53.571543351976,30.9927596361689,10.5519058424368));
#54854=CARTESIAN_POINT('Ctrl Pts',(53.506980897576,30.9431531616929,10.5561248806398));
#54855=CARTESIAN_POINT('Ctrl Pts',(53.4424395269197,30.8935628868827,10.5603425410588));
#54856=CARTESIAN_POINT('Ctrl Pts',(53.3803479709731,30.8407355003906,10.5645602014778));
#54857=CARTESIAN_POINT('Ctrl Pts',(53.3210396495258,30.7849488484367,10.5687778618967));
#54858=CARTESIAN_POINT('Ctrl Pts',(53.2617325622622,30.7291633573819,10.5729954345478));
#54859=CARTESIAN_POINT('Ctrl Pts',(53.2052089319147,30.6704190424451,10.5772130071988));
#54860=CARTESIAN_POINT('Ctrl Pts',(53.1517664495573,30.6090316942242,10.5814305798499));
#54861=CARTESIAN_POINT('Ctrl Pts',(53.0982332456,30.5475401375497,10.5856553120662));
#54862=CARTESIAN_POINT('Ctrl Pts',(53.0477919611186,30.4833969229783,10.5898800442825));
#54863=CARTESIAN_POINT('Ctrl Pts',(53.0007011465053,30.4169524848825,10.5941047764987));
#54864=CARTESIAN_POINT('Ctrl Pts',(52.9536220933168,30.3505246419819,10.5983284535438));
#54865=CARTESIAN_POINT('Ctrl Pts',(52.9098920688897,30.281797129621,10.602552130589));
#54866=CARTESIAN_POINT('Ctrl Pts',(52.8697248315904,30.211147372064,10.6067758076341));
#54867=CARTESIAN_POINT('Ctrl Pts',(52.8294847168386,30.1403694310744,10.6110071479103));
#54868=CARTESIAN_POINT('Ctrl Pts',(52.792820517365,30.0676626909834,10.6152384881866));
#54869=CARTESIAN_POINT('Ctrl Pts',(52.7598992055001,29.9934277429592,10.6194698284628));
#54870=CARTESIAN_POINT('Ctrl Pts',(52.727072510083,29.9194061475227,10.6236890077903));
#54871=CARTESIAN_POINT('Ctrl Pts',(52.6979673028113,29.8438655713314,10.6279081871178));
#54872=CARTESIAN_POINT('Ctrl Pts',(52.6726995063008,29.7672174802671,10.6321273664453));
#54873=CARTESIAN_POINT('Ctrl Pts',(52.6425523782678,29.6757682787574,10.6371612893411));
#54874=CARTESIAN_POINT('Ctrl Pts',(52.6177750447214,29.5824668337994,10.6421952122369));
#54875=CARTESIAN_POINT('Ctrl Pts',(52.5985610187568,29.4878945268862,10.6472291351327));
#54876=CARTESIAN_POINT('Ctrl Pts',(52.579555670576,29.3943493414858,10.6522083860989));
#54877=CARTESIAN_POINT('Ctrl Pts',(52.5659935010598,29.299560826227,10.6571876370652));
#54878=CARTESIAN_POINT('Ctrl Pts',(52.5580154729119,29.2041122717089,10.6621668880314));
#54879=CARTESIAN_POINT('Ctrl Pts',(52.5524045822788,29.1369839800369,10.6656687599336));
#54880=CARTESIAN_POINT('Ctrl Pts',(52.5495547759945,29.069529649616,10.6691706318358));
#54881=CARTESIAN_POINT('Ctrl Pts',(52.5495007823165,29.0019580941228,10.6726725037379));
#54882=CARTESIAN_POINT('',(52.5495005206114,28.9984026534493,11.4726725038167));
#54883=CARTESIAN_POINT('Ctrl Pts',(52.5495007823157,29.0019580931583,10.6726725037879));
#54884=CARTESIAN_POINT('Ctrl Pts',(52.5494359301699,28.9207974333899,10.6768786262003));
#54885=CARTESIAN_POINT('Ctrl Pts',(52.5534074481705,28.8395800658034,10.6810847486127));
#54886=CARTESIAN_POINT('Ctrl Pts',(52.5614055553208,28.7587379342298,10.6852908710251));
#54887=CARTESIAN_POINT('Ctrl Pts',(52.5694016866372,28.6779157737097,10.6894959543667));
#54888=CARTESIAN_POINT('Ctrl Pts',(52.5814223857094,28.5974691297911,10.6937010377083));
#54889=CARTESIAN_POINT('Ctrl Pts',(52.5974059177831,28.5178258342709,10.6979061210499));
#54890=CARTESIAN_POINT('Ctrl Pts',(52.6133904537395,28.4381775365697,10.7021114685015));
#54891=CARTESIAN_POINT('Ctrl Pts',(52.6333382235249,28.3593331452004,10.7063168159531));
#54892=CARTESIAN_POINT('Ctrl Pts',(52.6571364729459,28.2817098472068,10.7105221634047));
#54893=CARTESIAN_POINT('Ctrl Pts',(52.6809602811628,28.2040031835,10.7147320273069));
#54894=CARTESIAN_POINT('Ctrl Pts',(52.7086426895977,28.1275206795818,10.7189418912091));
#54895=CARTESIAN_POINT('Ctrl Pts',(52.7400213417708,28.0526633574339,10.7231517551112));
#54896=CARTESIAN_POINT('Ctrl Pts',(52.7714170884756,27.9777652543479,10.7273639124724));
#54897=CARTESIAN_POINT('Ctrl Pts',(52.8065128859592,27.9044945172938,10.7315760698336));
#54898=CARTESIAN_POINT('Ctrl Pts',(52.8450996785005,27.8332288765995,10.7357882271948));
#54899=CARTESIAN_POINT('Ctrl Pts',(52.8837567074427,27.761833516854,10.7400080516035));
#54900=CARTESIAN_POINT('Ctrl Pts',(52.9259171810606,27.6924509433078,10.7442278760122));
#54901=CARTESIAN_POINT('Ctrl Pts',(52.9713279963715,27.6254309214543,10.7484477004209));
#54902=CARTESIAN_POINT('Ctrl Pts',(53.0085710646733,27.5704653535739,10.7519085325509));
#54903=CARTESIAN_POINT('Ctrl Pts',(53.0479995146969,27.5170884186818,10.7553693646809));
#54904=CARTESIAN_POINT('Ctrl Pts',(53.089454357452,27.4654754489612,10.7588301968108));
#54905=CARTESIAN_POINT('Ctrl Pts',(53.1401538275023,27.4023525412707,10.7630628109823));
#54906=CARTESIAN_POINT('Ctrl Pts',(53.1940792366103,27.3416275503319,10.7672954251538));
#54907=CARTESIAN_POINT('Ctrl Pts',(53.2509752586573,27.2836484322345,10.7715280393253));
#54908=CARTESIAN_POINT('Ctrl Pts',(53.307790123871,27.2257520159052,10.7757546160701));
#54909=CARTESIAN_POINT('Ctrl Pts',(53.367566863529,27.1705940221001,10.7799811928148));
#54910=CARTESIAN_POINT('Ctrl Pts',(53.4300095449539,27.1184899093909,10.7842077695596));
#54911=CARTESIAN_POINT('Ctrl Pts',(53.4923829222331,27.0664436262132,10.7884296552936));
#54912=CARTESIAN_POINT('Ctrl Pts',(53.557416007092,27.0174447854202,10.7926515410277));
#54913=CARTESIAN_POINT('Ctrl Pts',(53.6247766352463,26.9717714756381,10.7968734267617));
#54914=CARTESIAN_POINT('Ctrl Pts',(53.6920918307458,26.9261289710869,10.8010924649647));
#54915=CARTESIAN_POINT('Ctrl Pts',(53.761731068165,26.8838078028496,10.8053115031677));
#54916=CARTESIAN_POINT('Ctrl Pts',(53.8333307849193,26.8450445033405,10.8095305413708));
#54917=CARTESIAN_POINT('Ctrl Pts',(53.9049071198164,26.8062938625119,10.8137482017897));
#54918=CARTESIAN_POINT('Ctrl Pts',(53.9784422544006,26.7710990040078,10.8179658622087));
#54919=CARTESIAN_POINT('Ctrl Pts',(54.0535466407057,26.7396512904685,10.8221835226276));
#54920=CARTESIAN_POINT('Ctrl Pts',(54.1286494641169,26.7082042313443,10.8264010952787));
#54921=CARTESIAN_POINT('Ctrl Pts',(54.2053210453675,26.6805043404856,10.8306186679297));
#54922=CARTESIAN_POINT('Ctrl Pts',(54.2831517320666,26.6566948959299,10.8348362405808));
#54923=CARTESIAN_POINT('Ctrl Pts',(54.3611145407053,26.6328450335118,10.839060972797));
#54924=CARTESIAN_POINT('Ctrl Pts',(54.4402399450273,26.6128989675693,10.8432857050133));
#54925=CARTESIAN_POINT('Ctrl Pts',(54.5201025922473,26.5969501195289,10.8475104372296));
#54926=CARTESIAN_POINT('Ctrl Pts',(54.5999452929337,26.5810052548805,10.8517341142747));
#54927=CARTESIAN_POINT('Ctrl Pts',(54.6805244040679,26.5690556590496,10.8559577913198));
#54928=CARTESIAN_POINT('Ctrl Pts',(54.7614081644119,26.5611428524838,10.8601814683649));
#54929=CARTESIAN_POINT('Ctrl Pts',(54.8424386762579,26.5532156893125,10.8644128086412));
#54930=CARTESIAN_POINT('Ctrl Pts',(54.9237744765769,26.5493399746473,10.8686441489174));
#54931=CARTESIAN_POINT('Ctrl Pts',(55.0049816993385,26.5495050637327,10.8728754891936));
#54932=CARTESIAN_POINT('Ctrl Pts',(55.0859555310684,26.5496696783491,10.8770946685211));
#54933=CARTESIAN_POINT('Ctrl Pts',(55.166801072977,26.5538517944617,10.8813138478487));
#54934=CARTESIAN_POINT('Ctrl Pts',(55.247095317281,26.5619897140952,10.8855330271762));
#54935=CARTESIAN_POINT('Ctrl Pts',(55.3276452370517,26.5701535467491,10.8897656413476));
#54936=CARTESIAN_POINT('Ctrl Pts',(55.4079399275819,26.5823288062798,10.8939982555191));
#54937=CARTESIAN_POINT('Ctrl Pts',(55.4875485147805,26.5984907462732,10.8982308696906));
#54938=CARTESIAN_POINT('Ctrl Pts',(55.5670435478046,26.6146296327769,10.9024574464354));
#54939=CARTESIAN_POINT('Ctrl Pts',(55.6458539697675,26.6347438137148,10.9066840231802));
#54940=CARTESIAN_POINT('Ctrl Pts',(55.7235540600729,26.6587567891926,10.910910599925));
#54941=CARTESIAN_POINT('Ctrl Pts',(55.8011679122755,26.6827431130481,10.915132485659));
#54942=CARTESIAN_POINT('Ctrl Pts',(55.8776734398775,26.7106194968103,10.919354371393));
#54943=CARTESIAN_POINT('Ctrl Pts',(55.9526565446198,26.74225870437,10.9235762571271));
#54944=CARTESIAN_POINT('Ctrl Pts',(56.0275890755831,26.7738765722654,10.9277952953301));
#54945=CARTESIAN_POINT('Ctrl Pts',(56.1010007961527,26.8092520433196,10.9320143335331));
#54946=CARTESIAN_POINT('Ctrl Pts',(56.1724953732078,26.8482089205022,10.9362333717361));
#54947=CARTESIAN_POINT('Ctrl Pts',(56.2439666027407,26.887153075789,10.9404510321551));
#54948=CARTESIAN_POINT('Ctrl Pts',(56.3135215244854,26.9296760924332,10.9446686925741));
#54949=CARTESIAN_POINT('Ctrl Pts',(56.380787548405,26.9755553857491,10.9488863529931));
#54950=CARTESIAN_POINT('Ctrl Pts',(56.4480521725441,27.0214337243342,10.9531039256441));
#54951=CARTESIAN_POINT('Ctrl Pts',(56.5130276104433,27.0706679379955,10.9573214982952));
#54952=CARTESIAN_POINT('Ctrl Pts',(56.5753706617782,27.1229924006525,10.9615390709462));
#54953=CARTESIAN_POINT('Ctrl Pts',(56.6378195439264,27.1754056870085,10.9657638031625));
#54954=CARTESIAN_POINT('Ctrl Pts',(56.6976267411355,27.2309194179019,10.9699885353788));
#54955=CARTESIAN_POINT('Ctrl Pts',(56.7544823267569,27.2892276553856,10.9742132675951));
#54956=CARTESIAN_POINT('Ctrl Pts',(56.8113237120996,27.3475213297754,10.9784369446402));
#54957=CARTESIAN_POINT('Ctrl Pts',(56.8652146676095,27.4086077513921,10.9826606216853));
#54958=CARTESIAN_POINT('Ctrl Pts',(56.9158853137214,27.4721473517821,10.9868842987304));
#54959=CARTESIAN_POINT('Ctrl Pts',(56.9666478941524,27.5358022352865,10.9911156390067));
#54960=CARTESIAN_POINT('Ctrl Pts',(57.0141782166597,27.601918814297,10.9953469792829));
#54961=CARTESIAN_POINT('Ctrl Pts',(57.058249013316,27.6701273560285,10.9995783195592));
#54962=CARTESIAN_POINT('Ctrl Pts',(57.1021931497031,27.7381398651735,11.0037974988867));
#54963=CARTESIAN_POINT('Ctrl Pts',(57.1426974634018,27.8082318926336,11.0080166782142));
#54964=CARTESIAN_POINT('Ctrl Pts',(57.1795834224522,27.8800150203813,11.0122358575417));
#54965=CARTESIAN_POINT('Ctrl Pts',(57.2165868349375,27.9520267222299,11.0164684717132));
#54966=CARTESIAN_POINT('Ctrl Pts',(57.2500864143564,28.0260081553786,11.0207010858847));
#54967=CARTESIAN_POINT('Ctrl Pts',(57.2798683504226,28.1015844198026,11.0249337000561));
#54968=CARTESIAN_POINT('Ctrl Pts',(57.3096078053533,28.1770528817816,11.0291602768009));
#54969=CARTESIAN_POINT('Ctrl Pts',(57.3356399802126,28.2541112282268,11.0333868535457));
#54970=CARTESIAN_POINT('Ctrl Pts',(57.3577972824058,28.3323607073578,11.0376134302905));
#54971=CARTESIAN_POINT('Ctrl Pts',(57.3799299925594,28.410523338628,11.0418353160245));
#54972=CARTESIAN_POINT('Ctrl Pts',(57.398196249521,28.4898740310127,11.0460572017586));
#54973=CARTESIAN_POINT('Ctrl Pts',(57.4124773467226,28.5699961610051,11.0502790874926));
#54974=CARTESIAN_POINT('Ctrl Pts',(57.426748811767,28.6500642511055,11.0544981256956));
#54975=CARTESIAN_POINT('Ctrl Pts',(57.4370403740825,28.7309022892708,11.0587171638986));
#54976=CARTESIAN_POINT('Ctrl Pts',(57.4432840681131,28.8120818994754,11.0629362021017));
#54977=CARTESIAN_POINT('Ctrl Pts',(57.4495257231808,28.8932349993791,11.0671538625206));
#54978=CARTESIAN_POINT('Ctrl Pts',(57.4517220995516,28.9747289869751,11.0713715229396));
#54979=CARTESIAN_POINT('Ctrl Pts',(57.4498570685586,29.0561301490586,11.0755891833586));
#54980=CARTESIAN_POINT('Ctrl Pts',(57.4479920763762,29.1375296172145,11.0798067560096));
#54981=CARTESIAN_POINT('Ctrl Pts',(57.4420658566851,29.2188357992994,11.0840243286607));
#54982=CARTESIAN_POINT('Ctrl Pts',(57.4321143848096,29.2996162031708,11.0882419013117));
#54983=CARTESIAN_POINT('Ctrl Pts',(57.4221460197545,29.3805337362913,11.092466633528));
#54984=CARTESIAN_POINT('Ctrl Pts',(57.4081387881945,29.4609232419479,11.0966913657443));
#54985=CARTESIAN_POINT('Ctrl Pts',(57.3901805942804,29.5403581929842,11.1009160979606));
#54986=CARTESIAN_POINT('Ctrl Pts',(57.3722268856136,29.6197733043086,11.1051397750057));
#54987=CARTESIAN_POINT('Ctrl Pts',(57.3503243337393,29.6982338944994,11.1093634520508));
#54988=CARTESIAN_POINT('Ctrl Pts',(57.32461085459,29.7753287204293,11.1135871290959));
#54989=CARTESIAN_POINT('Ctrl Pts',(57.2988507221733,29.8525634234056,11.1178184693721));
#54990=CARTESIAN_POINT('Ctrl Pts',(57.2692660136443,29.9284269759124,11.1220498096483));
#54991=CARTESIAN_POINT('Ctrl Pts',(57.2360431453476,30.0025274570525,11.1262811499246));
#54992=CARTESIAN_POINT('Ctrl Pts',(57.2029157601772,30.0764149720651,11.1305003292521));
#54993=CARTESIAN_POINT('Ctrl Pts',(57.1661713803383,30.1485491684762,11.1347195085796));
#54994=CARTESIAN_POINT('Ctrl Pts',(57.1260386277282,30.2185688340867,11.1389386879071));
#54995=CARTESIAN_POINT('Ctrl Pts',(57.0857780831406,30.2888114585264,11.1431713020786));
#54996=CARTESIAN_POINT('Ctrl Pts',(57.0419577887007,30.3571873027054,11.14740391625));
#54997=CARTESIAN_POINT('Ctrl Pts',(56.9947758215151,30.4233129212857,11.1516365304215));
#54998=CARTESIAN_POINT('Ctrl Pts',(56.9476611549754,30.4893442178802,11.1558631071663));
#54999=CARTESIAN_POINT('Ctrl Pts',(56.8971946069767,30.5531312888108,11.1600896839111));
#55000=CARTESIAN_POINT('Ctrl Pts',(56.8436194230284,30.6143164723908,11.1643162606559));
#55001=CARTESIAN_POINT('Ctrl Pts',(56.7901037013307,30.6754337475018,11.16853814639));
#55002=CARTESIAN_POINT('Ctrl Pts',(56.7334865037634,30.7339545255634,11.172760032124));
#55003=CARTESIAN_POINT('Ctrl Pts',(56.674052680683,30.7895524223387,11.176981917858));
#55004=CARTESIAN_POINT('Ctrl Pts',(56.6146589438731,30.8451128200567,11.181200956061));
#55005=CARTESIAN_POINT('Ctrl Pts',(56.5524526929481,30.8977539353105,11.1854199942641));
#55006=CARTESIAN_POINT('Ctrl Pts',(56.4877562600216,30.9471855486231,11.1896390324671));
#55007=CARTESIAN_POINT('Ctrl Pts',(56.4230809545914,30.9966010193729,11.1938566928861));
#55008=CARTESIAN_POINT('Ctrl Pts',(56.3559174509811,31.0428087878345,11.198074353305));
#55009=CARTESIAN_POINT('Ctrl Pts',(56.2866207783091,31.0855592110567,11.202292013724));
#55010=CARTESIAN_POINT('Ctrl Pts',(56.2173255476745,31.1283087446588,11.206509586375));
#55011=CARTESIAN_POINT('Ctrl Pts',(56.1458976322195,31.16760083316,11.2107271590261));
#55012=CARTESIAN_POINT('Ctrl Pts',(56.0727194022594,31.2032302044989,11.2149447316771));
#55013=CARTESIAN_POINT('Ctrl Pts',(55.999416948165,31.2389200586865,11.2191694638934));
#55014=CARTESIAN_POINT('Ctrl Pts',(55.9243586546465,31.2709345511826,11.2233941961097));
#55015=CARTESIAN_POINT('Ctrl Pts',(55.8479501585332,31.2991152164786,11.227618928326));
#55016=CARTESIAN_POINT('Ctrl Pts',(55.7715607462432,31.3272888433579,11.2318426053711));
#55017=CARTESIAN_POINT('Ctrl Pts',(55.6938222569342,31.3516304388611,11.2360662824162));
#55018=CARTESIAN_POINT('Ctrl Pts',(55.6151547332607,31.3720318092612,11.2402899594613));
#55019=CARTESIAN_POINT('Ctrl Pts',(55.5363444791156,31.3924701949007,11.2445212997376));
#55020=CARTESIAN_POINT('Ctrl Pts',(55.4566022782557,31.4089539741919,11.2487526400138));
#55021=CARTESIAN_POINT('Ctrl Pts',(55.376358369025,31.421426155815,11.2529839802901));
#55022=CARTESIAN_POINT('Ctrl Pts',(55.2963450822454,31.4338624921618,11.2572031596176));
#55023=CARTESIAN_POINT('Ctrl Pts',(55.2158334285267,31.442310294073,11.2614223389451));
#55024=CARTESIAN_POINT('Ctrl Pts',(55.135250863719,31.446764691151,11.2656415182726));
#55025=CARTESIAN_POINT('Ctrl Pts',(55.0544117053652,31.4512332720608,11.2698741324441));
#55026=CARTESIAN_POINT('Ctrl Pts',(54.9732005186985,31.4516995683122,11.2741067466156));
#55027=CARTESIAN_POINT('Ctrl Pts',(54.8920467806782,31.448120984028,11.2783393607871));
#55028=CARTESIAN_POINT('Ctrl Pts',(54.8110088008456,31.4445475042582,11.2825659375318));
#55029=CARTESIAN_POINT('Ctrl Pts',(54.7300285671472,31.4369406235007,11.2867925142766));
#55030=CARTESIAN_POINT('Ctrl Pts',(54.6495385182799,31.4253096709143,11.2910190910214));
#55031=CARTESIAN_POINT('Ctrl Pts',(54.5691378040462,31.4136916273384,11.2952409767554));
#55032=CARTESIAN_POINT('Ctrl Pts',(54.4892266510763,31.3980584524738,11.2994628624894));
#55033=CARTESIAN_POINT('Ctrl Pts',(54.4102339114659,31.3784714021437,11.3036847482234));
#55034=CARTESIAN_POINT('Ctrl Pts',(54.3312944500087,31.3588975626715,11.3079037864265));
#55035=CARTESIAN_POINT('Ctrl Pts',(54.2532726213765,31.33537525568,11.3121228246295));
#55036=CARTESIAN_POINT('Ctrl Pts',(54.1765873468506,31.3080168657602,11.3163418628325));
#55037=CARTESIAN_POINT('Ctrl Pts',(54.0999271149397,31.2806674100932,11.3205595232515));
#55038=CARTESIAN_POINT('Ctrl Pts',(54.0246030075348,31.2494845153099,11.3247771836704));
#55039=CARTESIAN_POINT('Ctrl Pts',(53.9510177095794,31.2146300829674,11.3289948440894));
#55040=CARTESIAN_POINT('Ctrl Pts',(53.8774339429061,31.1797763759323,11.3332124167404));
#55041=CARTESIAN_POINT('Ctrl Pts',(53.8055893330701,31.1412514831673,11.3374299893915));
#55042=CARTESIAN_POINT('Ctrl Pts',(53.7358642301629,31.0992643962632,11.3416475620425));
#55043=CARTESIAN_POINT('Ctrl Pts',(53.6660207649975,31.057206033933,11.3458722942588));
#55044=CARTESIAN_POINT('Ctrl Pts',(53.5983044055407,31.0116739593304,11.3500970264751));
#55045=CARTESIAN_POINT('Ctrl Pts',(53.5330689056756,30.9629221621105,11.3543217586914));
#55046=CARTESIAN_POINT('Ctrl Pts',(53.4678496990608,30.9141825411631,11.3585454357365));
#55047=CARTESIAN_POINT('Ctrl Pts',(53.4051104584196,30.8622251194076,11.3627691127816));
#55048=CARTESIAN_POINT('Ctrl Pts',(53.3451706109395,30.8073433384671,11.3669927898267));
#55049=CARTESIAN_POINT('Ctrl Pts',(53.285122011559,30.7523619827326,11.371224130103));
#55050=CARTESIAN_POINT('Ctrl Pts',(53.227883283205,30.6944459956986,11.3754554703792));
#55051=CARTESIAN_POINT('Ctrl Pts',(53.1737364537357,30.6339252460214,11.3796868106555));
#55052=CARTESIAN_POINT('Ctrl Pts',(53.1197452432368,30.573578434077,11.383905989983));
#55053=CARTESIAN_POINT('Ctrl Pts',(53.0688284046793,30.5106422180089,11.3881251693105));
#55054=CARTESIAN_POINT('Ctrl Pts',(53.0212227307852,30.4454725071196,11.392344348638));
#55055=CARTESIAN_POINT('Ctrl Pts',(52.9731764547246,30.3796996346016,11.3966025775031));
#55056=CARTESIAN_POINT('Ctrl Pts',(52.9283239109816,30.3114067320381,11.4008608063682));
#55057=CARTESIAN_POINT('Ctrl Pts',(52.8869376870544,30.2409342898031,11.4051190352333));
#55058=CARTESIAN_POINT('Ctrl Pts',(52.8456116405283,30.1705643176176,11.4093710724452));
#55059=CARTESIAN_POINT('Ctrl Pts',(52.8077421333248,30.0980214899934,11.4136231096571));
#55060=CARTESIAN_POINT('Ctrl Pts',(52.7735599568789,30.0236771875875,11.417875146869));
#55061=CARTESIAN_POINT('Ctrl Pts',(52.7394174626113,29.949419191677,11.4221222478798));
#55062=CARTESIAN_POINT('Ctrl Pts',(52.7089539847439,29.8733642885634,11.4263693488905));
#55063=CARTESIAN_POINT('Ctrl Pts',(52.6823549572621,29.7959093578243,11.4306164499013));
#55064=CARTESIAN_POINT('Ctrl Pts',(52.655780257259,29.7185252673887,11.4348596665121));
#55065=CARTESIAN_POINT('Ctrl Pts',(52.6330631283781,29.6397441259724,11.439102883123));
#55066=CARTESIAN_POINT('Ctrl Pts',(52.6143407820955,29.5599824515353,11.4433460997339));
#55067=CARTESIAN_POINT('Ctrl Pts',(52.5956282896561,29.4802627568275,11.4475870830781));
#55068=CARTESIAN_POINT('Ctrl Pts',(52.5809065043712,29.3995639991901,11.4518280664224));
#55069=CARTESIAN_POINT('Ctrl Pts',(52.5702623683183,29.3183163382389,11.4560690497666));
#55070=CARTESIAN_POINT('Ctrl Pts',(52.5596194925028,29.2370782967946,11.4603095309897));
#55071=CARTESIAN_POINT('Ctrl Pts',(52.5530533688563,29.1552919337269,11.4645500122128));
#55072=CARTESIAN_POINT('Ctrl Pts',(52.5505993707982,29.073394874928,11.4687904934359));
#55073=CARTESIAN_POINT('Ctrl Pts',(52.5498505213662,29.0484035894794,11.4700844968866));
#55074=CARTESIAN_POINT('Ctrl Pts',(52.5494842248953,29.023402023579,11.4713785003372));
#55075=CARTESIAN_POINT('Ctrl Pts',(52.549500520611,28.9984026540067,11.4726725037879));
#55076=CARTESIAN_POINT('',(52.5495001173786,28.9992415326165,12.2726725037456));
#55077=CARTESIAN_POINT('Ctrl Pts',(52.5495005206114,28.9984026534493,11.4726725038167));
#55078=CARTESIAN_POINT('Ctrl Pts',(52.5495606642625,28.906135896561,11.477448364322));
#55079=CARTESIAN_POINT('Ctrl Pts',(52.5548359378858,28.8140684437107,11.4822242248273));
#55080=CARTESIAN_POINT('Ctrl Pts',(52.5652348152121,28.7227478675557,11.4870000853325));
#55081=CARTESIAN_POINT('Ctrl Pts',(52.5756840754274,28.6309848403263,11.4917990850327));
#55082=CARTESIAN_POINT('Ctrl Pts',(52.5913065778112,28.5399761496053,11.4965980847329));
#55083=CARTESIAN_POINT('Ctrl Pts',(52.6119599482221,28.4502591873394,11.5013970844331));
#55084=CARTESIAN_POINT('Ctrl Pts',(52.6327297929416,28.360036267889,11.5062231480052));
#55085=CARTESIAN_POINT('Ctrl Pts',(52.6585872906741,28.2711198859228,11.5110492115772));
#55086=CARTESIAN_POINT('Ctrl Pts',(52.6893395576657,28.1840351905681,11.5158752751493));
#55087=CARTESIAN_POINT('Ctrl Pts',(52.6960768106901,28.164956544193,11.516932576434));
#55088=CARTESIAN_POINT('Ctrl Pts',(52.7030488182106,28.1459657252688,11.5179898777187));
#55089=CARTESIAN_POINT('Ctrl Pts',(52.7102532547224,28.1270681054685,11.5190471790034));
#55090=CARTESIAN_POINT('Ctrl Pts',(52.7390942298718,28.0514166950975,11.5232797931749));
#55091=CARTESIAN_POINT('Ctrl Pts',(52.7717420592589,27.9770554585001,11.5275124073464));
#55092=CARTESIAN_POINT('Ctrl Pts',(52.8080607394415,27.9043939905138,11.5317450215179));
#55093=CARTESIAN_POINT('Ctrl Pts',(52.844327614437,27.831836167289,11.5359715982626));
#55094=CARTESIAN_POINT('Ctrl Pts',(52.8842547346398,27.7609737092658,11.5401981750074));
#55095=CARTESIAN_POINT('Ctrl Pts',(52.9276574665477,27.6921977695216,11.5444247517522));
#55096=CARTESIAN_POINT('Ctrl Pts',(52.971012026449,27.6234981631065,11.5486466374862));
#55097=CARTESIAN_POINT('Ctrl Pts',(53.0178342864838,27.556880864373,11.5528685232203));
#55098=CARTESIAN_POINT('Ctrl Pts',(53.0678936484504,27.4927126032831,11.5570904089543));
#55099=CARTESIAN_POINT('Ctrl Pts',(53.1179192469296,27.4285876216954,11.5613094471573));
#55100=CARTESIAN_POINT('Ctrl Pts',(53.1711773260632,27.3669087624622,11.5655284853603));
#55101=CARTESIAN_POINT('Ctrl Pts',(53.2273946353952,27.3080128631179,11.5697475235634));
#55102=CARTESIAN_POINT('Ctrl Pts',(53.2835935862037,27.2491361970271,11.5739651839823));
#55103=CARTESIAN_POINT('Ctrl Pts',(53.3427495275366,27.1930410217581,11.5781828444013));
#55104=CARTESIAN_POINT('Ctrl Pts',(53.4045505967253,27.1400291799089,11.5824005048203));
#55105=CARTESIAN_POINT('Ctrl Pts',(53.4663503798572,27.087018441216,11.5866180774713));
#55106=CARTESIAN_POINT('Ctrl Pts',(53.5307948280387,27.0370912099325,11.5908356501224));
#55107=CARTESIAN_POINT('Ctrl Pts',(53.5975381665936,26.990509752241,11.5950532227734));
#55108=CARTESIAN_POINT('Ctrl Pts',(53.664394805695,26.9438492199224,11.5992779549897));
#55109=CARTESIAN_POINT('Ctrl Pts',(53.7335577602002,26.9005460920931,11.603502687206));
#55110=CARTESIAN_POINT('Ctrl Pts',(53.8046509895121,26.8608200185291,11.6077274194223));
#55111=CARTESIAN_POINT('Ctrl Pts',(53.8757264625446,26.8211038669686,11.6119510964674));
#55112=CARTESIAN_POINT('Ctrl Pts',(53.9487308190989,26.7849631708519,11.6161747735125));
#55113=CARTESIAN_POINT('Ctrl Pts',(54.0232659662694,26.7525701618622,11.6203984505577));
#55114=CARTESIAN_POINT('Ctrl Pts',(54.0979363463315,26.720118380596,11.6246297908339));
#55115=CARTESIAN_POINT('Ctrl Pts',(54.1741426315099,26.6914280394162,11.6288611311102));
#55116=CARTESIAN_POINT('Ctrl Pts',(54.2514686906535,26.6666223775548,11.6330924713864));
#55117=CARTESIAN_POINT('Ctrl Pts',(54.3285725132999,26.6418880076157,11.6373116507139));
#55118=CARTESIAN_POINT('Ctrl Pts',(54.4067892207011,26.621016054546,11.6415308300414));
#55119=CARTESIAN_POINT('Ctrl Pts',(54.4856973206717,26.6040778384856,11.6457500093689));
#55120=CARTESIAN_POINT('Ctrl Pts',(54.5648566823047,26.5870856872231,11.6499826235404));
#55121=CARTESIAN_POINT('Ctrl Pts',(54.6450062681451,26.5739891929746,11.6542152377119));
#55122=CARTESIAN_POINT('Ctrl Pts',(54.7257284593265,26.5648972563819,11.6584478518834));
#55123=CARTESIAN_POINT('Ctrl Pts',(54.8063355078815,26.555818288583,11.6626744286282));
#55124=CARTESIAN_POINT('Ctrl Pts',(54.8875130817777,26.5507325849851,11.666901005373));
#55125=CARTESIAN_POINT('Ctrl Pts',(54.9688325573186,26.5496982143996,11.6711275821177));
#55126=CARTESIAN_POINT('Ctrl Pts',(55.0500617776582,26.5486649918456,11.6753494678518));
#55127=CARTESIAN_POINT('Ctrl Pts',(55.1314321245319,26.5516741736254,11.6795713535858));
#55128=CARTESIAN_POINT('Ctrl Pts',(55.2125104377487,26.558731976237,11.6837932393198));
#55129=CARTESIAN_POINT('Ctrl Pts',(55.2935340661576,26.5657850185795,11.6880122775228));
#55130=CARTESIAN_POINT('Ctrl Pts',(55.3742655905007,26.5768812182241,11.6922313157259));
#55131=CARTESIAN_POINT('Ctrl Pts',(55.454273705188,26.5919747404201,11.6964503539289));
#55132=CARTESIAN_POINT('Ctrl Pts',(55.5342556921421,26.6070633336221,11.7006680143479));
#55133=CARTESIAN_POINT('Ctrl Pts',(55.6135142824507,26.6261465709193,11.7048856747668));
#55134=CARTESIAN_POINT('Ctrl Pts',(55.6916265046396,26.6491271773914,11.7091033351858));
#55135=CARTESIAN_POINT('Ctrl Pts',(55.7697371013428,26.6721073056457,11.7133209078369));
#55136=CARTESIAN_POINT('Ctrl Pts',(55.8467009320274,26.6989845095815,11.7175384804879));
#55137=CARTESIAN_POINT('Ctrl Pts',(55.9221097611905,26.7296115225986,11.7217560531389));
#55138=CARTESIAN_POINT('Ctrl Pts',(55.9976466010547,26.7602905266816,11.7259807853552));
#55139=CARTESIAN_POINT('Ctrl Pts',(56.0716227253,26.7947319000186,11.7302055175715));
#55140=CARTESIAN_POINT('Ctrl Pts',(56.1436491693487,26.8327397877855,11.7344302497878));
#55141=CARTESIAN_POINT('Ctrl Pts',(56.2156576240378,26.8707381826839,11.7386539268329));
#55142=CARTESIAN_POINT('Ctrl Pts',(56.2857169822456,26.9123010545674,11.742877603878));
#55143=CARTESIAN_POINT('Ctrl Pts',(56.3534660495926,26.9571882361313,11.7471012809231));
#55144=CARTESIAN_POINT('Ctrl Pts',(56.4213380375029,27.0021568587816,11.7513326211994));
#55145=CARTESIAN_POINT('Ctrl Pts',(56.486890982561,27.0504615684061,11.7555639614756));
#55146=CARTESIAN_POINT('Ctrl Pts',(56.5497949664561,27.1018203952346,11.7597953017519));
#55147=CARTESIAN_POINT('Ctrl Pts',(56.6125181631599,27.1530316158628,11.7640144810794));
#55148=CARTESIAN_POINT('Ctrl Pts',(56.6726073225128,27.2072790551564,11.7682336604069));
#55149=CARTESIAN_POINT('Ctrl Pts',(56.7297731586964,27.2642479815788,11.7724528397344));
#55150=CARTESIAN_POINT('Ctrl Pts',(56.7871210241398,27.3213983102546,11.7766854539058));
#55151=CARTESIAN_POINT('Ctrl Pts',(56.8417401930594,27.3815000627959,11.7809180680773));
#55152=CARTESIAN_POINT('Ctrl Pts',(56.893311964802,27.4442622155589,11.7851506822488));
#55153=CARTESIAN_POINT('Ctrl Pts',(56.9448101742546,27.5069348440041,11.7893772589936));
#55154=CARTESIAN_POINT('Ctrl Pts',(56.9932693274113,27.572259979749,11.7936038357384));
#55155=CARTESIAN_POINT('Ctrl Pts',(57.0384073716024,27.6399096951317,11.7978304124832));
#55156=CARTESIAN_POINT('Ctrl Pts',(57.0834953177914,27.7074843271639,11.8020522982172));
#55157=CARTESIAN_POINT('Ctrl Pts',(57.1252692226447,27.7773780278716,11.8062741839512));
#55158=CARTESIAN_POINT('Ctrl Pts',(57.1634880588499,27.8492308358259,11.8104960696852));
#55159=CARTESIAN_POINT('Ctrl Pts',(57.2016811176353,27.9210351812894,11.8147151078883));
#55160=CARTESIAN_POINT('Ctrl Pts',(57.2363236523884,27.9947956005885,11.8189341460913));
#55161=CARTESIAN_POINT('Ctrl Pts',(57.2672193073435,28.0701253512386,11.8231531842943));
#55162=CARTESIAN_POINT('Ctrl Pts',(57.298104872904,28.1454305019386,11.8273708447133));
#55163=CARTESIAN_POINT('Ctrl Pts',(57.3252458125059,28.222303536749,11.8315885051322));
#55164=CARTESIAN_POINT('Ctrl Pts',(57.3484934567948,28.3003366999819,11.8358061655512));
#55165=CARTESIAN_POINT('Ctrl Pts',(57.371740617309,28.3783682393742,11.8400237382023));
#55166=CARTESIAN_POINT('Ctrl Pts',(57.3910945120833,28.4575594136433,11.8442413108533));
#55167=CARTESIAN_POINT('Ctrl Pts',(57.4064564283203,28.5374876124947,11.8484588835043));
#55168=CARTESIAN_POINT('Ctrl Pts',(57.4218444222685,28.6175514939297,11.8526836157206));
#55169=CARTESIAN_POINT('Ctrl Pts',(57.4332267911302,28.6983544445862,11.8569083479369));
#55170=CARTESIAN_POINT('Ctrl Pts',(57.4405560702434,28.7794635676397,11.8611330801532));
#55171=CARTESIAN_POINT('Ctrl Pts',(57.4478835187922,28.860552432839,11.8653567571983));
#55172=CARTESIAN_POINT('Ctrl Pts',(57.4511599044275,28.941946850884,11.8695804342434));
#55173=CARTESIAN_POINT('Ctrl Pts',(57.4503900510317,29.0232130955424,11.8738041112885));
#55174=CARTESIAN_POINT('Ctrl Pts',(57.449618800852,29.1046267856634,11.8780354515648));
#55175=CARTESIAN_POINT('Ctrl Pts',(57.4447866679591,29.1859113725751,11.882266791841));
#55176=CARTESIAN_POINT('Ctrl Pts',(57.4359505679149,29.266636607905,11.8864981321173));
#55177=CARTESIAN_POINT('Ctrl Pts',(57.4271398629826,29.3471298374439,11.8907173114448));
#55178=CARTESIAN_POINT('Ctrl Pts',(57.4143483291803,29.4270664898922,11.8949364907723));
#55179=CARTESIAN_POINT('Ctrl Pts',(57.3976824838279,29.5060325649054,11.8991556700998));
#55180=CARTESIAN_POINT('Ctrl Pts',(57.3809635705649,29.5852500861869,11.9033882842713));
#55181=CARTESIAN_POINT('Ctrl Pts',(57.3602834239191,29.6637854655181,11.9076208984428));
#55182=CARTESIAN_POINT('Ctrl Pts',(57.3357126609721,29.7412129352451,11.9118535126142));
#55183=CARTESIAN_POINT('Ctrl Pts',(57.3111769459114,29.8185299619567,11.916080089359));
#55184=CARTESIAN_POINT('Ctrl Pts',(57.282761776114,29.8947417786923,11.9203066661038));
#55185=CARTESIAN_POINT('Ctrl Pts',(57.2505886758749,29.9694332684737,11.9245332428486));
#55186=CARTESIAN_POINT('Ctrl Pts',(57.2184512840515,30.0440418593505,11.9287551285826));
#55187=CARTESIAN_POINT('Ctrl Pts',(57.1825644321438,30.117133051607,11.9329770143167));
#55188=CARTESIAN_POINT('Ctrl Pts',(57.1430988494162,30.1883087021608,11.9371989000507));
#55189=CARTESIAN_POINT('Ctrl Pts',(57.1036598850002,30.2594363469456,11.9414179382537));
#55190=CARTESIAN_POINT('Ctrl Pts',(57.0606472083586,30.3286506107748,11.9456369764568));
#55191=CARTESIAN_POINT('Ctrl Pts',(57.0142783326064,30.395576242558,11.9498560146598));
#55192=CARTESIAN_POINT('Ctrl Pts',(56.9679245992385,30.46248001887,11.9540736750787));
#55193=CARTESIAN_POINT('Ctrl Pts',(56.918217107734,30.5270962658345,11.9582913354977));
#55194=CARTESIAN_POINT('Ctrl Pts',(56.8654169581344,30.5890782933212,11.9625089959167));
#55195=CARTESIAN_POINT('Ctrl Pts',(56.8126179072858,30.6510590309854,11.9667265685677));
#55196=CARTESIAN_POINT('Ctrl Pts',(56.7567266284403,30.7104053052919,11.9709441412188));
#55197=CARTESIAN_POINT('Ctrl Pts',(56.6980438784476,30.7668042440708,11.9751617138698));
#55198=CARTESIAN_POINT('Ctrl Pts',(56.6392615112077,30.8232989231997,11.9793864460861));
#55199=CARTESIAN_POINT('Ctrl Pts',(56.5776785285335,30.8768359328346,11.9836111783024));
#55200=CARTESIAN_POINT('Ctrl Pts',(56.5136322154018,30.9271397890391,11.9878359105187));
#55201=CARTESIAN_POINT('Ctrl Pts',(56.4496018985084,30.9774310813281,11.9920595875638));
#55202=CARTESIAN_POINT('Ctrl Pts',(56.3831098742635,31.0244905830628,11.9962832646089));
#55203=CARTESIAN_POINT('Ctrl Pts',(56.3145225892979,31.0680862197272,12.000506941654));
#55204=CARTESIAN_POINT('Ctrl Pts',(56.2458108629482,31.1117609541627,12.0047382819303));
#55205=CARTESIAN_POINT('Ctrl Pts',(56.1749966838042,31.1519590338415,12.0089696222065));
#55206=CARTESIAN_POINT('Ctrl Pts',(56.1024719399326,31.1884939734121,12.0132009624828));
#55207=CARTESIAN_POINT('Ctrl Pts',(56.030155633491,31.2249239109034,12.0174201418103));
#55208=CARTESIAN_POINT('Ctrl Pts',(55.9561390315075,31.2577116276957,12.0216393211378));
#55209=CARTESIAN_POINT('Ctrl Pts',(55.88082739603,31.2867210910828,12.0258585004653));
#55210=CARTESIAN_POINT('Ctrl Pts',(55.8052759508661,31.3158229273188,12.0300911146368));
#55211=CARTESIAN_POINT('Ctrl Pts',(55.7281402049313,31.341230622434,12.0343237288083));
#55212=CARTESIAN_POINT('Ctrl Pts',(55.6498157468709,31.3627716235639,12.0385563429798));
#55213=CARTESIAN_POINT('Ctrl Pts',(55.5716030112957,31.3842818984782,12.0427829197245));
#55214=CARTESIAN_POINT('Ctrl Pts',(55.4922053754433,31.4019363116889,12.0470094964693));
#55215=CARTESIAN_POINT('Ctrl Pts',(55.4120372078317,31.4156108108225,12.0512360732141));
#55216=CARTESIAN_POINT('Ctrl Pts',(55.3319580176029,31.4292701328455,12.0554579589482));
#55217=CARTESIAN_POINT('Ctrl Pts',(55.2511104505239,31.4389582401283,12.0596798446822));
#55218=CARTESIAN_POINT('Ctrl Pts',(55.1699214242054,31.4446015952699,12.0639017304162));
#55219=CARTESIAN_POINT('Ctrl Pts',(55.0887871573675,31.4502411441435,12.0681207686192));
#55220=CARTESIAN_POINT('Ctrl Pts',(55.0073123509276,31.4518413269117,12.0723398068223));
#55221=CARTESIAN_POINT('Ctrl Pts',(54.9259301892824,31.4493803120668,12.0765588450253));
#55222=CARTESIAN_POINT('Ctrl Pts',(54.8445746040842,31.4469201008996,12.0807765054443));
#55223=CARTESIAN_POINT('Ctrl Pts',(54.7633120675775,31.4404013399797,12.0849941658632));
#55224=CARTESIAN_POINT('Ctrl Pts',(54.6825755352627,31.4298543082223,12.0892118262822));
#55225=CARTESIAN_POINT('Ctrl Pts',(54.6018406830445,31.4193074959446,12.0934293989332));
#55226=CARTESIAN_POINT('Ctrl Pts',(54.5216322737369,31.4047326408381,12.0976469715843));
#55227=CARTESIAN_POINT('Ctrl Pts',(54.4423764846801,31.3862116974741,12.1018645442353));
#55228=CARTESIAN_POINT('Ctrl Pts',(54.3629861544929,31.3676593137739,12.1060892764516));
#55229=CARTESIAN_POINT('Ctrl Pts',(54.284552134791,31.345147545538,12.1103140086679));
#55230=CARTESIAN_POINT('Ctrl Pts',(54.2074891266635,31.3188093422365,12.1145387408842));
#55231=CARTESIAN_POINT('Ctrl Pts',(54.1304453658304,31.2924777171776,12.1187624179293));
#55232=CARTESIAN_POINT('Ctrl Pts',(54.0547723569769,31.2623217605063,12.1229860949744));
#55233=CARTESIAN_POINT('Ctrl Pts',(53.980864263903,31.2285225153473,12.1272097720195));
#55234=CARTESIAN_POINT('Ctrl Pts',(53.9068220756335,31.1946619465065,12.1314411122958));
#55235=CARTESIAN_POINT('Ctrl Pts',(53.8345516160845,31.1571450935697,12.135672452572));
#55236=CARTESIAN_POINT('Ctrl Pts',(53.764422658053,31.116199159358,12.1399037928482));
#55237=CARTESIAN_POINT('Ctrl Pts',(53.6944952519194,31.075370904504,12.1441229721757));
#55238=CARTESIAN_POINT('Ctrl Pts',(53.6266973901279,31.0311335709704,12.1483421515033));
#55239=CARTESIAN_POINT('Ctrl Pts',(53.5613638053301,30.9837530464717,12.1525613308308));
#55240=CARTESIAN_POINT('Ctrl Pts',(53.4963354145064,30.9365938514869,12.1567608010284));
#55241=CARTESIAN_POINT('Ctrl Pts',(53.4334980409898,30.8861391378274,12.1609602712261));
#55242=CARTESIAN_POINT('Ctrl Pts',(53.3732086710378,30.8326211343356,12.1651597414237));
#55243=CARTESIAN_POINT('Ctrl Pts',(53.3130055443728,30.7791796877648,12.169353204325));
#55244=CARTESIAN_POINT('Ctrl Pts',(53.2553435354469,30.7226839619698,12.1735466672263));
#55245=CARTESIAN_POINT('Ctrl Pts',(53.2005494727727,30.6634085637815,12.1777401301276));
#55246=CARTESIAN_POINT('Ctrl Pts',(53.145817827864,30.6042006881991,12.1819288161138));
#55247=CARTESIAN_POINT('Ctrl Pts',(53.0939479577934,30.5422197763119,12.1861175021));
#55248=CARTESIAN_POINT('Ctrl Pts',(53.0452313089151,30.4777786080311,12.1903061880862));
#55249=CARTESIAN_POINT('Ctrl Pts',(52.9965444562646,30.4133768534574,12.1944923121753));
#55250=CARTESIAN_POINT('Ctrl Pts',(52.9510072821594,30.3465182045079,12.1986784362644));
#55251=CARTESIAN_POINT('Ctrl Pts',(52.9088714062374,30.277549002719,12.2028645603535));
#55252=CARTESIAN_POINT('Ctrl Pts',(52.8667479021659,30.2086000515275,12.2070494553214));
#55253=CARTESIAN_POINT('Ctrl Pts',(52.8280239595776,30.1375421810614,12.2112343502892));
#55254=CARTESIAN_POINT('Ctrl Pts',(52.7929073850718,30.064749942066,12.215419245257));
#55255=CARTESIAN_POINT('Ctrl Pts',(52.7577899543323,29.9919559282056,12.2196042422635));
#55256=CARTESIAN_POINT('Ctrl Pts',(52.7262802696761,29.9174278885332,12.22378923927));
#55257=CARTESIAN_POINT('Ctrl Pts',(52.6985390761442,29.8415627522442,12.2279742362765));
#55258=CARTESIAN_POINT('Ctrl Pts',(52.6707711704879,29.7656245650623,12.2321632630361));
#55259=CARTESIAN_POINT('Ctrl Pts',(52.6467791619605,29.6883471559616,12.2363522897958));
#55260=CARTESIAN_POINT('Ctrl Pts',(52.6266744719774,29.6101443993322,12.2405413165554));
#55261=CARTESIAN_POINT('Ctrl Pts',(52.6065591563653,29.5319003113775,12.2447325572782));
#55262=CARTESIAN_POINT('Ctrl Pts',(52.5903353428762,29.4527303656458,12.248923798001));
#55263=CARTESIAN_POINT('Ctrl Pts',(52.5780631744243,29.3730579886831,12.2531150387239));
#55264=CARTESIAN_POINT('Ctrl Pts',(52.5657711586025,29.2932567602349,12.2573130578009));
#55265=CARTESIAN_POINT('Ctrl Pts',(52.5574435931298,29.2129519484643,12.261511076878));
#55266=CARTESIAN_POINT('Ctrl Pts',(52.5530886379128,29.1325708719454,12.2657090959551));
#55267=CARTESIAN_POINT('Ctrl Pts',(52.5506807300774,29.0881271947278,12.2680302318852));
#55268=CARTESIAN_POINT('Ctrl Pts',(52.5494863691203,29.0436601934439,12.2703513678154));
#55269=CARTESIAN_POINT('Ctrl Pts',(52.5495001173787,28.9992415326165,12.2726725037456));
#55270=CARTESIAN_POINT('',(52.5495009826471,29.0021945278826,13.0726725037477));
#55271=CARTESIAN_POINT('Ctrl Pts',(52.5495001173789,28.999241531807,12.2726725037879));
#55272=CARTESIAN_POINT('Ctrl Pts',(52.5495131316829,28.9571942176884,12.274869722924));
#55273=CARTESIAN_POINT('Ctrl Pts',(52.5506082944952,28.9151651062863,12.2770669420601));
#55274=CARTESIAN_POINT('Ctrl Pts',(52.5527831953695,28.8731924247765,12.2792641611962));
#55275=CARTESIAN_POINT('Ctrl Pts',(52.5569728167463,28.7923383289532,12.2834967753677));
#55276=CARTESIAN_POINT('Ctrl Pts',(52.565181565129,28.7115417280223,12.2877293895392));
#55277=CARTESIAN_POINT('Ctrl Pts',(52.5774059298484,28.631234191842,12.2919620037107));
#55278=CARTESIAN_POINT('Ctrl Pts',(52.5896128576594,28.5510412068216,12.2961885804556));
#55279=CARTESIAN_POINT('Ctrl Pts',(52.6058239561334,28.4713363564607,12.3004151572004));
#55280=CARTESIAN_POINT('Ctrl Pts',(52.6259837702042,28.3925486104503,12.3046417339452));
#55281=CARTESIAN_POINT('Ctrl Pts',(52.6461212092157,28.3138483097146,12.3088636196792));
#55282=CARTESIAN_POINT('Ctrl Pts',(52.6701985409968,28.2360635385855,12.3130855054132));
#55283=CARTESIAN_POINT('Ctrl Pts',(52.6981090637492,28.1596141555175,12.3173073911473));
#55284=CARTESIAN_POINT('Ctrl Pts',(52.7260007617196,28.0832163351875,12.3215264293503));
#55285=CARTESIAN_POINT('Ctrl Pts',(52.7577203569904,28.0081525493439,12.3257454675533));
#55286=CARTESIAN_POINT('Ctrl Pts',(52.7931113718505,27.9348273224756,12.3299645057563));
#55287=CARTESIAN_POINT('Ctrl Pts',(52.8284908292955,27.861526040953,12.3341821661753));
#55288=CARTESIAN_POINT('Ctrl Pts',(52.8675391235118,27.7899626089347,12.3383998265943));
#55289=CARTESIAN_POINT('Ctrl Pts',(52.9100522768151,27.7205201195976,12.3426174870132));
#55290=CARTESIAN_POINT('Ctrl Pts',(52.9525645454359,27.6510790753325,12.3468350596643));
#55291=CARTESIAN_POINT('Ctrl Pts',(52.9985412862296,27.5837592815786,12.3510526323153));
#55292=CARTESIAN_POINT('Ctrl Pts',(53.0477340858412,27.5189165957267,12.3552702049664));
#55293=CARTESIAN_POINT('Ctrl Pts',(53.0970103929788,27.4539638357925,12.3594949371826));
#55294=CARTESIAN_POINT('Ctrl Pts',(53.1495133997465,27.3914969690868,12.3637196693989));
#55295=CARTESIAN_POINT('Ctrl Pts',(53.2049527921878,27.3318406036215,12.3679444016152));
#55296=CARTESIAN_POINT('Ctrl Pts',(53.2603783380597,27.272199137959,12.3721680786603));
#55297=CARTESIAN_POINT('Ctrl Pts',(53.3187384542129,27.2153670798025,12.3763917557054));
#55298=CARTESIAN_POINT('Ctrl Pts',(53.3797072659948,27.1616306937588,12.3806154327505));
#55299=CARTESIAN_POINT('Ctrl Pts',(53.4407866965791,27.1077968110688,12.3848467730267));
#55300=CARTESIAN_POINT('Ctrl Pts',(53.5044839172587,27.0570701153811,12.3890781133029));
#55301=CARTESIAN_POINT('Ctrl Pts',(53.5704408284431,27.00969579586,12.3933094535792));
#55302=CARTESIAN_POINT('Ctrl Pts',(53.6362081782675,26.9624576309931,12.3975286329066));
#55303=CARTESIAN_POINT('Ctrl Pts',(53.7042218195668,26.9185527754667,12.4017478122341));
#55304=CARTESIAN_POINT('Ctrl Pts',(53.7741025915781,26.8781786611441,12.4059669915616));
#55305=CARTESIAN_POINT('Ctrl Pts',(53.8442058801495,26.8376759862922,12.4101996057331));
#55306=CARTESIAN_POINT('Ctrl Pts',(53.9164489565371,26.8005759568308,12.4144322199045));
#55307=CARTESIAN_POINT('Ctrl Pts',(53.9904678978455,26.7671105749009,12.418664834076));
#55308=CARTESIAN_POINT('Ctrl Pts',(54.064381258084,26.733692928196,12.4228914108208));
#55309=CARTESIAN_POINT('Ctrl Pts',(54.1400650323931,26.7038998217604,12.4271179875656));
#55310=CARTESIAN_POINT('Ctrl Pts',(54.2171292003915,26.677918269931,12.4313445643104));
#55311=CARTESIAN_POINT('Ctrl Pts',(54.2941078360873,26.6519655546154,12.4355664500444));
#55312=CARTESIAN_POINT('Ctrl Pts',(54.3724633832531,26.6298161358043,12.4397883357784));
#55313=CARTESIAN_POINT('Ctrl Pts',(54.4517855654801,26.6116090806185,12.4440102215125));
#55314=CARTESIAN_POINT('Ctrl Pts',(54.5310542473551,26.5934143055268,12.4482292597155));
#55315=CARTESIAN_POINT('Ctrl Pts',(54.6112878178253,26.5791567167086,12.4524482979185));
#55316=CARTESIAN_POINT('Ctrl Pts',(54.6920617649522,26.5689252801702,12.4566673361215));
#55317=CARTESIAN_POINT('Ctrl Pts',(54.772809334253,26.5586971848459,12.4608849965405));
#55318=CARTESIAN_POINT('Ctrl Pts',(54.8540964692445,26.5524926890319,12.4651026569595));
#55319=CARTESIAN_POINT('Ctrl Pts',(54.9354907760897,26.5503492473354,12.4693203173785));
#55320=CARTESIAN_POINT('Ctrl Pts',(55.0168833891502,26.548205850243,12.4735378900295));
#55321=CARTESIAN_POINT('Ctrl Pts',(55.0983827052123,26.5501233502976,12.4777554626806));
#55322=CARTESIAN_POINT('Ctrl Pts',(55.1795549856887,26.5560871011605,12.4819730353316));
#55323=CARTESIAN_POINT('Ctrl Pts',(55.2608650606469,26.5620609758237,12.4861977675479));
#55324=CARTESIAN_POINT('Ctrl Pts',(55.3418465235327,26.5720948098158,12.4904224997642));
#55325=CARTESIAN_POINT('Ctrl Pts',(55.4220690378045,26.5861217973297,12.4946472319805));
#55326=CARTESIAN_POINT('Ctrl Pts',(55.5022715156622,26.6001452814564,12.4988709090256));
#55327=CARTESIAN_POINT('Ctrl Pts',(55.5817149740569,26.6181598008781,12.5030945860707));
#55328=CARTESIAN_POINT('Ctrl Pts',(55.6599818805912,26.6400478463979,12.5073182631158));
#55329=CARTESIAN_POINT('Ctrl Pts',(55.7383907907371,26.661975604507,12.5115496033921));
#55330=CARTESIAN_POINT('Ctrl Pts',(55.8156184410779,26.6877907860973,12.5157809436683));
#55331=CARTESIAN_POINT('Ctrl Pts',(55.8912642110511,26.7173264893771,12.5200122839446));
#55332=CARTESIAN_POINT('Ctrl Pts',(55.9666925737087,26.7467773065098,12.5242314632721));
#55333=CARTESIAN_POINT('Ctrl Pts',(56.0405477552908,26.7799270258922,12.5284506425996));
#55334=CARTESIAN_POINT('Ctrl Pts',(56.1124577295447,26.8165650799769,12.5326698219271));
#55335=CARTESIAN_POINT('Ctrl Pts',(56.184596681808,26.8533197981096,12.5369024360986));
#55336=CARTESIAN_POINT('Ctrl Pts',(56.2550463114903,26.8937218271381,12.5411350502701));
#55337=CARTESIAN_POINT('Ctrl Pts',(56.3234138894252,26.937592201509,12.5453676644416));
#55338=CARTESIAN_POINT('Ctrl Pts',(56.3916839474295,26.9813999989101,12.5495942411864));
#55339=CARTESIAN_POINT('Ctrl Pts',(56.4578774644656,27.0286660669415,12.5538208179312));
#55340=CARTESIAN_POINT('Ctrl Pts',(56.5216252407799,27.0791650574239,12.558047394676));
#55341=CARTESIAN_POINT('Ctrl Pts',(56.5853022644443,27.1296079998745,12.56226928041));
#55342=CARTESIAN_POINT('Ctrl Pts',(56.6465385787679,27.1832764480855,12.566491166144));
#55343=CARTESIAN_POINT('Ctrl Pts',(56.7049941759336,27.2399019601078,12.570713051878));
#55344=CARTESIAN_POINT('Ctrl Pts',(56.7634103466118,27.2964892799782,12.5749320900811));
#55345=CARTESIAN_POINT('Ctrl Pts',(56.819049192248,27.3560293801257,12.5791511282841));
#55346=CARTESIAN_POINT('Ctrl Pts',(56.8716049812702,27.4182146023924,12.5833701664871));
#55347=CARTESIAN_POINT('Ctrl Pts',(56.9241436074878,27.4803795172328,12.5875878269061));
#55348=CARTESIAN_POINT('Ctrl Pts',(56.9736008769283,27.5451874842039,12.591805487325));
#55349=CARTESIAN_POINT('Ctrl Pts',(57.0197099761688,27.6122961907653,12.596023147744));
#55350=CARTESIAN_POINT('Ctrl Pts',(57.0658181158963,27.6794035008199,12.600240720395));
#55351=CARTESIAN_POINT('Ctrl Pts',(57.1085779618512,27.7488110717251,12.6044582930461));
#55352=CARTESIAN_POINT('Ctrl Pts',(57.1477656721151,27.8201470991332,12.6086758656971));
#55353=CARTESIAN_POINT('Ctrl Pts',(57.1870199057069,27.8916042234338,12.6129005979134));
#55354=CARTESIAN_POINT('Ctrl Pts',(57.2226896463142,27.9649959447701,12.6171253301297));
#55355=CARTESIAN_POINT('Ctrl Pts',(57.2545966567732,28.0399249168596,12.621350062346));
#55356=CARTESIAN_POINT('Ctrl Pts',(57.2864956981217,28.1148351746525,12.6255737393911));
#55357=CARTESIAN_POINT('Ctrl Pts',(57.3146337475737,28.1912814706043,12.6297974164362));
#55358=CARTESIAN_POINT('Ctrl Pts',(57.3388820698342,28.2688495959051,12.6340210934813));
#55359=CARTESIAN_POINT('Ctrl Pts',(57.3631743870536,28.3465584569833,12.6382524337576));
#55360=CARTESIAN_POINT('Ctrl Pts',(57.3835627565969,28.4253927640143,12.6424837740338));
#55361=CARTESIAN_POINT('Ctrl Pts',(57.3999690817405,28.5049256048937,12.64671511431));
#55362=CARTESIAN_POINT('Ctrl Pts',(57.4163282548078,28.5842298669453,12.6509342936375));
#55363=CARTESIAN_POINT('Ctrl Pts',(57.4287282543084,28.6642281903906,12.6551534729651));
#55364=CARTESIAN_POINT('Ctrl Pts',(57.4371431782213,28.7444938770808,12.6593726522926));
#55365=CARTESIAN_POINT('Ctrl Pts',(57.4455848972006,28.8250151483037,12.663605266464));
#55366=CARTESIAN_POINT('Ctrl Pts',(57.4500474912131,28.9061049721206,12.6678378806355));
#55367=CARTESIAN_POINT('Ctrl Pts',(57.450467279005,28.9873364884079,12.672070494807));
#55368=CARTESIAN_POINT('Ctrl Pts',(57.450886468009,29.0684521355645,12.6762970715518));
#55369=CARTESIAN_POINT('Ctrl Pts',(57.4472743017879,29.1497086130906,12.6805236482966));
#55370=CARTESIAN_POINT('Ctrl Pts',(57.4396188154356,29.2306735471884,12.6847502250414));
#55371=CARTESIAN_POINT('Ctrl Pts',(57.4319718257868,29.3115486195849,12.6889721107754));
#55372=CARTESIAN_POINT('Ctrl Pts',(57.4202904764019,29.3921323313502,12.6931939965094));
#55373=CARTESIAN_POINT('Ctrl Pts',(57.4046148426304,29.4719933353362,12.6974158822434));
#55374=CARTESIAN_POINT('Ctrl Pts',(57.3889497815877,29.5518004755516,12.7016349204465));
#55375=CARTESIAN_POINT('Ctrl Pts',(57.3692958759655,29.6308854214205,12.7058539586495));
#55376=CARTESIAN_POINT('Ctrl Pts',(57.3457447566737,29.7088242282385,12.7100729968525));
#55377=CARTESIAN_POINT('Ctrl Pts',(57.3222013283188,29.7867375830837,12.7142906572715));
#55378=CARTESIAN_POINT('Ctrl Pts',(57.2947633480454,29.8635050978406,12.7185083176904));
#55379=CARTESIAN_POINT('Ctrl Pts',(57.2635727028055,29.9387166074561,12.7227259781094));
#55380=CARTESIAN_POINT('Ctrl Pts',(57.2323827066312,30.0139265519484,12.7269435507604));
#55381=CARTESIAN_POINT('Ctrl Pts',(57.1974403797963,30.0875801270172,12.7311611234115));
#55382=CARTESIAN_POINT('Ctrl Pts',(57.1589357414466,30.1592871578277,12.7353786960625));
#55383=CARTESIAN_POINT('Ctrl Pts',(57.1203657393218,30.2311159153298,12.7396034282788));
#55384=CARTESIAN_POINT('Ctrl Pts',(57.0782215475278,30.300991105875,12.7438281604951));
#55385=CARTESIAN_POINT('Ctrl Pts',(57.0327394376947,30.3685469039973,12.7480528927114));
#55386=CARTESIAN_POINT('Ctrl Pts',(56.9872686874955,30.4360858293506,12.7522765697565));
#55387=CARTESIAN_POINT('Ctrl Pts',(56.9384619827175,30.5013061602331,12.7565002468016));
#55388=CARTESIAN_POINT('Ctrl Pts',(56.8865966885616,30.5638744146218,12.7607239238467));
#55389=CARTESIAN_POINT('Ctrl Pts',(56.8346372925762,30.6265561897625,12.764955264123));
#55390=CARTESIAN_POINT('Ctrl Pts',(56.7796085318711,30.6865759287903,12.7691866043992));
#55391=CARTESIAN_POINT('Ctrl Pts',(56.7218259951699,30.743635710909,12.7734179446755));
#55392=CARTESIAN_POINT('Ctrl Pts',(56.6642095265277,30.8005315021786,12.777637124003));
#55393=CARTESIAN_POINT('Ctrl Pts',(56.6038554843972,30.854484086363,12.7818563033305));
#55394=CARTESIAN_POINT('Ctrl Pts',(56.5411076928689,30.9052394413774,12.786075482658));
#55395=CARTESIAN_POINT('Ctrl Pts',(56.4781600978426,30.9561564131951,12.7903080968295));
#55396=CARTESIAN_POINT('Ctrl Pts',(56.4125693477172,31.0040451150984,12.794540711001));
#55397=CARTESIAN_POINT('Ctrl Pts',(56.3446588354071,31.0486197466494,12.7987733251724));
#55398=CARTESIAN_POINT('Ctrl Pts',(56.2768451910662,31.0931307966737,12.8029999019172));
#55399=CARTESIAN_POINT('Ctrl Pts',(56.2067187416237,31.1343369124013,12.807226478662));
#55400=CARTESIAN_POINT('Ctrl Pts',(56.1346356594244,31.1719926727231,12.8114530554068));
#55401=CARTESIAN_POINT('Ctrl Pts',(56.0626325810993,31.2096066395112,12.8156749411409));
#55402=CARTESIAN_POINT('Ctrl Pts',(55.9886775947289,31.2436778666138,12.8198968268749));
#55403=CARTESIAN_POINT('Ctrl Pts',(55.9131543422353,31.2740051445097,12.8241187126089));
#55404=CARTESIAN_POINT('Ctrl Pts',(55.8376820278334,31.3043119675972,12.8283377508119));
#55405=CARTESIAN_POINT('Ctrl Pts',(55.7606439780632,31.3308796840387,12.832556789015));
#55406=CARTESIAN_POINT('Ctrl Pts',(55.6824456923792,31.353554360314,12.836775827218));
#55407=CARTESIAN_POINT('Ctrl Pts',(55.6042729434042,31.3762216318668,12.840993487637));
#55408=CARTESIAN_POINT('Ctrl Pts',(55.5249411567974,31.3949982587529,12.8452111480559));
#55409=CARTESIAN_POINT('Ctrl Pts',(55.4448716327238,31.4097799651416,12.8494288084749));
#55410=CARTESIAN_POINT('Ctrl Pts',(55.3648037748668,31.4245613639285,12.853646381126));
#55411=CARTESIAN_POINT('Ctrl Pts',(55.2839986671085,31.4353479243268,12.857863953777));
#55412=CARTESIAN_POINT('Ctrl Pts',(55.2028870445195,31.4420866276949,12.8620815264281));
#55413=CARTESIAN_POINT('Ctrl Pts',(55.121637730419,31.4488367703885,12.8663062586444));
#55414=CARTESIAN_POINT('Ctrl Pts',(55.0400813258277,31.4515252691936,12.8705309908606));
#55415=CARTESIAN_POINT('Ctrl Pts',(54.9586533208412,31.4501511590354,12.8747557230769));
#55416=CARTESIAN_POINT('Ctrl Pts',(54.8772456533528,31.4487773920756,12.878979400122));
#55417=CARTESIAN_POINT('Ctrl Pts',(54.7959667850363,31.4433430975585,12.8832030771672));
#55418=CARTESIAN_POINT('Ctrl Pts',(54.7152474468644,31.4338993885292,12.8874267542123));
#55419=CARTESIAN_POINT('Ctrl Pts',(54.63438165551,31.4244385453004,12.8916580944885));
#55420=CARTESIAN_POINT('Ctrl Pts',(54.5540778825753,31.4109538269064,12.8958894347648));
#55421=CARTESIAN_POINT('Ctrl Pts',(54.4747578382954,31.3935477688085,12.900120775041));
#55422=CARTESIAN_POINT('Ctrl Pts',(54.3956657612624,31.3761917360374,12.9043399543685));
#55423=CARTESIAN_POINT('Ctrl Pts',(54.3175521833678,31.3549370732523,12.908559133696));
#55424=CARTESIAN_POINT('Ctrl Pts',(54.2408173628565,31.3299338989465,12.9127783130235));
#55425=CARTESIAN_POINT('Ctrl Pts',(54.1638382009078,31.3048511087438,12.917010927195));
#55426=CARTESIAN_POINT('Ctrl Pts',(54.0879602923918,31.2759025807811,12.9212435413664));
#55427=CARTESIAN_POINT('Ctrl Pts',(54.0135994292889,31.2432039952044,12.9254761555379));
#55428=CARTESIAN_POINT('Ctrl Pts',(53.9393446349751,31.2105520510897,12.9297027322827));
#55429=CARTESIAN_POINT('Ctrl Pts',(53.8666030099624,31.1741608588139,12.9339293090275));
#55430=CARTESIAN_POINT('Ctrl Pts',(53.7957743201799,31.1341955772754,12.9381558857723));
#55431=CARTESIAN_POINT('Ctrl Pts',(53.7250242420413,31.0942746525715,12.9423777715063));
#55432=CARTESIAN_POINT('Ctrl Pts',(53.6561832830115,31.0507877478164,12.9465996572403));
#55433=CARTESIAN_POINT('Ctrl Pts',(53.5896290776845,31.0039471329072,12.9508215429744));
#55434=CARTESIAN_POINT('Ctrl Pts',(53.523119761105,30.9571381105401,12.9550405811774));
#55435=CARTESIAN_POINT('Ctrl Pts',(53.4588945139114,30.9069801371739,12.9592596193804));
#55436=CARTESIAN_POINT('Ctrl Pts',(53.3973032136534,30.8537295544481,12.9634786575834));
#55437=CARTESIAN_POINT('Ctrl Pts',(53.3357320268686,30.8004963614212,12.9676963180024));
#55438=CARTESIAN_POINT('Ctrl Pts',(53.2767934299597,30.7441728682958,12.9719139784213));
#55439=CARTESIAN_POINT('Ctrl Pts',(53.2208042482739,30.6850557044323,12.9761316388403));
#55440=CARTESIAN_POINT('Ctrl Pts',(53.1648162317018,30.6259397707746,12.9803492114913));
#55441=CARTESIAN_POINT('Ctrl Pts',(53.1117778269088,30.5640306200612,12.9845667841424));
#55442=CARTESIAN_POINT('Ctrl Pts',(53.0619679997887,30.4996607003442,12.9887843567934));
#55443=CARTESIAN_POINT('Ctrl Pts',(53.0120736177038,30.4351815090918,12.9930090890097));
#55444=CARTESIAN_POINT('Ctrl Pts',(52.9654190646665,30.3682335603809,12.997233821226));
#55445=CARTESIAN_POINT('Ctrl Pts',(52.9222422313652,30.2991816289025,13.0014585534423));
#55446=CARTESIAN_POINT('Ctrl Pts',(52.8790761819308,30.2301469438683,13.0056822304874));
#55447=CARTESIAN_POINT('Ctrl Pts',(52.8393863238212,30.1590097443526,13.0099059075325));
#55448=CARTESIAN_POINT('Ctrl Pts',(52.8033642724133,30.0861591643446,13.0141295845776));
#55449=CARTESIAN_POINT('Ctrl Pts',(52.7672768643736,30.0131764078405,13.0183609248539));
#55450=CARTESIAN_POINT('Ctrl Pts',(52.7348707476153,29.938474485681,13.0225922651301));
#55451=CARTESIAN_POINT('Ctrl Pts',(52.7062894921986,29.8624629594375,13.0268236054064));
#55452=CARTESIAN_POINT('Ctrl Pts',(52.6777903798286,29.7866698916994,13.0310427847339));
#55453=CARTESIAN_POINT('Ctrl Pts',(52.6530942323866,29.7095751964007,13.0352619640614));
#55454=CARTESIAN_POINT('Ctrl Pts',(52.6322930276046,29.6315963448834,13.0394811433889));
#55455=CARTESIAN_POINT('Ctrl Pts',(52.6050199400275,29.5293559184811,13.0450130367821));
#55456=CARTESIAN_POINT('Ctrl Pts',(52.5843565008141,29.4252836172886,13.0505449301752));
#55457=CARTESIAN_POINT('Ctrl Pts',(52.5705005679496,29.3201292858624,13.0560768235684));
#55458=CARTESIAN_POINT('Ctrl Pts',(52.5566446350851,29.2149749544363,13.0616087169615));
#55459=CARTESIAN_POINT('Ctrl Pts',(52.5495963971629,29.1087382537186,13.0671406103546));
#55460=CARTESIAN_POINT('Ctrl Pts',(52.5495009826471,29.0021945278826,13.0726725037477));
#55461=CARTESIAN_POINT('',(52.5495001938469,28.9990252981815,13.8726725038318));
#55462=CARTESIAN_POINT('Ctrl Pts',(52.5495009826464,29.0021945271091,13.0726725037879));
#55463=CARTESIAN_POINT('Ctrl Pts',(52.5494289300536,28.9217376454537,13.0768499331819));
#55464=CARTESIAN_POINT('Ctrl Pts',(52.5533235784428,28.841186950602,13.081027362576));
#55465=CARTESIAN_POINT('Ctrl Pts',(52.5611859230216,28.7609683118659,13.08520479197));
#55466=CARTESIAN_POINT('Ctrl Pts',(52.5690438911062,28.6807943260201,13.0893798960404));
#55467=CARTESIAN_POINT('Ctrl Pts',(52.580865127151,28.6009525014319,13.0935550001108));
#55468=CARTESIAN_POINT('Ctrl Pts',(52.5965985987663,28.5218661750641,13.0977301041812));
#55469=CARTESIAN_POINT('Ctrl Pts',(52.6123283691213,28.4427984535589,13.1019042260687));
#55470=CARTESIAN_POINT('Ctrl Pts',(52.6319684549278,28.3644863432227,13.1060783479562));
#55471=CARTESIAN_POINT('Ctrl Pts',(52.6554165300878,28.28734398016,13.1102524698437));
#55472=CARTESIAN_POINT('Ctrl Pts',(52.6788666251593,28.2101949717435,13.1144269513069));
#55473=CARTESIAN_POINT('Ctrl Pts',(52.7061252202815,28.1342163645467,13.11860143277));
#55474=CARTESIAN_POINT('Ctrl Pts',(52.7370403045377,28.0598065801586,13.1227759142332));
#55475=CARTESIAN_POINT('Ctrl Pts',(52.7679875097762,27.9853194834994,13.1269547330109));
#55476=CARTESIAN_POINT('Ctrl Pts',(52.8025986026244,27.9124049018382,13.1311335517887));
#55477=CARTESIAN_POINT('Ctrl Pts',(52.8406739506139,27.8414400048152,13.1353123705664));
#55478=CARTESIAN_POINT('Ctrl Pts',(52.8787716922654,27.7704333704478,13.1394936470776));
#55479=CARTESIAN_POINT('Ctrl Pts',(52.9203374967399,27.7013791082765,13.1436749235887));
#55480=CARTESIAN_POINT('Ctrl Pts',(52.9651277559891,27.6346263513037,13.1478562000999));
#55481=CARTESIAN_POINT('Ctrl Pts',(53.0099918254053,27.5677635920176,13.1520443669645));
#55482=CARTESIAN_POINT('Ctrl Pts',(53.0580906682687,27.5032102855713,13.1562325338291));
#55483=CARTESIAN_POINT('Ctrl Pts',(53.1091401107616,27.4412828578382,13.1604207006937));
#55484=CARTESIAN_POINT('Ctrl Pts',(53.132556232595,27.4128770590317,13.162341791714));
#55485=CARTESIAN_POINT('Ctrl Pts',(53.1565926487538,27.3850232386561,13.1642628827342));
#55486=CARTESIAN_POINT('Ctrl Pts',(53.1812194676012,27.3577492198306,13.1661839737544));
#55487=CARTESIAN_POINT('Ctrl Pts',(53.2354781265375,27.2976581583562,13.1704165879259));
#55488=CARTESIAN_POINT('Ctrl Pts',(53.2928189273524,27.2401472304043,13.1746492020974));
#55489=CARTESIAN_POINT('Ctrl Pts',(53.3529668841377,27.1855490733412,13.1788818162689));
#55490=CARTESIAN_POINT('Ctrl Pts',(53.4130290455103,27.1310287954227,13.1831083930137));
#55491=CARTESIAN_POINT('Ctrl Pts',(53.475890068994,27.0794133460753,13.1873349697584));
#55492=CARTESIAN_POINT('Ctrl Pts',(53.5412363057285,27.0310005753491,13.1915615465032));
#55493=CARTESIAN_POINT('Ctrl Pts',(53.6065100157072,26.9826415371924,13.1957834322373));
#55494=CARTESIAN_POINT('Ctrl Pts',(53.6742630868148,26.9374783898175,13.2000053179713));
#55495=CARTESIAN_POINT('Ctrl Pts',(53.7441478561528,26.8957695841961,13.2042272037053));
#55496=CARTESIAN_POINT('Ctrl Pts',(53.8139854903811,26.8540889098706,13.2084462419083));
#55497=CARTESIAN_POINT('Ctrl Pts',(53.8859515694386,26.8158581874815,13.2126652801113));
#55498=CARTESIAN_POINT('Ctrl Pts',(53.9596694832852,26.7812925686355,13.2168843183144));
#55499=CARTESIAN_POINT('Ctrl Pts',(54.0333633235488,26.7467382376605,13.2211019787333));
#55500=CARTESIAN_POINT('Ctrl Pts',(54.1088074421907,26.7158468303473,13.2253196391523));
#55501=CARTESIAN_POINT('Ctrl Pts',(54.185601894513,26.6887869038578,13.2295372995712));
#55502=CARTESIAN_POINT('Ctrl Pts',(54.2623947487719,26.6617275404751,13.2337548722223));
#55503=CARTESIAN_POINT('Ctrl Pts',(54.3405374423082,26.638499652669,13.2379724448733));
#55504=CARTESIAN_POINT('Ctrl Pts',(54.4196127351737,26.6192226326623,13.2421900175244));
#55505=CARTESIAN_POINT('Ctrl Pts',(54.4988222627673,26.5999128888371,13.2464147497406));
#55506=CARTESIAN_POINT('Ctrl Pts',(54.5789671034754,26.5845675421948,13.2506394819569));
#55507=CARTESIAN_POINT('Ctrl Pts',(54.659617221074,26.5732553051855,13.2548642141732));
#55508=CARTESIAN_POINT('Ctrl Pts',(54.7402471954598,26.5619458935259,13.2590878912183));
#55509=CARTESIAN_POINT('Ctrl Pts',(54.8213817281834,26.5546675976121,13.2633115682634));
#55510=CARTESIAN_POINT('Ctrl Pts',(54.9025873812025,26.5514369455334,13.2675352453085));
#55511=CARTESIAN_POINT('Ctrl Pts',(54.9839403697499,26.548200431919,13.2717665855848));
#55512=CARTESIAN_POINT('Ctrl Pts',(55.0653642705953,26.5490262338384,13.275997925861));
#55513=CARTESIAN_POINT('Ctrl Pts',(55.1464265556148,26.5538786796623,13.2802292661372));
#55514=CARTESIAN_POINT('Ctrl Pts',(55.2272558661565,26.5587171794689,13.2844484454647));
#55515=CARTESIAN_POINT('Ctrl Pts',(55.3077251932352,26.56755907639,13.2886676247923));
#55516=CARTESIAN_POINT('Ctrl Pts',(55.3874157958816,26.5803183574897,13.2928868041198));
#55517=CARTESIAN_POINT('Ctrl Pts',(55.4673601518598,26.5931182670949,13.2971194182912));
#55518=CARTESIAN_POINT('Ctrl Pts',(55.546818147273,26.6099081818321,13.3013520324627));
#55519=CARTESIAN_POINT('Ctrl Pts',(55.6253610549565,26.630638524635,13.3055846466342));
#55520=CARTESIAN_POINT('Ctrl Pts',(55.7037919285573,26.6513392975505,13.309811223379));
#55521=CARTESIAN_POINT('Ctrl Pts',(55.7813098614613,26.675969217629,13.3140378001238));
#55522=CARTESIAN_POINT('Ctrl Pts',(55.85749425884,26.7044273381014,13.3182643768686));
#55523=CARTESIAN_POINT('Ctrl Pts',(55.9335941003594,26.7328538733553,13.3224862626026));
#55524=CARTESIAN_POINT('Ctrl Pts',(56.0083629142646,26.7651000047905,13.3267081483366));
#55525=CARTESIAN_POINT('Ctrl Pts',(56.0813946373982,26.8010148049142,13.3309300340707));
#55526=CARTESIAN_POINT('Ctrl Pts',(56.1543771028993,26.836905381619,13.3351490722737));
#55527=CARTESIAN_POINT('Ctrl Pts',(56.2256243887639,26.8764595081574,13.3393681104767));
#55528=CARTESIAN_POINT('Ctrl Pts',(56.2947509935872,26.9194784032351,13.3435871486797));
#55529=CARTESIAN_POINT('Ctrl Pts',(56.3638550241815,26.9624832499102,13.3478048090987));
#55530=CARTESIAN_POINT('Ctrl Pts',(56.4308393549625,27.0089503728386,13.3520224695177));
#55531=CARTESIAN_POINT('Ctrl Pts',(56.4953448657147,27.0586360509733,13.3562401299366));
#55532=CARTESIAN_POINT('Ctrl Pts',(56.5598490341317,27.1083206951678,13.3604577025877));
#55533=CARTESIAN_POINT('Ctrl Pts',(56.6218741177678,27.1612234769942,13.3646752752387));
#55534=CARTESIAN_POINT('Ctrl Pts',(56.6810928216502,27.2170594022805,13.3688928478898));
#55535=CARTESIAN_POINT('Ctrl Pts',(56.7404120525915,27.27299011217,13.3731175801061));
#55536=CARTESIAN_POINT('Ctrl Pts',(56.7969150323778,27.3318636073182,13.3773423123224));
#55537=CARTESIAN_POINT('Ctrl Pts',(56.8503100112058,27.3933565696049,13.3815670445387));
#55538=CARTESIAN_POINT('Ctrl Pts',(56.9036916540778,27.4548341733794,13.3857907215838));
#55539=CARTESIAN_POINT('Ctrl Pts',(56.9539665773336,27.5189295560783,13.3900143986289));
#55540=CARTESIAN_POINT('Ctrl Pts',(57.0008849527752,27.5852881368427,13.394238075674));
#55541=CARTESIAN_POINT('Ctrl Pts',(57.047888454601,27.6517671153402,13.3984694159503));
#55542=CARTESIAN_POINT('Ctrl Pts',(57.0915229883876,27.7205171047142,13.4027007562265));
#55543=CARTESIAN_POINT('Ctrl Pts',(57.1315830077382,27.7911558697988,13.4069320965027));
#55544=CARTESIAN_POINT('Ctrl Pts',(57.1715278938663,27.8615916177911,13.4111512758303));
#55545=CARTESIAN_POINT('Ctrl Pts',(57.207918654212,27.9339048551902,13.4153704551578));
#55546=CARTESIAN_POINT('Ctrl Pts',(57.2405994756744,28.0076975059955,13.4195896344853));
#55547=CARTESIAN_POINT('Ctrl Pts',(57.2733843604399,28.0817251296883,13.4238222486568));
#55548=CARTESIAN_POINT('Ctrl Pts',(57.3025575531594,28.1575169438805,13.4280548628283));
#55549=CARTESIAN_POINT('Ctrl Pts',(57.3279272409129,28.2346863316157,13.4322874769998));
#55550=CARTESIAN_POINT('Ctrl Pts',(57.3532607411888,28.3117456444653,13.4365140537445));
#55551=CARTESIAN_POINT('Ctrl Pts',(57.3748013680508,28.3901781905108,13.4407406304893));
#55552=CARTESIAN_POINT('Ctrl Pts',(57.3924048260317,28.4695762086971,13.4449672072341));
#55553=CARTESIAN_POINT('Ctrl Pts',(57.4099887462126,28.548886104277,13.4491890929682));
#55554=CARTESIAN_POINT('Ctrl Pts',(57.4236440802519,28.6291588915563,13.4534109787022));
#55555=CARTESIAN_POINT('Ctrl Pts',(57.4332763688275,28.7099717894661,13.4576328644362));
#55556=CARTESIAN_POINT('Ctrl Pts',(57.4429021607232,28.7907301815824,13.4618519026392));
#55557=CARTESIAN_POINT('Ctrl Pts',(57.4485102414036,28.8720275007288,13.4660709408423));
#55558=CARTESIAN_POINT('Ctrl Pts',(57.4500574863572,28.9534321619047,13.4702899790453));
#55559=CARTESIAN_POINT('Ctrl Pts',(57.4516042260371,29.0348102392863,13.4745076394643));
#55560=CARTESIAN_POINT('Ctrl Pts',(57.4490927547638,29.1162951249738,13.4787252998832));
#55561=CARTESIAN_POINT('Ctrl Pts',(57.4425320065654,29.1974528979361,13.4829429603022));
#55562=CARTESIAN_POINT('Ctrl Pts',(57.4359713948938,29.2786089820359,13.4871605329532));
#55563=CARTESIAN_POINT('Ctrl Pts',(57.4253617124377,29.3594375040021,13.4913781056043));
#55564=CARTESIAN_POINT('Ctrl Pts',(57.4107638398513,29.4395087694977,13.4955956782553));
#55565=CARTESIAN_POINT('Ctrl Pts',(57.3961411865605,29.5197159604404,13.4998204104716));
#55566=CARTESIAN_POINT('Ctrl Pts',(57.3775168813565,29.5991628635351,13.5040451426879));
#55567=CARTESIAN_POINT('Ctrl Pts',(57.3550033028067,29.6774287370413,13.5082698749042));
#55568=CARTESIAN_POINT('Ctrl Pts',(57.3324953472592,29.755675062825,13.5124935519493));
#55569=CARTESIAN_POINT('Ctrl Pts',(57.3061002320462,29.8327405147774,13.5167172289944));
#55570=CARTESIAN_POINT('Ctrl Pts',(57.2759793818649,29.9082224965977,13.5209409060395));
#55571=CARTESIAN_POINT('Ctrl Pts',(57.2458038818999,29.9838414291995,13.5251722463158));
#55572=CARTESIAN_POINT('Ctrl Pts',(57.2118893318033,30.0578707265719,13.529403586592));
#55573=CARTESIAN_POINT('Ctrl Pts',(57.1744444604506,30.1299298820794,13.5336349268683));
#55574=CARTESIAN_POINT('Ctrl Pts',(57.1371072063378,30.2017819382658,13.5378541061957));
#55575=CARTESIAN_POINT('Ctrl Pts',(57.096260197805,30.2716748108313,13.5420732855232));
#55576=CARTESIAN_POINT('Ctrl Pts',(57.0521525262661,30.3392610869206,13.5462924648507));
#55577=CARTESIAN_POINT('Ctrl Pts',(57.0079044056871,30.4070625733638,13.5505250790222));
#55578=CARTESIAN_POINT('Ctrl Pts',(56.9602102295495,30.4727949081355,13.5547576931936));
#55579=CARTESIAN_POINT('Ctrl Pts',(56.9092898788012,30.5360867191365,13.5589903073651));
#55580=CARTESIAN_POINT('Ctrl Pts',(56.8584421611521,30.5992882503118,13.5632168841099));
#55581=CARTESIAN_POINT('Ctrl Pts',(56.8043776975106,30.6600558128422,13.5674434608547));
#55582=CARTESIAN_POINT('Ctrl Pts',(56.7473599735678,30.7180463826024,13.5716700375995));
#55583=CARTESIAN_POINT('Ctrl Pts',(56.690405532696,30.7759725895454,13.5758919233335));
#55584=CARTESIAN_POINT('Ctrl Pts',(56.6305046685124,30.8311275983423,13.5801138090675));
#55585=CARTESIAN_POINT('Ctrl Pts',(56.5679605967124,30.8832020117761,13.5843356948016));
#55586=CARTESIAN_POINT('Ctrl Pts',(56.5054587089492,30.9352413026328,13.5885547330046));
#55587=CARTESIAN_POINT('Ctrl Pts',(56.4403175103725,30.9842038282754,13.5927737712076));
#55588=CARTESIAN_POINT('Ctrl Pts',(56.3728755483497,31.0298184595534,13.5969928094106));
#55589=CARTESIAN_POINT('Ctrl Pts',(56.3054556104129,31.0754181947558,13.6012104698296));
#55590=CARTESIAN_POINT('Ctrl Pts',(56.2357367856598,31.1176719467605,13.6054281302486));
#55591=CARTESIAN_POINT('Ctrl Pts',(56.1640879216899,31.1563509826964,13.6096457906675));
#55592=CARTESIAN_POINT('Ctrl Pts',(56.0924405487059,31.1950292137361,13.6138633633186));
#55593=CARTESIAN_POINT('Ctrl Pts',(56.0188636257034,31.2301326569648,13.6180809359696));
#55594=CARTESIAN_POINT('Ctrl Pts',(55.9437507346095,31.2614784546672,13.6222985086207));
#55595=CARTESIAN_POINT('Ctrl Pts',(55.8685103351858,31.2928774636128,13.626523240837));
#55596=CARTESIAN_POINT('Ctrl Pts',(55.791729181861,31.3205058846649,13.6307479730533));
#55597=CARTESIAN_POINT('Ctrl Pts',(55.7138213824043,31.344228931658,13.6349727052695));
#55598=CARTESIAN_POINT('Ctrl Pts',(55.6359330412375,31.3679460535713,13.6391963823147));
#55599=CARTESIAN_POINT('Ctrl Pts',(55.5569190739749,31.3877596592283,13.6434200593598));
#55600=CARTESIAN_POINT('Ctrl Pts',(55.4772050682852,31.4035859819867,13.6476437364049));
#55601=CARTESIAN_POINT('Ctrl Pts',(55.3973464334388,31.4194410192438,13.6518750766811));
#55602=CARTESIAN_POINT('Ctrl Pts',(55.3167856828188,31.4312942482234,13.6561064169574));
#55603=CARTESIAN_POINT('Ctrl Pts',(55.2359556271585,31.4391136078527,13.6603377572336));
#55604=CARTESIAN_POINT('Ctrl Pts',(55.1553578785446,31.4469104945006,13.6645569365611));
#55605=CARTESIAN_POINT('Ctrl Pts',(55.0744928294408,31.450696729456,13.6687761158887));
#55606=CARTESIAN_POINT('Ctrl Pts',(54.9937875040814,31.4504921250423,13.6729952952162));
#55607=CARTESIAN_POINT('Ctrl Pts',(54.9128251942782,31.4502868691208,13.6772279093877));
#55608=CARTESIAN_POINT('Ctrl Pts',(54.8317225056717,31.4460645270235,13.6814605235591));
#55609=CARTESIAN_POINT('Ctrl Pts',(54.750910657913,31.4378073651662,13.6856931377306));
#55610=CARTESIAN_POINT('Ctrl Pts',(54.6702140806669,31.429561981375,13.6899197144754));
#55611=CARTESIAN_POINT('Ctrl Pts',(54.5898079786112,31.4172932554024,13.6941462912202));
#55612=CARTESIAN_POINT('Ctrl Pts',(54.5101235308582,31.4010354630828,13.698372867965));
#55613=CARTESIAN_POINT('Ctrl Pts',(54.4305275236153,31.3847957150301,13.702594753699));
#55614=CARTESIAN_POINT('Ctrl Pts',(54.3516520320611,31.3645757902679,13.7068166394331));
#55615=CARTESIAN_POINT('Ctrl Pts',(54.2739216572553,31.3404615976762,13.7110385251671));
#55616=CARTESIAN_POINT('Ctrl Pts',(54.1962437091769,31.3163636693596,13.7152575633701));
#55617=CARTESIAN_POINT('Ctrl Pts',(54.1197097864442,31.2883768270864,13.7194766015731));
#55618=CARTESIAN_POINT('Ctrl Pts',(54.044731624488,31.2566374500009,13.7236956397761));
#55619=CARTESIAN_POINT('Ctrl Pts',(53.9697779476661,31.2249084378389,13.7279133001951));
#55620=CARTESIAN_POINT('Ctrl Pts',(53.8963794501245,31.1894295054698,13.7321309606141));
#55621=CARTESIAN_POINT('Ctrl Pts',(53.8249287996965,31.1503855292057,13.736348621033));
#55622=CARTESIAN_POINT('Ctrl Pts',(53.7534796361292,31.1113423654318,13.7405661936841));
#55623=CARTESIAN_POINT('Ctrl Pts',(53.6839786461747,31.0687345290583,13.7447837663351));
#55624=CARTESIAN_POINT('Ctrl Pts',(53.616793481816,31.0227926186471,13.7490013389862));
#55625=CARTESIAN_POINT('Ctrl Pts',(53.5494942668869,30.9767727192761,13.7532260712025));
#55626=CARTESIAN_POINT('Ctrl Pts',(53.4845191285391,30.9274076855743,13.7574508034188));
#55627=CARTESIAN_POINT('Ctrl Pts',(53.4222065694118,30.8749715038882,13.761675535635));
#55628=CARTESIAN_POINT('Ctrl Pts',(53.3599095734997,30.8225484186884,13.7658992126801));
#55629=CARTESIAN_POINT('Ctrl Pts',(53.3002741537448,30.7670560525255,13.7701228897253));
#55630=CARTESIAN_POINT('Ctrl Pts',(53.2436022659899,30.7088057964451,13.7743465667704));
#55631=CARTESIAN_POINT('Ctrl Pts',(53.1868275555596,30.6504498539755,13.7785779070466));
#55632=CARTESIAN_POINT('Ctrl Pts',(53.1330274304744,30.5893263714298,13.7828092473228));
#55633=CARTESIAN_POINT('Ctrl Pts',(53.0824644068832,30.5257809472956,13.7870405875991));
#55634=CARTESIAN_POINT('Ctrl Pts',(53.0320467023394,30.4624181538636,13.7912597669266));
#55635=CARTESIAN_POINT('Ctrl Pts',(52.9848477150114,30.3966477400224,13.7954789462541));
#55636=CARTESIAN_POINT('Ctrl Pts',(52.9410832981599,30.3288386903171,13.7996981255816));
#55637=CARTESIAN_POINT('Ctrl Pts',(52.8962263261542,30.2593368241167,13.8040226344542));
#55638=CARTESIAN_POINT('Ctrl Pts',(52.8548162274857,30.1874436103981,13.8083471433269));
#55639=CARTESIAN_POINT('Ctrl Pts',(52.8171099662843,30.1135265379436,13.8126716521995));
#55640=CARTESIAN_POINT('Ctrl Pts',(52.7794646483622,30.0397289350055,13.8169891715234));
#55641=CARTESIAN_POINT('Ctrl Pts',(52.7455114658633,29.9639143620006,13.8213066908472));
#55642=CARTESIAN_POINT('Ctrl Pts',(52.7154636607913,29.8864784062994,13.8256242101711));
#55643=CARTESIAN_POINT('Ctrl Pts',(52.685466354783,29.809172591327,13.8299344733682));
#55644=CARTESIAN_POINT('Ctrl Pts',(52.6593615204037,29.7302512227029,13.8342447365652));
#55645=CARTESIAN_POINT('Ctrl Pts',(52.6373154269118,29.6501321850909,13.8385549997623));
#55646=CARTESIAN_POINT('Ctrl Pts',(52.6152911752435,29.5700925241668,13.8428609926333));
#55647=CARTESIAN_POINT('Ctrl Pts',(52.5973177878601,29.488857972754,13.8471669855043));
#55648=CARTESIAN_POINT('Ctrl Pts',(52.5835123979253,29.4068635139934,13.8514729783753));
#55649=CARTESIAN_POINT('Ctrl Pts',(52.5697183850117,29.3249366268628,13.8557754226777));
#55650=CARTESIAN_POINT('Ctrl Pts',(52.5600856091676,29.2422515087223,13.8600778669802));
#55651=CARTESIAN_POINT('Ctrl Pts',(52.5546803144841,29.1592541541951,13.8643803112826));
#55652=CARTESIAN_POINT('Ctrl Pts',(52.5512077346424,29.1059332980501,13.8671443754511));
#55653=CARTESIAN_POINT('Ctrl Pts',(52.5494789304077,29.0524838000256,13.8699084396195));
#55654=CARTESIAN_POINT('Ctrl Pts',(52.5495001938466,28.9990252990303,13.8726725037879));
#55655=CARTESIAN_POINT('',(52.5495004475699,28.9985189396232,14.6726725037596));
#55656=CARTESIAN_POINT('Ctrl Pts',(52.5495001938469,28.9990252981815,13.8726725038318));
#55657=CARTESIAN_POINT('Ctrl Pts',(52.5495355260103,28.9101966350554,13.8772653771879));
#55658=CARTESIAN_POINT('Ctrl Pts',(52.5544050151296,28.8215184266261,13.881858250544));
#55659=CARTESIAN_POINT('Ctrl Pts',(52.5640346561721,28.733498417135,13.8864511239002));
#55660=CARTESIAN_POINT('Ctrl Pts',(52.5736906293279,28.6452377182093,13.8910565564016));
#55661=CARTESIAN_POINT('Ctrl Pts',(52.5881326985161,28.5576391306989,13.8956619889031));
#55662=CARTESIAN_POINT('Ctrl Pts',(52.6072358840093,28.4711993426373,13.9002674214045));
#55663=CARTESIAN_POINT('Ctrl Pts',(52.626421327776,28.3843873450441,13.9048926848879));
#55664=CARTESIAN_POINT('Ctrl Pts',(52.6503079795362,28.2987444485671,13.9095179483713));
#55665=CARTESIAN_POINT('Ctrl Pts',(52.6787204535448,28.2147538492877,13.9141432118546));
#55666=CARTESIAN_POINT('Ctrl Pts',(52.7038197685482,28.1405573358827,13.9182291265521));
#55667=CARTESIAN_POINT('Ctrl Pts',(52.7324501558775,28.0676500725619,13.9223150412496));
#55668=CARTESIAN_POINT('Ctrl Pts',(52.7644606708905,27.9963495837671,13.926400955947));
#55669=CARTESIAN_POINT('Ctrl Pts',(52.7976204819761,27.9224891432901,13.9306335701185));
#55670=CARTESIAN_POINT('Ctrl Pts',(52.8345063251939,27.850136473387,13.93486618429));
#55671=CARTESIAN_POINT('Ctrl Pts',(52.874958780294,27.7796926352142,13.9390987984615));
#55672=CARTESIAN_POINT('Ctrl Pts',(52.9153535337652,27.7093492785623,13.9433253752063));
#55673=CARTESIAN_POINT('Ctrl Pts',(52.9593045653985,27.6409097453732,13.947551951951));
#55674=CARTESIAN_POINT('Ctrl Pts',(53.0066049705101,27.5747538786564,13.9517785286958));
#55675=CARTESIAN_POINT('Ctrl Pts',(53.0538528776492,27.5086714372911,13.9560004144299));
#55676=CARTESIAN_POINT('Ctrl Pts',(53.1044425029408,27.4448680021315,13.9602223001639));
#55677=CARTESIAN_POINT('Ctrl Pts',(53.1581224634525,27.3836963805145,13.9644441858979));
#55678=CARTESIAN_POINT('Ctrl Pts',(53.2117662184956,27.3225660172593,13.9686632241009));
#55679=CARTESIAN_POINT('Ctrl Pts',(53.2684958634702,27.2640642903586,13.972882262304));
#55680=CARTESIAN_POINT('Ctrl Pts',(53.3280191598301,27.208511702493,13.977101300507));
#55681=CARTESIAN_POINT('Ctrl Pts',(53.3875230180515,27.1529772560772,13.981318960926));
#55682=CARTESIAN_POINT('Ctrl Pts',(53.4498183765196,27.1003903527954,13.9855366213449));
#55683=CARTESIAN_POINT('Ctrl Pts',(53.5145764689179,27.0510343298797,13.9897542817639));
#55684=CARTESIAN_POINT('Ctrl Pts',(53.5793332137248,27.0016793340441,13.993971854415));
#55685=CARTESIAN_POINT('Ctrl Pts',(53.646552220384,26.955555365559,13.998189427066));
#55686=CARTESIAN_POINT('Ctrl Pts',(53.7158731516393,26.9129042936848,14.0024069997171));
#55687=CARTESIAN_POINT('Ctrl Pts',(53.7853117590487,26.870180819233,14.0066317319334));
#55688=CARTESIAN_POINT('Ctrl Pts',(53.8568590323182,26.8309422815005,14.0108564641496));
#55689=CARTESIAN_POINT('Ctrl Pts',(53.9301268787407,26.7953862573215,14.0150811963659));
#55690=CARTESIAN_POINT('Ctrl Pts',(54.0033764257502,26.7598391136324,14.019304873411));
#55691=CARTESIAN_POINT('Ctrl Pts',(54.0783452492387,26.7279728070302,14.0235285504562));
#55692=CARTESIAN_POINT('Ctrl Pts',(54.1546259781385,26.6999363023686,14.0277522275013));
#55693=CARTESIAN_POINT('Ctrl Pts',(54.2310451070274,26.671848929657,14.0319835677775));
#55694=CARTESIAN_POINT('Ctrl Pts',(54.3087804534193,26.6476053841441,14.0362149080538));
#55695=CARTESIAN_POINT('Ctrl Pts',(54.3874094661352,26.6273046786789,14.04044624833));
#55696=CARTESIAN_POINT('Ctrl Pts',(54.4658124976416,26.6070623178096,14.0446654276575));
#55697=CARTESIAN_POINT('Ctrl Pts',(54.5451036028337,26.5907401739851,14.048884606985));
#55698=CARTESIAN_POINT('Ctrl Pts',(54.6248578754318,26.5783851180722,14.0531037863125));
#55699=CARTESIAN_POINT('Ctrl Pts',(54.704866104102,26.5659907208002,14.057336400484));
#55700=CARTESIAN_POINT('Ctrl Pts',(54.7856380316746,26.5575426447949,14.0615690146555));
#55701=CARTESIAN_POINT('Ctrl Pts',(54.8667504494212,26.5531255023458,14.065801628827));
#55702=CARTESIAN_POINT('Ctrl Pts',(54.94774716792,26.5487146605357,14.0700282055718));
#55703=CARTESIAN_POINT('Ctrl Pts',(55.0290829519683,26.5483233575919,14.0742547823165));
#55704=CARTESIAN_POINT('Ctrl Pts',(55.1103265405908,26.5519848234863,14.0784813590613));
#55705=CARTESIAN_POINT('Ctrl Pts',(55.1914799582377,26.5556422255776,14.0827032447954));
#55706=CARTESIAN_POINT('Ctrl Pts',(55.2725409220424,26.5633434379741,14.0869251305294));
#55707=CARTESIAN_POINT('Ctrl Pts',(55.3530766352391,26.5750696629288,14.0911470162634));
#55708=CARTESIAN_POINT('Ctrl Pts',(55.4335580295948,26.5867879789085,14.0953660544664));
#55709=CARTESIAN_POINT('Ctrl Pts',(55.5135144184293,26.6025258489624,14.0995850926695));
#55710=CARTESIAN_POINT('Ctrl Pts',(55.5925178611087,26.6222126179435,14.1038041308725));
#55711=CARTESIAN_POINT('Ctrl Pts',(55.6714955041441,26.6418929579435,14.1080217912915));
#55712=CARTESIAN_POINT('Ctrl Pts',(55.7495203686247,26.6655195236315,14.1122394517104));
#55713=CARTESIAN_POINT('Ctrl Pts',(55.8261758034848,26.6929707865447,14.1164571121294));
#55714=CARTESIAN_POINT('Ctrl Pts',(55.9028296431743,26.7204214782075,14.1206746847804));
#55715=CARTESIAN_POINT('Ctrl Pts',(55.9781136729493,26.7516965511231,14.1248922574315));
#55716=CARTESIAN_POINT('Ctrl Pts',(56.0516288388797,26.7866254191311,14.1291098300825));
#55717=CARTESIAN_POINT('Ctrl Pts',(56.1252688009121,26.8216135808443,14.1333345622988));
#55718=CARTESIAN_POINT('Ctrl Pts',(56.1971334695029,26.8602677470368,14.1375592945151));
#55719=CARTESIAN_POINT('Ctrl Pts',(56.2668458342363,26.9023699367434,14.1417840267314));
#55720=CARTESIAN_POINT('Ctrl Pts',(56.3365407875756,26.9444616109865,14.1460077037765));
#55721=CARTESIAN_POINT('Ctrl Pts',(56.4040841374098,26.9899993083908,14.1502313808216));
#55722=CARTESIAN_POINT('Ctrl Pts',(56.4691291551239,27.0387224124146,14.1544550578667));
#55723=CARTESIAN_POINT('Ctrl Pts',(56.5342921873072,27.087533917233,14.158686398143));
#55724=CARTESIAN_POINT('Ctrl Pts',(56.5969474701362,27.139542081124,14.1629177384192));
#55725=CARTESIAN_POINT('Ctrl Pts',(56.656781911933,27.1944463601733,14.1671490786954));
#55726=CARTESIAN_POINT('Ctrl Pts',(56.7164443884584,27.2491928433284,14.171368258023));
#55727=CARTESIAN_POINT('Ctrl Pts',(56.7733019560602,27.3068184344149,14.1755874373505));
#55728=CARTESIAN_POINT('Ctrl Pts',(56.8270839789517,27.3669922278636,14.179806616678));
#55729=CARTESIAN_POINT('Ctrl Pts',(56.8810372562578,27.4273576286044,14.1840392308495));
#55730=CARTESIAN_POINT('Ctrl Pts',(56.9320960180283,27.4905120197301,14.1882718450209));
#55731=CARTESIAN_POINT('Ctrl Pts',(56.979958894167,27.5561464660815,14.1925044591924));
#55732=CARTESIAN_POINT('Ctrl Pts',(57.027753498407,27.6216872910579,14.1967310359372));
#55733=CARTESIAN_POINT('Ctrl Pts',(57.0723609996019,27.6897007729706,14.200957612682));
#55734=CARTESIAN_POINT('Ctrl Pts',(57.1135187447903,27.7598432496575,14.2051841894268));
#55735=CARTESIAN_POINT('Ctrl Pts',(57.1546308096475,27.8299078763175,14.2094060751608));
#55736=CARTESIAN_POINT('Ctrl Pts',(57.1923004924596,27.9020964039528,14.2136279608948));
#55737=CARTESIAN_POINT('Ctrl Pts',(57.2263079463427,27.9760355582094,14.2178498466288));
#55738=CARTESIAN_POINT('Ctrl Pts',(57.2602924632527,28.0499248427994,14.2220688848319));
#55739=CARTESIAN_POINT('Ctrl Pts',(57.2906194633733,28.1255619879926,14.2262879230349));
#55740=CARTESIAN_POINT('Ctrl Pts',(57.3171152427982,28.2025495616703,14.2305069612379));
#55741=CARTESIAN_POINT('Ctrl Pts',(57.3436023696675,28.2795119940132,14.2347246216569));
#55742=CARTESIAN_POINT('Ctrl Pts',(57.3662606094634,28.3578235401146,14.2389422820758));
#55743=CARTESIAN_POINT('Ctrl Pts',(57.38496507815,28.4370685423562,14.2431599424948));
#55744=CARTESIAN_POINT('Ctrl Pts',(57.4036691576036,28.5163118955392,14.2473775151458));
#55745=CARTESIAN_POINT('Ctrl Pts',(57.4184195239614,28.5964882138468,14.2515950877969));
#55746=CARTESIAN_POINT('Ctrl Pts',(57.4291420239166,28.6771698935318,14.2558126604479));
#55747=CARTESIAN_POINT('Ctrl Pts',(57.4398827259147,28.7579885348765,14.2600373926642));
#55748=CARTESIAN_POINT('Ctrl Pts',(57.4465818196907,28.8393137910905,14.2642621248805));
#55749=CARTESIAN_POINT('Ctrl Pts',(57.4492169084032,28.9207107473131,14.2684868570968));
#55750=CARTESIAN_POINT('Ctrl Pts',(57.4518513389747,29.0020873737922,14.2727105341419));
#55751=CARTESIAN_POINT('Ctrl Pts',(57.4504238237014,29.0835351987591,14.276934211187));
#55752=CARTESIAN_POINT('Ctrl Pts',(57.4449642149757,29.1646214976492,14.2811578882321));
#55753=CARTESIAN_POINT('Ctrl Pts',(57.4394947006054,29.2458549155171,14.2853892285084));
#55754=CARTESIAN_POINT('Ctrl Pts',(57.4299785271914,29.3267250337392,14.2896205687846));
#55755=CARTESIAN_POINT('Ctrl Pts',(57.4164973511887,29.4068056067681,14.2938519090608));
#55756=CARTESIAN_POINT('Ctrl Pts',(57.4030549203305,29.4866560267772,14.2980710883884));
#55757=CARTESIAN_POINT('Ctrl Pts',(57.3856704264274,29.5657210070998,14.3022902677159));
#55758=CARTESIAN_POINT('Ctrl Pts',(57.3644741070784,29.6435933863519,14.3065094470434));
#55759=CARTESIAN_POINT('Ctrl Pts',(57.3432102937403,29.7217137292916,14.3107420612149));
#55760=CARTESIAN_POINT('Ctrl Pts',(57.3180312283172,29.798924408193,14.3149746753864));
#55761=CARTESIAN_POINT('Ctrl Pts',(57.2890319872906,29.874804441667,14.3192072895578));
#55762=CARTESIAN_POINT('Ctrl Pts',(57.2600741109585,29.950576239398,14.3234338663026));
#55763=CARTESIAN_POINT('Ctrl Pts',(57.2273070461421,30.0250207311223,14.3276604430474));
#55764=CARTESIAN_POINT('Ctrl Pts',(57.1908760768488,30.0977305069513,14.3318870197922));
#55765=CARTESIAN_POINT('Ctrl Pts',(57.1544855417128,30.1703595833488,14.3361089055262));
#55766=CARTESIAN_POINT('Ctrl Pts',(57.1144393892975,30.2412573562478,14.3403307912603));
#55767=CARTESIAN_POINT('Ctrl Pts',(57.0709310467267,30.3100362016767,14.3445526769943));
#55768=CARTESIAN_POINT('Ctrl Pts',(57.0274520491837,30.3787686579073,14.3487717151973));
#55769=CARTESIAN_POINT('Ctrl Pts',(56.9805157469836,30.445384633507,14.3529907534004));
#55770=CARTESIAN_POINT('Ctrl Pts',(56.9303609516672,30.5095220588909,14.3572097916034));
#55771=CARTESIAN_POINT('Ctrl Pts',(56.8802225350784,30.5736385393302,14.3614274520224));
#55772=CARTESIAN_POINT('Ctrl Pts',(56.8268679986246,30.6352777113171,14.3656451124413));
#55773=CARTESIAN_POINT('Ctrl Pts',(56.7705780194319,30.6941085346295,14.3698627728603));
#55774=CARTESIAN_POINT('Ctrl Pts',(56.7142892116124,30.7529381336947,14.3740803455114));
#55775=CARTESIAN_POINT('Ctrl Pts',(56.655065404513,30.8089591654391,14.3782979181624));
#55776=CARTESIAN_POINT('Ctrl Pts',(56.5932249138242,30.8618766403739,14.3825154908135));
#55777=CARTESIAN_POINT('Ctrl Pts',(56.531279445447,30.9148839456791,14.3867402230297));
#55778=CARTESIAN_POINT('Ctrl Pts',(56.4667087609621,30.9647768495918,14.390964955246));
#55779=CARTESIAN_POINT('Ctrl Pts',(56.399865485068,31.0112997970753,14.3951896874623));
#55780=CARTESIAN_POINT('Ctrl Pts',(56.333038903983,31.0578111249649,14.3994133645074));
#55781=CARTESIAN_POINT('Ctrl Pts',(56.2639412732173,31.1009539507217,14.4036370415525));
#55782=CARTESIAN_POINT('Ctrl Pts',(56.1929518247189,31.1405177396836,14.4078607185977));
#55783=CARTESIAN_POINT('Ctrl Pts',(56.1218335764694,31.1801533112311,14.4120920588739));
#55784=CARTESIAN_POINT('Ctrl Pts',(56.0488170686819,31.2161966624658,14.4163233991501));
#55785=CARTESIAN_POINT('Ctrl Pts',(55.9743043007145,31.2484842404627,14.4205547394264));
#55786=CARTESIAN_POINT('Ctrl Pts',(55.9000056837946,31.2806790233745,14.4247739187539));
#55787=CARTESIAN_POINT('Ctrl Pts',(55.8242198511984,31.3091395103577,14.4289930980814));
#55788=CARTESIAN_POINT('Ctrl Pts',(55.7473592416202,31.33375328901,14.4332122774089));
#55789=CARTESIAN_POINT('Ctrl Pts',(55.6702538900632,31.3584454436331,14.4374448915804));
#55790=CARTESIAN_POINT('Ctrl Pts',(55.591780121258,31.3793581641997,14.4416775057518));
#55791=CARTESIAN_POINT('Ctrl Pts',(55.5123428247275,31.3963420206536,14.4459101199233));
#55792=CARTESIAN_POINT('Ctrl Pts',(55.4330188380417,31.413301651231,14.4501366966681));
#55793=CARTESIAN_POINT('Ctrl Pts',(55.3527345038368,31.4263434519515,14.4543632734129));
#55794=CARTESIAN_POINT('Ctrl Pts',(55.2719106605359,31.4353674964339,14.4585898501577));
#55795=CARTESIAN_POINT('Ctrl Pts',(55.1911765223419,31.444381525272,14.4628117358917));
#55796=CARTESIAN_POINT('Ctrl Pts',(55.1099045242043,31.449386607094,14.4670336216257));
#55797=CARTESIAN_POINT('Ctrl Pts',(55.0285251167716,31.4503339706483,14.4712555073598));
#55798=CARTESIAN_POINT('Ctrl Pts',(54.9472005972257,31.4512806952354,14.4754745455628));
#55799=CARTESIAN_POINT('Ctrl Pts',(54.8657692755834,31.4481751316952,14.4796935837658));
#55800=CARTESIAN_POINT('Ctrl Pts',(54.784664874142,31.4410204901991,14.4839126219688));
#55801=CARTESIAN_POINT('Ctrl Pts',(54.7035869584412,31.433868185148,14.4881302823878));
#55802=CARTESIAN_POINT('Ctrl Pts',(54.6228362133186,31.422669468901,14.4923479428067));
#55803=CARTESIAN_POINT('Ctrl Pts',(54.5428431245178,31.4074795619484,14.4965656032257));
#55804=CARTESIAN_POINT('Ctrl Pts',(54.462851700343,31.392289971092,14.5007831758767));
#55805=CARTESIAN_POINT('Ctrl Pts',(54.3836183573154,31.3731094424833,14.5050007485278));
#55806=CARTESIAN_POINT('Ctrl Pts',(54.3055638313786,31.3500443948382,14.5092183211788));
#55807=CARTESIAN_POINT('Ctrl Pts',(54.2273768035225,31.3269401929859,14.5134430533951));
#55808=CARTESIAN_POINT('Ctrl Pts',(54.1503730443571,31.2999384110058,14.5176677856114));
#55809=CARTESIAN_POINT('Ctrl Pts',(54.0749588890643,31.269195715023,14.5218925178277));
#55810=CARTESIAN_POINT('Ctrl Pts',(53.9995635692477,31.238460697351,14.5261161948728));
#55811=CARTESIAN_POINT('Ctrl Pts',(53.9257574727214,31.2039868506371,14.5303398719179));
#55812=CARTESIAN_POINT('Ctrl Pts',(53.8539236554495,31.1659776689665,14.534563548963));
#55813=CARTESIAN_POINT('Ctrl Pts',(53.7819595064455,31.127899525313,14.5387948892393));
#55814=CARTESIAN_POINT('Ctrl Pts',(53.7119751884393,31.0862734660363,14.5430262295155));
#55815=CARTESIAN_POINT('Ctrl Pts',(53.6443267425252,31.0413476599951,14.5472575697917));
#55816=CARTESIAN_POINT('Ctrl Pts',(53.5768727194719,30.9965509715356,14.5514767491192));
#55817=CARTESIAN_POINT('Ctrl Pts',(53.5117414766369,30.9484738153338,14.5556959284468));
#55818=CARTESIAN_POINT('Ctrl Pts',(53.4492518403369,30.8974009579689,14.5599151077743));
#55819=CARTESIAN_POINT('Ctrl Pts',(53.3873827660839,30.8468352867359,14.5640923879531));
#55820=CARTESIAN_POINT('Ctrl Pts',(53.3278597894437,30.7931340933857,14.568269668132));
#55821=CARTESIAN_POINT('Ctrl Pts',(53.2710240049294,30.7365460715079,14.5724469483109));
#55822=CARTESIAN_POINT('Ctrl Pts',(53.2142047566346,30.6799745137638,14.5766230131212));
#55823=CARTESIAN_POINT('Ctrl Pts',(53.1600715331763,30.6205180773484,14.5807990779316));
#55824=CARTESIAN_POINT('Ctrl Pts',(53.1089340860591,30.5584671825646,14.584975142742));
#55825=CARTESIAN_POINT('Ctrl Pts',(53.0579134800667,30.4965580644386,14.5891416658928));
#55826=CARTESIAN_POINT('Ctrl Pts',(53.0098753147622,30.4320666680182,14.5933081890436));
#55827=CARTESIAN_POINT('Ctrl Pts',(52.9650908239207,30.3653186057138,14.5974747121944));
#55828=CARTESIAN_POINT('Ctrl Pts',(52.92033330881,30.298610748796,14.6016387256593));
#55829=CARTESIAN_POINT('Ctrl Pts',(52.8788258453699,30.2296493187588,14.6058027391242));
#55830=CARTESIAN_POINT('Ctrl Pts',(52.8407980088952,30.1587911855072,14.6099667525891));
#55831=CARTESIAN_POINT('Ctrl Pts',(52.8027807185668,30.0879527031299,14.6141296112606));
#55832=CARTESIAN_POINT('Ctrl Pts',(52.7682413646764,30.0152189829851,14.6182924699321));
#55833=CARTESIAN_POINT('Ctrl Pts',(52.7373641541067,29.9409725176001,14.6224553286035));
#55834=CARTESIAN_POINT('Ctrl Pts',(52.7063244605155,29.866335350147,14.6266400931999));
#55835=CARTESIAN_POINT('Ctrl Pts',(52.6789857771242,29.7901699093691,14.6308248577962));
#55836=CARTESIAN_POINT('Ctrl Pts',(52.655486019538,29.7128845947404,14.6350096223926));
#55837=CARTESIAN_POINT('Ctrl Pts',(52.6320877087135,29.6359329152514,14.6391763216614));
#55838=CARTESIAN_POINT('Ctrl Pts',(52.6124953239584,29.5578714887528,14.6433430209302));
#55839=CARTESIAN_POINT('Ctrl Pts',(52.5967942336395,29.4791161597482,14.6475097201991));
#55840=CARTESIAN_POINT('Ctrl Pts',(52.5809910317977,29.399848648059,14.6517035174591));
#55841=CARTESIAN_POINT('Ctrl Pts',(52.5691299991165,29.3198786600043,14.6558973147192));
#55842=CARTESIAN_POINT('Ctrl Pts',(52.5612452194669,29.2396359122226,14.6600911119793));
#55843=CARTESIAN_POINT('Ctrl Pts',(52.5533604398173,29.1593931644409,14.6642849092394));
#55844=CARTESIAN_POINT('Ctrl Pts',(52.5494518791718,29.07887814682,14.6684787064995));
#55845=CARTESIAN_POINT('Ctrl Pts',(52.5495004475699,28.9985189396232,14.6726725037596));
#55846=CARTESIAN_POINT('',(52.5495009444406,29.0021514419089,15.4726725038256));
#55847=CARTESIAN_POINT('Ctrl Pts',(52.5495004475702,28.9985189390796,14.672672503788));
#55848=CARTESIAN_POINT('Ctrl Pts',(52.5495542816505,28.9094473905506,14.6773209819052));
#55849=CARTESIAN_POINT('Ctrl Pts',(52.5544642569436,28.8205244575737,14.6819694600225));
#55850=CARTESIAN_POINT('Ctrl Pts',(52.5641836615108,28.7321399336424,14.6866179381398));
#55851=CARTESIAN_POINT('Ctrl Pts',(52.5730335449504,28.6516625001486,14.6908505523113));
#55852=CARTESIAN_POINT('Ctrl Pts',(52.5858925348933,28.5714744670663,14.6950831664828));
#55853=CARTESIAN_POINT('Ctrl Pts',(52.6027322144458,28.4920064819864,14.6993157806543));
#55854=CARTESIAN_POINT('Ctrl Pts',(52.6195478737765,28.4126518505255,14.703542357399));
#55855=CARTESIAN_POINT('Ctrl Pts',(52.6403328498171,28.334015677833,14.7077689341438));
#55856=CARTESIAN_POINT('Ctrl Pts',(52.6650070179837,28.2565230172126,14.7119955108886));
#55857=CARTESIAN_POINT('Ctrl Pts',(52.6896538006809,28.179116364472,14.7162173966227));
#55858=CARTESIAN_POINT('Ctrl Pts',(52.7181810582898,28.1028511423937,14.7204392823567));
#55859=CARTESIAN_POINT('Ctrl Pts',(52.7504580308852,28.028140350055,14.7246611680907));
#55860=CARTESIAN_POINT('Ctrl Pts',(52.7827132336635,27.9534799478291,14.7288802062937));
#55861=CARTESIAN_POINT('Ctrl Pts',(52.8187129447186,27.8803723184514,14.7330992444967));
#55862=CARTESIAN_POINT('Ctrl Pts',(52.8582775963539,27.8092122793209,14.7373182826997));
#55863=CARTESIAN_POINT('Ctrl Pts',(52.8978293276164,27.7380754784647,14.7415359431187));
#55864=CARTESIAN_POINT('Ctrl Pts',(52.9409434619016,27.6688854104762,14.7457536035377));
#55865=CARTESIAN_POINT('Ctrl Pts',(52.9873942478509,27.602012755274,14.7499712639566));
#55866=CARTESIAN_POINT('Ctrl Pts',(53.033844067177,27.5351414916665,14.7541888366076));
#55867=CARTESIAN_POINT('Ctrl Pts',(53.083630134129,27.4705879258279,14.7584064092587));
#55868=CARTESIAN_POINT('Ctrl Pts',(53.1364839079387,27.4086929822852,14.7626239819097));
#55869=CARTESIAN_POINT('Ctrl Pts',(53.1894274039829,27.3466929686171,14.766848714126));
#55870=CARTESIAN_POINT('Ctrl Pts',(53.2454487228273,27.2873609621562,14.7710734463423));
#55871=CARTESIAN_POINT('Ctrl Pts',(53.3042392968181,27.2310042714738,14.7752981785586));
#55872=CARTESIAN_POINT('Ctrl Pts',(53.3630151872463,27.1746616564661,14.7795218556036));
#55873=CARTESIAN_POINT('Ctrl Pts',(53.4245585835907,27.1212931605337,14.7837455326487));
#55874=CARTESIAN_POINT('Ctrl Pts',(53.488527630144,27.0711657600608,14.7879692096938));
#55875=CARTESIAN_POINT('Ctrl Pts',(53.5526127389776,27.020947410907,14.7922005499701));
#55876=CARTESIAN_POINT('Ctrl Pts',(53.6191319126329,26.9739821778735,14.7964318902463));
#55877=CARTESIAN_POINT('Ctrl Pts',(53.68771349525,26.9304941702303,14.8006632305225));
#55878=CARTESIAN_POINT('Ctrl Pts',(53.7560979731549,26.8871311479096,14.80488240985));
#55879=CARTESIAN_POINT('Ctrl Pts',(53.8265325839536,26.847225542496,14.8091015891776));
#55880=CARTESIAN_POINT('Ctrl Pts',(53.8986274024896,26.8109525698484,14.8133207685051));
#55881=CARTESIAN_POINT('Ctrl Pts',(53.9709517876213,26.774564095657,14.8175533826766));
#55882=CARTESIAN_POINT('Ctrl Pts',(54.0452159771998,26.7416961109572,14.8217859968481));
#55883=CARTESIAN_POINT('Ctrl Pts',(54.121043262982,26.7125592238376,14.8260186110196));
#55884=CARTESIAN_POINT('Ctrl Pts',(54.1967623882608,26.6834638977515,14.8302451877643));
#55885=CARTESIAN_POINT('Ctrl Pts',(54.274039751417,26.65808926419,14.8344717645091));
#55886=CARTESIAN_POINT('Ctrl Pts',(54.3524751871284,26.6365995119922,14.8386983412539));
#55887=CARTESIAN_POINT('Ctrl Pts',(54.4308235685887,26.6151336109309,14.842920226988));
#55888=CARTESIAN_POINT('Ctrl Pts',(54.5103270228847,26.5975441458926,14.847142112722));
#55889=CARTESIAN_POINT('Ctrl Pts',(54.5905679301628,26.5839462691842,14.851363998456));
#55890=CARTESIAN_POINT('Ctrl Pts',(54.6707547174373,26.570357563822,14.855583036659));
#55891=CARTESIAN_POINT('Ctrl Pts',(54.7516775129992,26.5607551772571,14.8598020748621));
#55892=CARTESIAN_POINT('Ctrl Pts',(54.8329073772553,26.555203422486,14.8640211130651));
#55893=CARTESIAN_POINT('Ctrl Pts',(54.9141107147993,26.5496534807155,14.8682387734841));
#55894=CARTESIAN_POINT('Ctrl Pts',(54.9956204587805,26.5481515754134,14.872456433903));
#55895=CARTESIAN_POINT('Ctrl Pts',(55.0770027743105,26.5507101390916,14.876674094322));
#55896=CARTESIAN_POINT('Ctrl Pts',(55.1583833963052,26.5532686495271,14.8808916669731));
#55897=CARTESIAN_POINT('Ctrl Pts',(55.2396361308393,26.5598874451701,14.8851092396241));
#55898=CARTESIAN_POINT('Ctrl Pts',(55.3203288080082,26.5705268668372,14.8893268122752));
#55899=CARTESIAN_POINT('Ctrl Pts',(55.4011584655055,26.581184349517,14.8935515444915));
#55900=CARTESIAN_POINT('Ctrl Pts',(55.4814257004644,26.5958760528818,14.8977762767078));
#55901=CARTESIAN_POINT('Ctrl Pts',(55.5607047502234,26.6145104416332,14.9020010089241));
#55902=CARTESIAN_POINT('Ctrl Pts',(55.6399639992082,26.6331401762506,14.9062246859692));
#55903=CARTESIAN_POINT('Ctrl Pts',(55.7182351145354,26.6557104774701,14.9104483630143));
#55904=CARTESIAN_POINT('Ctrl Pts',(55.7951080431562,26.682079930259,14.9146720400594));
#55905=CARTESIAN_POINT('Ctrl Pts',(55.872120446224,26.7084972264813,14.9189033803357));
#55906=CARTESIAN_POINT('Ctrl Pts',(55.9477291602737,26.73872727672,14.9231347206119));
#55907=CARTESIAN_POINT('Ctrl Pts',(56.0215438670464,26.7725803319311,14.9273660608881));
#55908=CARTESIAN_POINT('Ctrl Pts',(56.0951464290126,26.8063360928474,14.9315852402157));
#55909=CARTESIAN_POINT('Ctrl Pts',(56.1669649164557,26.8436937775061,14.9358044195432));
#55910=CARTESIAN_POINT('Ctrl Pts',(56.2366400783236,26.8844216945044,14.9400235988707));
#55911=CARTESIAN_POINT('Ctrl Pts',(56.3065371020408,26.9252792986212,14.9442562130422));
#55912=CARTESIAN_POINT('Ctrl Pts',(56.3745370814643,26.969680616962,14.9484888272137));
#55913=CARTESIAN_POINT('Ctrl Pts',(56.4402582729453,27.0174243123621,14.9527214413852));
#55914=CARTESIAN_POINT('Ctrl Pts',(56.5058857193175,27.0650999058637,14.95694801813));
#55915=CARTESIAN_POINT('Ctrl Pts',(56.5692404608935,27.1161081366173,14.9611745948748));
#55916=CARTESIAN_POINT('Ctrl Pts',(56.6299669216089,27.170202720392,14.9654011716195));
#55917=CARTESIAN_POINT('Ctrl Pts',(56.6906259829848,27.2242372654426,14.9696230573536));
#55918=CARTESIAN_POINT('Ctrl Pts',(56.748662214615,27.2813510496237,14.9738449430876));
#55919=CARTESIAN_POINT('Ctrl Pts',(56.8037516712548,27.3412564518752,14.9780668288216));
#55920=CARTESIAN_POINT('Ctrl Pts',(56.8588039717645,27.4011214497907,14.9822858670246));
#55921=CARTESIAN_POINT('Ctrl Pts',(56.9109131310076,27.4637739851927,14.9865049052277));
#55922=CARTESIAN_POINT('Ctrl Pts',(56.9597916865599,27.5288892647762,14.9907239434307));
#55923=CARTESIAN_POINT('Ctrl Pts',(57.008654280158,27.5939832800834,14.9949416038497));
#55924=CARTESIAN_POINT('Ctrl Pts',(57.0542880865565,27.6615380711573,14.9991592642686));
#55925=CARTESIAN_POINT('Ctrl Pts',(57.0964464969875,27.7311964946182,15.0033769246876));
#55926=CARTESIAN_POINT('Ctrl Pts',(57.1386040301179,27.8008534685137,15.0075944973386));
#55927=CARTESIAN_POINT('Ctrl Pts',(57.1772860715491,27.8726135897216,15.0118120699897));
#55928=CARTESIAN_POINT('Ctrl Pts',(57.2122906147601,27.9460927527319,15.0160296426407));
#55929=CARTESIAN_POINT('Ctrl Pts',(57.2473545801392,28.0196966507271,15.020254374857));
#55930=CARTESIAN_POINT('Ctrl Pts',(57.2787283561513,28.095025007502,15.0244791070733));
#55931=CARTESIAN_POINT('Ctrl Pts',(57.3062569393779,28.1716708507053,15.0287038392896));
#55932=CARTESIAN_POINT('Ctrl Pts',(57.3337786470522,28.2482975508056,15.0329275163347));
#55933=CARTESIAN_POINT('Ctrl Pts',(57.3574569672904,28.3262406271011,15.0371511933798));
#55934=CARTESIAN_POINT('Ctrl Pts',(57.3771872893792,28.4050791302922,15.0413748704249));
#55935=CARTESIAN_POINT('Ctrl Pts',(57.3969534091905,28.4840606741717,15.0456062107011));
#55936=CARTESIAN_POINT('Ctrl Pts',(57.4127571253136,28.5639404346521,15.0498375509774));
#55937=CARTESIAN_POINT('Ctrl Pts',(57.4245451144589,28.6442877033983,15.0540688912536));
#55938=CARTESIAN_POINT('Ctrl Pts',(57.4362992247094,28.7244040526358,15.0582880705811));
#55939=CARTESIAN_POINT('Ctrl Pts',(57.4440606988487,28.8049847653453,15.0625072499086));
#55940=CARTESIAN_POINT('Ctrl Pts',(57.4478283089082,28.8856023596947,15.0667264292361));
#55941=CARTESIAN_POINT('Ctrl Pts',(57.4516079159106,28.9664766591326,15.0709590434076));
#55942=CARTESIAN_POINT('Ctrl Pts',(57.4513822135804,29.0476888708402,15.075191657579));
#55943=CARTESIAN_POINT('Ctrl Pts',(57.4471122670599,29.1288091704997,15.0794242717505));
#55944=CARTESIAN_POINT('Ctrl Pts',(57.4428484112173,29.2098137596685,15.0836508484953));
#55945=CARTESIAN_POINT('Ctrl Pts',(57.4345517928504,29.2907262371267,15.0878774252401));
#55946=CARTESIAN_POINT('Ctrl Pts',(57.4222354254891,29.3711142593674,15.0921040019849));
#55947=CARTESIAN_POINT('Ctrl Pts',(57.4099327278693,29.4514130602122,15.0963258877189));
#55948=CARTESIAN_POINT('Ctrl Pts',(57.3936192161576,29.5311881055644,15.1005477734529));
#55949=CARTESIAN_POINT('Ctrl Pts',(57.3733597981023,29.6100110808436,15.104769659187));
#55950=CARTESIAN_POINT('Ctrl Pts',(57.3531140443962,29.6887808924702,15.10898869739));
#55951=CARTESIAN_POINT('Ctrl Pts',(57.3289277854457,29.7665994606097,15.113207735593));
#55952=CARTESIAN_POINT('Ctrl Pts',(57.300916971293,29.8430488367917,15.117426773796));
#55953=CARTESIAN_POINT('Ctrl Pts',(57.272915304451,29.9194732473946,15.121644434215));
#55954=CARTESIAN_POINT('Ctrl Pts',(57.2410917224622,29.994528918152,15.125862094634));
#55955=CARTESIAN_POINT('Ctrl Pts',(57.2056115521912,30.0678145582642,15.130079755053));
#55956=CARTESIAN_POINT('Ctrl Pts',(57.1701321202491,30.1410986733299,15.134297327704));
#55957=CARTESIAN_POINT('Ctrl Pts',(57.1309964548012,30.2126124133733,15.1385149003551));
#55958=CARTESIAN_POINT('Ctrl Pts',(57.0884167807263,30.2819772228791,15.1427324730061));
#55959=CARTESIAN_POINT('Ctrl Pts',(57.0457648252755,30.3514597830249,15.1469572052224));
#55960=CARTESIAN_POINT('Ctrl Pts',(56.9996574082299,30.418785715986,15.1511819374387));
#55961=CARTESIAN_POINT('Ctrl Pts',(56.9503515242788,30.4836034449081,15.155406669655));
#55962=CARTESIAN_POINT('Ctrl Pts',(56.9010579549893,30.5484049849227,15.1596303467001));
#55963=CARTESIAN_POINT('Ctrl Pts',(56.8485678329195,30.6106992308592,15.1638540237452));
#55964=CARTESIAN_POINT('Ctrl Pts',(56.7931773108047,30.6701692674741,15.1680777007903));
#55965=CARTESIAN_POINT('Ctrl Pts',(56.737686290861,30.7297472035878,15.1723090410666));
#55966=CARTESIAN_POINT('Ctrl Pts',(56.6792846884101,30.7864903653685,15.1765403813428));
#55967=CARTESIAN_POINT('Ctrl Pts',(56.6183047632273,30.8401195459306,15.1807717216191));
#55968=CARTESIAN_POINT('Ctrl Pts',(56.557500095456,30.8935945952547,15.1849909009466));
#55969=CARTESIAN_POINT('Ctrl Pts',(56.4941323135716,30.9439733205334,15.1892100802741));
#55970=CARTESIAN_POINT('Ctrl Pts',(56.428559331612,30.9910219702615,15.1934292596016));
#55971=CARTESIAN_POINT('Ctrl Pts',(56.3627775500939,31.038220433785,15.1976618737731));
#55972=CARTESIAN_POINT('Ctrl Pts',(56.2945318256093,31.0822431025086,15.2018944879445));
#55973=CARTESIAN_POINT('Ctrl Pts',(56.2241615094716,31.1228233201866,15.206127102116));
#55974=CARTESIAN_POINT('Ctrl Pts',(56.1538915699823,31.1633456539945,15.2103536788608));
#55975=CARTESIAN_POINT('Ctrl Pts',(56.0815034569499,31.2004350591713,15.2145802556056));
#55976=CARTESIAN_POINT('Ctrl Pts',(56.0073669155911,31.2338670836405,15.2188068323504));
#55977=CARTESIAN_POINT('Ctrl Pts',(55.9333126572084,31.2672620024339,15.2230287180844));
#55978=CARTESIAN_POINT('Ctrl Pts',(55.8575142477203,31.297007416272,15.2272506038184));
#55979=CARTESIAN_POINT('Ctrl Pts',(55.780366304033,31.3229245966088,15.2314724895525));
#55980=CARTESIAN_POINT('Ctrl Pts',(55.7032703942412,31.3488242966111,15.2356915277555));
#55981=CARTESIAN_POINT('Ctrl Pts',(55.6248271972518,31.3709007436843,15.2399105659585));
#55982=CARTESIAN_POINT('Ctrl Pts',(55.5454504220818,31.3890236681646,15.2441296041615));
#55983=CARTESIAN_POINT('Ctrl Pts',(55.4660995684727,31.4071406743586,15.2483472645805));
#55984=CARTESIAN_POINT('Ctrl Pts',(55.3858161946883,31.4213066186349,15.2525649249995));
#55985=CARTESIAN_POINT('Ctrl Pts',(55.3050269176534,31.4314417183035,15.2567825854184));
#55986=CARTESIAN_POINT('Ctrl Pts',(55.2242393218128,31.4415766070646,15.2610001580695));
#55987=CARTESIAN_POINT('Ctrl Pts',(55.1429463047345,31.4476807613341,15.2652177307205));
#55988=CARTESIAN_POINT('Ctrl Pts',(55.0615809437297,31.4497261147666,15.2694353033715));
#55989=CARTESIAN_POINT('Ctrl Pts',(54.9800774604782,31.4517749403008,15.2736600355878));
#55990=CARTESIAN_POINT('Ctrl Pts',(54.8985018544371,31.4497511678989,15.2778847678041));
#55991=CARTESIAN_POINT('Ctrl Pts',(54.8172889452573,31.4436789724665,15.2821095000204));
#55992=CARTESIAN_POINT('Ctrl Pts',(54.7360963198532,31.4376082936285,15.2863331770655));
#55993=CARTESIAN_POINT('Ctrl Pts',(54.6552666700635,31.4274912927601,15.2905568541106));
#55994=CARTESIAN_POINT('Ctrl Pts',(54.5752270581772,31.4134038613326,15.2947805311557));
#55995=CARTESIAN_POINT('Ctrl Pts',(54.4950422263703,31.399290870365,15.299011871432));
#55996=CARTESIAN_POINT('Ctrl Pts',(54.4156507513243,31.3811931559315,15.3032432117082));
#55997=CARTESIAN_POINT('Ctrl Pts',(54.337467721308,31.35923742546,15.3074745519844));
#55998=CARTESIAN_POINT('Ctrl Pts',(54.2595093907386,31.3373447961562,15.311693731312));
#55999=CARTESIAN_POINT('Ctrl Pts',(54.1827529735009,31.3116165207669,15.3159129106395));
#56000=CARTESIAN_POINT('Ctrl Pts',(54.1075893949453,31.2822255721085,15.320132089967));
#56001=CARTESIAN_POINT('Ctrl Pts',(54.0321864781508,31.2527410358638,15.3243647041385));
#56002=CARTESIAN_POINT('Ctrl Pts',(53.9581061256139,31.2194607768503,15.32859731831));
#56003=CARTESIAN_POINT('Ctrl Pts',(53.8857567584493,31.1825242836355,15.3328299324814));
#56004=CARTESIAN_POINT('Ctrl Pts',(53.8135105908636,31.1456404768601,15.3370565092262));
#56005=CARTESIAN_POINT('Ctrl Pts',(53.7429909150328,31.105111003566,15.341283085971));
#56006=CARTESIAN_POINT('Ctrl Pts',(53.6745872966152,31.0611238234774,15.3455096627158));
#56007=CARTESIAN_POINT('Ctrl Pts',(53.6062595982932,31.0171854640652,15.3497315484498));
#56008=CARTESIAN_POINT('Ctrl Pts',(53.5400436795272,30.9697972732653,15.3539534341839));
#56009=CARTESIAN_POINT('Ctrl Pts',(53.4763042920924,30.9191929657291,15.3581753199179));
#56010=CARTESIAN_POINT('Ctrl Pts',(53.4126078948977,30.8686227892289,15.3623943581209));
#56011=CARTESIAN_POINT('Ctrl Pts',(53.3513850744741,30.8148410922616,15.366613396324));
#56012=CARTESIAN_POINT('Ctrl Pts',(53.2929703278242,30.7581239854775,15.370832434527));
#56013=CARTESIAN_POINT('Ctrl Pts',(53.2345746573009,30.7014254004328,15.375050094946));
#56014=CARTESIAN_POINT('Ctrl Pts',(53.178985572454,30.6417936326464,15.3792677553649));
#56015=CARTESIAN_POINT('Ctrl Pts',(53.1265022476143,30.5795431053965,15.3834854157839));
#56016=CARTESIAN_POINT('Ctrl Pts',(53.0740200149327,30.5172938735565,15.387702988435));
#56017=CARTESIAN_POINT('Ctrl Pts',(53.0246437122983,30.4524263465249,15.391920561086));
#56018=CARTESIAN_POINT('Ctrl Pts',(52.9786326501071,30.3852885211345,15.3961381337371));
#56019=CARTESIAN_POINT('Ctrl Pts',(52.932543481567,30.3180367255342,15.4003628659534));
#56020=CARTESIAN_POINT('Ctrl Pts',(52.889831247212,30.2485073059185,15.4045875981696));
#56021=CARTESIAN_POINT('Ctrl Pts',(52.8507123846899,30.1770781608181,15.4088123303859));
#56022=CARTESIAN_POINT('Ctrl Pts',(52.811603292514,30.1056668558956,15.413036007431));
#56023=CARTESIAN_POINT('Ctrl Pts',(52.7760859615526,30.0323572030995,15.4172596844762));
#56024=CARTESIAN_POINT('Ctrl Pts',(52.7443292251793,29.95754874843,15.4214833615213));
#56025=CARTESIAN_POINT('Ctrl Pts',(52.7125148709512,29.8826045649931,15.4257147017975));
#56026=CARTESIAN_POINT('Ctrl Pts',(52.6844749073509,29.8061565825541,15.4299460420738));
#56027=CARTESIAN_POINT('Ctrl Pts',(52.6603290233795,29.7286219672503,15.43417738235));
#56028=CARTESIAN_POINT('Ctrl Pts',(52.6362525351169,29.651310187838,15.4383965616775));
#56029=CARTESIAN_POINT('Ctrl Pts',(52.616047806141,29.572918474828,15.442615741005));
#56030=CARTESIAN_POINT('Ctrl Pts',(52.5997825625659,29.493868912807,15.4468349203325));
#56031=CARTESIAN_POINT('Ctrl Pts',(52.5767052804375,29.3817126431234,15.4528211320508));
#56032=CARTESIAN_POINT('Ctrl Pts',(52.5614830118809,29.2678893779456,15.4588073437692));
#56033=CARTESIAN_POINT('Ctrl Pts',(52.5543005723774,29.1533119686342,15.4647935554875));
#56034=CARTESIAN_POINT('Ctrl Pts',(52.551149438172,29.1030437006629,15.4674198715877));
#56035=CARTESIAN_POINT('Ctrl Pts',(52.5495452631465,29.0526305694615,15.4700461876878));
#56036=CARTESIAN_POINT('Ctrl Pts',(52.5495009444412,29.0021514426317,15.472672503788));
#56037=CARTESIAN_POINT('',(52.5495000114917,28.9997626798325,16.2726725038352));
#56038=CARTESIAN_POINT('Ctrl Pts',(52.5495009444406,29.0021514419089,15.4726725038256));
#56039=CARTESIAN_POINT('Ctrl Pts',(52.549430024194,28.9213730595116,15.4768752224453));
#56040=CARTESIAN_POINT('Ctrl Pts',(52.5533576597404,28.8404682849032,15.4810779410649));
#56041=CARTESIAN_POINT('Ctrl Pts',(52.5612936946831,28.7598712711745,15.4852806596846));
#56042=CARTESIAN_POINT('Ctrl Pts',(52.5691505346619,28.6800785479546,15.4894414387021));
#56043=CARTESIAN_POINT('Ctrl Pts',(52.5809360959679,28.6005879586768,15.4936022177195));
#56044=CARTESIAN_POINT('Ctrl Pts',(52.5966076728007,28.5218205655202,15.497762996737));
#56045=CARTESIAN_POINT('Ctrl Pts',(52.6122717977342,28.4430906265831,15.5019217972869));
#56046=CARTESIAN_POINT('Ctrl Pts',(52.6318181789659,28.3650836706248,15.5060805978368));
#56047=CARTESIAN_POINT('Ctrl Pts',(52.6551526313549,28.2882127651059,15.5102393983867));
#56048=CARTESIAN_POINT('Ctrl Pts',(52.6784836046501,28.2113533207985,15.5143975788724));
#56049=CARTESIAN_POINT('Ctrl Pts',(52.7056013878003,28.1356300487177,15.5185557593582));
#56050=CARTESIAN_POINT('Ctrl Pts',(52.7363617703766,28.0614414161132,15.5227139398439));
#56051=CARTESIAN_POINT('Ctrl Pts',(52.7676927790396,27.9858765337503,15.5269492574151));
#56052=CARTESIAN_POINT('Ctrl Pts',(52.8028027287989,27.9119042896829,15.5311845749863));
#56053=CARTESIAN_POINT('Ctrl Pts',(52.8414884899115,27.839923144436,15.5354198925574));
#56054=CARTESIAN_POINT('Ctrl Pts',(52.8795176709094,27.7691636731909,15.5395833277301));
#56055=CARTESIAN_POINT('Ctrl Pts',(52.9210019170919,27.7003286210923,15.5437467629028));
#56056=CARTESIAN_POINT('Ctrl Pts',(52.9657035541437,27.6337686065764,15.5479101980755));
#56057=CARTESIAN_POINT('Ctrl Pts',(53.0115628629572,27.5654848375327,15.5521814568459));
#56058=CARTESIAN_POINT('Ctrl Pts',(53.0608082015571,27.4995960132654,15.5564527156163));
#56059=CARTESIAN_POINT('Ctrl Pts',(53.113139302838,27.4364441297142,15.5607239743867));
#56060=CARTESIAN_POINT('Ctrl Pts',(53.1654704041189,27.373292246163,15.5649952331571));
#56061=CARTESIAN_POINT('Ctrl Pts',(53.2208868506974,27.3128776476264,15.5692664919275));
#56062=CARTESIAN_POINT('Ctrl Pts',(53.2790499887541,27.2554996965341,15.5735377506979));
#56063=CARTESIAN_POINT('Ctrl Pts',(53.3366868905738,27.1986408776289,15.5777703648694));
#56064=CARTESIAN_POINT('Ctrl Pts',(53.397251858526,27.1445358045864,15.5820029790409));
#56065=CARTESIAN_POINT('Ctrl Pts',(53.4604511639577,27.0935006867453,15.5862355932123));
#56066=CARTESIAN_POINT('Ctrl Pts',(53.5235603215144,27.0425383657077,15.5904621699571));
#56067=CARTESIAN_POINT('Ctrl Pts',(53.5892959949858,26.9946375920394,15.5946887467019));
#56068=CARTESIAN_POINT('Ctrl Pts',(53.6573278653092,26.9500776139754,15.5989153234467));
#56069=CARTESIAN_POINT('Ctrl Pts',(53.7252842281344,26.9055670923271,15.6031372091807));
#56070=CARTESIAN_POINT('Ctrl Pts',(53.7955313372712,26.8643902519524,15.6073590949148));
#56071=CARTESIAN_POINT('Ctrl Pts',(53.8677071906201,26.8267850442659,15.6115809806488));
#56072=CARTESIAN_POINT('Ctrl Pts',(53.9398343635942,26.7892052001257,15.6158000188518));
#56073=CARTESIAN_POINT('Ctrl Pts',(54.0138872862032,26.755192418376,15.6200190570549));
#56074=CARTESIAN_POINT('Ctrl Pts',(54.0894775569006,26.7249397523115,15.6242380952579));
#56075=CARTESIAN_POINT('Ctrl Pts',(54.1650431425715,26.6946969656648,15.6284557556768));
#56076=CARTESIAN_POINT('Ctrl Pts',(54.2421446483471,26.6682120286141,15.6326734160958));
#56077=CARTESIAN_POINT('Ctrl Pts',(54.3203730665648,26.6456301307251,15.6368910765148));
#56078=CARTESIAN_POINT('Ctrl Pts',(54.3985998568789,26.6230487027569,15.6411086491658));
#56079=CARTESIAN_POINT('Ctrl Pts',(54.4779530663593,26.604370280173,15.6453262218169));
#56080=CARTESIAN_POINT('Ctrl Pts',(54.5580092589447,26.5896899712233,15.649543794468));
#56081=CARTESIAN_POINT('Ctrl Pts',(54.6382013513901,26.574984741629,15.6537685266842));
#56082=CARTESIAN_POINT('Ctrl Pts',(54.7190983552261,26.5642912891443,15.6579932589005));
#56083=CARTESIAN_POINT('Ctrl Pts',(54.8002669849083,26.5576533880953,15.6622179911168));
#56084=CARTESIAN_POINT('Ctrl Pts',(54.881415341874,26.5510171449317,15.6664416681619));
#56085=CARTESIAN_POINT('Ctrl Pts',(54.9628347224271,26.5484344211631,15.670665345207));
#56086=CARTESIAN_POINT('Ctrl Pts',(55.0440914571839,26.5498966974016,15.6748890222522));
#56087=CARTESIAN_POINT('Ctrl Pts',(55.125495620149,26.551361626722,15.6791203625284));
#56088=CARTESIAN_POINT('Ctrl Pts',(55.2067360827534,26.5568861912774,15.6833517028047));
#56089=CARTESIAN_POINT('Ctrl Pts',(55.2873830972079,26.5664098115255,15.6875830430809));
#56090=CARTESIAN_POINT('Ctrl Pts',(55.3677983306794,26.5759060607162,15.6918022224084));
#56091=CARTESIAN_POINT('Ctrl Pts',(55.4476230875475,26.5893782517992,15.6960214017359));
#56092=CARTESIAN_POINT('Ctrl Pts',(55.5264442901062,26.6067163437205,15.7002405810634));
#56093=CARTESIAN_POINT('Ctrl Pts',(55.605516477626,26.6241096441414,15.7044731952349));
#56094=CARTESIAN_POINT('Ctrl Pts',(55.6838727952094,26.6454582217696,15.7087058094064));
#56095=CARTESIAN_POINT('Ctrl Pts',(55.7610880923709,26.6706878342199,15.7129384235779));
#56096=CARTESIAN_POINT('Ctrl Pts',(55.8381932491612,26.695881458997,15.7171650003226));
#56097=CARTESIAN_POINT('Ctrl Pts',(55.9141601801648,26.7249449804399,15.7213915770674));
#56098=CARTESIAN_POINT('Ctrl Pts',(55.9885748189535,26.7577533415498,15.7256181538122));
#56099=CARTESIAN_POINT('Ctrl Pts',(56.06290686611,26.790525289178,15.7298400395463));
#56100=CARTESIAN_POINT('Ctrl Pts',(56.1356896214532,26.827033631375,15.7340619252803));
#56101=CARTESIAN_POINT('Ctrl Pts',(56.2065264110986,26.8671042525896,15.7382838110143));
#56102=CARTESIAN_POINT('Ctrl Pts',(56.2773154235262,26.9071478474128,15.7425028492173));
#56103=CARTESIAN_POINT('Ctrl Pts',(56.3461606736869,26.9507487212528,15.7467218874204));
#56104=CARTESIAN_POINT('Ctrl Pts',(56.4126887774916,26.9976861714633,15.7509409256234));
#56105=CARTESIAN_POINT('Ctrl Pts',(56.4791951556432,27.0446082936139,15.7551585860424));
#56106=CARTESIAN_POINT('Ctrl Pts',(56.5433855108962,27.0948645606454,15.7593762464613));
#56107=CARTESIAN_POINT('Ctrl Pts',(56.6049153904789,27.1481909279291,15.7635939068803));
#56108=CARTESIAN_POINT('Ctrl Pts',(56.6664439896479,27.2015161855112,15.7678114795314));
#56109=CARTESIAN_POINT('Ctrl Pts',(56.7253118729403,27.2579111111848,15.7720290521824));
#56110=CARTESIAN_POINT('Ctrl Pts',(56.7812087422233,27.3170722931073,15.7762466248335));
#56111=CARTESIAN_POINT('Ctrl Pts',(56.8372004995652,27.3763339044417,15.7804713570498));
#56112=CARTESIAN_POINT('Ctrl Pts',(56.8902108313902,27.4383708279268,15.784696089266));
#56113=CARTESIAN_POINT('Ctrl Pts',(56.9399671376895,27.5028434434954,15.7889208214823));
#56114=CARTESIAN_POINT('Ctrl Pts',(56.9897110168295,27.5672999563521,15.7931444985274));
#56115=CARTESIAN_POINT('Ctrl Pts',(57.0362022471007,27.634190549858,15.7973681755725));
#56116=CARTESIAN_POINT('Ctrl Pts',(57.0792118848184,27.7031468132322,15.8015918526176));
#56117=CARTESIAN_POINT('Ctrl Pts',(57.1222995570996,27.7722281874466,15.8058231928939));
#56118=CARTESIAN_POINT('Ctrl Pts',(57.1618927863232,27.8433823143637,15.8100545331701));
#56119=CARTESIAN_POINT('Ctrl Pts',(57.1978084330948,27.9162157311451,15.8142858734464));
#56120=CARTESIAN_POINT('Ctrl Pts',(57.2336208576457,27.9888398233648,15.8185050527739));
#56121=CARTESIAN_POINT('Ctrl Pts',(57.2657767058958,28.0631331148853,15.8227242321014));
#56122=CARTESIAN_POINT('Ctrl Pts',(57.2941434032208,28.1386891992674,15.8269434114289));
#56123=CARTESIAN_POINT('Ctrl Pts',(57.3226004266787,28.214485871718,15.8311760256004));
#56124=CARTESIAN_POINT('Ctrl Pts',(57.3473499436632,28.2918353105073,15.8354086397718));
#56125=CARTESIAN_POINT('Ctrl Pts',(57.3682227782928,28.3703404710679,15.8396412539433));
#56126=CARTESIAN_POINT('Ctrl Pts',(57.3890658397837,28.4487336513884,15.8438678306881));
#56127=CARTESIAN_POINT('Ctrl Pts',(57.406043083288,28.5282788340695,15.8480944074329));
#56128=CARTESIAN_POINT('Ctrl Pts',(57.4190339916735,28.6085606086146,15.8523209841777));
#56129=CARTESIAN_POINT('Ctrl Pts',(57.432010481655,28.6887532796861,15.8565428699117));
#56130=CARTESIAN_POINT('Ctrl Pts',(57.4410093539002,28.7696804619158,15.8607647556457));
#56131=CARTESIAN_POINT('Ctrl Pts',(57.4459607113437,28.8509146265958,15.8649866413798));
#56132=CARTESIAN_POINT('Ctrl Pts',(57.4509087292501,28.9320940013509,15.8692056795828));
#56133=CARTESIAN_POINT('Ctrl Pts',(57.451814626031,29.0135794848453,15.8734247177858));
#56134=CARTESIAN_POINT('Ctrl Pts',(57.4486602620347,29.094937722387,15.8776437559888));
#56135=CARTESIAN_POINT('Ctrl Pts',(57.4455069281387,29.1762693912945,15.8818614164078));
#56136=CARTESIAN_POINT('Ctrl Pts',(57.4382959846715,29.2574734329289,15.8860790768268));
#56137=CARTESIAN_POINT('Ctrl Pts',(57.427061398562,29.3381171655067,15.8902967372457));
#56138=CARTESIAN_POINT('Ctrl Pts',(57.41582704624,29.418759219919,15.8945143098968));
#56139=CARTESIAN_POINT('Ctrl Pts',(57.4005692830146,29.4988405285149,15.8987318825478));
#56140=CARTESIAN_POINT('Ctrl Pts',(57.38137369184,29.5779356277409,15.9029494551989));
#56141=CARTESIAN_POINT('Ctrl Pts',(57.3621455150769,29.6571649953173,15.9071741874152));
#56142=CARTESIAN_POINT('Ctrl Pts',(57.3389662460126,29.7354043501289,15.9113989196315));
#56143=CARTESIAN_POINT('Ctrl Pts',(57.3119723628627,29.812240138973,15.9156236518477));
#56144=CARTESIAN_POINT('Ctrl Pts',(57.2849852217183,29.8890567372731,15.9198473288929));
#56145=CARTESIAN_POINT('Ctrl Pts',(57.254185567653,29.964470047114,15.924071005938));
#56146=CARTESIAN_POINT('Ctrl Pts',(57.2197577957976,30.0380874616312,15.9282946829831));
#56147=CARTESIAN_POINT('Ctrl Pts',(57.1852675598924,30.1118384439513,15.9325260232593));
#56148=CARTESIAN_POINT('Ctrl Pts',(57.1471362691119,30.1837866075215,15.9367573635356));
#56149=CARTESIAN_POINT('Ctrl Pts',(57.1055942687773,30.253564128911,15.9409887038118));
#56150=CARTESIAN_POINT('Ctrl Pts',(57.0641716609055,30.3231411084376,15.9452078831393));
#56151=CARTESIAN_POINT('Ctrl Pts',(57.0193582434643,30.3905595729623,15.9494270624668));
#56152=CARTESIAN_POINT('Ctrl Pts',(56.9714227466952,30.4554870675525,15.9536462417943));
#56153=CARTESIAN_POINT('Ctrl Pts',(56.9233346122044,30.5206213063203,15.9578788559658));
#56154=CARTESIAN_POINT('Ctrl Pts',(56.8719256086231,30.5834909223741,15.9621114701373));
#56155=CARTESIAN_POINT('Ctrl Pts',(56.8174366874645,30.643737855334,15.9663440843087));
#56156=CARTESIAN_POINT('Ctrl Pts',(56.7630254896356,30.7038988517011,15.9705706610535));
#56157=CARTESIAN_POINT('Ctrl Pts',(56.7055434087358,30.7614442534303,15.9747972377983));
#56158=CARTESIAN_POINT('Ctrl Pts',(56.6452732919455,30.8160468179017,15.9790238145431));
#56159=CARTESIAN_POINT('Ctrl Pts',(56.5850700680058,30.8705887798493,15.9832457002771));
#56160=CARTESIAN_POINT('Ctrl Pts',(56.5220852992742,30.9221940841614,15.9874675860112));
#56161=CARTESIAN_POINT('Ctrl Pts',(56.4566395555974,30.970571352443,15.9916894717452));
#56162=CARTESIAN_POINT('Ctrl Pts',(56.3912379530452,31.0189159917573,15.9959085099482));
#56163=CARTESIAN_POINT('Ctrl Pts',(56.3233790447604,31.0640366437438,16.0001275481512));
#56164=CARTESIAN_POINT('Ctrl Pts',(56.25341646435,31.1056821737613,16.0043465863543));
#56165=CARTESIAN_POINT('Ctrl Pts',(56.1834767311677,31.1473141038671,16.0085642467732));
#56166=CARTESIAN_POINT('Ctrl Pts',(56.1114350890396,31.1854729283111,16.0127819071922));
#56167=CARTESIAN_POINT('Ctrl Pts',(56.0376729739848,31.2199515870986,16.0169995676112));
#56168=CARTESIAN_POINT('Ctrl Pts',(55.9639123938918,31.2544295283982,16.0212171402622));
#56169=CARTESIAN_POINT('Ctrl Pts',(55.888431833396,31.2852272606572,16.0254347129133));
#56170=CARTESIAN_POINT('Ctrl Pts',(55.8116347734886,31.3121849503152,16.0296522855643));
#56171=CARTESIAN_POINT('Ctrl Pts',(55.7347073462809,31.3391884021577,16.0338770177806));
#56172=CARTESIAN_POINT('Ctrl Pts',(55.6564593889215,31.3623386143548,16.0381017499969));
#56173=CARTESIAN_POINT('Ctrl Pts',(55.5773120991202,31.3815249295797,16.0423264822132));
#56174=CARTESIAN_POINT('Ctrl Pts',(55.4981845771843,31.4007064528212,16.0465501592583));
#56175=CARTESIAN_POINT('Ctrl Pts',(55.4181586339014,31.4159259926763,16.0507738363034));
#56176=CARTESIAN_POINT('Ctrl Pts',(55.3376639826716,31.4271244889388,16.0549975133486));
#56177=CARTESIAN_POINT('Ctrl Pts',(55.2570232859202,31.4383433032001,16.0592288536248));
#56178=CARTESIAN_POINT('Ctrl Pts',(55.175912645807,31.4455264527967,16.0634601939011));
#56179=CARTESIAN_POINT('Ctrl Pts',(55.0947660020834,31.4486669138225,16.0676915341773));
#56180=CARTESIAN_POINT('Ctrl Pts',(55.0138525752865,31.4517983491064,16.0719107135048));
#56181=CARTESIAN_POINT('Ctrl Pts',(54.9329038058637,31.4509103904747,16.0761298928323));
#56182=CARTESIAN_POINT('Ctrl Pts',(54.8523448623591,31.4460474669001,16.0803490721598));
#56183=CARTESIAN_POINT('Ctrl Pts',(54.771529400524,31.4411690586507,16.0845816863313));
#56184=CARTESIAN_POINT('Ctrl Pts',(54.6908056775416,31.4322721592,16.0888143005027));
#56185=CARTESIAN_POINT('Ctrl Pts',(54.6106052176895,31.4193639563963,16.0930469146742));
#56186=CARTESIAN_POINT('Ctrl Pts',(54.5305191562626,31.4064741659317,16.097273491419));
#56187=CARTESIAN_POINT('Ctrl Pts',(54.4509553303829,31.3895845094472,16.1015000681638));
#56188=CARTESIAN_POINT('Ctrl Pts',(54.3723422216486,31.3687540951469,16.1057266449086));
#56189=CARTESIAN_POINT('Ctrl Pts',(54.2938163643621,31.3479468001944,16.1099485306426));
#56190=CARTESIAN_POINT('Ctrl Pts',(54.2162395743571,31.3232075565149,16.1141704163767));
#56191=CARTESIAN_POINT('Ctrl Pts',(54.1400307856651,31.2946466395496,16.1183923021107));
#56192=CARTESIAN_POINT('Ctrl Pts',(54.0638733974379,31.2661049860372,16.1226113403137));
#56193=CARTESIAN_POINT('Ctrl Pts',(53.9890826118921,31.2337469411841,16.1268303785167));
#56194=CARTESIAN_POINT('Ctrl Pts',(53.9160616055209,31.1977324238802,16.1310494167197));
#56195=CARTESIAN_POINT('Ctrl Pts',(53.8430644451482,31.1617296676045,16.1352670771387));
#56196=CARTESIAN_POINT('Ctrl Pts',(53.7718363324972,31.122073015557,16.1394847375576));
#56197=CARTESIAN_POINT('Ctrl Pts',(53.7027586087915,31.0789697022649,16.1437023979766));
#56198=CARTESIAN_POINT('Ctrl Pts',(53.6336823225671,31.0358672859364,16.1479199706277));
#56199=CARTESIAN_POINT('Ctrl Pts',(53.56675672981,30.9893185978865,16.1521375432787));
#56200=CARTESIAN_POINT('Ctrl Pts',(53.5023355583198,30.9395750746302,16.1563551159298));
#56201=CARTESIAN_POINT('Ctrl Pts',(53.4378050282915,30.8897471089638,16.160579848146));
#56202=CARTESIAN_POINT('Ctrl Pts',(53.3757877952056,30.8367137425227,16.1648045803623));
#56203=CARTESIAN_POINT('Ctrl Pts',(53.3166059815924,30.7807680446339,16.1690293125786));
#56204=CARTESIAN_POINT('Ctrl Pts',(53.2574389492577,30.7248363197699,16.1732529896237));
#56205=CARTESIAN_POINT('Ctrl Pts',(53.2011062272324,30.6659940694652,16.1774766666688));
#56206=CARTESIAN_POINT('Ctrl Pts',(53.1478912930289,30.6045695957365,16.1817003437139));
#56207=CARTESIAN_POINT('Ctrl Pts',(53.0945798082758,30.5430336764749,16.1859316839902));
#56208=CARTESIAN_POINT('Ctrl Pts',(53.0443977033076,30.4789065377686,16.1901630242664));
#56209=CARTESIAN_POINT('Ctrl Pts',(52.9975871071046,30.4125483554082,16.1943943645427));
#56210=CARTESIAN_POINT('Ctrl Pts',(52.9509110454044,30.3463808876679,16.1986135438702));
#56211=CARTESIAN_POINT('Ctrl Pts',(52.9075873121655,30.2779956123529,16.2028327231977));
#56212=CARTESIAN_POINT('Ctrl Pts',(52.8678101013429,30.2077733587328,16.2070519025252));
#56213=CARTESIAN_POINT('Ctrl Pts',(52.8261868754805,30.1342921703196,16.2114668891588));
#56214=CARTESIAN_POINT('Ctrl Pts',(52.788303131255,30.0585462817474,16.2158818757924));
#56215=CARTESIAN_POINT('Ctrl Pts',(52.7544002788845,29.9809343212091,16.220296862426));
#56216=CARTESIAN_POINT('Ctrl Pts',(52.7205854081671,29.9035237722959,16.2247003916808));
#56217=CARTESIAN_POINT('Ctrl Pts',(52.6907310153447,29.8242571676171,16.2291039209355));
#56218=CARTESIAN_POINT('Ctrl Pts',(52.6650326032107,29.7435573319732,16.2335074501903));
#56219=CARTESIAN_POINT('Ctrl Pts',(52.639373597316,29.6629812423809,16.2379042270229));
#56220=CARTESIAN_POINT('Ctrl Pts',(52.6178580208794,29.5809766782397,16.2423010038556));
#56221=CARTESIAN_POINT('Ctrl Pts',(52.6006334744758,29.4979864718987,16.2466977806882));
#56222=CARTESIAN_POINT('Ctrl Pts',(52.5834410517142,29.4151510416315,16.2510863575671));
#56223=CARTESIAN_POINT('Ctrl Pts',(52.5705238034113,29.3313340272056,16.2554749344459));
#56224=CARTESIAN_POINT('Ctrl Pts',(52.5619792507151,29.2469920566668,16.2598635113248));
#56225=CARTESIAN_POINT('Ctrl Pts',(52.5536662209177,29.1649354131899,16.2641331754791));
#56226=CARTESIAN_POINT('Ctrl Pts',(52.5494920101768,29.0823822816067,16.2684028396335));
#56227=CARTESIAN_POINT('Ctrl Pts',(52.5495000114916,28.9997626807474,16.2726725037879));
#56228=CARTESIAN_POINT('',(52.5495007998519,28.9980200824703,17.0726725037486));
#56229=CARTESIAN_POINT('Ctrl Pts',(52.5495000114917,28.9997626798325,16.2726725038352));
#56230=CARTESIAN_POINT('Ctrl Pts',(52.5495083514886,28.9136462633258,16.277122878478));
#56231=CARTESIAN_POINT('Ctrl Pts',(52.5540604740065,28.8276303692676,16.2815732531209));
#56232=CARTESIAN_POINT('Ctrl Pts',(52.5630991174095,28.7421932149272,16.2860236277637));
#56233=CARTESIAN_POINT('Ctrl Pts',(52.572165603043,28.6564928838203,16.2904877111404));
#56234=CARTESIAN_POINT('Ctrl Pts',(52.5857461974439,28.5713752385803,16.2949517945171));
#56235=CARTESIAN_POINT('Ctrl Pts',(52.6037321076618,28.4873105831509,16.2994158778938));
#56236=CARTESIAN_POINT('Ctrl Pts',(52.6217470390047,28.4031102853858,16.3038871642821));
#56237=CARTESIAN_POINT('Ctrl Pts',(52.6441813651551,28.3199667357462,16.3083584506705));
#56238=CARTESIAN_POINT('Ctrl Pts',(52.6708765315756,28.2383346411747,16.3128297370589));
#56239=CARTESIAN_POINT('Ctrl Pts',(52.697646299248,28.1564744207934,16.3173135187266));
#56240=CARTESIAN_POINT('Ctrl Pts',(52.728700575226,28.0761344581581,16.3217973003944));
#56241=CARTESIAN_POINT('Ctrl Pts',(52.7638324599678,27.9977500397076,16.3262810820621));
#56242=CARTESIAN_POINT('Ctrl Pts',(52.7833519533301,27.9541991699804,16.328772299005));
#56243=CARTESIAN_POINT('Ctrl Pts',(52.8041293765503,27.9112515299105,16.3312635159478));
#56244=CARTESIAN_POINT('Ctrl Pts',(52.8261233377633,27.8689781136589,16.3337547328906));
#56245=CARTESIAN_POINT('Ctrl Pts',(52.863491400864,27.7971549586266,16.3379873470621));
#56246=CARTESIAN_POINT('Ctrl Pts',(52.9044922481289,27.7270521427378,16.3422199612336));
#56247=CARTESIAN_POINT('Ctrl Pts',(52.948943574148,27.6590608559778,16.3464525754051));
#56248=CARTESIAN_POINT('Ctrl Pts',(52.9933314945241,27.5911665524043,16.3506791521498));
#56249=CARTESIAN_POINT('Ctrl Pts',(53.0411598662639,27.5253781815362,16.3549057288946));
#56250=CARTESIAN_POINT('Ctrl Pts',(53.0922002035034,27.4620630095848,16.3591323056394));
#56251=CARTESIAN_POINT('Ctrl Pts',(53.1431838918788,27.3988181101425,16.3633541913734));
#56252=CARTESIAN_POINT('Ctrl Pts',(53.1973721722039,27.3380413152227,16.3675760771075));
#56253=CARTESIAN_POINT('Ctrl Pts',(53.2544937151468,27.2800703329677,16.3717979628415));
#56254=CARTESIAN_POINT('Ctrl Pts',(53.3115767313805,27.2221384503424,16.3760170010445));
#56255=CARTESIAN_POINT('Ctrl Pts',(53.3715887557567,27.1670089518904,16.3802360392476));
#56256=CARTESIAN_POINT('Ctrl Pts',(53.4342195362188,27.114984936601,16.3844550774506));
#56257=CARTESIAN_POINT('Ctrl Pts',(53.4968298637513,27.0629779104584,16.3886727378696));
#56258=CARTESIAN_POINT('Ctrl Pts',(53.5620568919404,27.0140746500654,16.3928903982885));
#56259=CARTESIAN_POINT('Ctrl Pts',(53.6295560472169,26.9685390423933,16.3971080587075));
#56260=CARTESIAN_POINT('Ctrl Pts',(53.6970537978615,26.9230043823,16.4013256313585));
#56261=CARTESIAN_POINT('Ctrl Pts',(53.7668231958184,26.8808374944166,16.4055432040096));
#56262=CARTESIAN_POINT('Ctrl Pts',(53.8384905429322,26.8422590444768,16.4097607766606));
#56263=CARTESIAN_POINT('Ctrl Pts',(53.9102795493723,26.8036151054626,16.4139855088769));
#56264=CARTESIAN_POINT('Ctrl Pts',(53.9839725399857,26.7685720135591,16.4182102410932));
#56265=CARTESIAN_POINT('Ctrl Pts',(54.0591706641969,26.7373046137643,16.4224349733095));
#56266=CARTESIAN_POINT('Ctrl Pts',(54.134350006888,26.7060450233305,16.4266586503546));
#56267=CARTESIAN_POINT('Ctrl Pts',(54.2110332854379,26.6785593764845,16.4308823273997));
#56268=CARTESIAN_POINT('Ctrl Pts',(54.28880520915,26.6549728744708,16.4351060044448));
#56269=CARTESIAN_POINT('Ctrl Pts',(54.3667182384014,26.6313435782722,16.4393373447211));
#56270=CARTESIAN_POINT('Ctrl Pts',(54.445723408118,26.6116276776904,16.4435686849973));
#56271=CARTESIAN_POINT('Ctrl Pts',(54.5253931562493,26.5958996289953,16.4478000252736));
#56272=CARTESIAN_POINT('Ctrl Pts',(54.6048339320789,26.5802167829975,16.4520192046011));
#56273=CARTESIAN_POINT('Ctrl Pts',(54.6849350089078,26.568498880775,16.4562383839286));
#56274=CARTESIAN_POINT('Ctrl Pts',(54.7652694833726,26.5607681876124,16.4604575632561));
#56275=CARTESIAN_POINT('Ctrl Pts',(54.8458597614063,26.5530128781326,16.4646901774276));
#56276=CARTESIAN_POINT('Ctrl Pts',(54.9269846661948,26.5492413936723,16.4689227915991));
#56277=CARTESIAN_POINT('Ctrl Pts',(55.0082168104974,26.5495137759977,16.4731554057706));
#56278=CARTESIAN_POINT('Ctrl Pts',(55.0893330847734,26.5497857697952,16.4773819825153));
#56279=CARTESIAN_POINT('Ctrl Pts',(55.1705558340651,26.554090172453,16.4816085592601));
#56280=CARTESIAN_POINT('Ctrl Pts',(55.2514525983209,26.5624352642858,16.4858351360049));
#56281=CARTESIAN_POINT('Ctrl Pts',(55.332259576536,26.5707710940329,16.4900570217389));
#56282=CARTESIAN_POINT('Ctrl Pts',(55.412740828855,26.5831386544429,16.494278907473));
#56283=CARTESIAN_POINT('Ctrl Pts',(55.4924653652614,26.5994941962124,16.498500793207));
#56284=CARTESIAN_POINT('Ctrl Pts',(55.5721361299403,26.6158387066761,16.50271983141));
#56285=CARTESIAN_POINT('Ctrl Pts',(55.6510507384723,26.6361657632645,16.5069388696131));
#56286=CARTESIAN_POINT('Ctrl Pts',(55.7287860423086,26.6603801260598,16.5111579078161));
#56287=CARTESIAN_POINT('Ctrl Pts',(55.8064959606288,26.6845865813269,16.515375568235));
#56288=CARTESIAN_POINT('Ctrl Pts',(55.8830268958855,26.7126776836939,16.519593228654));
#56289=CARTESIAN_POINT('Ctrl Pts',(55.957969906901,26.7445080564382,16.523810889073));
#56290=CARTESIAN_POINT('Ctrl Pts',(56.0329113583808,26.7763377668045,16.528028461724));
#56291=CARTESIAN_POINT('Ctrl Pts',(56.1062645241991,26.8119064101505,16.5322460343751));
#56292=CARTESIAN_POINT('Ctrl Pts',(56.1776408627946,26.8510206496394,16.5364636070261));
#56293=CARTESIAN_POINT('Ctrl Pts',(56.2491383667132,26.8902012877354,16.5406883392424));
#56294=CARTESIAN_POINT('Ctrl Pts',(56.3186519197543,26.9329393398588,16.5449130714587));
#56295=CARTESIAN_POINT('Ctrl Pts',(56.3858177229479,26.978995425843,16.549137803675));
#56296=CARTESIAN_POINT('Ctrl Pts',(56.4529667507777,27.0250400088366,16.5533614807201));
#56297=CARTESIAN_POINT('Ctrl Pts',(56.5177688434134,27.074400669101,16.5575851577652));
#56298=CARTESIAN_POINT('Ctrl Pts',(56.5798928943025,27.1267972099817,16.5618088348103));
#56299=CARTESIAN_POINT('Ctrl Pts',(56.6421296600028,27.1792888165596,16.5660401750865));
#56300=CARTESIAN_POINT('Ctrl Pts',(56.7016783328847,27.2348269938406,16.5702715153628));
#56301=CARTESIAN_POINT('Ctrl Pts',(56.7582436920257,27.2930936260439,16.574502855639));
#56302=CARTESIAN_POINT('Ctrl Pts',(56.8146464812982,27.3511927988891,16.5787220349665));
#56303=CARTESIAN_POINT('Ctrl Pts',(56.8680828441032,27.4120043674583,16.5829412142941));
#56304=CARTESIAN_POINT('Ctrl Pts',(56.918301697223,27.4751823556794,16.5871603936216));
#56305=CARTESIAN_POINT('Ctrl Pts',(56.9686804587996,27.5385615172444,16.5913930077931));
#56306=CARTESIAN_POINT('Ctrl Pts',(57.0160085386848,27.6045579347712,16.5956256219645));
#56307=CARTESIAN_POINT('Ctrl Pts',(57.0600029023717,27.6728457918463,16.599858236136));
#56308=CARTESIAN_POINT('Ctrl Pts',(57.1039345122297,27.7410362427052,16.6040848128808));
#56309=CARTESIAN_POINT('Ctrl Pts',(57.1445416008929,27.811511254128,16.6083113896256));
#56310=CARTESIAN_POINT('Ctrl Pts',(57.1815817910237,27.8839125755237,16.6125379663704));
#56311=CARTESIAN_POINT('Ctrl Pts',(57.2185808708324,27.9562335398365,16.6167598521044));
#56312=CARTESIAN_POINT('Ctrl Pts',(57.2520207078107,28.0304761544739,16.6209817378384));
#56313=CARTESIAN_POINT('Ctrl Pts',(57.2817033686652,28.1062550769813,16.6252036235725));
#56314=CARTESIAN_POINT('Ctrl Pts',(57.3113660094856,28.1819828889555,16.6294226617755));
#56315=CARTESIAN_POINT('Ctrl Pts',(57.3372763381311,28.2592445193989,16.6336416999785));
#56316=CARTESIAN_POINT('Ctrl Pts',(57.3592838818366,28.3376331719461,16.6378607381815));
#56317=CARTESIAN_POINT('Ctrl Pts',(57.3812842386806,28.4159962256173,16.6420783986005));
#56318=CARTESIAN_POINT('Ctrl Pts',(57.3993842162074,28.4954851235652,16.6462960590195));
#56319=CARTESIAN_POINT('Ctrl Pts',(57.4134831321724,28.5756776924088,16.6505137194384));
#56320=CARTESIAN_POINT('Ctrl Pts',(57.4275817547442,28.6558685924754,16.6547312920895));
#56321=CARTESIAN_POINT('Ctrl Pts',(57.4376794020145,28.7367626765894,16.6589488647405));
#56322=CARTESIAN_POINT('Ctrl Pts',(57.4437267274599,28.8179287735577,16.6631664373916));
#56323=CARTESIAN_POINT('Ctrl Pts',(57.4497843185781,28.8992326545108,16.6673911696079));
#56324=CARTESIAN_POINT('Ctrl Pts',(57.4517777966085,28.9808090064826,16.6716159018241));
#56325=CARTESIAN_POINT('Ctrl Pts',(57.4497099072213,29.0622223469638,16.6758406340404));
#56326=CARTESIAN_POINT('Ctrl Pts',(57.4476425343112,29.1436153536094,16.6800643110855));
#56327=CARTESIAN_POINT('Ctrl Pts',(57.4415158787183,29.2248449669468,16.6842879881306));
#56328=CARTESIAN_POINT('Ctrl Pts',(57.4313847217911,29.3054809071624,16.6885116651758));
#56329=CARTESIAN_POINT('Ctrl Pts',(57.4212351833929,29.3862631492473,16.692743005452));
#56330=CARTESIAN_POINT('Ctrl Pts',(57.4070667047341,29.4664491068097,16.6969743457282));
#56331=CARTESIAN_POINT('Ctrl Pts',(57.3889854108488,29.5456179586045,16.7012056860045));
#56332=CARTESIAN_POINT('Ctrl Pts',(57.3709560829302,29.6245592776825,16.705424865332));
#56333=CARTESIAN_POINT('Ctrl Pts',(57.349036604091,29.7024889138234,16.7096440446595));
#56334=CARTESIAN_POINT('Ctrl Pts',(57.3233804978824,29.7790079024373,16.713863223987));
#56335=CARTESIAN_POINT('Ctrl Pts',(57.2976426966906,29.8557705452298,16.7180958381585));
#56336=CARTESIAN_POINT('Ctrl Pts',(57.268048681599,29.9313990355144,16.72232845233));
#56337=CARTESIAN_POINT('Ctrl Pts',(57.234717671421,30.0054785820886,16.7265610665014));
#56338=CARTESIAN_POINT('Ctrl Pts',(57.2014342047993,30.0794524611453,16.7307876432462));
#56339=CARTESIAN_POINT('Ctrl Pts',(57.1644245191242,30.1518813645678,16.735014219991));
#56340=CARTESIAN_POINT('Ctrl Pts',(57.1238571736111,30.2223669482199,16.7392407967358));
#56341=CARTESIAN_POINT('Ctrl Pts',(57.083334853154,30.2927743010362,16.7434626824698));
#56342=CARTESIAN_POINT('Ctrl Pts',(57.0392629492597,30.3612422191618,16.7476845682039));
#56343=CARTESIAN_POINT('Ctrl Pts',(56.9918569418559,30.4273948904141,16.7519064539379));
#56344=CARTESIAN_POINT('Ctrl Pts',(56.944482908334,30.4935029437412,16.7561254921409));
#56345=CARTESIAN_POINT('Ctrl Pts',(56.8937795074125,30.5572984749663,16.7603445303439));
#56346=CARTESIAN_POINT('Ctrl Pts',(56.8400060526505,30.6184338034685,16.764563568547));
#56347=CARTESIAN_POINT('Ctrl Pts',(56.7862501583383,30.6795491674013,16.7687812289659));
#56348=CARTESIAN_POINT('Ctrl Pts',(56.7294265077996,30.7380057052982,16.7729988893849));
#56349=CARTESIAN_POINT('Ctrl Pts',(56.6698344192217,30.7934891308236,16.7772165498039));
#56350=CARTESIAN_POINT('Ctrl Pts',(56.6102435707326,30.84897140176,16.7814341224549));
#56351=CARTESIAN_POINT('Ctrl Pts',(56.5478847395449,30.9014803676415,16.785651695106));
#56352=CARTESIAN_POINT('Ctrl Pts',(56.4830927386459,30.9507399054143,16.789869267757));
#56353=CARTESIAN_POINT('Ctrl Pts',(56.4181907497049,31.000083064005,16.7940939999733));
#56354=CARTESIAN_POINT('Ctrl Pts',(56.3508476987579,31.0461654754529,16.7983187321896));
#56355=CARTESIAN_POINT('Ctrl Pts',(56.281430374265,31.0887523658661,16.8025434644059));
#56356=CARTESIAN_POINT('Ctrl Pts',(56.2120303874769,31.1313286197568,16.806767141451));
#56357=CARTESIAN_POINT('Ctrl Pts',(56.1405575823523,31.1704108934794,16.8109908184961));
#56358=CARTESIAN_POINT('Ctrl Pts',(56.067402711464,31.2058108943332,16.8152144955412));
#56359=CARTESIAN_POINT('Ctrl Pts',(55.9941151119893,31.2412751232012,16.8194458358175));
#56360=CARTESIAN_POINT('Ctrl Pts',(55.9191397766967,31.2730435458163,16.8236771760937));
#56361=CARTESIAN_POINT('Ctrl Pts',(55.8428874756168,31.3009760871092,16.8279085163699));
#56362=CARTESIAN_POINT('Ctrl Pts',(55.7668543250338,31.3288283497716,16.8321276956975));
#56363=CARTESIAN_POINT('Ctrl Pts',(55.6895519983229,31.3528666946968,16.836346875025));
#56364=CARTESIAN_POINT('Ctrl Pts',(55.6113987353919,31.3730027046679,16.8405660543525));
#56365=CARTESIAN_POINT('Ctrl Pts',(55.5329966143747,31.3932028323575,16.844798668524));
#56366=CARTESIAN_POINT('Ctrl Pts',(55.4534465231365,31.4095508370058,16.8490312826954));
#56367=CARTESIAN_POINT('Ctrl Pts',(55.3731613018205,31.4219209096962,16.8532638968669));
#56368=CARTESIAN_POINT('Ctrl Pts',(55.2929905998342,31.4342733376394,16.8574904736117));
#56369=CARTESIAN_POINT('Ctrl Pts',(55.2120873057286,31.4426590330567,16.8617170503565));
#56370=CARTESIAN_POINT('Ctrl Pts',(55.1308773243872,31.4470025288016,16.8659436271013));
#56371=CARTESIAN_POINT('Ctrl Pts',(55.0497574767212,31.4513412037691,16.8701655128353));
#56372=CARTESIAN_POINT('Ctrl Pts',(54.9683320797156,31.4516465687934,16.8743873985693));
#56373=CARTESIAN_POINT('Ctrl Pts',(54.8870336815561,31.4478947814188,16.8786092843034));
#56374=CARTESIAN_POINT('Ctrl Pts',(54.8057901166451,31.4441455245083,16.8828283225064));
#56375=CARTESIAN_POINT('Ctrl Pts',(54.7246738433155,31.436344571335,16.8870473607094));
#56376=CARTESIAN_POINT('Ctrl Pts',(54.6441176753538,31.4245201630435,16.8912663989124));
#56377=CARTESIAN_POINT('Ctrl Pts',(54.5635878140997,31.4126996161726,16.8954840593314));
#56378=CARTESIAN_POINT('Ctrl Pts',(54.4836181542365,31.3968582909499,16.8997017197504));
#56379=CARTESIAN_POINT('Ctrl Pts',(54.4046352761339,31.3770761652871,16.9039193801693));
#56380=CARTESIAN_POINT('Ctrl Pts',(54.325654041635,31.3572944512828,16.9081369528204));
#56381=CARTESIAN_POINT('Ctrl Pts',(54.247659998412,31.3335722138928,16.9123545254714));
#56382=CARTESIAN_POINT('Ctrl Pts',(54.1710670379086,31.3060399810841,16.9165720981225));
#56383=CARTESIAN_POINT('Ctrl Pts',(54.0943440565751,31.2784610107718,16.9207968303388));
#56384=CARTESIAN_POINT('Ctrl Pts',(54.0190273560809,31.2470592626936,16.925021562555));
#56385=CARTESIAN_POINT('Ctrl Pts',(53.9455135506227,31.212014597167,16.9292462947713));
#56386=CARTESIAN_POINT('Ctrl Pts',(53.8720181060084,31.176978684413,16.9334699718164));
#56387=CARTESIAN_POINT('Ctrl Pts',(53.8003250561296,31.1383019137261,16.9376936488615));
#56388=CARTESIAN_POINT('Ctrl Pts',(53.7308050716692,31.0962095515238,16.9419173259067));
#56389=CARTESIAN_POINT('Ctrl Pts',(53.6611589535809,31.0540408190173,16.9461486661829));
#56390=CARTESIAN_POINT('Ctrl Pts',(53.593694166273,31.0084443712258,16.9503800064591));
#56391=CARTESIAN_POINT('Ctrl Pts',(53.5287518317834,30.9596885154328,16.9546113467354));
#56392=CARTESIAN_POINT('Ctrl Pts',(53.4639961427416,30.9110727848542,16.9588305260629));
#56393=CARTESIAN_POINT('Ctrl Pts',(53.4017487236058,30.8593161374303,16.9630497053904));
#56394=CARTESIAN_POINT('Ctrl Pts',(53.3423114311109,30.8047212689428,16.9672688847179));
#56395=CARTESIAN_POINT('Ctrl Pts',(53.2835680460246,30.7507637744359,16.9714388067581));
#56396=CARTESIAN_POINT('Ctrl Pts',(53.2273369812938,30.6938201153398,16.9756087287983));
#56397=CARTESIAN_POINT('Ctrl Pts',(53.1739438484535,30.634157024707,16.9797786508385));
#56398=CARTESIAN_POINT('Ctrl Pts',(53.1206398580088,30.5745935444649,16.9839416109939));
#56399=CARTESIAN_POINT('Ctrl Pts',(53.0701647033382,30.512320006737,16.9881045711492));
#56400=CARTESIAN_POINT('Ctrl Pts',(53.0228091583226,30.447641746285,16.9922675313046));
#56401=CARTESIAN_POINT('Ctrl Pts',(52.9754979972637,30.3830241054945,16.9964265897281));
#56402=CARTESIAN_POINT('Ctrl Pts',(52.931300928673,30.3160065967259,17.0005856481515));
#56403=CARTESIAN_POINT('Ctrl Pts',(52.8904694793152,30.2469287198149,17.004744706575));
#56404=CARTESIAN_POINT('Ctrl Pts',(52.8496629348429,30.1778929765201,17.0089012282069));
#56405=CARTESIAN_POINT('Ctrl Pts',(52.8122181796767,30.1067997705884,17.0130577498389));
#56406=CARTESIAN_POINT('Ctrl Pts',(52.7783433561058,30.0340174111884,17.0172142714708));
#56407=CARTESIAN_POINT('Ctrl Pts',(52.7444781103174,29.9612556303046,17.021369617886));
#56408=CARTESIAN_POINT('Ctrl Pts',(52.7141809930965,29.8868060793133,17.0255249643012));
#56409=CARTESIAN_POINT('Ctrl Pts',(52.687613375193,29.8110600146806,17.0296803107164));
#56410=CARTESIAN_POINT('Ctrl Pts',(52.6610324672833,29.7352760593467,17.033837735774));
#56411=CARTESIAN_POINT('Ctrl Pts',(52.6381849466468,29.6581947472086,17.0379951608317));
#56412=CARTESIAN_POINT('Ctrl Pts',(52.6191829795114,29.5802245814782,17.0421525858894));
#56413=CARTESIAN_POINT('Ctrl Pts',(52.6001756703733,29.5022324960787,17.0463111797196));
#56414=CARTESIAN_POINT('Ctrl Pts',(52.5850161616061,29.4233515301268,17.0504697735497));
#56415=CARTESIAN_POINT('Ctrl Pts',(52.5737654496017,29.3440002274034,17.0546283673798));
#56416=CARTESIAN_POINT('Ctrl Pts',(52.5625012777943,29.2645539926524,17.0587919363488));
#56417=CARTESIAN_POINT('Ctrl Pts',(52.5551552817256,29.1846367754754,17.0629555053177));
#56418=CARTESIAN_POINT('Ctrl Pts',(52.5517364939461,29.104671175233,17.0671190742866));
#56419=CARTESIAN_POINT('Ctrl Pts',(52.5502164841563,29.0691180777464,17.0689702174406));
#56420=CARTESIAN_POINT('Ctrl Pts',(52.5494720885549,29.033555406209,17.0708213605946));
#56421=CARTESIAN_POINT('Ctrl Pts',(52.5495007998519,28.9980200824703,17.0726725037486));
#56422=CARTESIAN_POINT('',(52.5495006756093,29.0018196594696,17.8726725038366));
#56423=CARTESIAN_POINT('Ctrl Pts',(52.5495007998525,28.9980200817158,17.0726725037879));
#56424=CARTESIAN_POINT('Ctrl Pts',(52.5496038336256,28.8704975568272,17.0793155401837));
#56425=CARTESIAN_POINT('Ctrl Pts',(52.559664163214,28.7433683178552,17.0859585765795));
#56426=CARTESIAN_POINT('Ctrl Pts',(52.5794817419324,28.617846088125,17.0926016129752));
#56427=CARTESIAN_POINT('Ctrl Pts',(52.580844176456,28.6092165869286,17.0930583136779));
#56428=CARTESIAN_POINT('Ctrl Pts',(52.5822527123098,28.6005946686822,17.0935150143807));
#56429=CARTESIAN_POINT('Ctrl Pts',(52.5837072777295,28.5919807231239,17.0939717150834));
#56430=CARTESIAN_POINT('Ctrl Pts',(52.5971879099513,28.5121483343735,17.0982043292549));
#56431=CARTESIAN_POINT('Ctrl Pts',(52.6146542582931,28.4328362864386,17.1024369434264));
#56432=CARTESIAN_POINT('Ctrl Pts',(52.6360530944036,28.3544728684856,17.1066695575979));
#56433=CARTESIAN_POINT('Ctrl Pts',(52.6574214070836,28.2762212285905,17.1108961343427));
#56434=CARTESIAN_POINT('Ctrl Pts',(52.6827109453337,28.1989159756004,17.1151227110875));
#56435=CARTESIAN_POINT('Ctrl Pts',(52.7118171822583,28.1229768289311,17.1193492878323));
#56436=CARTESIAN_POINT('Ctrl Pts',(52.7408911146304,28.0471219659212,17.1235711735663));
#56437=CARTESIAN_POINT('Ctrl Pts',(52.773773163146,27.9726306280977,17.1277930593003));
#56438=CARTESIAN_POINT('Ctrl Pts',(52.8103089458219,27.8999075778588,17.1320149450344));
#56439=CARTESIAN_POINT('Ctrl Pts',(52.8468200862455,27.8272335770619,17.1362339832374));
#56440=CARTESIAN_POINT('Ctrl Pts',(52.8869798584444,27.7563259091673,17.1404530214404));
#56441=CARTESIAN_POINT('Ctrl Pts',(52.9305862035729,27.687568367816,17.1446720596435));
#56442=CARTESIAN_POINT('Ctrl Pts',(52.9741783084588,27.618833280171,17.1488897200624));
#56443=CARTESIAN_POINT('Ctrl Pts',(53.0212145024397,27.5522473166407,17.1531073804814));
#56444=CARTESIAN_POINT('Ctrl Pts',(53.0714480133359,27.4881675077133,17.1573250409004));
#56445=CARTESIAN_POINT('Ctrl Pts',(53.1216804788918,27.4240890322624,17.1615426135514));
#56446=CARTESIAN_POINT('Ctrl Pts',(53.175109841548,27.3625169725988,17.1657601862025));
#56447=CARTESIAN_POINT('Ctrl Pts',(53.2314483286741,27.3037761834445,17.1699777588535));
#56448=CARTESIAN_POINT('Ctrl Pts',(53.2878824535298,27.2449356785186,17.1742024910698));
#56449=CARTESIAN_POINT('Ctrl Pts',(53.3472352601923,27.1889363973004,17.178427223286));
#56450=CARTESIAN_POINT('Ctrl Pts',(53.4091809563462,27.1360673240837,17.1826519555023));
#56451=CARTESIAN_POINT('Ctrl Pts',(53.4711111809132,27.0832114554722,17.1868756325474));
#56452=CARTESIAN_POINT('Ctrl Pts',(53.5356326177369,27.0334844991816,17.1910993095925));
#56453=CARTESIAN_POINT('Ctrl Pts',(53.6023885701024,26.9871332530394,17.1953229866376));
#56454=CARTESIAN_POINT('Ctrl Pts',(53.6692656411725,26.9406979094844,17.1995543269139));
#56455=CARTESIAN_POINT('Ctrl Pts',(53.7383849344819,26.8976507624229,17.2037856671901));
#56456=CARTESIAN_POINT('Ctrl Pts',(53.809362477328,26.8581940938532,17.2080170074664));
#56457=CARTESIAN_POINT('Ctrl Pts',(53.8801360294271,26.8188508244653,17.2122361867938));
#56458=CARTESIAN_POINT('Ctrl Pts',(53.9527567188956,26.7830775494876,17.2164553661213));
#56459=CARTESIAN_POINT('Ctrl Pts',(54.0268251565367,26.7510266844513,17.2206745454487));
#56460=CARTESIAN_POINT('Ctrl Pts',(54.1011294452352,26.7188737620387,17.2249071596202));
#56461=CARTESIAN_POINT('Ctrl Pts',(54.1771670859999,26.6903474328163,17.2291397737917));
#56462=CARTESIAN_POINT('Ctrl Pts',(54.2545498415163,26.6656362084678,17.2333723879632));
#56463=CARTESIAN_POINT('Ctrl Pts',(54.3318222177978,26.6409602323606,17.237598964708));
#56464=CARTESIAN_POINT('Ctrl Pts',(54.4104354592304,26.6200886929779,17.2418255414527));
#56465=CARTESIAN_POINT('Ctrl Pts',(54.4899805900535,26.6031624061114,17.2460521181975));
#56466=CARTESIAN_POINT('Ctrl Pts',(54.5694374349925,26.5862549054633,17.2502740039316));
#56467=CARTESIAN_POINT('Ctrl Pts',(54.6498236621059,26.5732840529162,17.2544958896656));
#56468=CARTESIAN_POINT('Ctrl Pts',(54.7307157008067,26.5643407019437,17.2587177753996));
#56469=CARTESIAN_POINT('Ctrl Pts',(54.8115531803359,26.5554033829842,17.2629368136026));
#56470=CARTESIAN_POINT('Ctrl Pts',(54.8928953333469,26.5504882214594,17.2671558518057));
#56471=CARTESIAN_POINT('Ctrl Pts',(54.974310223053,26.5496346628798,17.2713748900087));
#56472=CARTESIAN_POINT('Ctrl Pts',(55.0556985256243,26.5487813830412,17.2755925504277));
#56473=CARTESIAN_POINT('Ctrl Pts',(55.1371590535514,26.5519870769218,17.2798102108466));
#56474=CARTESIAN_POINT('Ctrl Pts',(55.2182579776805,26.5592391134774,17.2840278712656));
#56475=CARTESIAN_POINT('Ctrl Pts',(55.2993552141717,26.5664909991208,17.2882454439166));
#56476=CARTESIAN_POINT('Ctrl Pts',(55.3800903992291,26.5777890174768,17.2924630165677));
#56477=CARTESIAN_POINT('Ctrl Pts',(55.4600343728646,26.5930686287758,17.2966805892187));
#56478=CARTESIAN_POINT('Ctrl Pts',(55.5401140558626,26.6083741780688,17.300905321435));
#56479=CARTESIAN_POINT('Ctrl Pts',(55.6193993814666,26.6276747557694,17.3051300536513));
#56480=CARTESIAN_POINT('Ctrl Pts',(55.6974705807617,26.6508544023471,17.3093547858676));
#56481=CARTESIAN_POINT('Ctrl Pts',(55.7755222809558,26.6740282595649,17.3135784629127));
#56482=CARTESIAN_POINT('Ctrl Pts',(55.8523600286027,26.7010790733834,17.3178021399578));
#56483=CARTESIAN_POINT('Ctrl Pts',(55.9275826174791,26.731841994536,17.322025817003));
#56484=CARTESIAN_POINT('Ctrl Pts',(56.0029416865075,26.7626607304141,17.3262571572792));
#56485=CARTESIAN_POINT('Ctrl Pts',(56.0766793184366,26.7972048357748,17.3304884975554));
#56486=CARTESIAN_POINT('Ctrl Pts',(56.1484167989744,26.8352623471115,17.3347198378317));
#56487=CARTESIAN_POINT('Ctrl Pts',(56.219948104692,26.8732104804703,17.3389390171592));
#56488=CARTESIAN_POINT('Ctrl Pts',(56.2894903921097,26.9146515470883,17.3431581964868));
#56489=CARTESIAN_POINT('Ctrl Pts',(56.3566983834342,26.95933350437,17.3473773758143));
#56490=CARTESIAN_POINT('Ctrl Pts',(56.4241203805653,27.0041577393498,17.3516099899858));
#56491=CARTESIAN_POINT('Ctrl Pts',(56.4894439381013,27.0524102740276,17.3558426041573));
#56492=CARTESIAN_POINT('Ctrl Pts',(56.5522995709792,27.1038680710621,17.3600752183287));
#56493=CARTESIAN_POINT('Ctrl Pts',(56.6150655461986,27.1552524683808,17.3643017950735));
#56494=CARTESIAN_POINT('Ctrl Pts',(56.6753702319868,27.209832755635,17.3685283718183));
#56495=CARTESIAN_POINT('Ctrl Pts',(56.7328728617713,27.2673425338699,17.3727549485631));
#56496=CARTESIAN_POINT('Ctrl Pts',(56.7903116702955,27.3247884829104,17.3769768342971));
#56497=CARTESIAN_POINT('Ctrl Pts',(56.8449542754861,27.3851571355647,17.3811987200312));
#56498=CARTESIAN_POINT('Ctrl Pts',(56.8964938749885,27.4481426508434,17.3854206057652));
#56499=CARTESIAN_POINT('Ctrl Pts',(56.9479987126293,27.5110856843453,17.3896396439682));
#56500=CARTESIAN_POINT('Ctrl Pts',(56.9964044077957,27.5766417164459,17.3938586821712));
#56501=CARTESIAN_POINT('Ctrl Pts',(57.0414427258633,27.6444699018392,17.3980777203743));
#56502=CARTESIAN_POINT('Ctrl Pts',(57.0864663360583,27.7122759370201,17.4022953807932));
#56503=CARTESIAN_POINT('Ctrl Pts',(57.1281244962423,27.7823522652168,17.4065130412122));
#56504=CARTESIAN_POINT('Ctrl Pts',(57.1661916247125,27.8543281032401,17.4107307016311));
#56505=CARTESIAN_POINT('Ctrl Pts',(57.2042579610201,27.9263024434734,17.4149482742822));
#56506=CARTESIAN_POINT('Ctrl Pts',(57.2387331980426,28.0001758037414,17.4191658469332));
#56507=CARTESIAN_POINT('Ctrl Pts',(57.2694378383232,28.075553058317,17.4233834195843));
#56508=CARTESIAN_POINT('Ctrl Pts',(57.3001946014463,28.151058269994,17.4276081518006));
#56509=CARTESIAN_POINT('Ctrl Pts',(57.3271677851512,28.2280720513354,17.4318328840168));
#56510=CARTESIAN_POINT('Ctrl Pts',(57.3502261366816,28.3061791611239,17.4360576162331));
#56511=CARTESIAN_POINT('Ctrl Pts',(57.3732787291469,28.3842667628427,17.4402812932782));
#56512=CARTESIAN_POINT('Ctrl Pts',(57.3924183558645,28.4634466888392,17.4445049703233));
#56513=CARTESIAN_POINT('Ctrl Pts',(57.4075648795666,28.5432926531385,17.4487286473685));
#56514=CARTESIAN_POINT('Ctrl Pts',(57.4227388843736,28.6232834860138,17.4529599876447));
#56515=CARTESIAN_POINT('Ctrl Pts',(57.433905243613,28.7039423106955,17.4571913279209));
#56516=CARTESIAN_POINT('Ctrl Pts',(57.4410355852555,28.7848360589776,17.4614226681972));
#56517=CARTESIAN_POINT('Ctrl Pts',(57.4481454341668,28.8654973171592,17.4656418475247));
#56518=CARTESIAN_POINT('Ctrl Pts',(57.4512424993765,28.9463916922957,17.4698610268522));
#56519=CARTESIAN_POINT('Ctrl Pts',(57.4503502310631,29.0270923444712,17.4740802061797));
#56520=CARTESIAN_POINT('Ctrl Pts',(57.4494551215608,29.1080499662103,17.4783128203512));
#56521=CARTESIAN_POINT('Ctrl Pts',(57.4445418755774,29.1891137329985,17.4825454345226));
#56522=CARTESIAN_POINT('Ctrl Pts',(57.4355964344949,29.2698522897355,17.4867780486941));
#56523=CARTESIAN_POINT('Ctrl Pts',(57.4266637532443,29.3504756805022,17.4910046254389));
#56524=CARTESIAN_POINT('Ctrl Pts',(57.4137103509408,29.4307743246597,17.4952312021837));
#56525=CARTESIAN_POINT('Ctrl Pts',(57.3967741761517,29.5103173508045,17.4994577789285));
#56526=CARTESIAN_POINT('Ctrl Pts',(57.3798567985556,29.5897720934011,17.5036796646625));
#56527=CARTESIAN_POINT('Ctrl Pts',(57.3589655280866,29.6684724323045,17.5079015503966));
#56528=CARTESIAN_POINT('Ctrl Pts',(57.3341898884331,29.7459945138784,17.5121234361306));
#56529=CARTESIAN_POINT('Ctrl Pts',(57.3094309591802,29.8234643092124,17.5163424743336));
#56530=CARTESIAN_POINT('Ctrl Pts',(57.2807930051219,29.8997569841993,17.5205615125366));
#56531=CARTESIAN_POINT('Ctrl Pts',(57.2484159087534,29.9744619804101,17.5247805507397));
#56532=CARTESIAN_POINT('Ctrl Pts',(57.2160493855642,30.0491425806927,17.5289982111586));
#56533=CARTESIAN_POINT('Ctrl Pts',(57.1799463296203,30.1222361059529,17.5332158715776));
#56534=CARTESIAN_POINT('Ctrl Pts',(57.1402949563538,30.1933514779002,17.5374335319966));
#56535=CARTESIAN_POINT('Ctrl Pts',(57.1006444082174,30.2644653699635,17.5416511046476));
#56536=CARTESIAN_POINT('Ctrl Pts',(57.0574459168223,30.3336007853902,17.5458686772987));
#56537=CARTESIAN_POINT('Ctrl Pts',(57.0109332050363,30.4003920504211,17.5500862499497));
#56538=CARTESIAN_POINT('Ctrl Pts',(56.9643415353231,30.4672966973563,17.554310982166));
#56539=CARTESIAN_POINT('Ctrl Pts',(56.9144246556321,30.5318488489673,17.5585357143823));
#56540=CARTESIAN_POINT('Ctrl Pts',(56.8614594266659,30.5937123494774,17.5627604465986));
#56541=CARTESIAN_POINT('Ctrl Pts',(56.8085074263209,30.6555603989295,17.5669841236437));
#56542=CARTESIAN_POINT('Ctrl Pts',(56.7525089351073,30.7147208162159,17.5712078006888));
#56543=CARTESIAN_POINT('Ctrl Pts',(56.6937779056618,30.7708943097463,17.5754314777339));
#56544=CARTESIAN_POINT('Ctrl Pts',(56.6349403175358,30.8271697216904,17.5796628180102));
#56545=CARTESIAN_POINT('Ctrl Pts',(56.5733606355525,30.8804470747078,17.5838941582864));
#56546=CARTESIAN_POINT('Ctrl Pts',(56.5093866824929,30.9304668069441,17.5881254985627));
#56547=CARTESIAN_POINT('Ctrl Pts',(56.4455965917354,30.9803427815623,17.5923446778902));
#56548=CARTESIAN_POINT('Ctrl Pts',(56.3794263939126,31.0269796410378,17.5965638572177));
#56549=CARTESIAN_POINT('Ctrl Pts',(56.3112468994102,31.0701646839774,17.6007830365452));
#56550=CARTESIAN_POINT('Ctrl Pts',(56.2428503056097,31.1134872380936,17.6050156507167));
#56551=CARTESIAN_POINT('Ctrl Pts',(56.1721771979242,31.1534970634126,17.6092482648881));
#56552=CARTESIAN_POINT('Ctrl Pts',(56.099581754371,31.1899475371466,17.6134808790596));
#56553=CARTESIAN_POINT('Ctrl Pts',(56.0270898614016,31.2263460177023,17.6177074558044));
#56554=CARTESIAN_POINT('Ctrl Pts',(55.9526814902978,31.2591950236907,17.6219340325492));
#56555=CARTESIAN_POINT('Ctrl Pts',(55.8767387260929,31.2882918205878,17.626160609294));
#56556=CARTESIAN_POINT('Ctrl Pts',(55.8008802495623,31.3173563234097,17.630382495028));
#56557=CARTESIAN_POINT('Ctrl Pts',(55.7234911953972,31.34267672666,17.634604380762));
#56558=CARTESIAN_POINT('Ctrl Pts',(55.6449758394887,31.3640973788057,17.6388262664961));
#56559=CARTESIAN_POINT('Ctrl Pts',(55.5665134397529,31.3855035833857,17.6430453046991));
#56560=CARTESIAN_POINT('Ctrl Pts',(55.4869266940282,31.4030151388351,17.6472643429021));
#56561=CARTESIAN_POINT('Ctrl Pts',(55.4066361412256,31.4165258737802,17.6514833811051));
#56562=CARTESIAN_POINT('Ctrl Pts',(55.3263718083903,31.4300321966118,17.6557010415241));
#56563=CARTESIAN_POINT('Ctrl Pts',(55.2454045826773,31.4395402165839,17.659918701943));
#56564=CARTESIAN_POINT('Ctrl Pts',(55.1641649750556,31.4449949102125,17.664136362362));
#56565=CARTESIAN_POINT('Ctrl Pts',(55.0829270579994,31.450449490331,17.668353935013));
#56566=CARTESIAN_POINT('Ctrl Pts',(55.0014172338872,31.4518508818626,17.6725715076641));
#56567=CARTESIAN_POINT('Ctrl Pts',(54.9200694780109,31.4491960643555,17.6767890803151));
#56568=CARTESIAN_POINT('Ctrl Pts',(54.8385836297736,31.4465367401474,17.6810138125314));
#56569=CARTESIAN_POINT('Ctrl Pts',(54.7572608669687,31.4398074455723,17.6852385447477));
#56570=CARTESIAN_POINT('Ctrl Pts',(54.6765338887316,31.4290574148959,17.689463276964));
#56571=CARTESIAN_POINT('Ctrl Pts',(54.5958270729041,31.4183100691525,17.6936869540091));
#56572=CARTESIAN_POINT('Ctrl Pts',(54.5157161986539,31.4035441008954,17.6979106310542));
#56573=CARTESIAN_POINT('Ctrl Pts',(54.4366232353861,31.3848599269335,17.7021343080993));
#56574=CARTESIAN_POINT('Ctrl Pts',(54.35738676975,31.3661418533287,17.7063656483756));
#56575=CARTESIAN_POINT('Ctrl Pts',(54.2791723534683,31.3434914965236,17.7105969886518));
#56576=CARTESIAN_POINT('Ctrl Pts',(54.2023870685746,31.3170593133588,17.714828328928));
#56577=CARTESIAN_POINT('Ctrl Pts',(54.1258224659828,31.290703096768,17.7190475082555));
#56578=CARTESIAN_POINT('Ctrl Pts',(54.050679182682,31.2605870094316,17.7232666875831));
#56579=CARTESIAN_POINT('Ctrl Pts',(53.9773375074395,31.2269063016458,17.7274858669106));
#56580=CARTESIAN_POINT('Ctrl Pts',(53.9037622953201,31.1931183466874,17.7317184810821));
#56581=CARTESIAN_POINT('Ctrl Pts',(53.831726547693,31.1556173422235,17.7359510952536));
#56582=CARTESIAN_POINT('Ctrl Pts',(53.7616299527723,31.1145661200656,17.740183709425));
#56583=CARTESIAN_POINT('Ctrl Pts',(53.6916333440625,31.0735734536215,17.7444102861698));
#56584=CARTESIAN_POINT('Ctrl Pts',(53.6235707919222,31.0290408601542,17.7486368629146));
#56585=CARTESIAN_POINT('Ctrl Pts',(53.5578203625849,30.9811784733903,17.7528634396594));
#56586=CARTESIAN_POINT('Ctrl Pts',(53.4921429086105,30.9333692083335,17.7570853253934));
#56587=CARTESIAN_POINT('Ctrl Pts',(53.4287728521125,30.882237765319,17.7613072111275));
#56588=CARTESIAN_POINT('Ctrl Pts',(53.3680608456444,30.8280385243427,17.7655290968615));
#56589=CARTESIAN_POINT('Ctrl Pts',(53.3073897875418,30.7738758390736,17.7697481350645));
#56590=CARTESIAN_POINT('Ctrl Pts',(53.249373564519,30.7166497738978,17.7739671732676));
#56591=CARTESIAN_POINT('Ctrl Pts',(53.194330177525,30.6566552876815,17.7781862114706));
#56592=CARTESIAN_POINT('Ctrl Pts',(53.1393047656944,30.5966803934772,17.7824038718896));
#56593=CARTESIAN_POINT('Ctrl Pts',(53.08725057572,30.5339392156945,17.7866215323086));
#56594=CARTESIAN_POINT('Ctrl Pts',(53.0384481332066,30.4687629229658,17.7908391927275));
#56595=CARTESIAN_POINT('Ctrl Pts',(52.9896467062535,30.4035879865311,17.7950567653786));
#56596=CARTESIAN_POINT('Ctrl Pts',(52.944097169718,30.3359784084635,17.7992743380296));
#56597=CARTESIAN_POINT('Ctrl Pts',(52.9020383137302,30.2662965738498,17.8034919106807));
#56598=CARTESIAN_POINT('Ctrl Pts',(52.8599080604843,30.1964964504286,17.807716642897));
#56599=CARTESIAN_POINT('Ctrl Pts',(52.821280584898,30.124617432033,17.8119413751133));
#56600=CARTESIAN_POINT('Ctrl Pts',(52.7863501497853,30.0510492807878,17.8161661073296));
#56601=CARTESIAN_POINT('Ctrl Pts',(52.751428438915,29.9774995039597,17.8203897843747));
#56602=CARTESIAN_POINT('Ctrl Pts',(52.7202020810638,29.9022618766242,17.8246134614198));
#56603=CARTESIAN_POINT('Ctrl Pts',(52.6928165645635,29.8257450243552,17.8288371384649));
#56604=CARTESIAN_POINT('Ctrl Pts',(52.6653813611339,29.7490893436866,17.8330684787412));
#56605=CARTESIAN_POINT('Ctrl Pts',(52.6418010605464,29.6711502456553,17.8372998190174));
#56606=CARTESIAN_POINT('Ctrl Pts',(52.6221710715952,29.5923511097663,17.8415311592937));
#56607=CARTESIAN_POINT('Ctrl Pts',(52.6025974995886,29.5137784440243,17.8457503386212));
#56608=CARTESIAN_POINT('Ctrl Pts',(52.5869515693831,29.4343511400944,17.8499695179486));
#56609=CARTESIAN_POINT('Ctrl Pts',(52.5752765296161,29.3544944882071,17.8541886972761));
#56610=CARTESIAN_POINT('Ctrl Pts',(52.5582274655429,29.2378797955064,17.8603499661134));
#56611=CARTESIAN_POINT('Ctrl Pts',(52.5495884372501,29.1200064603412,17.8665112349507));
#56612=CARTESIAN_POINT('Ctrl Pts',(52.54950067561,29.001819660402,17.872672503788));
#56613=CARTESIAN_POINT('',(52.5495000568352,29.0005277777255,18.6726725037365));
#56614=CARTESIAN_POINT('Ctrl Pts',(52.5495006756093,29.0018196594696,17.8726725038366));
#56615=CARTESIAN_POINT('Ctrl Pts',(52.5494413295004,28.9218994314936,17.8768388744494));
#56616=CARTESIAN_POINT('Ctrl Pts',(52.5532959555911,28.8418332794805,17.8810052450622));
#56617=CARTESIAN_POINT('Ctrl Pts',(52.5610808602745,28.7620426931559,17.8851716156751));
#56618=CARTESIAN_POINT('Ctrl Pts',(52.5688560852825,28.6823513176769,17.8893328058628));
#56619=CARTESIAN_POINT('Ctrl Pts',(52.5805518371758,28.6029353014929,17.8934939960506));
#56620=CARTESIAN_POINT('Ctrl Pts',(52.5961323871062,28.5242156479242,17.8976551862384));
#56621=CARTESIAN_POINT('Ctrl Pts',(52.6117024114061,28.4455491743774,17.9018135652834));
#56622=CARTESIAN_POINT('Ctrl Pts',(52.6311519359377,28.3675785991837,17.9059719443284));
#56623=CARTESIAN_POINT('Ctrl Pts',(52.6543936213352,28.2907179923565,17.9101303233734));
#56624=CARTESIAN_POINT('Ctrl Pts',(52.6776272024671,28.2138841864583,17.9142872524113));
#56625=CARTESIAN_POINT('Ctrl Pts',(52.7046501817746,28.1381600393539,17.9184441814493));
#56626=CARTESIAN_POINT('Ctrl Pts',(52.7353249134837,28.0639460472215,17.9226011104873));
#56627=CARTESIAN_POINT('Ctrl Pts',(52.7659989747984,27.9897336770311,17.9267579486758));
#56628=CARTESIAN_POINT('Ctrl Pts',(52.8003244449853,27.9170318385339,17.9309147868643));
#56629=CARTESIAN_POINT('Ctrl Pts',(52.8381155503269,27.8462210453204,17.9350716250529));
#56630=CARTESIAN_POINT('Ctrl Pts',(52.8759426076556,27.7753428873473,17.9392324177855));
#56631=CARTESIAN_POINT('Ctrl Pts',(52.9172416560433,27.706359789992,17.9433932105182));
#56632=CARTESIAN_POINT('Ctrl Pts',(52.9617813453634,27.6396269019524,17.9475540032508));
#56633=CARTESIAN_POINT('Ctrl Pts',(53.0063433731053,27.5728605447213,17.9517168827861));
#56634=CARTESIAN_POINT('Ctrl Pts',(53.0541489895768,27.508347027116,17.9558797623214));
#56635=CARTESIAN_POINT('Ctrl Pts',(53.1049255277811,27.4464096438429,17.9600426418568));
#56636=CARTESIAN_POINT('Ctrl Pts',(53.1557875461254,27.3843679916224,17.9642125294225));
#56637=CARTESIAN_POINT('Ctrl Pts',(53.2096301480244,27.3249114858323,17.9683824169883));
#56638=CARTESIAN_POINT('Ctrl Pts',(53.2661430915665,27.2683272621314,17.972552304554));
#56639=CARTESIAN_POINT('Ctrl Pts',(53.3038158933783,27.2306069433592,17.9753320455832));
#56640=CARTESIAN_POINT('Ctrl Pts',(53.3426746141094,27.1941622340057,17.9781117866124));
#56641=CARTESIAN_POINT('Ctrl Pts',(53.3826196680679,27.1590678687471,17.9808915276415));
#56642=CARTESIAN_POINT('Ctrl Pts',(53.4434426007408,27.1056309096298,17.985124141813));
#56643=CARTESIAN_POINT('Ctrl Pts',(53.507029759057,27.0551121253094,17.9893567559845));
#56644=CARTESIAN_POINT('Ctrl Pts',(53.573069651168,27.0078102425768,17.9935893701559));
#56645=CARTESIAN_POINT('Ctrl Pts',(53.6390153435737,26.9605758315384,17.9978159469007));
#56646=CARTESIAN_POINT('Ctrl Pts',(53.7074064465877,26.916549476781,18.0020425236455));
#56647=CARTESIAN_POINT('Ctrl Pts',(53.7778970725188,26.8759908934654,18.0062691003903));
#56648=CARTESIAN_POINT('Ctrl Pts',(53.8483094620179,26.8354773254807,18.0104909861243));
#56649=CARTESIAN_POINT('Ctrl Pts',(53.920816343652,26.798424111841,18.0147128718583));
#56650=CARTESIAN_POINT('Ctrl Pts',(53.9950425833535,26.7650479108654,18.0189347575923));
#56651=CARTESIAN_POINT('Ctrl Pts',(54.069218759758,26.7316942211024,18.0231537957954));
#56652=CARTESIAN_POINT('Ctrl Pts',(54.1451115684634,26.7020128084663,18.0273728339984));
#56653=CARTESIAN_POINT('Ctrl Pts',(54.222322111688,26.6761739841308,18.0315918722014));
#56654=CARTESIAN_POINT('Ctrl Pts',(54.299507440764,26.6503435978133,18.0358095326203));
#56655=CARTESIAN_POINT('Ctrl Pts',(54.3780092095653,26.6283534550563,18.0400271930393));
#56656=CARTESIAN_POINT('Ctrl Pts',(54.457410711455,26.6103248936401,18.0442448534582));
#56657=CARTESIAN_POINT('Ctrl Pts',(54.5368105610295,26.5922967073915,18.0484624261093));
#56658=CARTESIAN_POINT('Ctrl Pts',(54.6171096531889,26.5782300402885,18.0526799987603));
#56659=CARTESIAN_POINT('Ctrl Pts',(54.6978797678661,26.5681953994337,18.0568975714114));
#56660=CARTESIAN_POINT('Ctrl Pts',(54.7787869943267,26.5581437242153,18.0611223036277));
#56661=CARTESIAN_POINT('Ctrl Pts',(54.8601663796607,26.5521378272465,18.065347035844));
#56662=CARTESIAN_POINT('Ctrl Pts',(54.9415828339573,26.5501963987471,18.0695717680603));
#56663=CARTESIAN_POINT('Ctrl Pts',(55.0229789536403,26.5482554551399,18.0737954451054));
#56664=CARTESIAN_POINT('Ctrl Pts',(55.1044116583295,26.5503769165849,18.0780191221505));
#56665=CARTESIAN_POINT('Ctrl Pts',(55.1854484935347,26.5565272446279,18.0822427991956));
#56666=CARTESIAN_POINT('Ctrl Pts',(55.2666323579732,26.5626887315225,18.0864741394718));
#56667=CARTESIAN_POINT('Ctrl Pts',(55.347418455313,26.5728936349655,18.090705479748));
#56668=CARTESIAN_POINT('Ctrl Pts',(55.4273812512561,26.5870566695269,18.0949368200243));
#56669=CARTESIAN_POINT('Ctrl Pts',(55.507114232674,26.6011789992701,18.0991559993518));
#56670=CARTESIAN_POINT('Ctrl Pts',(55.5860282135153,26.6192365564029,18.1033751786794));
#56671=CARTESIAN_POINT('Ctrl Pts',(55.6637171569014,26.6410956387266,18.107594358007));
#56672=CARTESIAN_POINT('Ctrl Pts',(55.7416534798717,26.6630243254298,18.1118269721784));
#56673=CARTESIAN_POINT('Ctrl Pts',(55.8186468108733,26.6888603710492,18.1160595863499));
#56674=CARTESIAN_POINT('Ctrl Pts',(55.8942769939244,26.7185051154698,18.1202922005214));
#56675=CARTESIAN_POINT('Ctrl Pts',(55.9697992976208,26.748107574446,18.1245187772662));
#56676=CARTESIAN_POINT('Ctrl Pts',(56.0439618862847,26.7815077739578,18.128745354011));
#56677=CARTESIAN_POINT('Ctrl Pts',(56.1163586027489,26.8185569638268,18.1329719307557));
#56678=CARTESIAN_POINT('Ctrl Pts',(56.1886749672412,26.8555650333853,18.1371938164898));
#56679=CARTESIAN_POINT('Ctrl Pts',(56.2592289424201,26.8962138354806,18.1414157022238));
#56680=CARTESIAN_POINT('Ctrl Pts',(56.3276345665331,26.9403066471568,18.1456375879578));
#56681=CARTESIAN_POINT('Ctrl Pts',(56.3959940531739,26.9843697195989,18.1498566261608));
#56682=CARTESIAN_POINT('Ctrl Pts',(56.4622076771272,27.0318719371499,18.1540756643639));
#56683=CARTESIAN_POINT('Ctrl Pts',(56.5259154168102,27.0825714118276,18.1582947025669));
#56684=CARTESIAN_POINT('Ctrl Pts',(56.5896023518681,27.1332543299053,18.1625123629859));
#56685=CARTESIAN_POINT('Ctrl Pts',(56.6507846645958,27.1871321425254,18.1667300234048));
#56686=CARTESIAN_POINT('Ctrl Pts',(56.7091337183731,27.2439213620342,18.1709476838238));
#56687=CARTESIAN_POINT('Ctrl Pts',(56.7674815579286,27.3007093997806,18.1751652564748));
#56688=CARTESIAN_POINT('Ctrl Pts',(56.822995923674,27.3604083991097,18.1793828291259));
#56689=CARTESIAN_POINT('Ctrl Pts',(56.8753845491235,27.4226975423499,18.1836004017769));
#56690=CARTESIAN_POINT('Ctrl Pts',(56.9278621071921,27.4850924248915,18.1878251339932));
#56691=CARTESIAN_POINT('Ctrl Pts',(56.9772030080718,27.5500858911485,18.1920498662095));
#56692=CARTESIAN_POINT('Ctrl Pts',(57.0231547106364,27.6173231516983,18.1962745984258));
#56693=CARTESIAN_POINT('Ctrl Pts',(57.0690949362814,27.684543619037,18.2004982754709));
#56694=CARTESIAN_POINT('Ctrl Pts',(57.1116474309916,27.7540063513879,18.204721952516));
#56695=CARTESIAN_POINT('Ctrl Pts',(57.1506048990952,27.825330336653,18.2089456295611));
#56696=CARTESIAN_POINT('Ctrl Pts',(57.1896330497057,27.896783728636,18.2131769698373));
#56697=CARTESIAN_POINT('Ctrl Pts',(57.2250529357812,27.9701047027709,18.2174083101136));
#56698=CARTESIAN_POINT('Ctrl Pts',(57.2567044356771,28.0448898806968,18.2216396503898));
#56699=CARTESIAN_POINT('Ctrl Pts',(57.2882649685881,28.1194601246646,18.2258588297173));
#56700=CARTESIAN_POINT('Ctrl Pts',(57.316078668915,28.1954857112511,18.2300780090449));
#56701=CARTESIAN_POINT('Ctrl Pts',(57.3400366426309,28.2725532588947,18.2342971883724));
#56702=CARTESIAN_POINT('Ctrl Pts',(57.3640709040827,28.3498662074554,18.2385298025439));
#56703=CARTESIAN_POINT('Ctrl Pts',(57.384314208715,28.4285153199078,18.2427624167154));
#56704=CARTESIAN_POINT('Ctrl Pts',(57.4006205818658,28.5080944481689,18.2469950308868));
#56705=CARTESIAN_POINT('Ctrl Pts',(57.4169036955065,28.5875600642757,18.2512216076316));
#56706=CARTESIAN_POINT('Ctrl Pts',(57.4292609386188,28.6679526101207,18.2554481843764));
#56707=CARTESIAN_POINT('Ctrl Pts',(57.4375959743156,28.7488504111088,18.2596747611212));
#56708=CARTESIAN_POINT('Ctrl Pts',(57.445921759088,28.8296584249054,18.2638966468553));
#56709=CARTESIAN_POINT('Ctrl Pts',(57.450234159399,28.9109701198137,18.2681185325893));
#56710=CARTESIAN_POINT('Ctrl Pts',(57.4504880735377,28.9923546452433,18.2723404183233));
#56711=CARTESIAN_POINT('Ctrl Pts',(57.4507418164192,29.0736842793345,18.2765594565263));
#56712=CARTESIAN_POINT('Ctrl Pts',(57.4469425082454,29.1550861830391,18.2807784947294));
#56713=CARTESIAN_POINT('Ctrl Pts',(57.439097054718,29.2361266771583,18.2849975329324));
#56714=CARTESIAN_POINT('Ctrl Pts',(57.4312541632297,29.3171407064068,18.2892151933514));
#56715=CARTESIAN_POINT('Ctrl Pts',(57.4193677951843,29.3977930984244,18.2934328537704));
#56716=CARTESIAN_POINT('Ctrl Pts',(57.4034968371366,29.4776538536161,18.2976505141893));
#56717=CARTESIAN_POINT('Ctrl Pts',(57.3876262093575,29.5575129469358,18.3018680868404));
#56718=CARTESIAN_POINT('Ctrl Pts',(57.36777124814,29.636579980775,18.3060856594915));
#56719=CARTESIAN_POINT('Ctrl Pts',(57.34404195333,29.7144351412331,18.3103032321425));
#56720=CARTESIAN_POINT('Ctrl Pts',(57.3202723767163,29.7924224651759,18.3145279643588));
#56721=CARTESIAN_POINT('Ctrl Pts',(57.2926154438239,29.8691933530088,18.3187526965751));
#56722=CARTESIAN_POINT('Ctrl Pts',(57.2612312773784,29.9443428192165,18.3229774287914));
#56723=CARTESIAN_POINT('Ctrl Pts',(57.2298549494574,30.0194735160572,18.3272011058365));
#56724=CARTESIAN_POINT('Ctrl Pts',(57.1947534696254,30.0929831896066,18.3314247828816));
#56725=CARTESIAN_POINT('Ctrl Pts',(57.1561335885112,30.1644905317322,18.3356484599267));
#56726=CARTESIAN_POINT('Ctrl Pts',(57.1174436373911,30.2361276132495,18.339879800203));
#56727=CARTESIAN_POINT('Ctrl Pts',(57.0752227691256,30.3057547046768,18.3441111404792));
#56728=CARTESIAN_POINT('Ctrl Pts',(57.0297221773078,30.3730178924344,18.3483424807555));
#56729=CARTESIAN_POINT('Ctrl Pts',(56.984352355017,30.440087764569,18.352561660083));
#56730=CARTESIAN_POINT('Ctrl Pts',(56.9357219759435,30.5048069887044,18.3567808394104));
#56731=CARTESIAN_POINT('Ctrl Pts',(56.8841185129737,30.566859176528,18.3610000187379));
#56732=CARTESIAN_POINT('Ctrl Pts',(56.832350732628,30.6291089528869,18.3652326329094));
#56733=CARTESIAN_POINT('Ctrl Pts',(56.777398344353,30.6889061877296,18.3694652470808));
#56734=CARTESIAN_POINT('Ctrl Pts',(56.7195225666831,30.7459073264832,18.3736978612523));
#56735=CARTESIAN_POINT('Ctrl Pts',(56.6617293433756,30.8028271584646,18.3779244379971));
#56736=CARTESIAN_POINT('Ctrl Pts',(56.6010213409389,30.8569584925041,18.3821510147419));
#56737=CARTESIAN_POINT('Ctrl Pts',(56.5376998247819,30.9079909588009,18.3863775914867));
#56738=CARTESIAN_POINT('Ctrl Pts',(56.4744485881753,30.9589667849695,18.3905994772207));
#56739=CARTESIAN_POINT('Ctrl Pts',(56.408589961409,31.006850287408,18.3948213629547));
#56740=CARTESIAN_POINT('Ctrl Pts',(56.3404607994197,31.0513690782546,18.3990432486887));
#56741=CARTESIAN_POINT('Ctrl Pts',(56.2723775884375,31.0958578425572,18.4032622868918));
#56742=CARTESIAN_POINT('Ctrl Pts',(56.2020272716181,31.1369861490226,18.4074813250948));
#56743=CARTESIAN_POINT('Ctrl Pts',(56.1297773894836,31.1745236950219,18.4117003632978));
#56744=CARTESIAN_POINT('Ctrl Pts',(56.0575511015265,31.2120489826272,18.4159180237168));
#56745=CARTESIAN_POINT('Ctrl Pts',(55.983426892104,31.24598562449,18.4201356841357));
#56746=CARTESIAN_POINT('Ctrl Pts',(55.9077975136121,31.2761489240117,18.4243533445547));
#56747=CARTESIAN_POINT('Ctrl Pts',(55.8321697089388,31.3063115958466,18.4285709172057));
#56748=CARTESIAN_POINT('Ctrl Pts',(55.7550372294031,31.3327009104592,18.4327884898568));
#56749=CARTESIAN_POINT('Ctrl Pts',(55.6768121095004,31.3551805914693,18.4370060625078));
#56750=CARTESIAN_POINT('Ctrl Pts',(55.5984541980857,31.3776984329939,18.4412307947241));
#56751=CARTESIAN_POINT('Ctrl Pts',(55.5190003840752,31.3962932332051,18.4454555269404));
#56752=CARTESIAN_POINT('Ctrl Pts',(55.4388775504767,31.4108788326433,18.4496802591567));
#56753=CARTESIAN_POINT('Ctrl Pts',(55.3587747283963,31.4254607891751,18.4539039362018));
#56754=CARTESIAN_POINT('Ctrl Pts',(55.278003685843,31.4360355079212,18.4581276132469));
#56755=CARTESIAN_POINT('Ctrl Pts',(55.1969968289068,31.4425688320702,18.462351290292));
#56756=CARTESIAN_POINT('Ctrl Pts',(55.1158429971282,31.44911400996,18.4665826305683));
#56757=CARTESIAN_POINT('Ctrl Pts',(55.0344529616031,31.4516031252468,18.4708139708445));
#56758=CARTESIAN_POINT('Ctrl Pts',(54.953260343965,31.4500542146152,18.4750453111207));
#56759=CARTESIAN_POINT('Ctrl Pts',(54.8723010753831,31.4485097555809,18.4792644904482));
#56760=CARTESIAN_POINT('Ctrl Pts',(54.7915385399024,31.4429505645957,18.4834836697758));
#56761=CARTESIAN_POINT('Ctrl Pts',(54.7113946324922,31.4334455391164,18.4877028491033));
#56762=CARTESIAN_POINT('Ctrl Pts',(54.630995528323,31.4239102474351,18.4919354632748));
#56763=CARTESIAN_POINT('Ctrl Pts',(54.5509199747245,31.4103684607044,18.4961680774462));
#56764=CARTESIAN_POINT('Ctrl Pts',(54.4715983615203,31.3928522642344,18.5004006916177));
#56765=CARTESIAN_POINT('Ctrl Pts',(54.3923898931491,31.375361052974,18.5046272683625));
#56766=CARTESIAN_POINT('Ctrl Pts',(54.31393367909,31.3539067909197,18.5088538451073));
#56767=CARTESIAN_POINT('Ctrl Pts',(54.2366540744935,31.328573221527,18.5130804218521));
#56768=CARTESIAN_POINT('Ctrl Pts',(54.1594602413094,31.3032677694628,18.5173023075861));
#56769=CARTESIAN_POINT('Ctrl Pts',(54.0834408619762,31.274091709223,18.5215241933202));
#56770=CARTESIAN_POINT('Ctrl Pts',(54.0090078064033,31.241179315055,18.5257460790542));
#56771=CARTESIAN_POINT('Ctrl Pts',(53.9346249536182,31.2082891192762,18.5299651172572));
#56772=CARTESIAN_POINT('Ctrl Pts',(53.8618267233971,31.171667781972,18.5341841554602));
#56773=CARTESIAN_POINT('Ctrl Pts',(53.7910063887513,31.1314982284674,18.5384031936632));
#56774=CARTESIAN_POINT('Ctrl Pts',(53.7202091814448,31.0913417928746,18.5426208540822));
#56775=CARTESIAN_POINT('Ctrl Pts',(53.6513889907435,31.0476396712413,18.5468385145012));
#56776=CARTESIAN_POINT('Ctrl Pts',(53.5849145595345,31.0006207652083,18.5510561749201));
#56777=CARTESIAN_POINT('Ctrl Pts',(53.5184415116332,30.9536028376208,18.5552737475712));
#56778=CARTESIAN_POINT('Ctrl Pts',(53.4543145047537,30.9032685320856,18.5594913202222));
#56779=CARTESIAN_POINT('Ctrl Pts',(53.3928721628732,30.8498892845606,18.5637088928733));
#56780=CARTESIAN_POINT('Ctrl Pts',(53.3313255191841,30.7964194227802,18.5679336250896));
#56781=CARTESIAN_POINT('Ctrl Pts',(53.2724730112602,30.7398945834016,18.5721583573059));
#56782=CARTESIAN_POINT('Ctrl Pts',(53.2166193072832,30.6806259413817,18.5763830895222));
#56783=CARTESIAN_POINT('Ctrl Pts',(53.1607795533546,30.6213721023266,18.5806067665673));
#56784=CARTESIAN_POINT('Ctrl Pts',(53.1079373918087,30.5593761996001,18.5848304436124));
#56785=CARTESIAN_POINT('Ctrl Pts',(53.0583568764645,30.4949823513431,18.5890541206575));
#56786=CARTESIAN_POINT('Ctrl Pts',(53.0086864046808,30.4304716700666,18.5932854609337));
#56787=CARTESIAN_POINT('Ctrl Pts',(52.9622896710225,30.3635547313774,18.59751680121));
#56788=CARTESIAN_POINT('Ctrl Pts',(52.9193876098304,30.2946050872265,18.6017481414862));
#56789=CARTESIAN_POINT('Ctrl Pts',(52.8766088499405,30.225853605604,18.6059673208138));
#56790=CARTESIAN_POINT('Ctrl Pts',(52.8373048501513,30.1550815253587,18.6101865001413));
#56791=CARTESIAN_POINT('Ctrl Pts',(52.8016474974991,30.0826802504655,18.6144056794688));
#56792=CARTESIAN_POINT('Ctrl Pts',(52.7633087932116,30.0048345647455,18.6189421314637));
#56793=CARTESIAN_POINT('Ctrl Pts',(52.7290586323875,29.9248486151305,18.6234785834587));
#56794=CARTESIAN_POINT('Ctrl Pts',(52.6991232085006,29.8431584906405,18.6280150354536));
#56795=CARTESIAN_POINT('Ctrl Pts',(52.6692884075535,29.7617429538938,18.632536238921));
#56796=CARTESIAN_POINT('Ctrl Pts',(52.6437395674428,29.6786349946326,18.6370574423884));
#56797=CARTESIAN_POINT('Ctrl Pts',(52.6226552075422,29.5942911641392,18.6415786458558));
#56798=CARTESIAN_POINT('Ctrl Pts',(52.6016158173398,29.5101272260691,18.6460902062913));
#56799=CARTESIAN_POINT('Ctrl Pts',(52.5850220414241,29.4247330115307,18.6506017667268));
#56800=CARTESIAN_POINT('Ctrl Pts',(52.5730034217597,29.3385821306712,18.6551133271622));
#56801=CARTESIAN_POINT('Ctrl Pts',(52.5610198208791,29.2526822685771,18.6596117422147));
#56802=CARTESIAN_POINT('Ctrl Pts',(52.5535848700389,29.1660304884529,18.6641101572671));
#56803=CARTESIAN_POINT('Ctrl Pts',(52.5507773309078,29.0791111067095,18.6686085723195));
#56804=CARTESIAN_POINT('Ctrl Pts',(52.5499318741305,29.0529363761211,18.6699632161252));
#56805=CARTESIAN_POINT('Ctrl Pts',(52.5495057017596,29.026737460879,18.6713178599309));
#56806=CARTESIAN_POINT('Ctrl Pts',(52.5495000568352,29.0005277777256,18.6726725037366));
#56807=CARTESIAN_POINT('',(52.5495009896071,28.9977977140258,19.4726725037492));
#56808=CARTESIAN_POINT('Ctrl Pts',(52.549500056835,29.0005277767301,18.672672503788));
#56809=CARTESIAN_POINT('Ctrl Pts',(52.5494819283997,28.916356332626,18.6770228930965));
#56810=CARTESIAN_POINT('Ctrl Pts',(52.5538049015165,28.8322364052644,18.6813732824049));
#56811=CARTESIAN_POINT('Ctrl Pts',(52.5624270296726,28.7486272402795,18.6857236717134));
#56812=CARTESIAN_POINT('Ctrl Pts',(52.5710574791649,28.664937382924,18.6900782596432));
#56813=CARTESIAN_POINT('Ctrl Pts',(52.5839953011645,28.581759688051,18.6944328475731));
#56814=CARTESIAN_POINT('Ctrl Pts',(52.6011471071535,28.4995451583989,18.6987874355029));
#56815=CARTESIAN_POINT('Ctrl Pts',(52.6183331992217,28.4171662837284,18.7031507281573));
#56816=CARTESIAN_POINT('Ctrl Pts',(52.639750009848,28.33575483198,18.7075140208117));
#56817=CARTESIAN_POINT('Ctrl Pts',(52.665253688106,28.255748759425,18.711877313466));
#56818=CARTESIAN_POINT('Ctrl Pts',(52.6907866110946,28.1756509449646,18.7162456094504));
#56819=CARTESIAN_POINT('Ctrl Pts',(52.720415592244,28.096962114604,18.7206139054347));
#56820=CARTESIAN_POINT('Ctrl Pts',(52.753948715331,28.0201000680494,18.7249822014191));
#56821=CARTESIAN_POINT('Ctrl Pts',(52.787551620376,27.9430780726558,18.729359587766));
#56822=CARTESIAN_POINT('Ctrl Pts',(52.8250747045283,27.8678908291701,18.733736974113));
#56823=CARTESIAN_POINT('Ctrl Pts',(52.8662802307517,27.794931455759,18.7381143604599));
#56824=CARTESIAN_POINT('Ctrl Pts',(52.8756751444272,27.778296623545,18.7391124102513));
#56825=CARTESIAN_POINT('Ctrl Pts',(52.8852613138506,27.7617774819803,18.7401104600428));
#56826=CARTESIAN_POINT('Ctrl Pts',(52.8950356178758,27.7453784634447,18.7411085098342));
#56827=CARTESIAN_POINT('Ctrl Pts',(52.9364873150637,27.6758321153096,18.7453411240057));
#56828=CARTESIAN_POINT('Ctrl Pts',(52.9814664335564,27.6082129377665,18.7495737381772));
#56829=CARTESIAN_POINT('Ctrl Pts',(53.0297683907496,27.5429009450588,18.7538063523487));
#56830=CARTESIAN_POINT('Ctrl Pts',(53.0780014497362,27.4776821137761,18.7580329290935));
#56831=CARTESIAN_POINT('Ctrl Pts',(53.1295476598027,27.4147643014129,18.7622595058383));
#56832=CARTESIAN_POINT('Ctrl Pts',(53.1841577158776,27.3545009725943,18.7664860825831));
#56833=CARTESIAN_POINT('Ctrl Pts',(53.2387071611137,27.2943045290927,18.7707079683171));
#56834=CARTESIAN_POINT('Ctrl Pts',(53.2963133851737,27.2367570576029,18.7749298540511));
#56835=CARTESIAN_POINT('Ctrl Pts',(53.3566860171766,27.1821800408575,18.7791517397851));
#56836=CARTESIAN_POINT('Ctrl Pts',(53.4170179297115,27.1276398346173,18.7833707779882));
#56837=CARTESIAN_POINT('Ctrl Pts',(53.4801122007157,27.0760664147599,18.7875898161912));
#56838=CARTESIAN_POINT('Ctrl Pts',(53.5456415992744,27.0277444657857,18.7918088543942));
#56839=CARTESIAN_POINT('Ctrl Pts',(53.6111495983205,26.9794382969984,18.7960265148132));
#56840=CARTESIAN_POINT('Ctrl Pts',(53.6790907720557,26.9343817658965,18.8002441752322));
#56841=CARTESIAN_POINT('Ctrl Pts',(53.7491058887694,26.8928184291598,18.8044618356511));
#56842=CARTESIAN_POINT('Ctrl Pts',(53.819119548495,26.8512559573404,18.8086794083022));
#56843=CARTESIAN_POINT('Ctrl Pts',(53.8912066653263,26.8131867714811,18.8128969809532));
#56844=CARTESIAN_POINT('Ctrl Pts',(53.9649814264467,26.7788095978958,18.8171145536043));
#56845=CARTESIAN_POINT('Ctrl Pts',(54.0388814243465,26.7443740671375,18.8213392858206));
#56846=CARTESIAN_POINT('Ctrl Pts',(54.1144743751778,26.7136432854959,18.8255640180369));
#56847=CARTESIAN_POINT('Ctrl Pts',(54.191352000615,26.686768783046,18.8297887502531));
#56848=CARTESIAN_POINT('Ctrl Pts',(54.2682104250593,26.6599009927848,18.8340124272983));
#56849=CARTESIAN_POINT('Ctrl Pts',(54.3463524292999,26.6368876669712,18.8382361043434));
#56850=CARTESIAN_POINT('Ctrl Pts',(54.4253561879548,26.6178298257097,18.8424597813885));
#56851=CARTESIAN_POINT('Ctrl Pts',(54.5045032871294,26.5987374068419,18.8466911216648));
#56852=CARTESIAN_POINT('Ctrl Pts',(54.5845148075763,26.5836149013123,18.850922461941));
#56853=CARTESIAN_POINT('Ctrl Pts',(54.6649596022408,26.5725119605095,18.8551538022173));
#56854=CARTESIAN_POINT('Ctrl Pts',(54.7451731971052,26.5614409297601,18.8593729815447));
#56855=CARTESIAN_POINT('Ctrl Pts',(54.8258171182594,26.5543663469128,18.8635921608722));
#56856=CARTESIAN_POINT('Ctrl Pts',(54.9064638889266,26.5512857974183,18.8678113401997));
#56857=CARTESIAN_POINT('Ctrl Pts',(54.9873674575863,26.5481954387409,18.8720439543712));
#56858=CARTESIAN_POINT('Ctrl Pts',(55.0685747979384,26.5491131232658,18.8762765685427));
#56859=CARTESIAN_POINT('Ctrl Pts',(55.1496557695137,26.5540741220039,18.8805091827141));
#56860=CARTESIAN_POINT('Ctrl Pts',(55.2306210866964,26.559028044343,18.8847357594589));
#56861=CARTESIAN_POINT('Ctrl Pts',(55.3114599332799,26.568013797945,18.8889623362037));
#56862=CARTESIAN_POINT('Ctrl Pts',(55.3917400923376,26.5810146858537,18.8931889129485));
#56863=CARTESIAN_POINT('Ctrl Pts',(55.471931149715,26.5940011442824,18.8974107986825));
#56864=CARTESIAN_POINT('Ctrl Pts',(55.5515642953984,26.610993808402,18.9016326844165));
#56865=CARTESIAN_POINT('Ctrl Pts',(55.63021178342,26.6319241232514,18.9058545701506));
#56866=CARTESIAN_POINT('Ctrl Pts',(55.7088062261496,26.6528403212524,18.9100736083536));
#56867=CARTESIAN_POINT('Ctrl Pts',(55.7864158837948,26.6776887761234,18.9142926465566));
#56868=CARTESIAN_POINT('Ctrl Pts',(55.8626238110411,26.7063499807894,18.9185116847596));
#56869=CARTESIAN_POINT('Ctrl Pts',(55.9388068515567,26.7350018257508,18.9227293451786));
#56870=CARTESIAN_POINT('Ctrl Pts',(56.0135886362644,26.7674637844002,18.9269470055975));
#56871=CARTESIAN_POINT('Ctrl Pts',(56.086569297644,26.8035671165689,18.9311646660165));
#56872=CARTESIAN_POINT('Ctrl Pts',(56.1595484403236,26.8396696974409,18.9353822386675));
#56873=CARTESIAN_POINT('Ctrl Pts',(56.2307261183335,26.8794132941344,18.9395998113186));
#56874=CARTESIAN_POINT('Ctrl Pts',(56.2997255982198,26.9225824638913,18.9438173839696));
#56875=CARTESIAN_POINT('Ctrl Pts',(56.368842208579,26.9658249157261,18.9480421161859));
#56876=CARTESIAN_POINT('Ctrl Pts',(56.4357728268587,27.0125043275949,18.9522668484022));
#56877=CARTESIAN_POINT('Ctrl Pts',(56.5001680787598,27.0623607184333,18.9564915806185));
#56878=CARTESIAN_POINT('Ctrl Pts',(56.5645472472712,27.1122046571151,18.9607152576636));
#56879=CARTESIAN_POINT('Ctrl Pts',(56.6263919756417,27.1652236684644,18.9649389347087));
#56880=CARTESIAN_POINT('Ctrl Pts',(56.6853878835814,27.2211189101356,18.9691626117538));
#56881=CARTESIAN_POINT('Ctrl Pts',(56.744490830784,27.2771155653741,18.97339395203));
#56882=CARTESIAN_POINT('Ctrl Pts',(56.8007343061655,27.335998543005,18.9776252923063));
#56883=CARTESIAN_POINT('Ctrl Pts',(56.8538419440844,27.397433216258,18.9818566325825));
#56884=CARTESIAN_POINT('Ctrl Pts',(56.9067969496889,27.458691325146,18.9860758119101));
#56885=CARTESIAN_POINT('Ctrl Pts',(56.9566339039521,27.5224860720422,18.9902949912376));
#56886=CARTESIAN_POINT('Ctrl Pts',(57.0031221135569,27.5884575641593,18.9945141705652));
#56887=CARTESIAN_POINT('Ctrl Pts',(57.0497583523855,27.654639124783,18.9987467847366));
#56888=CARTESIAN_POINT('Ctrl Pts',(57.0931979170176,27.7232574787165,19.0029793989081));
#56889=CARTESIAN_POINT('Ctrl Pts',(57.1331770524215,27.7939710148498,19.0072120130796));
#56890=CARTESIAN_POINT('Ctrl Pts',(57.1730991613426,27.8645836847635,19.0114385898244));
#56891=CARTESIAN_POINT('Ctrl Pts',(57.2095704177916,27.9372852001382,19.0156651665692));
#56892=CARTESIAN_POINT('Ctrl Pts',(57.2423695283531,28.011703916676,19.0198917433139));
#56893=CARTESIAN_POINT('Ctrl Pts',(57.2751322356999,28.0860400370559,19.024113629048));
#56894=CARTESIAN_POINT('Ctrl Pts',(57.304230709071,28.1620891486405,19.028335514782));
#56895=CARTESIAN_POINT('Ctrl Pts',(57.3294895888474,28.2394551259447,19.032557400516));
#56896=CARTESIAN_POINT('Ctrl Pts',(57.3547314322926,28.3167689222964,19.036776438719));
#56897=CARTESIAN_POINT('Ctrl Pts',(57.3761386816807,28.395397379886,19.0409954769221));
#56898=CARTESIAN_POINT('Ctrl Pts',(57.3935845971956,28.4749256947176,19.0452145151251));
#56899=CARTESIAN_POINT('Ctrl Pts',(57.4110248155106,28.554428038501,19.049432175544));
#56900=CARTESIAN_POINT('Ctrl Pts',(57.4245061695532,28.6348292025262,19.053649835963));
#56901=CARTESIAN_POINT('Ctrl Pts',(57.4339525146333,28.715701905546,19.057867496382));
#56902=CARTESIAN_POINT('Ctrl Pts',(57.4433986631386,28.7965729256356,19.062085069033));
#56903=CARTESIAN_POINT('Ctrl Pts',(57.4488099169007,28.8779150036628,19.0663026416841));
#56904=CARTESIAN_POINT('Ctrl Pts',(57.4501619007443,28.9592948388912,19.0705202143351));
#56905=CARTESIAN_POINT('Ctrl Pts',(57.451516179656,29.0408128209371,19.0747449465514));
#56906=CARTESIAN_POINT('Ctrl Pts',(57.4487973939351,29.1223682214935,19.0789696787677));
#56907=CARTESIAN_POINT('Ctrl Pts',(57.4420334226068,29.2035264426833,19.083194410984));
#56908=CARTESIAN_POINT('Ctrl Pts',(57.4352711406513,29.2846643937561,19.0874180880291));
#56909=CARTESIAN_POINT('Ctrl Pts',(57.4244657763874,29.3654049046216,19.0916417650742));
#56910=CARTESIAN_POINT('Ctrl Pts',(57.40969685743,29.4453215751475,19.0958654421193));
#56911=CARTESIAN_POINT('Ctrl Pts',(57.3949011424752,29.5253832425355,19.1000967823955));
#56912=CARTESIAN_POINT('Ctrl Pts',(57.3761276087181,29.6046176290603,19.1043281226718));
#56913=CARTESIAN_POINT('Ctrl Pts',(57.3535064958576,29.6826107411665,19.108559462948));
#56914=CARTESIAN_POINT('Ctrl Pts',(57.3309503964859,29.7603796996537,19.1127786422755));
#56915=CARTESIAN_POINT('Ctrl Pts',(57.304569031496,29.8369141057922,19.116997821603));
#56916=CARTESIAN_POINT('Ctrl Pts',(57.2745386984091,29.9118245222845,19.1212170009306));
#56917=CARTESIAN_POINT('Ctrl Pts',(57.2444127417879,29.986973470889,19.125449615102));
#56918=CARTESIAN_POINT('Ctrl Pts',(57.2105024694546,30.0607675607763,19.1296822292735));
#56919=CARTESIAN_POINT('Ctrl Pts',(57.1729508449742,30.132799574208,19.133914843445));
#56920=CARTESIAN_POINT('Ctrl Pts',(57.1354527843602,30.2047288407361,19.1381414201898));
#56921=CARTESIAN_POINT('Ctrl Pts',(57.0943239006092,30.2749006143076,19.1423679969346));
#56922=CARTESIAN_POINT('Ctrl Pts',(57.0497554660202,30.3429269449677,19.1465945736794));
#56923=CARTESIAN_POINT('Ctrl Pts',(57.0052364972329,30.4108777742778,19.1508164594134));
#56924=CARTESIAN_POINT('Ctrl Pts',(56.957285816278,30.4766875054828,19.1550383451475));
#56925=CARTESIAN_POINT('Ctrl Pts',(56.9061402372876,30.5399933914771,19.1592602308815));
#56926=CARTESIAN_POINT('Ctrl Pts',(56.8550291544041,30.6032565796147,19.1634792690845));
#56927=CARTESIAN_POINT('Ctrl Pts',(56.8007277444122,30.6640189161582,19.1676983072875));
#56928=CARTESIAN_POINT('Ctrl Pts',(56.7435149581103,30.7219482689226,19.1719173454906));
#56929=CARTESIAN_POINT('Ctrl Pts',(56.6863208554184,30.7798587040725,19.1761350059096));
#56930=CARTESIAN_POINT('Ctrl Pts',(56.626217590731,30.8349376624633,19.1803526663285));
#56931=CARTESIAN_POINT('Ctrl Pts',(56.5635221251068,30.8868886597523,19.1845703267475));
#56932=CARTESIAN_POINT('Ctrl Pts',(56.5008279641517,30.9388385759604,19.1887878993986));
#56933=CARTESIAN_POINT('Ctrl Pts',(56.4355420679637,30.9876603649891,19.1930054720496));
#56934=CARTESIAN_POINT('Ctrl Pts',(56.3680146302662,31.0330976910561,19.1972230447007));
#56935=CARTESIAN_POINT('Ctrl Pts',(56.3003725609702,31.0786121495228,19.2014477769169));
#56936=CARTESIAN_POINT('Ctrl Pts',(56.2304817244137,31.1207303892901,19.2056725091332));
#56937=CARTESIAN_POINT('Ctrl Pts',(56.1587218496236,31.1592392005531,19.2098972413495));
#56938=CARTESIAN_POINT('Ctrl Pts',(56.0869798976145,31.1977383938366,19.2141209183946));
#56939=CARTESIAN_POINT('Ctrl Pts',(56.0133702712092,31.2326297809141,19.2183445954397));
#56940=CARTESIAN_POINT('Ctrl Pts',(55.9382939404934,31.2637479389794,19.2225682724848));
#56941=CARTESIAN_POINT('Ctrl Pts',(55.8630813949891,31.2949225562946,19.2267996127611));
#56942=CARTESIAN_POINT('Ctrl Pts',(55.7863972657798,31.3223101064796,19.2310309530373));
#56943=CARTESIAN_POINT('Ctrl Pts',(55.708659723701,31.3457944594538,19.2352622933136));
#56944=CARTESIAN_POINT('Ctrl Pts',(55.6311456007294,31.3692113179712,19.239481472641));
#56945=CARTESIAN_POINT('Ctrl Pts',(55.5525845737257,31.3887473558927,19.2437006519685));
#56946=CARTESIAN_POINT('Ctrl Pts',(55.4733992890323,31.4043384460478,19.247919831296));
#56947=CARTESIAN_POINT('Ctrl Pts',(55.3939618600558,31.4199791818443,19.2521524454675));
#56948=CARTESIAN_POINT('Ctrl Pts',(55.313600736226,31.431707951975,19.2563850596389));
#56949=CARTESIAN_POINT('Ctrl Pts',(55.232735331535,31.4394229882198,19.2606176738104));
#56950=CARTESIAN_POINT('Ctrl Pts',(55.1519852737505,31.4471270196898,19.2648442505552));
#56951=CARTESIAN_POINT('Ctrl Pts',(55.0707328223517,31.4508286445337,19.2690708273));
#56952=CARTESIAN_POINT('Ctrl Pts',(54.9894075283417,31.450477106513,19.2732974040448));
#56953=CARTESIAN_POINT('Ctrl Pts',(54.908172495991,31.4501259586587,19.2775192897789));
#56954=CARTESIAN_POINT('Ctrl Pts',(54.8268652438744,31.4457305885304,19.2817411755129));
#56955=CARTESIAN_POINT('Ctrl Pts',(54.7459189752196,31.4372921619795,19.2859630612469));
#56956=CARTESIAN_POINT('Ctrl Pts',(54.6650273023129,31.4288594268856,19.2901820994499));
#56957=CARTESIAN_POINT('Ctrl Pts',(54.5844965901632,31.4163890993054,19.294401137653));
#56958=CARTESIAN_POINT('Ctrl Pts',(54.5047573006657,31.3999343571765,19.298620175856));
#56959=CARTESIAN_POINT('Ctrl Pts',(54.4250440511127,31.3834849885663,19.302837836275));
#56960=CARTESIAN_POINT('Ctrl Pts',(54.3461221655603,31.3630538832531,19.3070554966939));
#56961=CARTESIAN_POINT('Ctrl Pts',(54.2684128964103,31.3387455098538,19.3112731571129));
#56962=CARTESIAN_POINT('Ctrl Pts',(54.1907052443613,31.3144376423027,19.3154907297639));
#56963=CARTESIAN_POINT('Ctrl Pts',(54.1142106015545,31.2862528068968,19.319708302415));
#56964=CARTESIAN_POINT('Ctrl Pts',(54.0393346346563,31.2543452055595,19.323925875066));
#56965=CARTESIAN_POINT('Ctrl Pts',(53.9643315616201,31.2223834392858,19.3281506072823));
#56966=CARTESIAN_POINT('Ctrl Pts',(53.890953091797,31.1866864461052,19.3323753394986));
#56967=CARTESIAN_POINT('Ctrl Pts',(53.8195847957387,31.1474566807153,19.3366000717149));
#56968=CARTESIAN_POINT('Ctrl Pts',(53.7482343246607,31.1082367133707,19.34082374876));
#56969=CARTESIAN_POINT('Ctrl Pts',(53.678893408997,31.0654860010185,19.3450474258051));
#56970=CARTESIAN_POINT('Ctrl Pts',(53.6119190980081,31.019450831173,19.3492711028502));
#56971=CARTESIAN_POINT('Ctrl Pts',(53.5448232721356,30.9733321373879,19.3535024431265));
#56972=CARTESIAN_POINT('Ctrl Pts',(53.4801030023543,30.9239173596677,19.3577337834027));
#56973=CARTESIAN_POINT('Ctrl Pts',(53.4180833540453,30.871494048949,19.3619651236789));
#56974=CARTESIAN_POINT('Ctrl Pts',(53.3562419513309,30.8192214037765,19.3661843030065));
#56975=CARTESIAN_POINT('Ctrl Pts',(53.2970859434363,30.7639578672298,19.370403482334));
#56976=CARTESIAN_POINT('Ctrl Pts',(53.2408992108594,30.7060230548398,19.3746226616615));
#56977=CARTESIAN_POINT('Ctrl Pts',(53.1852939713217,30.6486878268816,19.3787981754598));
#56978=CARTESIAN_POINT('Ctrl Pts',(53.1323780650783,30.5885105338161,19.3829736892582));
#56979=CARTESIAN_POINT('Ctrl Pts',(53.0824613640708,30.5257771232126,19.3871492030566));
#56980=CARTESIAN_POINT('Ctrl Pts',(53.0326089849624,30.4631245499245,19.3913193363516));
#56981=CARTESIAN_POINT('Ctrl Pts',(52.9857484413835,30.3979227611001,19.3954894696466));
#56982=CARTESIAN_POINT('Ctrl Pts',(52.9421529231358,30.3304945164267,19.3996596029416));
#56983=CARTESIAN_POINT('Ctrl Pts',(52.8985993948141,30.263131216663,19.4038257196864));
#56984=CARTESIAN_POINT('Ctrl Pts',(52.8583049111373,30.1935461143265,19.4079918364312));
#56985=CARTESIAN_POINT('Ctrl Pts',(52.821501474637,30.1220937683594,19.412157953176));
#56986=CARTESIAN_POINT('Ctrl Pts',(52.7847215164527,30.0506870045695,19.416321412196));
#56987=CARTESIAN_POINT('Ctrl Pts',(52.7514284031959,29.9774157853516,19.420484871216));
#56988=CARTESIAN_POINT('Ctrl Pts',(52.7218091490529,29.902660897935,19.424648330236));
#56989=CARTESIAN_POINT('Ctrl Pts',(52.6921886781063,29.827902939475,19.4288119602972));
#56990=CARTESIAN_POINT('Ctrl Pts',(52.6662425610509,29.7516616285719,19.4329755903583));
#56991=CARTESIAN_POINT('Ctrl Pts',(52.6441099351468,29.674338381175,19.4371392204195));
#56992=CARTESIAN_POINT('Ctrl Pts',(52.6219780086933,29.5970175774014,19.4413027188987));
#56993=CARTESIAN_POINT('Ctrl Pts',(52.6036594574649,29.5186153673356,19.445466217378));
#56994=CARTESIAN_POINT('Ctrl Pts',(52.5892431215636,29.4395469520672,19.4496297158572));
#56995=CARTESIAN_POINT('Ctrl Pts',(52.574813058599,29.3604032487958,19.4537971787701));
#56996=CARTESIAN_POINT('Ctrl Pts',(52.5642927093787,29.2805925461025,19.457964641683));
#56997=CARTESIAN_POINT('Ctrl Pts',(52.5577193561152,29.2005380425392,19.4621321045959));
#56998=CARTESIAN_POINT('Ctrl Pts',(52.5521775537746,29.1330464263994,19.4656455709803));
#56999=CARTESIAN_POINT('Ctrl Pts',(52.549440251177,29.065381790129,19.4691590373647));
#57000=CARTESIAN_POINT('Ctrl Pts',(52.5495009896071,28.9977977140258,19.4726725037492));
#57001=CARTESIAN_POINT('',(52.549500306966,29.0012265563159,20.2726725038154));
#57002=CARTESIAN_POINT('Ctrl Pts',(52.5495009896078,28.9977977132792,19.472672503788));
#57003=CARTESIAN_POINT('Ctrl Pts',(52.5495996360256,28.8880331912387,19.4783787881767));
#57004=CARTESIAN_POINT('Ctrl Pts',(52.5570768997099,28.7785906334685,19.4840850725655));
#57005=CARTESIAN_POINT('Ctrl Pts',(52.571782136799,28.6702906449134,19.4897913569543));
#57006=CARTESIAN_POINT('Ctrl Pts',(52.5816900546492,28.5973215806758,19.4936360686452));
#57007=CARTESIAN_POINT('Ctrl Pts',(52.5948782273449,28.5248705095064,19.4974807803361));
#57008=CARTESIAN_POINT('Ctrl Pts',(52.6112889351492,28.4531822070749,19.501325492027));
#57009=CARTESIAN_POINT('Ctrl Pts',(52.6293553598906,28.3742610943379,19.5055581061985));
#57010=CARTESIAN_POINT('Ctrl Pts',(52.6513708184919,28.2960895275474,19.5097907203699));
#57011=CARTESIAN_POINT('Ctrl Pts',(52.6772574486544,28.2190920091532,19.5140233345414));
#57012=CARTESIAN_POINT('Ctrl Pts',(52.7031071539696,28.1422043204892,19.5182499112862));
#57013=CARTESIAN_POINT('Ctrl Pts',(52.7328169169065,28.0664877907818,19.5224764880309));
#57014=CARTESIAN_POINT('Ctrl Pts',(52.7662581568425,27.9923554058462,19.5267030647757));
#57015=CARTESIAN_POINT('Ctrl Pts',(52.7996622808747,27.9183052992732,19.5309249505097));
#57016=CARTESIAN_POINT('Ctrl Pts',(52.8367894626801,27.8458362652206,19.5351468362438));
#57017=CARTESIAN_POINT('Ctrl Pts',(52.8774622130622,27.7753434795744,19.5393687219778));
#57018=CARTESIAN_POINT('Ctrl Pts',(52.9181075309351,27.7048982391265,19.5435877601808));
#57019=CARTESIAN_POINT('Ctrl Pts',(52.9622934363404,27.6364270011302,19.5478067983838));
#57020=CARTESIAN_POINT('Ctrl Pts',(53.0097960531247,27.570301255564,19.5520258365868));
#57021=CARTESIAN_POINT('Ctrl Pts',(53.0572831572861,27.5041971042555,19.5562434970057));
#57022=CARTESIAN_POINT('Ctrl Pts',(53.1080845509981,27.4404373012421,19.5604611574247));
#57023=CARTESIAN_POINT('Ctrl Pts',(53.161933264215,27.3793640369285,19.5646788178436));
#57024=CARTESIAN_POINT('Ctrl Pts',(53.2157808568606,27.3182920435263,19.5688963904946));
#57025=CARTESIAN_POINT('Ctrl Pts',(53.2726753348195,27.2599068253392,19.5731139631456));
#57026=CARTESIAN_POINT('Ctrl Pts',(53.3323106532854,27.2045160839332,19.5773315357967));
#57027=CARTESIAN_POINT('Ctrl Pts',(53.3920472060373,27.1490313136479,19.581556268013));
#57028=CARTESIAN_POINT('Ctrl Pts',(53.4545335661553,27.0965515084368,19.5857810002293));
#57029=CARTESIAN_POINT('Ctrl Pts',(53.5194278031398,27.0473463645888,19.5900057324456));
#57030=CARTESIAN_POINT('Ctrl Pts',(53.5843058321073,26.9981535102421,19.5942294094907));
#57031=CARTESIAN_POINT('Ctrl Pts',(53.6515901382957,26.952233926921,19.5984530865358));
#57032=CARTESIAN_POINT('Ctrl Pts',(53.7209103735222,26.9098134108562,19.6026767635808));
#57033=CARTESIAN_POINT('Ctrl Pts',(53.7903563799615,26.8673159291011,19.6069081038571));
#57034=CARTESIAN_POINT('Ctrl Pts',(53.8618452885203,26.8283304249911,19.6111394441333));
#57035=CARTESIAN_POINT('Ctrl Pts',(53.9349820901553,26.7930366786668,19.6153707844095));
#57036=CARTESIAN_POINT('Ctrl Pts',(54.0079086952979,26.7578443672087,19.6195899637371));
#57037=CARTESIAN_POINT('Ctrl Pts',(54.0824732823083,26.7263227221686,19.6238091430648));
#57038=CARTESIAN_POINT('Ctrl Pts',(54.1582683298632,26.6986008504632,19.6280283223924));
#57039=CARTESIAN_POINT('Ctrl Pts',(54.2343047263982,26.6707907058999,19.6322609365639));
#57040=CARTESIAN_POINT('Ctrl Pts',(54.3118622421014,26.6467011639797,19.6364935507353));
#57041=CARTESIAN_POINT('Ctrl Pts',(54.3905424053107,26.6264980113184,19.6407261649068));
#57042=CARTESIAN_POINT('Ctrl Pts',(54.4691103386549,26.6063236765574,19.6449527416516));
#57043=CARTESIAN_POINT('Ctrl Pts',(54.5487972928023,26.5900248353889,19.6491793183964));
#57044=CARTESIAN_POINT('Ctrl Pts',(54.6291868454381,26.5777184609538,19.6534058951411));
#57045=CARTESIAN_POINT('Ctrl Pts',(54.7094871749796,26.5654257451693,19.6576277808752));
#57046=CARTESIAN_POINT('Ctrl Pts',(54.7904880966581,26.5571167613228,19.6618496666092));
#57047=CARTESIAN_POINT('Ctrl Pts',(54.8717615017094,26.5528577610698,19.6660715523432));
#57048=CARTESIAN_POINT('Ctrl Pts',(54.9529800903693,26.5486016333804,19.6702905905463));
#57049=CARTESIAN_POINT('Ctrl Pts',(55.034470334681,26.5483900883593,19.6745096287493));
#57050=CARTESIAN_POINT('Ctrl Pts',(55.1157987411205,26.5522375724848,19.6787286669523));
#57051=CARTESIAN_POINT('Ctrl Pts',(55.1971005886676,26.5560838001624,19.6829463273713));
#57052=CARTESIAN_POINT('Ctrl Pts',(55.2782402396263,26.5639864026279,19.6871639877902));
#57053=CARTESIAN_POINT('Ctrl Pts',(55.3587853173447,26.5759077274044,19.6913816482092));
#57054=CARTESIAN_POINT('Ctrl Pts',(55.4393287189506,26.5878288041026,19.6955992208602));
#57055=CARTESIAN_POINT('Ctrl Pts',(55.5192771125469,26.60376836766,19.6998167935113));
#57056=CARTESIAN_POINT('Ctrl Pts',(55.5982057792581,26.6236372129529,19.7040343661623));
#57057=CARTESIAN_POINT('Ctrl Pts',(55.6772684317915,26.643539786721,19.7082590983786));
#57058=CARTESIAN_POINT('Ctrl Pts',(55.7553074411604,26.6673848736874,19.7124838305949));
#57059=CARTESIAN_POINT('Ctrl Pts',(55.8319104320743,26.6950324768002,19.7167085628112));
#57060=CARTESIAN_POINT('Ctrl Pts',(55.9084942905876,26.7226731746341,19.7209322398563));
#57061=CARTESIAN_POINT('Ctrl Pts',(55.9836424260476,26.7541142898905,19.7251559169014));
#57062=CARTESIAN_POINT('Ctrl Pts',(56.0569638170305,26.7891680888208,19.7293795939465));
#57063=CARTESIAN_POINT('Ctrl Pts',(56.1304182387257,26.8242854876335,19.7336109342228));
#57064=CARTESIAN_POINT('Ctrl Pts',(56.202038882535,26.8630284477427,19.737842274499));
#57065=CARTESIAN_POINT('Ctrl Pts',(56.2714599010994,26.9051634980514,19.7420736147753));
#57066=CARTESIAN_POINT('Ctrl Pts',(56.3406814023974,26.9471774514613,19.7462927941028));
#57067=CARTESIAN_POINT('Ctrl Pts',(56.407715574752,26.9925636991414,19.7505119734303));
#57068=CARTESIAN_POINT('Ctrl Pts',(56.4722322650878,27.0410506878343,19.7547311527579));
#57069=CARTESIAN_POINT('Ctrl Pts',(56.5369543915045,27.0896920703265,19.7589637669293));
#57070=CARTESIAN_POINT('Ctrl Pts',(56.5993836810645,27.1416349050295,19.7631963811008));
#57071=CARTESIAN_POINT('Ctrl Pts',(56.6591641394782,27.1966351982282,19.7674289952723));
#57072=CARTESIAN_POINT('Ctrl Pts',(56.7188593266812,27.2515570386729,19.7716555720171));
#57073=CARTESIAN_POINT('Ctrl Pts',(56.7759128479175,27.3095273638339,19.7758821487618));
#57074=CARTESIAN_POINT('Ctrl Pts',(56.8299998825219,27.3702605484404,19.7801087255066));
#57075=CARTESIAN_POINT('Ctrl Pts',(56.8840268867811,27.4309263262448,19.7843306112407));
#57076=CARTESIAN_POINT('Ctrl Pts',(56.9350936391157,27.4943485252869,19.7885524969747));
#57077=CARTESIAN_POINT('Ctrl Pts',(56.9829115032094,27.5602041045898,19.7927743827087));
#57078=CARTESIAN_POINT('Ctrl Pts',(57.0306971156364,27.6260152663466,19.7969934209117));
#57079=CARTESIAN_POINT('Ctrl Pts',(57.0752379196429,27.6942561737829,19.8012124591147));
#57080=CARTESIAN_POINT('Ctrl Pts',(57.1162858029343,27.7645710662693,19.8054314973177));
#57081=CARTESIAN_POINT('Ctrl Pts',(57.1573202814835,27.8348629964755,19.8096491577367));
#57082=CARTESIAN_POINT('Ctrl Pts',(57.1948638705751,27.9072271657966,19.8138668181557));
#57083=CARTESIAN_POINT('Ctrl Pts',(57.2287127678591,27.9812803877505,19.8180844785746));
#57084=CARTESIAN_POINT('Ctrl Pts',(57.2625609607603,28.0553320686848,19.8223020512256));
#57085=CARTESIAN_POINT('Ctrl Pts',(57.2927144226679,28.1310723093763,19.8265196238767));
#57086=CARTESIAN_POINT('Ctrl Pts',(57.3190167637917,28.2080962815763,19.8307371965277));
#57087=CARTESIAN_POINT('Ctrl Pts',(57.3453637546093,28.2852510062735,19.834961928744));
#57088=CARTESIAN_POINT('Ctrl Pts',(57.3678463937328,28.3636933806243,19.8391866609603));
#57089=CARTESIAN_POINT('Ctrl Pts',(57.3863576167803,28.4430012793239,19.8434113931766));
#57090=CARTESIAN_POINT('Ctrl Pts',(57.4048642164555,28.5222893700436,19.8476350702217));
#57091=CARTESIAN_POINT('Ctrl Pts',(57.4194013213343,28.6024420903557,19.8518587472668));
#57092=CARTESIAN_POINT('Ctrl Pts',(57.4299135348426,28.6830292392211,19.8560824243119));
#57093=CARTESIAN_POINT('Ctrl Pts',(57.4404448211921,28.7637626014313,19.8603137645881));
#57094=CARTESIAN_POINT('Ctrl Pts',(57.446936585103,28.8449315029823,19.8645451048643));
#57095=CARTESIAN_POINT('Ctrl Pts',(57.4493855004242,28.9261019600266,19.8687764451406));
#57096=CARTESIAN_POINT('Ctrl Pts',(57.4518273775182,29.0070391317058,19.8729956244681));
#57097=CARTESIAN_POINT('Ctrl Pts',(57.4502497054639,29.0879773964062,19.8772148037957));
#57098=CARTESIAN_POINT('Ctrl Pts',(57.4447005343835,29.168491979587,19.8814339831233));
#57099=CARTESIAN_POINT('Ctrl Pts',(57.4391336934574,29.2492629398444,19.8856665972948));
#57100=CARTESIAN_POINT('Ctrl Pts',(57.4295492888961,29.3299079239494,19.8898992114663));
#57101=CARTESIAN_POINT('Ctrl Pts',(57.4159581852052,29.4099954845359,19.8941318256378));
#57102=CARTESIAN_POINT('Ctrl Pts',(57.4023864679476,29.4899688077372,19.8983584023826));
#57103=CARTESIAN_POINT('Ctrl Pts',(57.3848194797224,29.5693858324206,19.9025849791275));
#57104=CARTESIAN_POINT('Ctrl Pts',(57.3633199775803,29.64781859619,19.9068115558723));
#57105=CARTESIAN_POINT('Ctrl Pts',(57.3418443373963,29.7261643086731,19.9110334416063));
#57106=CARTESIAN_POINT('Ctrl Pts',(57.3164449780063,29.8035274851064,19.9152553273403));
#57107=CARTESIAN_POINT('Ctrl Pts',(57.2872357404877,29.8794901462982,19.9194772130743));
#57108=CARTESIAN_POINT('Ctrl Pts',(57.2580462036938,29.9554015730315,19.9236962512774));
#57109=CARTESIAN_POINT('Ctrl Pts',(57.2250520586072,30.0299139281105,19.9279152894805));
#57110=CARTESIAN_POINT('Ctrl Pts',(57.1884166536857,30.1026254123097,19.9321343276835));
#57111=CARTESIAN_POINT('Ctrl Pts',(57.1517932125517,30.1753131515891,19.9363519881025));
#57112=CARTESIAN_POINT('Ctrl Pts',(57.1115310819357,30.2462007733704,19.9405696485215));
#57113=CARTESIAN_POINT('Ctrl Pts',(57.0678407381616,30.3149087160708,19.9447873089405));
#57114=CARTESIAN_POINT('Ctrl Pts',(57.0241513035672,30.383615228985,19.9490048815916));
#57115=CARTESIAN_POINT('Ctrl Pts',(56.9770340479185,30.4501417616265,19.9532224542427));
#57116=CARTESIAN_POINT('Ctrl Pts',(56.9267434126354,30.5141367414689,19.9574400268938));
#57117=CARTESIAN_POINT('Ctrl Pts',(56.8763674061899,30.5782403563641,19.96166475911));
#57118=CARTESIAN_POINT('Ctrl Pts',(56.8228075305529,30.6398034530804,19.9658894913263));
#57119=CARTESIAN_POINT('Ctrl Pts',(56.7663595891434,30.698506417957,19.9701142235425));
#57120=CARTESIAN_POINT('Ctrl Pts',(56.7099257461982,30.7571947211536,19.9743379005877));
#57121=CARTESIAN_POINT('Ctrl Pts',(56.6506056339709,30.813024017022,19.9785615776328));
#57122=CARTESIAN_POINT('Ctrl Pts',(56.5887299580062,30.8657136357259,19.982785254678));
#57123=CARTESIAN_POINT('Ctrl Pts',(56.5267420178696,30.9184988518729,19.9870165949542));
#57124=CARTESIAN_POINT('Ctrl Pts',(56.4621896170737,30.96813272266,19.9912479352305));
#57125=CARTESIAN_POINT('Ctrl Pts',(56.3954349814589,31.0143761968711,19.9954792755068));
#57126=CARTESIAN_POINT('Ctrl Pts',(56.328872199882,31.0604867664955,19.9996984548341));
#57127=CARTESIAN_POINT('Ctrl Pts',(56.2601202556544,31.1032262319335,20.0039176341614));
#57128=CARTESIAN_POINT('Ctrl Pts',(56.189561618902,31.1424036512374,20.0081368134887));
#57129=CARTESIAN_POINT('Ctrl Pts',(56.1187783071086,31.1817058205179,20.0123694276602));
#57130=CARTESIAN_POINT('Ctrl Pts',(56.0459135024077,31.2175693745498,20.0166020418316));
#57131=CARTESIAN_POINT('Ctrl Pts',(55.9713350283798,31.2497685464604,20.0208346560031));
#57132=CARTESIAN_POINT('Ctrl Pts',(55.8968629335426,31.2819217892755,20.0250612327478));
#57133=CARTESIAN_POINT('Ctrl Pts',(55.8206824472001,31.3104208486512,20.0292878094926));
#57134=CARTESIAN_POINT('Ctrl Pts',(55.7431867199957,31.3350853837113,20.0335143862373));
#57135=CARTESIAN_POINT('Ctrl Pts',(55.6657770040739,31.3597225439937,20.0377362719714));
#57136=CARTESIAN_POINT('Ctrl Pts',(55.5870553882782,31.3805334962032,20.0419581577054));
#57137=CARTESIAN_POINT('Ctrl Pts',(55.5074344592735,31.3973861848984,20.0461800434394));
#57138=CARTESIAN_POINT('Ctrl Pts',(55.4278672321169,31.4142275069776,20.0503990816424));
#57139=CARTESIAN_POINT('Ctrl Pts',(55.3474023497371,31.427115771904,20.0546181198454));
#57140=CARTESIAN_POINT('Ctrl Pts',(55.2664657784925,31.4359692606625,20.0588371580484));
#57141=CARTESIAN_POINT('Ctrl Pts',(55.1855556381812,31.4448198581943,20.0630548184674));
#57142=CARTESIAN_POINT('Ctrl Pts',(55.1041745763518,31.4496382457765,20.0672724788863));
#57143=CARTESIAN_POINT('Ctrl Pts',(55.0227555623159,31.4503943426281,20.0714901393053));
#57144=CARTESIAN_POINT('Ctrl Pts',(54.9413382425788,31.4511504237456,20.0757077119563));
#57145=CARTESIAN_POINT('Ctrl Pts',(54.859883436744,31.4478443790698,20.0799252846073));
#57146=CARTESIAN_POINT('Ctrl Pts',(54.7788245708301,31.4404982441156,20.0841428572583));
#57147=CARTESIAN_POINT('Ctrl Pts',(54.6976281029607,31.4331396386869,20.0883675894746));
#57148=CARTESIAN_POINT('Ctrl Pts',(54.6168293848757,31.4217272633144,20.092592321691));
#57149=CARTESIAN_POINT('Ctrl Pts',(54.5368575521966,31.4063352474339,20.0968170539073));
#57150=CARTESIAN_POINT('Ctrl Pts',(54.4569056933225,31.390947075871,20.1010407309524));
#57151=CARTESIAN_POINT('Ctrl Pts',(54.3777807545964,31.3715813829267,20.1052644079975));
#57152=CARTESIAN_POINT('Ctrl Pts',(54.2998982053227,31.3483627758695,20.1094880850425));
#57153=CARTESIAN_POINT('Ctrl Pts',(54.2218743497963,31.3251020421179,20.1137194253188));
#57154=CARTESIAN_POINT('Ctrl Pts',(54.1450978278075,31.297974579116,20.117950765595));
#57155=CARTESIAN_POINT('Ctrl Pts',(54.0699663575865,31.2671540913619,20.1221821058712));
#57156=CARTESIAN_POINT('Ctrl Pts',(53.9950508165709,31.2364221822475,20.1264012851989));
#57157=CARTESIAN_POINT('Ctrl Pts',(53.9217712608793,31.202018716437,20.1306204645265));
#57158=CARTESIAN_POINT('Ctrl Pts',(53.8504960744794,31.1641605705706,20.1348396438542));
#57159=CARTESIAN_POINT('Ctrl Pts',(53.7789939313854,31.1261818756035,20.1390722580256));
#57160=CARTESIAN_POINT('Ctrl Pts',(53.7092430190922,31.0845851869611,20.143304872197));
#57161=CARTESIAN_POINT('Ctrl Pts',(53.6416329600019,31.0395561366746,20.1475374863684));
#57162=CARTESIAN_POINT('Ctrl Pts',(53.5741193403127,30.9945913161002,20.1517640631132));
#57163=CARTESIAN_POINT('Ctrl Pts',(53.5087408921651,30.9462041132224,20.1559906398579));
#57164=CARTESIAN_POINT('Ctrl Pts',(53.4458629215627,30.8946261350004,20.1602172166026));
#57165=CARTESIAN_POINT('Ctrl Pts',(53.3830547382254,30.8431054023605,20.1644391023366));
#57166=CARTESIAN_POINT('Ctrl Pts',(53.3227418753958,30.7884012242506,20.1686609880707));
#57167=CARTESIAN_POINT('Ctrl Pts',(53.2652597170226,30.730787797685,20.1728828738047));
#57168=CARTESIAN_POINT('Ctrl Pts',(53.2078163285839,30.6732132295903,20.1771019120077));
#57169=CARTESIAN_POINT('Ctrl Pts',(53.1532001799829,30.6127336381475,20.1813209502106));
#57170=CARTESIAN_POINT('Ctrl Pts',(53.1017117156202,30.5496618467867,20.1855399884136));
#57171=CARTESIAN_POINT('Ctrl Pts',(53.0502400655128,30.4866106523734,20.1897576488325));
#57172=CARTESIAN_POINT('Ctrl Pts',(53.001894364779,30.4209692987631,20.1939753092514));
#57173=CARTESIAN_POINT('Ctrl Pts',(52.9569355547793,30.3530845955354,20.1981929696703));
#57174=CARTESIAN_POINT('Ctrl Pts',(52.9119776803554,30.2852013049627,20.2024105423212));
#57175=CARTESIAN_POINT('Ctrl Pts',(52.870406812062,30.2150751455486,20.2066281149722));
#57176=CARTESIAN_POINT('Ctrl Pts',(52.832440423427,30.1430816821237,20.2108456876232));
#57177=CARTESIAN_POINT('Ctrl Pts',(52.7944095847245,30.0709660057692,20.2150704198396));
#57178=CARTESIAN_POINT('Ctrl Pts',(52.7599956858202,29.9969770963422,20.219295152056));
#57179=CARTESIAN_POINT('Ctrl Pts',(52.7293701668518,29.9215152797525,20.2235198842723));
#57180=CARTESIAN_POINT('Ctrl Pts',(52.6987522969291,29.8460723105456,20.2277435613174));
#57181=CARTESIAN_POINT('Ctrl Pts',(52.6719210482788,29.7691576169731,20.2319672383624));
#57182=CARTESIAN_POINT('Ctrl Pts',(52.648998079005,29.6911875414659,20.2361909154074));
#57183=CARTESIAN_POINT('Ctrl Pts',(52.6260335194273,29.6130760009028,20.2404222556836));
#57184=CARTESIAN_POINT('Ctrl Pts',(52.6069915192758,29.5339057046566,20.2446535959598));
#57185=CARTESIAN_POINT('Ctrl Pts',(52.5919428889606,29.4541048336809,20.248884936236));
#57186=CARTESIAN_POINT('Ctrl Pts',(52.5769375086802,29.3745333118474,20.2531041155639));
#57187=CARTESIAN_POINT('Ctrl Pts',(52.5659025545103,29.2943352973498,20.2573232948918));
#57188=CARTESIAN_POINT('Ctrl Pts',(52.5588566533828,29.2139378677712,20.2615424742197));
#57189=CARTESIAN_POINT('Ctrl Pts',(52.5526610497839,29.143242779234,20.2652524840758));
#57190=CARTESIAN_POINT('Ctrl Pts',(52.5495358689406,29.0722747171758,20.2689624939319));
#57191=CARTESIAN_POINT('Ctrl Pts',(52.5495003069663,29.0012265568403,20.272672503788));
#57192=CARTESIAN_POINT('',(52.5495003092563,29.0012311234037,21.072672503762));
#57193=CARTESIAN_POINT('Ctrl Pts',(52.549500306966,29.0012265563159,20.2726725038154));
#57194=CARTESIAN_POINT('Ctrl Pts',(52.5494602204554,28.9211389315022,20.276854538593));
#57195=CARTESIAN_POINT('Ctrl Pts',(52.5533505212183,28.8408938744122,20.2810365733706));
#57196=CARTESIAN_POINT('Ctrl Pts',(52.5611912006416,28.7609144710107,20.2852186081482));
#57197=CARTESIAN_POINT('Ctrl Pts',(52.5692395086798,28.6788171372802,20.2895113871664));
#57198=CARTESIAN_POINT('Ctrl Pts',(52.5814504704765,28.5970002272627,20.2938041661846));
#57199=CARTESIAN_POINT('Ctrl Pts',(52.597788511568,28.5159233378427,20.2980969452028));
#57200=CARTESIAN_POINT('Ctrl Pts',(52.6136681749886,28.437121129673,20.3022692866461));
#57201=CARTESIAN_POINT('Ctrl Pts',(52.633446299331,28.3590184693443,20.3064416280894));
#57202=CARTESIAN_POINT('Ctrl Pts',(52.6570377636194,28.2820318886647,20.3106139695326));
#57203=CARTESIAN_POINT('Ctrl Pts',(52.6806175758626,28.2050833323785,20.3147842502174));
#57204=CARTESIAN_POINT('Ctrl Pts',(52.7080068516926,28.129250216667,20.3189545309021));
#57205=CARTESIAN_POINT('Ctrl Pts',(52.7390700458616,28.0549359849833,20.3231248115869));
#57206=CARTESIAN_POINT('Ctrl Pts',(52.7701279301895,27.9806344563317,20.3272943794175));
#57207=CARTESIAN_POINT('Ctrl Pts',(52.8048583016476,27.9078517353656,20.3314639472481));
#57208=CARTESIAN_POINT('Ctrl Pts',(52.8430772801611,27.8369717842447,20.3356335150786));
#57209=CARTESIAN_POINT('Ctrl Pts',(52.8832646755621,27.7624412569391,20.3400178308708));
#57210=CARTESIAN_POINT('Ctrl Pts',(52.9273094397009,27.6900152887277,20.3444021466631));
#57211=CARTESIAN_POINT('Ctrl Pts',(52.9749438292944,27.6201095132267,20.3487864624553));
#57212=CARTESIAN_POINT('Ctrl Pts',(53.020301483121,27.5535449578141,20.3529612252614));
#57213=CARTESIAN_POINT('Ctrl Pts',(53.0689131459155,27.489265569475,20.3571359880676));
#57214=CARTESIAN_POINT('Ctrl Pts',(53.1205052786273,27.4275974299397,20.3613107508737));
#57215=CARTESIAN_POINT('Ctrl Pts',(53.1721317381003,27.3658882595846,20.3654882913531));
#57216=CARTESIAN_POINT('Ctrl Pts',(53.2267422873025,27.3067941411329,20.3696658318325));
#57217=CARTESIAN_POINT('Ctrl Pts',(53.2840263694769,27.2506044617213,20.3738433723119));
#57218=CARTESIAN_POINT('Ctrl Pts',(53.341399074354,27.1943278527288,20.3780273757547));
#57219=CARTESIAN_POINT('Ctrl Pts',(53.4014532028681,27.1409649548513,20.3822113791975));
#57220=CARTESIAN_POINT('Ctrl Pts',(53.4638457085829,27.0907644872984,20.3863953826403));
#57221=CARTESIAN_POINT('Ctrl Pts',(53.4730411491932,27.083365915744,20.3870120232886));
#57222=CARTESIAN_POINT('Ctrl Pts',(53.4822873330595,27.0760359569583,20.3876286639368));
#57223=CARTESIAN_POINT('Ctrl Pts',(53.4915831133027,27.0687753248453,20.3882453045851));
#57224=CARTESIAN_POINT('Ctrl Pts',(53.5553892397709,27.0189384312525,20.3924779187563));
#57225=CARTESIAN_POINT('Ctrl Pts',(53.6217865330381,26.9721744096337,20.3967105329275));
#57226=CARTESIAN_POINT('Ctrl Pts',(53.6904467768475,26.9287635080148,20.4009431470987));
#57227=CARTESIAN_POINT('Ctrl Pts',(53.7590090832661,26.885414527971,20.4051697238432));
#57228=CARTESIAN_POINT('Ctrl Pts',(53.8298275398407,26.8454094146431,20.4093963005877));
#57229=CARTESIAN_POINT('Ctrl Pts',(53.9025418437445,26.8089874840001,20.4136228773322));
#57230=CARTESIAN_POINT('Ctrl Pts',(53.9751754431973,26.7726059774795,20.4178447630663));
#57231=CARTESIAN_POINT('Ctrl Pts',(54.049700295733,26.7397999585165,20.4220666488004));
#57232=CARTESIAN_POINT('Ctrl Pts',(54.1257293863423,26.7107640698052,20.4262885345345));
#57233=CARTESIAN_POINT('Ctrl Pts',(54.2017071976815,26.6817477649029,20.4305075727372));
#57234=CARTESIAN_POINT('Ctrl Pts',(54.2791867992283,26.6564967052678,20.43472661094));
#57235=CARTESIAN_POINT('Ctrl Pts',(54.3577601272413,26.6351578919854,20.4389456491427));
#57236=CARTESIAN_POINT('Ctrl Pts',(54.4363077960701,26.6138260471814,20.4431633095614));
#57237=CARTESIAN_POINT('Ctrl Pts',(54.5159480340786,26.5964040331587,20.4473809699801));
#57238=CARTESIAN_POINT('Ctrl Pts',(54.5962578253218,26.5829889312653,20.4515986303988));
#57239=CARTESIAN_POINT('Ctrl Pts',(54.6765659453488,26.5695741085351,20.4558162030496));
#57240=CARTESIAN_POINT('Ctrl Pts',(54.757543132515,26.5601661075289,20.4600337757003));
#57241=CARTESIAN_POINT('Ctrl Pts',(54.8387578108094,26.5548105990691,20.4642513483511));
#57242=CARTESIAN_POINT('Ctrl Pts',(54.9201103555698,26.5494459993336,20.4684760805677));
#57243=CARTESIAN_POINT('Ctrl Pts',(55.0017007320943,26.5481476868118,20.4727008127844));
#57244=CARTESIAN_POINT('Ctrl Pts',(55.0830934970774,26.5509092052879,20.476925545001));
#57245=CARTESIAN_POINT('Ctrl Pts',(55.1644659333525,26.5536700340454,20.4811492220458));
#57246=CARTESIAN_POINT('Ctrl Pts',(55.2456403940463,26.560488605887,20.4853728990907));
#57247=CARTESIAN_POINT('Ctrl Pts',(55.3261870817444,26.5713064751387,20.4895965761355));
#57248=CARTESIAN_POINT('Ctrl Pts',(55.4068799093768,26.5821439717984,20.4938279164115));
#57249=CARTESIAN_POINT('Ctrl Pts',(55.4869422296769,26.5969951820191,20.4980592566875));
#57250=CARTESIAN_POINT('Ctrl Pts',(55.5659541409433,26.6157503988993,20.5022905969635));
#57251=CARTESIAN_POINT('Ctrl Pts',(55.6447389705763,26.6344517129537,20.5065097762925));
#57252=CARTESIAN_POINT('Ctrl Pts',(55.7224790069256,26.6570344163943,20.5107289556215));
#57253=CARTESIAN_POINT('Ctrl Pts',(55.7987766080229,26.6833415917586,20.5149481349506));
#57254=CARTESIAN_POINT('Ctrl Pts',(55.8753171583144,26.7097325352489,20.5191807491216));
#57255=CARTESIAN_POINT('Ctrl Pts',(55.9506907393684,26.7399698887984,20.5234133632927));
#57256=CARTESIAN_POINT('Ctrl Pts',(56.0244835908758,26.7739309035822,20.5276459774637));
#57257=CARTESIAN_POINT('Ctrl Pts',(56.0981711838093,26.8078434761672,20.5318725542081));
#57258=CARTESIAN_POINT('Ctrl Pts',(56.1702821069487,26.8454689681559,20.5360991309525));
#57259=CARTESIAN_POINT('Ctrl Pts',(56.2404194668725,26.8866354322541,20.5403257076968));
#57260=CARTESIAN_POINT('Ctrl Pts',(56.3104789824573,26.9277562063493,20.544547593431));
#57261=CARTESIAN_POINT('Ctrl Pts',(56.3785688885819,26.9724099095512,20.5487694791651));
#57262=CARTESIAN_POINT('Ctrl Pts',(56.4443152227609,27.0203778675461,20.5529913648992));
#57263=CARTESIAN_POINT('Ctrl Pts',(56.5100172130679,27.0683134726348,20.5572104031018));
#57264=CARTESIAN_POINT('Ctrl Pts',(56.5733783964576,27.119558619795,20.5614294413044));
#57265=CARTESIAN_POINT('Ctrl Pts',(56.6340533144811,27.1738510423755,20.565648479507));
#57266=CARTESIAN_POINT('Ctrl Pts',(56.6947084182886,27.2281257350301,20.5698661399255));
#57267=CARTESIAN_POINT('Ctrl Pts',(56.7526786529445,27.285445417305,20.574083800344));
#57268=CARTESIAN_POINT('Ctrl Pts',(56.8076522939434,27.345508103918,20.5783014607626));
#57269=CARTESIAN_POINT('Ctrl Pts',(56.8626247909617,27.4055695406493,20.5825190334132));
#57270=CARTESIAN_POINT('Ctrl Pts',(56.9146005055265,27.4683735247527,20.5867366060638));
#57271=CARTESIAN_POINT('Ctrl Pts',(56.9633061774716,27.5335829026154,20.5909541787144));
#57272=CARTESIAN_POINT('Ctrl Pts',(57.0120945300272,27.5989029770553,20.5951789109312));
#57273=CARTESIAN_POINT('Ctrl Pts',(57.0576014540899,27.6666362408167,20.599403643148));
#57274=CARTESIAN_POINT('Ctrl Pts',(57.09959530961,27.7364139183008,20.6036283753648));
#57275=CARTESIAN_POINT('Ctrl Pts',(57.1415786767147,27.8061741680626,20.6078520524095));
#57276=CARTESIAN_POINT('Ctrl Pts',(57.1800505284885,27.8779773895188,20.6120757294541));
#57277=CARTESIAN_POINT('Ctrl Pts',(57.214825908578,27.9514312398839,20.6162994064988));
#57278=CARTESIAN_POINT('Ctrl Pts',(57.2496643834006,28.0250183612891,20.6205307467746));
#57279=CARTESIAN_POINT('Ctrl Pts',(57.280792805333,28.1002616661367,20.6247620870504));
#57280=CARTESIAN_POINT('Ctrl Pts',(57.3080746044668,28.1767492057608,20.6289934273262));
#57281=CARTESIAN_POINT('Ctrl Pts',(57.3352779952332,28.2530169188596,20.6332126066561));
#57282=CARTESIAN_POINT('Ctrl Pts',(57.3586567923574,28.3305212645066,20.6374317859861));
#57283=CARTESIAN_POINT('Ctrl Pts',(57.3781261455574,28.4088432645937,20.641650965316));
#57284=CARTESIAN_POINT('Ctrl Pts',(57.3976574936843,28.4874146600572,20.6458835794894));
#57285=CARTESIAN_POINT('Ctrl Pts',(57.41332707702,28.5671011610222,20.6501161936629));
#57286=CARTESIAN_POINT('Ctrl Pts',(57.4250126089298,28.6474888703437,20.6543488078364));
#57287=CARTESIAN_POINT('Ctrl Pts',(57.4366814725256,28.7277619141462,20.6585753845831));
#57288=CARTESIAN_POINT('Ctrl Pts',(57.4443775053466,28.8087337238667,20.6628019613299));
#57289=CARTESIAN_POINT('Ctrl Pts',(57.4480288720224,28.8899777670446,20.6670285380767));
#57290=CARTESIAN_POINT('Ctrl Pts',(57.4516761861019,28.9711316386948,20.6712504238102));
#57291=CARTESIAN_POINT('Ctrl Pts',(57.4512877331433,29.0525566816944,20.6754723095438));
#57292=CARTESIAN_POINT('Ctrl Pts',(57.4468433571991,29.1338201604047,20.6796941952773));
#57293=CARTESIAN_POINT('Ctrl Pts',(57.442401978846,29.2150288294664,20.6839132334823));
#57294=CARTESIAN_POINT('Ctrl Pts',(57.4339101359348,29.2960756880045,20.6881322716873));
#57295=CARTESIAN_POINT('Ctrl Pts',(57.4213997564911,29.3765281785804,20.6923513098923));
#57296=CARTESIAN_POINT('Ctrl Pts',(57.4088934624811,29.4569543963059,20.6965689703133));
#57297=CARTESIAN_POINT('Ctrl Pts',(57.3923713094257,29.5367861728579,20.7007866307342));
#57298=CARTESIAN_POINT('Ctrl Pts',(57.3719169071258,29.6155976248256,20.7050042911551));
#57299=CARTESIAN_POINT('Ctrl Pts',(57.3514629304743,29.6944074367566,20.7092218638082));
#57300=CARTESIAN_POINT('Ctrl Pts',(57.3270769851119,29.7721965169635,20.7134394364612));
#57301=CARTESIAN_POINT('Ctrl Pts',(57.2988931209399,29.848552101226,20.7176570091142));
#57302=CARTESIAN_POINT('Ctrl Pts',(57.2706614131126,29.9250373032813,20.7218817413281));
#57303=CARTESIAN_POINT('Ctrl Pts',(57.2386190488923,30.0000837025487,20.7261064735421));
#57304=CARTESIAN_POINT('Ctrl Pts',(57.2029492615242,30.0732962317784,20.730331205756));
#57305=CARTESIAN_POINT('Ctrl Pts',(57.1672883830236,30.1464904754851,20.734554882803));
#57306=CARTESIAN_POINT('Ctrl Pts',(57.1280021365455,30.2178513669816,20.7387785598501));
#57307=CARTESIAN_POINT('Ctrl Pts',(57.0853189387287,30.2870101684833,20.7430022368971));
#57308=CARTESIAN_POINT('Ctrl Pts',(57.0425582986253,30.3562944482997,20.7472335771752));
#57309=CARTESIAN_POINT('Ctrl Pts',(56.9963886542809,30.4233682697559,20.7514649174534));
#57310=CARTESIAN_POINT('Ctrl Pts',(56.9470812098606,30.4878928093811,20.7556962577315));
#57311=CARTESIAN_POINT('Ctrl Pts',(56.8979154760785,30.5522319041146,20.7599154370481));
#57312=CARTESIAN_POINT('Ctrl Pts',(56.8456303118749,30.6140360569888,20.7641346163648));
#57313=CARTESIAN_POINT('Ctrl Pts',(56.7905309740915,30.6730060014295,20.7683537956815));
#57314=CARTESIAN_POINT('Ctrl Pts',(56.7352561871496,30.732163719944,20.7725864098504));
#57315=CARTESIAN_POINT('Ctrl Pts',(56.6769436737209,30.7886891570702,20.7768190240193));
#57316=CARTESIAN_POINT('Ctrl Pts',(56.6158740482287,30.8422544097548,20.7810516381881));
#57317=CARTESIAN_POINT('Ctrl Pts',(56.5548915328232,30.8957432566359,20.7852782149303));
#57318=CARTESIAN_POINT('Ctrl Pts',(56.4911600626649,30.946280001575,20.7895047916725));
#57319=CARTESIAN_POINT('Ctrl Pts',(56.4249983167076,30.9935721826361,20.7937313684147));
#57320=CARTESIAN_POINT('Ctrl Pts',(56.3589100025761,31.0408118748889,20.7979532541494));
#57321=CARTESIAN_POINT('Ctrl Pts',(56.2903971482431,31.0848138898379,20.8021751398841));
#57322=CARTESIAN_POINT('Ctrl Pts',(56.2198117703657,31.1253257385345,20.8063970256187));
#57323=CARTESIAN_POINT('Ctrl Pts',(56.1492740001902,31.1658102632148,20.8106160638192));
#57324=CARTESIAN_POINT('Ctrl Pts',(56.0766668845959,31.2028090662687,20.8148351020197));
#57325=CARTESIAN_POINT('Ctrl Pts',(56.0023706453165,31.2361134451114,20.8190541402202));
#57326=CARTESIAN_POINT('Ctrl Pts',(55.9280986684798,31.2694069479582,20.8232718006366));
#57327=CARTESIAN_POINT('Ctrl Pts',(55.8521390869959,31.2990082326812,20.827489461053));
#57328=CARTESIAN_POINT('Ctrl Pts',(55.7748946598559,31.3247555820187,20.8317071214695));
#57329=CARTESIAN_POINT('Ctrl Pts',(55.6976518401427,31.3505023955637,20.835924694118));
#57330=CARTESIAN_POINT('Ctrl Pts',(55.6191246690153,31.3723952873945,20.8401422667666));
#57331=CARTESIAN_POINT('Ctrl Pts',(55.5397323603883,31.3903219927762,20.8443598394151));
#57332=CARTESIAN_POINT('Ctrl Pts',(55.4602052787772,31.4082791297655,20.8485845716344));
#57333=CARTESIAN_POINT('Ctrl Pts',(55.3798105768262,31.4222565066309,20.8528093038538));
#57334=CARTESIAN_POINT('Ctrl Pts',(55.2989793992393,31.4321927491115,20.8570340360731));
#57335=CARTESIAN_POINT('Ctrl Pts',(55.2181684101908,31.4421265098985,20.8612577131158));
#57336=CARTESIAN_POINT('Ctrl Pts',(55.1369216299782,31.4480211421537,20.8654813901585));
#57337=CARTESIAN_POINT('Ctrl Pts',(55.0556727153591,31.4498675063694,20.8697050672012));
#57338=CARTESIAN_POINT('Ctrl Pts',(54.9742763867188,31.4517172205371,20.8739364074751));
#57339=CARTESIAN_POINT('Ctrl Pts',(54.8928783816584,31.4495040006416,20.8781677477489));
#57340=CARTESIAN_POINT('Ctrl Pts',(54.8119105576179,31.4432708838081,20.8823990880228));
#57341=CARTESIAN_POINT('Ctrl Pts',(54.7311754362634,31.4370556810417,20.8866182673642));
#57342=CARTESIAN_POINT('Ctrl Pts',(54.6508684676596,31.426843796904,20.8908374467055));
#57343=CARTESIAN_POINT('Ctrl Pts',(54.5714068662368,31.4127283675729,20.8950566260469));
#57344=CARTESIAN_POINT('Ctrl Pts',(54.4916922409749,31.3985679914995,20.8992892402163));
#57345=CARTESIAN_POINT('Ctrl Pts',(54.4125318989979,31.3804264777048,20.9035218543858));
#57346=CARTESIAN_POINT('Ctrl Pts',(54.3343536603774,31.3583607019595,20.9077544685552));
#57347=CARTESIAN_POINT('Ctrl Pts',(54.2562869356745,31.3363264009717,20.9119810452979));
#57348=CARTESIAN_POINT('Ctrl Pts',(54.17919997537,31.3103790807106,20.9162076220406));
#57349=CARTESIAN_POINT('Ctrl Pts',(54.1035115929932,31.2806268406082,20.9204341987833));
#57350=CARTESIAN_POINT('Ctrl Pts',(54.0279072159099,31.2509076220288,20.9246560845179));
#57351=CARTESIAN_POINT('Ctrl Pts',(53.9536987625856,31.2173920438296,20.9288779702524));
#57352=CARTESIAN_POINT('Ctrl Pts',(53.8812896652721,31.1802379312756,20.933099855987));
#57353=CARTESIAN_POINT('Ctrl Pts',(53.808929405695,31.1431088780419,20.9373188941878));
#57354=CARTESIAN_POINT('Ctrl Pts',(53.7383665040388,31.1023463760024,20.9415379323887));
#57355=CARTESIAN_POINT('Ctrl Pts',(53.6699830183152,31.0581557468836,20.9457569705896));
#57356=CARTESIAN_POINT('Ctrl Pts',(53.6016218641454,31.0139795488135,20.9499746310064));
#57357=CARTESIAN_POINT('Ctrl Pts',(53.5354391023518,30.9663776988673,20.9541922914232));
#57358=CARTESIAN_POINT('Ctrl Pts',(53.471789647773,30.9156000024395,20.95840995184));
#57359=CARTESIAN_POINT('Ctrl Pts',(53.4081415177153,30.8648233626764,20.9626275244889));
#57360=CARTESIAN_POINT('Ctrl Pts',(53.3470269524701,30.810871298457,20.9668450971377));
#57361=CARTESIAN_POINT('Ctrl Pts',(53.2887683429225,30.7540343399762,20.9710626697866));
#57362=CARTESIAN_POINT('Ctrl Pts',(53.2304108360649,30.6971008975191,20.9752874020054));
#57363=CARTESIAN_POINT('Ctrl Pts',(53.1749193191843,30.6372730886131,20.9795121342242));
#57364=CARTESIAN_POINT('Ctrl Pts',(53.1225799900837,30.5748791561152,20.9837368664431));
#57365=CARTESIAN_POINT('Ctrl Pts',(53.0702537333381,30.5125008072262,20.987960543486));
#57366=CARTESIAN_POINT('Ctrl Pts',(53.0210783544406,30.4475580008846,20.9921842205289));
#57367=CARTESIAN_POINT('Ctrl Pts',(52.9752976029293,30.3804095237632,20.9964078975718));
#57368=CARTESIAN_POINT('Ctrl Pts',(52.9294337890823,30.3131392157595,21.0006392378458));
#57369=CARTESIAN_POINT('Ctrl Pts',(52.8869771541804,30.2436556369514,21.0048705781199));
#57370=CARTESIAN_POINT('Ctrl Pts',(52.8481267011361,30.1723444697001,21.0091019183939));
#57371=CARTESIAN_POINT('Ctrl Pts',(52.8093879048685,30.1012382517985,21.0133210977334));
#57372=CARTESIAN_POINT('Ctrl Pts',(52.7742347124606,30.0283153826651,21.0175402770729));
#57373=CARTESIAN_POINT('Ctrl Pts',(52.7428161308091,29.9539765356991,21.0217594564124));
#57374=CARTESIAN_POINT('Ctrl Pts',(52.7078707023516,29.8712928904894,21.026452253541));
#57375=CARTESIAN_POINT('Ctrl Pts',(52.6774339914087,29.786596450014,21.0311450506696));
#57376=CARTESIAN_POINT('Ctrl Pts',(52.6517168253079,29.700368746774,21.0358378477981));
#57377=CARTESIAN_POINT('Ctrl Pts',(52.6260780328311,29.6144038243387,21.0405163435252));
#57378=CARTESIAN_POINT('Ctrl Pts',(52.6051302149797,29.5269172078913,21.0451948392523));
#57379=CARTESIAN_POINT('Ctrl Pts',(52.5890358675761,29.4384087158869,21.0498733349793));
#57380=CARTESIAN_POINT('Ctrl Pts',(52.5730253979727,29.3503614974848,21.0545274481129));
#57381=CARTESIAN_POINT('Ctrl Pts',(52.5618180620469,29.2613032944131,21.0591815612465));
#57382=CARTESIAN_POINT('Ctrl Pts',(52.5555258256322,29.1717447549387,21.0638356743802));
#57383=CARTESIAN_POINT('Ctrl Pts',(52.551543440014,29.115062739819,21.0667812841741));
#57384=CARTESIAN_POINT('Ctrl Pts',(52.549528920529,29.0581806662824,21.0697268939681));
#57385=CARTESIAN_POINT('Ctrl Pts',(52.5495003092563,29.0012311234037,21.072672503762));
#57386=CARTESIAN_POINT('',(52.5495009304611,28.9978645400587,21.872672503788));
#57387=CARTESIAN_POINT('Ctrl Pts',(52.549500309256,29.0012311229018,21.072672503788));
#57388=CARTESIAN_POINT('Ctrl Pts',(52.5494587751325,28.9185591518343,21.0769485586139));
#57389=CARTESIAN_POINT('Ctrl Pts',(52.5536052143625,28.8358914090988,21.0812246134398));
#57390=CARTESIAN_POINT('Ctrl Pts',(52.561911940885,28.7536732535821,21.0855006682658));
#57391=CARTESIAN_POINT('Ctrl Pts',(52.5702215590747,28.6714264769786,21.0897782116356));
#57392=CARTESIAN_POINT('Ctrl Pts',(52.5826942985601,28.5896300427903,21.0940557550055));
#57393=CARTESIAN_POINT('Ctrl Pts',(52.5992507594021,28.508722752645,21.0983332983753));
#57394=CARTESIAN_POINT('Ctrl Pts',(52.6158308998912,28.4276997459772,21.1026169596419));
#57395=CARTESIAN_POINT('Ctrl Pts',(52.6365063365672,28.3475688614418,21.1069006209084));
#57396=CARTESIAN_POINT('Ctrl Pts',(52.6611468274167,28.2687571627038,21.111184282175));
#57397=CARTESIAN_POINT('Ctrl Pts',(52.6858051125588,28.1898885495789,21.1154710369157));
#57398=CARTESIAN_POINT('Ctrl Pts',(52.7144340011585,28.1123414389407,21.1197577916565));
#57399=CARTESIAN_POINT('Ctrl Pts',(52.7468546537972,28.0365238462294,21.1240445463972));
#57400=CARTESIAN_POINT('Ctrl Pts',(52.7793422161115,27.9605497813275,21.1283401481335));
#57401=CARTESIAN_POINT('Ctrl Pts',(52.8156369841557,27.8863127692337,21.1326357498698));
#57402=CARTESIAN_POINT('Ctrl Pts',(52.8555135416277,27.8141972845966,21.136931351606));
#57403=CARTESIAN_POINT('Ctrl Pts',(52.8911945340563,27.7496693457663,21.1407749966633));
#57404=CARTESIAN_POINT('Ctrl Pts',(52.9297425079146,27.6868398079593,21.1446186417206));
#57405=CARTESIAN_POINT('Ctrl Pts',(52.9709676970025,27.6259628231403,21.1484622867778));
#57406=CARTESIAN_POINT('Ctrl Pts',(53.0163647916923,27.5589252108114,21.1526949009266));
#57407=CARTESIAN_POINT('Ctrl Pts',(53.0651721812789,27.494015173616,21.1569275150754));
#57408=CARTESIAN_POINT('Ctrl Pts',(53.1171636882252,27.4316002827525,21.1611601292241));
#57409=CARTESIAN_POINT('Ctrl Pts',(53.1690810341687,27.3692744208701,21.1653867059462));
#57410=CARTESIAN_POINT('Ctrl Pts',(53.2241731819283,27.3094369904735,21.1696132826683));
#57411=CARTESIAN_POINT('Ctrl Pts',(53.2821708386307,27.2524264758388,21.1738398593905));
#57412=CARTESIAN_POINT('Ctrl Pts',(53.3401041250387,27.1954792358917,21.1780617451302));
#57413=CARTESIAN_POINT('Ctrl Pts',(53.4009361831773,27.1413530014533,21.1822836308699));
#57414=CARTESIAN_POINT('Ctrl Pts',(53.4643585689652,27.0903519577447,21.1865055166096));
#57415=CARTESIAN_POINT('Ctrl Pts',(53.5277381778993,27.0393853129974,21.1907245547902));
#57416=CARTESIAN_POINT('Ctrl Pts',(53.5937042834803,26.9915399629406,21.1949435929708));
#57417=CARTESIAN_POINT('Ctrl Pts',(53.6619137672141,26.9470812281951,21.1991626311515));
#57418=CARTESIAN_POINT('Ctrl Pts',(53.7301009762197,26.90263701205,21.2033802915482));
#57419=CARTESIAN_POINT('Ctrl Pts',(53.800529719589,26.8615774683478,21.207597951945));
#57420=CARTESIAN_POINT('Ctrl Pts',(53.8728273054669,26.8241250112428,21.2118156123417));
#57421=CARTESIAN_POINT('Ctrl Pts',(53.9451233868624,26.7866733335078,21.2160331849707));
#57422=CARTESIAN_POINT('Ctrl Pts',(54.0192878204168,26.7528288057658,21.2202507575997));
#57423=CARTESIAN_POINT('Ctrl Pts',(54.0949239652938,26.7227675521808,21.2244683302287));
#57424=CARTESIAN_POINT('Ctrl Pts',(54.1706885076261,26.6926552675912,21.2286930624716));
#57425=CARTESIAN_POINT('Ctrl Pts',(54.2479293258799,26.6663392792888,21.2329177947145));
#57426=CARTESIAN_POINT('Ctrl Pts',(54.3262300755266,26.6439472970931,21.2371425269573));
#57427=CARTESIAN_POINT('Ctrl Pts',(54.4045112678511,26.6215609077839,21.2413662039811));
#57428=CARTESIAN_POINT('Ctrl Pts',(54.4838514033151,26.603096649577,21.2455898810048));
#57429=CARTESIAN_POINT('Ctrl Pts',(54.5638235285909,26.5886310245445,21.2498135580286));
#57430=CARTESIAN_POINT('Ctrl Pts',(54.6439407513546,26.574139153794,21.254044898284));
#57431=CARTESIAN_POINT('Ctrl Pts',(54.7246917934493,26.5636604748885,21.2582762385395));
#57432=CARTESIAN_POINT('Ctrl Pts',(54.8056433606426,26.5572196687509,21.2625075787949));
#57433=CARTESIAN_POINT('Ctrl Pts',(54.8863622742927,26.5507973733897,21.2667267582444));
#57434=CARTESIAN_POINT('Ctrl Pts',(54.9672801044456,26.5483897026228,21.2709459376938));
#57435=CARTESIAN_POINT('Ctrl Pts',(55.047970226455,26.5499695701127,21.2751651171433));
#57436=CARTESIAN_POINT('Ctrl Pts',(55.1289172820323,26.5515544682182,21.2793977313082));
#57437=CARTESIAN_POINT('Ctrl Pts',(55.2099362412056,26.5571582613561,21.2836303454731));
#57438=CARTESIAN_POINT('Ctrl Pts',(55.2905956447453,26.5667913321593,21.287862959638));
#57439=CARTESIAN_POINT('Ctrl Pts',(55.3711399952143,26.576410662291,21.292089536376));
#57440=CARTESIAN_POINT('Ctrl Pts',(55.4513253512424,26.5900478004067,21.2963161131139));
#57441=CARTESIAN_POINT('Ctrl Pts',(55.5307211804204,26.6076611279643,21.3005426898519));
#57442=CARTESIAN_POINT('Ctrl Pts',(55.6100288895813,26.6252549068032,21.3047645755876));
#57443=CARTESIAN_POINT('Ctrl Pts',(55.6885483618252,26.6468160061563,21.3089864613233));
#57444=CARTESIAN_POINT('Ctrl Pts',(55.7658565217118,26.6722512940286,21.313208347059));
#57445=CARTESIAN_POINT('Ctrl Pts',(55.8431125394759,26.6976694265333,21.3174273852546));
#57446=CARTESIAN_POINT('Ctrl Pts',(55.9191584273671,26.7269564130436,21.3216464234502));
#57447=CARTESIAN_POINT('Ctrl Pts',(55.9935848337678,26.759968877871,21.3258654616459));
#57448=CARTESIAN_POINT('Ctrl Pts',(56.0679869352143,26.7929705620295,21.3300831220573));
#57449=CARTESIAN_POINT('Ctrl Pts',(56.1407701811375,26.8296951201886,21.3343007824686));
#57450=CARTESIAN_POINT('Ctrl Pts',(56.2115451111847,26.8699510114637,21.33851844288));
#57451=CARTESIAN_POINT('Ctrl Pts',(56.2823185684291,26.9102060650271,21.3427360155233));
#57452=CARTESIAN_POINT('Ctrl Pts',(56.3510833896731,26.9539920749009,21.3469535881666));
#57453=CARTESIAN_POINT('Ctrl Pts',(56.4174759059308,27.0010722108826,21.3511711608098));
#57454=CARTESIAN_POINT('Ctrl Pts',(56.4839811274529,27.0482322682091,21.3553958930347));
#57455=CARTESIAN_POINT('Ctrl Pts',(56.5481056057051,27.0986973697519,21.3596206252596));
#57456=CARTESIAN_POINT('Ctrl Pts',(56.6095155561762,27.1521878005525,21.3638453574845));
#57457=CARTESIAN_POINT('Ctrl Pts',(56.6709101686245,27.205664871345,21.3680690345215));
#57458=CARTESIAN_POINT('Ctrl Pts',(56.7295912880466,27.2621654217142,21.3722927115585));
#57459=CARTESIAN_POINT('Ctrl Pts',(56.7852623088348,27.321372960228,21.3765163885955));
#57460=CARTESIAN_POINT('Ctrl Pts',(56.8410343363732,27.380687921975,21.3807477288634));
#57461=CARTESIAN_POINT('Ctrl Pts',(56.8937850490903,27.4427193322646,21.3849790691314));
#57462=CARTESIAN_POINT('Ctrl Pts',(56.9432578582719,27.507117169278,21.3892104093993));
#57463=CARTESIAN_POINT('Ctrl Pts',(56.9925884822932,27.5713299265086,21.3934295887691));
#57464=CARTESIAN_POINT('Ctrl Pts',(57.0386598283554,27.6378951047047,21.3976487681389));
#57465=CARTESIAN_POINT('Ctrl Pts',(57.081262362369,27.7064400945507,21.4018679475087));
#57466=CARTESIAN_POINT('Ctrl Pts',(57.1240005533097,27.7752033484717,21.4061005617814));
#57467=CARTESIAN_POINT('Ctrl Pts',(57.1634067378801,27.8462148067079,21.4103331760541));
#57468=CARTESIAN_POINT('Ctrl Pts',(57.1992373201145,27.9191182026625,21.4145657903268));
#57469=CARTESIAN_POINT('Ctrl Pts',(57.2350167933919,27.9919176087766,21.4187923671731));
#57470=CARTESIAN_POINT('Ctrl Pts',(57.2672305909045,28.0666031792486,21.4230189440194));
#57471=CARTESIAN_POINT('Ctrl Pts',(57.2956792411472,28.1427911154416,21.4272455208658));
#57472=CARTESIAN_POINT('Ctrl Pts',(57.324096315829,28.2188944895624,21.4314674065745));
#57473=CARTESIAN_POINT('Ctrl Pts',(57.3487563852033,28.2964964830853,21.4356892922832));
#57474=CARTESIAN_POINT('Ctrl Pts',(57.3695072481432,28.375191508543,21.4399111779918));
#57475=CARTESIAN_POINT('Ctrl Pts',(57.3902441158939,28.453833459014,21.4441302162965));
#57476=CARTESIAN_POINT('Ctrl Pts',(57.4070768954282,28.5335665292747,21.4483492546013));
#57477=CARTESIAN_POINT('Ctrl Pts',(57.4199030025417,28.6139692910017,21.452568292906));
#57478=CARTESIAN_POINT('Ctrl Pts',(57.4327249211158,28.6943457961152,21.4567859534264));
#57479=CARTESIAN_POINT('Ctrl Pts',(57.4415426926126,28.77539109998,21.4610036139469));
#57480=CARTESIAN_POINT('Ctrl Pts',(57.4463049638303,28.8566742383964,21.4652212744674));
#57481=CARTESIAN_POINT('Ctrl Pts',(57.4510671359466,28.9379556853355,21.4694388472196));
#57482=CARTESIAN_POINT('Ctrl Pts',(57.4517739495821,29.0194744931645,21.4736564199719));
#57483=CARTESIAN_POINT('Ctrl Pts',(57.4484260821981,29.1007966765922,21.4778739927241));
#57484=CARTESIAN_POINT('Ctrl Pts',(57.4450725317982,29.1822569046934,21.48209872482));
#57485=CARTESIAN_POINT('Ctrl Pts',(57.4376505486444,29.2635193739974,21.4863234569158));
#57486=CARTESIAN_POINT('Ctrl Pts',(57.4262130521348,29.3441518206411,21.4905481890116));
#57487=CARTESIAN_POINT('Ctrl Pts',(57.414778411665,29.4247641326805,21.4947718661561));
#57488=CARTESIAN_POINT('Ctrl Pts',(57.3993303722698,29.5047462829996,21.4989955433006));
#57489=CARTESIAN_POINT('Ctrl Pts',(57.3799729426143,29.583677173122,21.5032192204451));
#57490=CARTESIAN_POINT('Ctrl Pts',(57.3605803918034,29.6627512715168,21.5074505608188));
#57491=CARTESIAN_POINT('Ctrl Pts',(57.3372644090129,29.7407698515431,21.5116819011926));
#57492=CARTESIAN_POINT('Ctrl Pts',(57.3101789142712,29.8173271279338,21.5159132415663));
#57493=CARTESIAN_POINT('Ctrl Pts',(57.2831712679286,29.8936643654639,21.5201324203356));
#57494=CARTESIAN_POINT('Ctrl Pts',(57.2524159990534,29.9685482987032,21.5243515991049));
#57495=CARTESIAN_POINT('Ctrl Pts',(57.2181115911092,30.041600316526,21.5285707778742));
#57496=CARTESIAN_POINT('Ctrl Pts',(57.1836979469842,30.1148849552832,21.5328033918549));
#57497=CARTESIAN_POINT('Ctrl Pts',(57.1455845058485,30.1865985476052,21.5370360058357));
#57498=CARTESIAN_POINT('Ctrl Pts',(57.1039374992242,30.2563428072618,21.5412686198164));
#57499=CARTESIAN_POINT('Ctrl Pts',(57.0623498981447,30.32598758328,21.5454951963707));
#57500=CARTESIAN_POINT('Ctrl Pts',(57.0172389784502,30.3936682102684,21.549721772925));
#57501=CARTESIAN_POINT('Ctrl Pts',(56.968818087626,30.4590084262391,21.5539483494793));
#57502=CARTESIAN_POINT('Ctrl Pts',(56.9204509356576,30.5242761258149,21.558170235261));
#57503=CARTESIAN_POINT('Ctrl Pts',(56.8687813869854,30.5872082041524,21.5623921210426));
#57504=CARTESIAN_POINT('Ctrl Pts',(56.8140668002175,30.6474561889011,21.5666140068243));
#57505=CARTESIAN_POINT('Ctrl Pts',(56.7593891198028,30.7076635348818,21.5708330448388));
#57506=CARTESIAN_POINT('Ctrl Pts',(56.7016707921346,30.7651900400527,21.5750520828532));
#57507=CARTESIAN_POINT('Ctrl Pts',(56.6412094749597,30.819720228305,21.5792711208676));
#57508=CARTESIAN_POINT('Ctrl Pts',(56.5807679022313,30.8742326089998,21.5834887810992));
#57509=CARTESIAN_POINT('Ctrl Pts',(56.5175854636253,30.925750305101,21.5877064413307));
#57510=CARTESIAN_POINT('Ctrl Pts',(56.4519957060219,30.9739956230179,21.5919241015622));
#57511=CARTESIAN_POINT('Ctrl Pts',(56.386407313295,31.0222399369839,21.5961416740272));
#57512=CARTESIAN_POINT('Ctrl Pts',(56.3184120760833,31.067211733845,21.6003592464922));
#57513=CARTESIAN_POINT('Ctrl Pts',(56.2483744009694,31.108675319959,21.6045768189572));
#57514=CARTESIAN_POINT('Ctrl Pts',(56.1782178261752,31.1502092968609,21.6088015513974));
#57515=CARTESIAN_POINT('Ctrl Pts',(56.1060122779705,31.1882229090948,21.6130262838376));
#57516=CARTESIAN_POINT('Ctrl Pts',(56.0321491596884,31.2225252219389,21.6172510162778));
#57517=CARTESIAN_POINT('Ctrl Pts',(55.9583044965698,31.2568189641349,21.6214746931421));
#57518=CARTESIAN_POINT('Ctrl Pts',(55.8828035316091,31.2874031059727,21.6256983700064));
#57519=CARTESIAN_POINT('Ctrl Pts',(55.8060561151941,31.3141356462313,21.6299220468707));
#57520=CARTESIAN_POINT('Ctrl Pts',(55.7291694519662,31.3409166887223,21.6341533869707));
#57521=CARTESIAN_POINT('Ctrl Pts',(55.6510322648193,31.3638320329228,21.6383847270707));
#57522=CARTESIAN_POINT('Ctrl Pts',(55.5720687308181,31.3827898810471,21.6426160671707));
#57523=CARTESIAN_POINT('Ctrl Pts',(55.4933321169684,31.4016932493684,21.646835247527));
#57524=CARTESIAN_POINT('Ctrl Pts',(55.4137743621044,31.4166618343841,21.6510544278833));
#57525=CARTESIAN_POINT('Ctrl Pts',(55.3338211098633,31.4276560128259,21.6552736082396));
#57526=CARTESIAN_POINT('Ctrl Pts',(55.2536132871638,31.438685196636,21.6595062224294));
#57527=CARTESIAN_POINT('Ctrl Pts',(55.1727091253607,31.4457556181,21.6637388366191));
#57528=CARTESIAN_POINT('Ctrl Pts',(55.0915332135982,31.4487898890694,21.6679714508089));
#57529=CARTESIAN_POINT('Ctrl Pts',(55.0104730916868,31.4518198319348,21.6721980275701));
#57530=CARTESIAN_POINT('Ctrl Pts',(54.929142450058,31.4508250416212,21.6764246043314));
#57531=CARTESIAN_POINT('Ctrl Pts',(54.8479730533334,31.4457796420543,21.6806511810926));
#57532=CARTESIAN_POINT('Ctrl Pts',(54.7668937456387,31.4407398423214,21.6848730668223));
#57533=CARTESIAN_POINT('Ctrl Pts',(54.6859757885639,31.4316583950109,21.689094952552));
#57534=CARTESIAN_POINT('Ctrl Pts',(54.6056515956935,31.418561470383,21.6933168382817));
#57535=CARTESIAN_POINT('Ctrl Pts',(54.5253815786919,31.4054733791742,21.6975358764966));
#57536=CARTESIAN_POINT('Ctrl Pts',(54.4457049878306,31.3883752641321,21.7017549147115));
#57537=CARTESIAN_POINT('Ctrl Pts',(54.3670484975769,31.3673450626346,21.7059739529264));
#57538=CARTESIAN_POINT('Ctrl Pts',(54.2884176936976,31.3463217288428,21.7101916133555));
#57539=CARTESIAN_POINT('Ctrl Pts',(54.2108067772946,31.3213689785938,21.7144092737846));
#57540=CARTESIAN_POINT('Ctrl Pts',(54.1346302679803,31.2926154228095,21.7186269342137));
#57541=CARTESIAN_POINT('Ctrl Pts',(54.0584553439017,31.2638624653878,21.7228445068731));
#57542=CARTESIAN_POINT('Ctrl Pts',(53.9837152017648,31.2313090248411,21.7270620795326));
#57543=CARTESIAN_POINT('Ctrl Pts',(53.9108059306148,31.1951324627949,21.731279652192));
#57544=CARTESIAN_POINT('Ctrl Pts',(53.8377728923112,31.1588944892158,21.7355043843931));
#57545=CARTESIAN_POINT('Ctrl Pts',(53.7665773616964,31.11902129613,21.7397291165942));
#57546=CARTESIAN_POINT('Ctrl Pts',(53.6975925798467,31.0757372574412,21.7439538487953));
#57547=CARTESIAN_POINT('Ctrl Pts',(53.6286250273542,31.0324640291971,21.7481775258445));
#57548=CARTESIAN_POINT('Ctrl Pts',(53.5618674893088,30.9857819434466,21.7524012028938));
#57549=CARTESIAN_POINT('Ctrl Pts',(53.4976622028408,30.9359574874534,21.756624879943));
#57550=CARTESIAN_POINT('Ctrl Pts',(53.4333404255097,30.8860426324572,21.7608562202208));
#57551=CARTESIAN_POINT('Ctrl Pts',(53.3715805073717,30.8329743168813,21.7650875604986));
#57552=CARTESIAN_POINT('Ctrl Pts',(53.3126903731069,30.7770583763607,21.7693189007764));
#57553=CARTESIAN_POINT('Ctrl Pts',(53.2539694908919,30.7213031399661,21.7735380800526));
#57554=CARTESIAN_POINT('Ctrl Pts',(53.1981021728646,30.6627170119578,21.7777572593289));
#57555=CARTESIAN_POINT('Ctrl Pts',(53.1453533765797,30.6016354617189,21.7819764386051));
#57556=CARTESIAN_POINT('Ctrl Pts',(53.0928691983639,30.540860331399,21.7861744520699));
#57557=CARTESIAN_POINT('Ctrl Pts',(53.0432691804079,30.4773793757769,21.7903724655347));
#57558=CARTESIAN_POINT('Ctrl Pts',(52.9968478027444,30.41149974305,21.7945704789996));
#57559=CARTESIAN_POINT('Ctrl Pts',(52.9504882732555,30.3457078831388,21.7987628993631));
#57560=CARTESIAN_POINT('Ctrl Pts',(52.9072992512303,30.2775240690775,21.8029553197265));
#57561=CARTESIAN_POINT('Ctrl Pts',(52.8675363449773,30.2072899444654,21.80714774009));
#57562=CARTESIAN_POINT('Ctrl Pts',(52.8278137653434,30.1371270496766,21.8113359085978));
#57563=CARTESIAN_POINT('Ctrl Pts',(52.7915106365121,30.0649183802912,21.8155240771056));
#57564=CARTESIAN_POINT('Ctrl Pts',(52.7588395490466,29.9910348546253,21.8197122456134));
#57565=CARTESIAN_POINT('Ctrl Pts',(52.7261912053985,29.917202762614,21.8238974985482));
#57566=CARTESIAN_POINT('Ctrl Pts',(52.6971700725693,29.8416985607465,21.828082751483));
#57567=CARTESIAN_POINT('Ctrl Pts',(52.6719422981615,29.7649167189378,21.8322680044178));
#57568=CARTESIAN_POINT('Ctrl Pts',(52.6467190670668,29.6881487049025,21.8364525036233));
#57569=CARTESIAN_POINT('Ctrl Pts',(52.6252879935756,29.6101039537651,21.8406370028287));
#57570=CARTESIAN_POINT('Ctrl Pts',(52.6077662033998,29.5311946087863,21.8448215020342));
#57571=CARTESIAN_POINT('Ctrl Pts',(52.5902459033006,29.4522919743648,21.8490056453841));
#57572=CARTESIAN_POINT('Ctrl Pts',(52.5766343209221,29.3725253552373,21.8531897887341));
#57573=CARTESIAN_POINT('Ctrl Pts',(52.5669976351947,29.2923178798019,21.8573739320841));
#57574=CARTESIAN_POINT('Ctrl Pts',(52.5573558623475,29.2120680635605,21.8615602842058));
#57575=CARTESIAN_POINT('Ctrl Pts',(52.5516932194495,29.1313773970183,21.8657466363275));
#57576=CARTESIAN_POINT('Ctrl Pts',(52.5500239961797,29.0506737674197,21.8699329884492));
#57577=CARTESIAN_POINT('Ctrl Pts',(52.5496598873948,29.0330698308851,21.8708461602288));
#57578=CARTESIAN_POINT('Ctrl Pts',(52.5494855924957,29.0154652775853,21.8717593320084));
#57579=CARTESIAN_POINT('Ctrl Pts',(52.5495009304611,28.9978645400587,21.872672503788));
#57580=CARTESIAN_POINT('',(52.5491321430934,29.0004423866234,22.672672503788));
#57581=CARTESIAN_POINT('Ctrl Pts',(52.5506947500799,28.9978548628947,21.8726730601105));
#57582=CARTESIAN_POINT('Ctrl Pts',(52.548747042966,28.7666343434887,21.8846751297305));
#57583=CARTESIAN_POINT('Ctrl Pts',(52.6846919919135,27.7240147216207,21.9389114761391));
#57584=CARTESIAN_POINT('Ctrl Pts',(54.1644763874256,26.2292359076652,22.0353820993358));
#57585=CARTESIAN_POINT('Ctrl Pts',(56.869326740188,26.7907356786193,22.1620849297015));
#57586=CARTESIAN_POINT('Ctrl Pts',(57.870850319864,29.365312819345,22.2887877600669));
#57587=CARTESIAN_POINT('Ctrl Pts',(56.2564582705911,31.6070189140945,22.4154905904323));
#57588=CARTESIAN_POINT('Ctrl Pts',(53.4971863067911,31.4732108227925,22.5421934207978));
#57589=CARTESIAN_POINT('Ctrl Pts',(52.5567672100938,29.8579006357823,22.6279207252497));
#57590=CARTESIAN_POINT('Ctrl Pts',(52.5455403995099,29.0245626904411,22.6714137529131));
#57591=CARTESIAN_POINT('Ctrl Pts',(52.5456007000401,29.000443024056,22.672672503788));
#57592=CARTESIAN_POINT('',(52.5495006321937,29.0017602218196,23.4726725037595));
#57593=CARTESIAN_POINT('Ctrl Pts',(52.5495000399198,29.0004423202172,22.672672503788));
#57594=CARTESIAN_POINT('Ctrl Pts',(52.5494854961293,28.919868209688,22.6768841776903));
#57595=CARTESIAN_POINT('Ctrl Pts',(52.5534492292258,28.8391374882827,22.6810958515925));
#57596=CARTESIAN_POINT('Ctrl Pts',(52.5614115129766,28.7586777238696,22.6853075254948));
#57597=CARTESIAN_POINT('Ctrl Pts',(52.569362527487,28.6783318363859,22.6895132384985));
#57598=CARTESIAN_POINT('Ctrl Pts',(52.5813008096307,28.5982566078266,22.6937189515022));
#57599=CARTESIAN_POINT('Ctrl Pts',(52.597194621011,28.5188798895268,22.6979246645059));
#57600=CARTESIAN_POINT('Ctrl Pts',(52.6130706107374,28.4395921759584,22.7021256616639));
#57601=CARTESIAN_POINT('Ctrl Pts',(52.6328932252952,28.3610018745935,22.706326658822));
#57602=CARTESIAN_POINT('Ctrl Pts',(52.6565790673927,28.2835304733502,22.71052765598));
#57603=CARTESIAN_POINT('Ctrl Pts',(52.6802505614431,28.206106001547,22.7147261083222));
#57604=CARTESIAN_POINT('Ctrl Pts',(52.7077805016829,28.1297995327349,22.7189245606644));
#57605=CARTESIAN_POINT('Ctrl Pts',(52.7390349626928,28.0550199208054,22.7231230130067));
#57606=CARTESIAN_POINT('Ctrl Pts',(52.7702802942635,27.9802621520272,22.7273202389795));
#57607=CARTESIAN_POINT('Ctrl Pts',(52.8052478053248,27.9070307876049,22.7315174649523));
#57608=CARTESIAN_POINT('Ctrl Pts',(52.8437550311147,27.8357157202139,22.7357146909251));
#57609=CARTESIAN_POINT('Ctrl Pts',(52.8822630871812,27.7643991151575,22.7399120073967));
#57610=CARTESIAN_POINT('Ctrl Pts',(52.9243107847905,27.6949993015931,22.7441093238684));
#57611=CARTESIAN_POINT('Ctrl Pts',(52.9696699184124,27.6278811969073,22.74830664034));
#57612=CARTESIAN_POINT('Ctrl Pts',(53.0150744453103,27.5606959235962,22.7525081572875));
#57613=CARTESIAN_POINT('Ctrl Pts',(53.0637967619506,27.495797308667,22.756709674235));
#57614=CARTESIAN_POINT('Ctrl Pts',(53.1155659285187,27.4335203543486,22.7609111911824));
#57615=CARTESIAN_POINT('Ctrl Pts',(53.1673618396172,27.371211227059,22.7651148786806));
#57616=CARTESIAN_POINT('Ctrl Pts',(53.2222074163188,27.311526802737,22.7693185661787));
#57617=CARTESIAN_POINT('Ctrl Pts',(53.2797938234318,27.2547662162058,22.7735222536768));
#57618=CARTESIAN_POINT('Ctrl Pts',(53.3374798801209,27.1979074091279,22.777733215386));
#57619=CARTESIAN_POINT('Ctrl Pts',(53.3979158884207,27.1439828571651,22.7819441770951));
#57620=CARTESIAN_POINT('Ctrl Pts',(53.460759110503,27.0932520528133,22.7861551388043));
#57621=CARTESIAN_POINT('Ctrl Pts',(53.5077387025736,27.0553273186115,22.7893031197124));
#57622=CARTESIAN_POINT('Ctrl Pts',(53.5560628805733,27.01918660076,22.7924511006206));
#57623=CARTESIAN_POINT('Ctrl Pts',(53.605578671413,26.9849219845421,22.7955990815287));
#57624=CARTESIAN_POINT('Ctrl Pts',(53.6721564963022,26.9388505479405,22.7998317862498));
#57625=CARTESIAN_POINT('Ctrl Pts',(53.7411438564632,26.8959965689133,22.8040644909709));
#57626=CARTESIAN_POINT('Ctrl Pts',(53.8121968913307,26.8566208863023,22.808297195692));
#57627=CARTESIAN_POINT('Ctrl Pts',(53.8831485682075,26.8173013735661,22.81252386241));
#57628=CARTESIAN_POINT('Ctrl Pts',(53.9561596643074,26.781450525695,22.816750529128));
#57629=CARTESIAN_POINT('Ctrl Pts',(54.0308566493132,26.7492864651805,22.820977195846));
#57630=CARTESIAN_POINT('Ctrl Pts',(54.1054687422099,26.717158958684,22.8251990590147));
#57631=CARTESIAN_POINT('Ctrl Pts',(54.1817624918819,26.6887100955654,22.8294209221834));
#57632=CARTESIAN_POINT('Ctrl Pts',(54.2593403113337,26.6641118443759,22.8336427853521));
#57633=CARTESIAN_POINT('Ctrl Pts',(54.3368678372452,26.639529540182,22.8378619114955));
#57634=CARTESIAN_POINT('Ctrl Pts',(54.4156773384656,26.6187930314796,22.842081037639));
#57635=CARTESIAN_POINT('Ctrl Pts',(54.4953529332376,26.602025523904,22.8463001637825));
#57636=CARTESIAN_POINT('Ctrl Pts',(54.5750024913493,26.5852634956711,22.8505179111857));
#57637=CARTESIAN_POINT('Ctrl Pts',(54.6555171267196,26.5724679883814,22.8547356585889));
#57638=CARTESIAN_POINT('Ctrl Pts',(54.736468911574,26.563711508168,22.8589534059921));
#57639=CARTESIAN_POINT('Ctrl Pts',(54.8174189913709,26.5549552123892,22.8631710645584));
#57640=CARTESIAN_POINT('Ctrl Pts',(54.8988057403859,26.5502378233306,22.8673887231247));
#57641=CARTESIAN_POINT('Ctrl Pts',(54.9801956520729,26.5495800282802,22.871606381691));
#57642=CARTESIAN_POINT('Ctrl Pts',(55.0617200464984,26.5489211463374,22.875831009208));
#57643=CARTESIAN_POINT('Ctrl Pts',(55.1432471471763,26.5523352820255,22.8800556367249));
#57644=CARTESIAN_POINT('Ctrl Pts',(55.2243426530845,26.5597908646989,22.8842802642418));
#57645=CARTESIAN_POINT('Ctrl Pts',(55.3054214966236,26.5672449155036,22.8885040237414));
#57646=CARTESIAN_POINT('Ctrl Pts',(55.3860684642249,26.5787386663093,22.8927277832411));
#57647=CARTESIAN_POINT('Ctrl Pts',(55.4658578327119,26.5941889663357,22.8969515427407));
#57648=CARTESIAN_POINT('Ctrl Pts',(55.5457919129972,26.6096672881492,22.9011829627575));
#57649=CARTESIAN_POINT('Ctrl Pts',(55.6248648333497,26.6291163886836,22.9054143827744));
#57650=CARTESIAN_POINT('Ctrl Pts',(55.7026637074587,26.6524025123074,22.9096458027913));
#57651=CARTESIAN_POINT('Ctrl Pts',(55.7802287671693,26.6756186525151,22.9138645058256));
#57652=CARTESIAN_POINT('Ctrl Pts',(55.8565270271489,26.7026485535667,22.9180832088599));
#57653=CARTESIAN_POINT('Ctrl Pts',(55.931170698421,26.7333126857897,22.9223019118942));
#57654=CARTESIAN_POINT('Ctrl Pts',(56.0060634968536,26.7640791611592,22.9265346950707));
#57655=CARTESIAN_POINT('Ctrl Pts',(56.0795690231587,26.7986185579771,22.9307674782472));
#57656=CARTESIAN_POINT('Ctrl Pts',(56.1512812722436,26.8367844115343,22.9350002614237));
#57657=CARTESIAN_POINT('Ctrl Pts',(56.2228912622086,26.8748958419399,22.9392270088018));
#57658=CARTESIAN_POINT('Ctrl Pts',(56.2927126471501,26.9166232419716,22.9434537561799));
#57659=CARTESIAN_POINT('Ctrl Pts',(56.3603591041834,26.961772005475,22.947680503558));
#57660=CARTESIAN_POINT('Ctrl Pts',(56.427927663553,27.0068687783296,22.9519023836634));
#57661=CARTESIAN_POINT('Ctrl Pts',(56.493325888301,27.055378827783,22.9561242637689));
#57662=CARTESIAN_POINT('Ctrl Pts',(56.5561930932482,27.1070622549786,22.9603461438744));
#57663=CARTESIAN_POINT('Ctrl Pts',(56.6190205601834,27.1587130133662,22.9645653553529));
#57664=CARTESIAN_POINT('Ctrl Pts',(56.679319825331,27.2135328734199,22.9687845668314));
#57665=CARTESIAN_POINT('Ctrl Pts',(56.7367611320787,27.2712400339837,22.9730037783098));
#57666=CARTESIAN_POINT('Ctrl Pts',(56.7941836897897,27.3289283587352,22.9772216126234));
#57667=CARTESIAN_POINT('Ctrl Pts',(56.8487498142394,27.3895017834338,22.981439446937));
#57668=CARTESIAN_POINT('Ctrl Pts',(56.9001657205332,27.4526408030097,22.9856572812506));
#57669=CARTESIAN_POINT('Ctrl Pts',(56.9515805615183,27.5157785143805,22.989875028173));
#57670=CARTESIAN_POINT('Ctrl Pts',(56.9998450217247,27.5814813540094,22.9940927750954));
#57671=CARTESIAN_POINT('Ctrl Pts',(57.0447057472779,27.6493969283876,22.9983105220178));
#57672=CARTESIAN_POINT('Ctrl Pts',(57.0896384950068,27.7174215386179,23.0025350403713));
#57673=CARTESIAN_POINT('Ctrl Pts',(57.1311563189547,27.7876656008117,23.0067595587248));
#57674=CARTESIAN_POINT('Ctrl Pts',(57.1690492973634,27.859747661433,23.0109840770783));
#57675=CARTESIAN_POINT('Ctrl Pts',(57.2069362845994,27.9318183253237,23.0152079275028));
#57676=CARTESIAN_POINT('Ctrl Pts',(57.2411993949561,28.0057259750564,23.0194317779273));
#57677=CARTESIAN_POINT('Ctrl Pts',(57.2716766127879,28.0810682196636,23.0236556283517));
#57678=CARTESIAN_POINT('Ctrl Pts',(57.3022091107209,28.1565471213279,23.0278871400687));
#57679=CARTESIAN_POINT('Ctrl Pts',(57.3289418398862,28.2334653780283,23.0321186517856));
#57680=CARTESIAN_POINT('Ctrl Pts',(57.3517622218452,28.3114038179733,23.0363501635025));
#57681=CARTESIAN_POINT('Ctrl Pts',(57.374510776033,28.3890969445644,23.0405683564215));
#57682=CARTESIAN_POINT('Ctrl Pts',(57.3933715521117,28.4678033798409,23.0447865493405));
#57683=CARTESIAN_POINT('Ctrl Pts',(57.4082840533503,28.5471002667491,23.0490047422596));
#57684=CARTESIAN_POINT('Ctrl Pts',(57.4232450343868,28.6266549438826,23.0532366483134));
#57685=CARTESIAN_POINT('Ctrl Pts',(57.4342876721786,28.707099976781,23.0574685543673));
#57686=CARTESIAN_POINT('Ctrl Pts',(57.4413137261738,28.7880152354636,23.0617004604211));
#57687=CARTESIAN_POINT('Ctrl Pts',(57.4483297544047,28.868815032849,23.0659263277949));
#57688=CARTESIAN_POINT('Ctrl Pts',(57.4513405422157,28.9500832642489,23.0701521951687));
#57689=CARTESIAN_POINT('Ctrl Pts',(57.4502989434788,29.0313900873962,23.0743780625424));
#57690=CARTESIAN_POINT('Ctrl Pts',(57.4492582824699,29.1126237118335,23.0786001254625));
#57691=CARTESIAN_POINT('Ctrl Pts',(57.4441724786708,29.1938953965611,23.0828221883826));
#57692=CARTESIAN_POINT('Ctrl Pts',(57.4350463452106,29.2747718083732,23.0870442513027));
#57693=CARTESIAN_POINT('Ctrl Pts',(57.4259282784988,29.3555767321143,23.0912625822678));
#57694=CARTESIAN_POINT('Ctrl Pts',(57.412777039292,29.4359866172132,23.0954809132328));
#57695=CARTESIAN_POINT('Ctrl Pts',(57.3956494303402,29.5155715827224,23.0996992441979));
#57696=CARTESIAN_POINT('Ctrl Pts',(57.378527405954,29.5951305990483,23.1039161997494));
#57697=CARTESIAN_POINT('Ctrl Pts',(57.3574316843034,29.6738647759658,23.1081331553008));
#57698=CARTESIAN_POINT('Ctrl Pts',(57.332470278992,29.751353876425,23.1123501108523));
#57699=CARTESIAN_POINT('Ctrl Pts',(57.3075093735703,29.8288414250484,23.1165669819529));
#57700=CARTESIAN_POINT('Ctrl Pts',(57.2786830820212,29.9050835048136,23.1207838530535));
#57701=CARTESIAN_POINT('Ctrl Pts',(57.2461490167081,29.9796758875982,23.1250007241541));
#57702=CARTESIAN_POINT('Ctrl Pts',(57.2135478320734,30.0544221580103,23.12922629486));
#57703=CARTESIAN_POINT('Ctrl Pts',(57.1772237493577,30.1275114901386,23.1334518655659));
#57704=CARTESIAN_POINT('Ctrl Pts',(57.137382692401,30.1985597507946,23.1376774362718));
#57705=CARTESIAN_POINT('Ctrl Pts',(57.0975659613505,30.2695646312428,23.1419004269549));
#57706=CARTESIAN_POINT('Ctrl Pts',(57.0542368184479,30.3385305499311,23.146123417638));
#57707=CARTESIAN_POINT('Ctrl Pts',(57.0076445567346,30.4051026951131,23.150346408321));
#57708=CARTESIAN_POINT('Ctrl Pts',(56.9609675864406,30.4717958739544,23.15457707675));
#57709=CARTESIAN_POINT('Ctrl Pts',(56.911015927208,30.5360862138174,23.158807745179));
#57710=CARTESIAN_POINT('Ctrl Pts',(56.8580798572149,30.5976512429852,23.1630384136079));
#57711=CARTESIAN_POINT('Ctrl Pts',(56.8052390749021,30.6591054518972,23.1672614666136));
#57712=CARTESIAN_POINT('Ctrl Pts',(56.749424987471,30.7178438735892,23.1714845196193));
#57713=CARTESIAN_POINT('Ctrl Pts',(56.6909606339623,30.7735846143869,23.175707572625));
#57714=CARTESIAN_POINT('Ctrl Pts',(56.6323519679936,30.8294629447232,23.1799410497461));
#57715=CARTESIAN_POINT('Ctrl Pts',(56.5708617343952,30.8825367923476,23.1841745268672));
#57716=CARTESIAN_POINT('Ctrl Pts',(56.5067891491679,30.932494944353,23.1884080039883));
#57717=CARTESIAN_POINT('Ctrl Pts',(56.4428079928384,30.9823818081662,23.1926354401147));
#57718=CARTESIAN_POINT('Ctrl Pts',(56.3762521668127,31.0291615235634,23.1968628762411));
#57719=CARTESIAN_POINT('Ctrl Pts',(56.3074568365328,31.0725604624724,23.2010903123675));
#57720=CARTESIAN_POINT('Ctrl Pts',(56.2387408920317,31.1159093215496,23.2053128702804));
#57721=CARTESIAN_POINT('Ctrl Pts',(56.1677909702052,31.1558849113241,23.2095354281933));
#57722=CARTESIAN_POINT('Ctrl Pts',(56.0949731587571,31.1922554667742,23.2137579861062));
#57723=CARTESIAN_POINT('Ctrl Pts',(56.0222014869416,31.228602976708,23.217977868475));
#57724=CARTESIAN_POINT('Ctrl Pts',(55.9475646893086,31.2613497799502,23.2221977508437));
#57725=CARTESIAN_POINT('Ctrl Pts',(55.8714545274654,31.2903094237592,23.2264176332125));
#57726=CARTESIAN_POINT('Ctrl Pts',(55.7953693443882,31.3192595632372,23.2306361306485));
#57727=CARTESIAN_POINT('Ctrl Pts',(55.7178121910653,31.3444248466661,23.2348546280845));
#57728=CARTESIAN_POINT('Ctrl Pts',(55.6391946167058,31.3656670289739,23.2390731255206));
#57729=CARTESIAN_POINT('Ctrl Pts',(55.5605788317492,31.3869087277916,23.24329152694));
#57730=CARTESIAN_POINT('Ctrl Pts',(55.4809031223186,31.4042273830283,23.2475099283594));
#57731=CARTESIAN_POINT('Ctrl Pts',(55.4005926132802,31.4175350686568,23.2517283297788));
#57732=CARTESIAN_POINT('Ctrl Pts',(55.3201849206094,31.4308588578967,23.2559518358798));
#57733=CARTESIAN_POINT('Ctrl Pts',(55.239141352318,31.4401618984881,23.2601753419808));
#57734=CARTESIAN_POINT('Ctrl Pts',(55.1578953815873,31.4454077979906,23.2643988480818));
#57735=CARTESIAN_POINT('Ctrl Pts',(55.0766307334054,31.4506549034611,23.2686233251149));
#57736=CARTESIAN_POINT('Ctrl Pts',(54.9951640556022,31.4518430123114,23.2728478021481));
#57737=CARTESIAN_POINT('Ctrl Pts',(54.9139289520395,31.4489879592809,23.2770722791813));
#57738=CARTESIAN_POINT('Ctrl Pts',(54.8325469465271,31.4461277432995,23.2813043955709));
#57739=CARTESIAN_POINT('Ctrl Pts',(54.7513978161741,31.4392097931619,23.2855365119605));
#57740=CARTESIAN_POINT('Ctrl Pts',(54.6709103675634,31.4283019301196,23.2897686283501));
#57741=CARTESIAN_POINT('Ctrl Pts',(54.590768889633,31.4174409539009,23.2939825532303));
#57742=CARTESIAN_POINT('Ctrl Pts',(54.5112838436527,31.4026244700762,23.2981964781104));
#57743=CARTESIAN_POINT('Ctrl Pts',(54.4328647967604,31.3839689409148,23.3024104029905));
#57744=CARTESIAN_POINT('Ctrl Pts',(54.3540815518368,31.3652267707234,23.3066438984113));
#57745=CARTESIAN_POINT('Ctrl Pts',(54.2760824579198,31.3425403614949,23.3108773938321));
#57746=CARTESIAN_POINT('Ctrl Pts',(54.1992914755943,31.3159913879253,23.3151108892528));
#57747=CARTESIAN_POINT('Ctrl Pts',(54.1226097793403,31.2894801978679,23.3193383597203));
#57748=CARTESIAN_POINT('Ctrl Pts',(54.0471332150036,31.2591175119583,23.3235658301878));
#57749=CARTESIAN_POINT('Ctrl Pts',(53.9732737720535,31.2250356183322,23.3277933006553));
#57750=CARTESIAN_POINT('Ctrl Pts',(53.8994991426381,31.1909928612843,23.3320159166763));
#57751=CARTESIAN_POINT('Ctrl Pts',(53.8273383633754,31.1532395782488,23.3362385326972));
#57752=CARTESIAN_POINT('Ctrl Pts',(53.7571851303894,31.1119567821986,23.3404611487182));
#57753=CARTESIAN_POINT('Ctrl Pts',(53.6870761096498,31.0707000035546,23.3446811035455));
#57754=CARTESIAN_POINT('Ctrl Pts',(53.6189725226876,31.0259183624577,23.3489010583729));
#57755=CARTESIAN_POINT('Ctrl Pts',(53.5532440202676,30.9778390695678,23.3531210132002));
#57756=CARTESIAN_POINT('Ctrl Pts',(53.4875368691057,30.9297753947636,23.3573395972166));
#57757=CARTESIAN_POINT('Ctrl Pts',(53.4242036447361,30.8784164694774,23.3615581812331));
#57758=CARTESIAN_POINT('Ctrl Pts',(53.3635843207133,30.8240323392376,23.3657767652496));
#57759=CARTESIAN_POINT('Ctrl Pts',(53.3029661765759,30.7696492675224,23.3699952671561));
#57760=CARTESIAN_POINT('Ctrl Pts',(53.2450621725797,30.7122414188741,23.3742137690627));
#57761=CARTESIAN_POINT('Ctrl Pts',(53.190177453739,30.6521176111419,23.3784322709693));
#57762=CARTESIAN_POINT('Ctrl Pts',(53.1352288323094,30.5919238009201,23.3826556845015));
#57763=CARTESIAN_POINT('Ctrl Pts',(53.0833068366663,30.5290080549053,23.3868790980337));
#57764=CARTESIAN_POINT('Ctrl Pts',(53.0346778820942,30.463714187562,23.391102511566));
#57765=CARTESIAN_POINT('Ctrl Pts',(52.9860351509877,30.3984018225311,23.3953271215871));
#57766=CARTESIAN_POINT('Ctrl Pts',(52.9406875724281,30.3307103846163,23.3995517316081));
#57767=CARTESIAN_POINT('Ctrl Pts',(52.8988578576523,30.2610122710151,23.4037763416292));
#57768=CARTESIAN_POINT('Ctrl Pts',(52.8569523224409,30.1911878227886,23.4080086091678));
#57769=CARTESIAN_POINT('Ctrl Pts',(52.8185776136158,30.1193498405798,23.4122408767063));
#57770=CARTESIAN_POINT('Ctrl Pts',(52.7839102182845,30.0458949896506,23.4164731442449));
#57771=CARTESIAN_POINT('Ctrl Pts',(52.7493976737093,29.9727682435327,23.4206865072819));
#57772=CARTESIAN_POINT('Ctrl Pts',(52.7185594783011,29.8980394955953,23.424899870319));
#57773=CARTESIAN_POINT('Ctrl Pts',(52.6915207808602,29.8221155300805,23.429113233356));
#57774=CARTESIAN_POINT('Ctrl Pts',(52.6599923408405,29.7335844831239,23.4340262201626));
#57775=CARTESIAN_POINT('Ctrl Pts',(52.6335319134128,29.6431573818611,23.4389392069691));
#57776=CARTESIAN_POINT('Ctrl Pts',(52.6123377738553,29.5513794916768,23.4438521937757));
#57777=CARTESIAN_POINT('Ctrl Pts',(52.5913329406732,29.460421362997,23.4487212977097));
#57778=CARTESIAN_POINT('Ctrl Pts',(52.575500818871,29.3681366175074,23.4535904016438));
#57779=CARTESIAN_POINT('Ctrl Pts',(52.5649881187031,29.2750770581904,23.4584595055778));
#57780=CARTESIAN_POINT('Ctrl Pts',(52.5547592011312,29.1845295731178,23.4631971716384));
#57781=CARTESIAN_POINT('Ctrl Pts',(52.5495663494456,29.0932487390193,23.4679348376989));
#57782=CARTESIAN_POINT('Ctrl Pts',(52.5495006321937,29.0017602218196,23.4726725037595));
#57783=CARTESIAN_POINT('',(57.0573849385052,27.6687909762881,23.799499905797));
#57784=CARTESIAN_POINT('Ctrl Pts',(52.5495006321933,29.001760221269,23.472672503788));
#57785=CARTESIAN_POINT('Ctrl Pts',(52.5494421473559,28.92034031141,23.4768887743692));
#57786=CARTESIAN_POINT('Ctrl Pts',(52.5534458492211,28.8388797722771,23.4811050449504));
#57787=CARTESIAN_POINT('Ctrl Pts',(52.5614972674082,28.7578127312551,23.4853213155316));
#57788=CARTESIAN_POINT('Ctrl Pts',(52.5695478980543,28.6767536197193,23.4895371737028));
#57789=CARTESIAN_POINT('Ctrl Pts',(52.5816454122911,28.5960883915437,23.493753031874));
#57790=CARTESIAN_POINT('Ctrl Pts',(52.5977234365795,28.5162463820906,23.4979688900453));
#57791=CARTESIAN_POINT('Ctrl Pts',(52.6138047898605,28.4363878411622,23.5021856211198));
#57792=CARTESIAN_POINT('Ctrl Pts',(52.6338681970555,28.3573533120643,23.5064023521943));
#57793=CARTESIAN_POINT('Ctrl Pts',(52.6577964014843,28.2795608609326,23.5106190832688));
#57794=CARTESIAN_POINT('Ctrl Pts',(52.6817534461576,28.2016746479262,23.5148408966953));
#57795=CARTESIAN_POINT('Ctrl Pts',(52.7095844488888,28.1250339452557,23.5190627101217));
#57796=CARTESIAN_POINT('Ctrl Pts',(52.741122754398,28.0500400854238,23.5232845235481));
#57797=CARTESIAN_POINT('Ctrl Pts',(52.7726819768628,27.9749964878775,23.5275091369818));
#57798=CARTESIAN_POINT('Ctrl Pts',(52.8079531945684,27.9016023248674,23.5317337504154));
#57799=CARTESIAN_POINT('Ctrl Pts',(52.8467233334473,27.830235131627,23.5359583638491));
#57800=CARTESIAN_POINT('Ctrl Pts',(52.885563189113,27.7587396053051,23.5401905740178));
#57801=CARTESIAN_POINT('Ctrl Pts',(52.9279142852273,27.6892787211411,23.5444227841866));
#57802=CARTESIAN_POINT('Ctrl Pts',(52.9735199245037,27.6222014829386,23.5486549943553));
#57803=CARTESIAN_POINT('Ctrl Pts',(52.9992421148269,27.5843690237346,23.5510420174773));
#57804=CARTESIAN_POINT('Ctrl Pts',(53.0259988654998,27.5472942432224,23.5534290405994));
#57805=CARTESIAN_POINT('Ctrl Pts',(53.0537387209796,27.5110348278802,23.5558160637214));
#57806=CARTESIAN_POINT('Ctrl Pts',(53.1030160851922,27.4466232300167,23.5600563961144));
#57807=CARTESIAN_POINT('Ctrl Pts',(53.1555846095254,27.3845426287641,23.5642967285075));
#57808=CARTESIAN_POINT('Ctrl Pts',(53.2111960290357,27.3251475875581,23.5685370609005));
#57809=CARTESIAN_POINT('Ctrl Pts',(53.2667279960875,27.2658374044997,23.5727713350983));
#57810=CARTESIAN_POINT('Ctrl Pts',(53.325293909279,27.2092054952295,23.5770056092962));
#57811=CARTESIAN_POINT('Ctrl Pts',(53.3866041889151,27.1555748302592,23.581239883494));
#57812=CARTESIAN_POINT('Ctrl Pts',(53.4478429967745,27.10200668464,23.5854692216338));
#57813=CARTESIAN_POINT('Ctrl Pts',(53.5118194654066,27.0514331320413,23.5896985597736));
#57814=CARTESIAN_POINT('Ctrl Pts',(53.5782070003551,27.0041405570129,23.5939278979134));
#57815=CARTESIAN_POINT('Ctrl Pts',(53.644551936521,26.956878328135,23.5981545222206));
#57816=CARTESIAN_POINT('Ctrl Pts',(53.7133044916079,26.9128931648167,23.6023811465278));
#57817=CARTESIAN_POINT('Ctrl Pts',(53.784105685571,26.872430667137,23.606607770835));
#57818=CARTESIAN_POINT('Ctrl Pts',(53.8548828865358,26.8319818813254,23.6108329628303));
#57819=CARTESIAN_POINT('Ctrl Pts',(53.9277069460756,26.7950536195464,23.6150581548256));
#57820=CARTESIAN_POINT('Ctrl Pts',(54.0021918461236,26.7618469359631,23.619283346821));
#57821=CARTESIAN_POINT('Ctrl Pts',(54.0766740573049,26.728641451124,23.623508386289));
#57822=CARTESIAN_POINT('Ctrl Pts',(54.1528165667252,26.6991574647628,23.6277334257571));
#57823=CARTESIAN_POINT('Ctrl Pts',(54.2302121063722,26.6735484426225,23.6319584652252));
#57824=CARTESIAN_POINT('Ctrl Pts',(54.30768071855,26.6479152418789,23.6361874937387));
#57825=CARTESIAN_POINT('Ctrl Pts',(54.3864042842766,26.6261644605585,23.6404165222523));
#57826=CARTESIAN_POINT('Ctrl Pts',(54.4659595540915,26.608399897112,23.6446455507658));
#57827=CARTESIAN_POINT('Ctrl Pts',(54.5455503242964,26.5906274064857,23.6488764664222));
#57828=CARTESIAN_POINT('Ctrl Pts',(54.6259730814925,26.576844757245,23.6531073820787));
#57829=CARTESIAN_POINT('Ctrl Pts',(54.7067959688153,26.5671042673191,23.6573382977351));
#57830=CARTESIAN_POINT('Ctrl Pts',(54.7877612686191,26.5573466143422,23.6615766683986));
#57831=CARTESIAN_POINT('Ctrl Pts',(54.8691276446669,26.5516453877608,23.6658150390621));
#57832=CARTESIAN_POINT('Ctrl Pts',(54.950459840218,26.5500008117208,23.6700534097256));
#57833=CARTESIAN_POINT('Ctrl Pts',(55.0301952929976,26.5483885225862,23.6742085711793));
#57834=CARTESIAN_POINT('Ctrl Pts',(55.1098974842549,26.5506749356976,23.678363732633));
#57835=CARTESIAN_POINT('Ctrl Pts',(55.1891616966146,26.5568118978405,23.6825188940868));
#57836=CARTESIAN_POINT('Ctrl Pts',(55.2690802523531,26.5629995219457,23.6867083573055));
#57837=CARTESIAN_POINT('Ctrl Pts',(55.3488563077395,26.5731252336513,23.6908978205242));
#57838=CARTESIAN_POINT('Ctrl Pts',(55.4280656812847,26.5871779960995,23.695087283743));
#57839=CARTESIAN_POINT('Ctrl Pts',(55.5103202362572,26.6017710129305,23.6994378096619));
#57840=CARTESIAN_POINT('Ctrl Pts',(55.5919631422334,26.6205992052271,23.7037883355808));
#57841=CARTESIAN_POINT('Ctrl Pts',(55.6725214939679,26.6435906361264,23.7081388614997));
#57842=CARTESIAN_POINT('Ctrl Pts',(55.7498998283755,26.6656744870287,23.7123176516829));
#57843=CARTESIAN_POINT('Ctrl Pts',(55.8262771079175,26.6915989493626,23.7164964418661));
#57844=CARTESIAN_POINT('Ctrl Pts',(55.901243442004,26.7212480371386,23.7206752320493));
#57845=CARTESIAN_POINT('Ctrl Pts',(55.9761666697665,26.7508800764194,23.7248516193902));
#57846=CARTESIAN_POINT('Ctrl Pts',(56.0496801212606,26.7842323172225,23.729028006731));
#57847=CARTESIAN_POINT('Ctrl Pts',(56.1213906170083,26.8211394413396,23.7332043940718));
#57848=CARTESIAN_POINT('Ctrl Pts',(56.1930829059465,26.8580371949878,23.7373797210562));
#57849=CARTESIAN_POINT('Ctrl Pts',(56.2629727261088,26.8984878223256,23.7415550480406));
#57850=CARTESIAN_POINT('Ctrl Pts',(56.3306898170856,26.9422792073013,23.7457303750249));
#57851=CARTESIAN_POINT('Ctrl Pts',(56.3984114598277,26.986073535819,23.7499059826638));
#57852=CARTESIAN_POINT('Ctrl Pts',(56.4639596861817,27.033208807563,23.7540815903027));
#57853=CARTESIAN_POINT('Ctrl Pts',(56.526992974048,27.0834294411089,23.7582571979416));
#57854=CARTESIAN_POINT('Ctrl Pts',(56.5900869053925,27.1336983912507,23.7624368228764));
#57855=CARTESIAN_POINT('Ctrl Pts',(56.6506606990727,27.1870583289571,23.7666164478112));
#57856=CARTESIAN_POINT('Ctrl Pts',(56.708406379522,27.2432137601835,23.7707960727461));
#57857=CARTESIAN_POINT('Ctrl Pts',(56.7661851835194,27.2994014027738,23.774978095159));
#57858=CARTESIAN_POINT('Ctrl Pts',(56.8211323240713,27.3583873813232,23.779160117572));
#57859=CARTESIAN_POINT('Ctrl Pts',(56.8729788290211,27.4198416041299,23.783342139985));
#57860=CARTESIAN_POINT('Ctrl Pts',(56.924903432116,27.4813883975123,23.7875304619199));
#57861=CARTESIAN_POINT('Ctrl Pts',(56.9737177969051,27.5454104741242,23.7917187838548));
#57862=CARTESIAN_POINT('Ctrl Pts',(57.0191955923614,27.6115478366943,23.7959071057896));
#57863=CARTESIAN_POINT('Ctrl Pts',(57.0321994179502,27.6304590156364,23.7971047057921));
#57864=CARTESIAN_POINT('Ctrl Pts',(57.0449307307273,27.6495429851411,23.7983023057946));
#57865=CARTESIAN_POINT('Ctrl Pts',(57.0573849385052,27.6687909762881,23.799499905797));
#57866=CARTESIAN_POINT('',(55.2147522011135,26.5589281571169,23.7995));
#57867=CARTESIAN_POINT('Origin',(55.,29.,23.7995));
#57868=CARTESIAN_POINT('',(52.5498441316087,29.0016533468466,23.5883274660079));
#57869=CARTESIAN_POINT('Ctrl Pts',(55.2147522011135,26.5589281571169,23.7995));
#57870=CARTESIAN_POINT('Ctrl Pts',(54.4050310115761,26.4876932984426,23.7572657232115));
#57871=CARTESIAN_POINT('Ctrl Pts',(53.003287825418,27.0942572053241,23.6868748886155));
#57872=CARTESIAN_POINT('Ctrl Pts',(52.5563761394599,28.4582876769929,23.6164840540196));
#57873=CARTESIAN_POINT('Ctrl Pts',(52.5520032102007,29.0016513069589,23.5883274962121));
#57874=CARTESIAN_POINT('',(52.5495000174313,29.0002922856895,22.7883274962497));
#57875=CARTESIAN_POINT('Ctrl Pts',(52.5495005579738,29.0016536714534,23.5883274612015));
#57876=CARTESIAN_POINT('Ctrl Pts',(52.5495642388273,29.0960193905902,23.5834424895806));
#57877=CARTESIAN_POINT('Ctrl Pts',(52.5550827318315,29.1901514168606,23.5785575179597));
#57878=CARTESIAN_POINT('Ctrl Pts',(52.5659516932184,29.2834767896203,23.5736725463388));
#57879=CARTESIAN_POINT('Ctrl Pts',(52.5769354492301,29.3777878362438,23.5687359811511));
#57880=CARTESIAN_POINT('Ctrl Pts',(52.5933831868479,29.4712749581831,23.5637994159634));
#57881=CARTESIAN_POINT('Ctrl Pts',(52.6151379068873,29.5633675947673,23.5588628507757));
#57882=CARTESIAN_POINT('Ctrl Pts',(52.6338942271615,29.6427673288729,23.5546066802735));
#57883=CARTESIAN_POINT('Ctrl Pts',(52.6565946040389,29.7211307824724,23.5503505097713));
#57884=CARTESIAN_POINT('Ctrl Pts',(52.68311033603,29.7981055913782,23.5460943392691));
#57885=CARTESIAN_POINT('Ctrl Pts',(52.7095081791768,29.874738170574,23.5418570916849));
#57886=CARTESIAN_POINT('Ctrl Pts',(52.7397606807718,29.95020067919,23.5376198441007));
#57887=CARTESIAN_POINT('Ctrl Pts',(52.7737445873222,30.0240786529964,23.5333825965165));
#57888=CARTESIAN_POINT('Ctrl Pts',(52.8076799722184,30.0978511450657,23.5291513988037));
#57889=CARTESIAN_POINT('Ctrl Pts',(52.8453359879674,30.1700431784693,23.5249202010908));
#57890=CARTESIAN_POINT('Ctrl Pts',(52.886540194497,30.2402571912806,23.520689003378));
#57891=CARTESIAN_POINT('Ctrl Pts',(52.9276965756498,30.3103897072764,23.5164627167808));
#57892=CARTESIAN_POINT('Ctrl Pts',(52.9723927284683,30.3785483684405,23.5122364301837));
#57893=CARTESIAN_POINT('Ctrl Pts',(53.0204095276617,30.444358616074,23.5080101435865));
#57894=CARTESIAN_POINT('Ctrl Pts',(53.0683956795213,30.5101268594786,23.5037865544706));
#57895=CARTESIAN_POINT('Ctrl Pts',(53.1196979977247,30.5735492917698,23.4995629653547));
#57896=CARTESIAN_POINT('Ctrl Pts',(53.1740537421329,30.6342798148974,23.4953393762388));
#57897=CARTESIAN_POINT('Ctrl Pts',(53.2283913086446,30.694990028246,23.4911171995949));
#57898=CARTESIAN_POINT('Ctrl Pts',(53.2857799645017,30.7530097754057,23.486895022951));
#57899=CARTESIAN_POINT('Ctrl Pts',(53.3459172452173,30.8080266840759,23.482672846307));
#57900=CARTESIAN_POINT('Ctrl Pts',(53.4060526859771,30.8630419094528,23.4784507988445));
#57901=CARTESIAN_POINT('Ctrl Pts',(53.4689362417597,30.9150541670806,23.474228751382));
#57902=CARTESIAN_POINT('Ctrl Pts',(53.5342302610026,30.9637895310444,23.4700067039195));
#57903=CARTESIAN_POINT('Ctrl Pts',(53.5995868324059,31.0125715838526,23.4657806117038));
#57904=CARTESIAN_POINT('Ctrl Pts',(53.6673581086993,31.0580701932019,23.4615545194881));
#57905=CARTESIAN_POINT('Ctrl Pts',(53.7371755937771,31.1000535157581,23.4573284272724));
#57906=CARTESIAN_POINT('Ctrl Pts',(53.8070246807587,31.1420558414754,23.4531004221755));
#57907=CARTESIAN_POINT('Ctrl Pts',(53.8789214131283,31.1805394904803,23.4488724170785));
#57908=CARTESIAN_POINT('Ctrl Pts',(53.9524728912223,31.2153187595414,23.4446444119816));
#57909=CARTESIAN_POINT('Ctrl Pts',(54.0261553873424,31.2501599812824,23.4404088754944));
#57910=CARTESIAN_POINT('Ctrl Pts',(54.1014980905841,31.2812834579993,23.4361733390072));
#57911=CARTESIAN_POINT('Ctrl Pts',(54.1780884412599,31.3085518490191,23.4319378025201));
#57912=CARTESIAN_POINT('Ctrl Pts',(54.2537124722551,31.3354762021454,23.427755704648));
#57913=CARTESIAN_POINT('Ctrl Pts',(54.330552406019,31.358642164411,23.4235736067758));
#57914=CARTESIAN_POINT('Ctrl Pts',(54.4082007613574,31.3779663393627,23.4193915089037));
#57915=CARTESIAN_POINT('Ctrl Pts',(54.4869164102734,31.3975561293133,23.4151519271843));
#57916=CARTESIAN_POINT('Ctrl Pts',(54.5667466705475,31.4132683160261,23.4109123454649));
#57917=CARTESIAN_POINT('Ctrl Pts',(54.6472759233404,31.424981644414,23.4066727637455));
#57918=CARTESIAN_POINT('Ctrl Pts',(54.7276931921117,31.4366786842411,23.4024390775907));
#57919=CARTESIAN_POINT('Ctrl Pts',(54.8088070682774,31.4443878454646,23.3982053914359));
#57920=CARTESIAN_POINT('Ctrl Pts',(54.8901894976013,31.4480383786949,23.3939717052811));
#57921=CARTESIAN_POINT('Ctrl Pts',(54.9714818060851,31.4516848694172,23.389742707403));
#57922=CARTESIAN_POINT('Ctrl Pts',(55.0530416165865,31.4512816445403,23.385513709525));
#57923=CARTESIAN_POINT('Ctrl Pts',(55.1344348921067,31.4468096594922,23.3812847116469));
#57924=CARTESIAN_POINT('Ctrl Pts',(55.2157788324529,31.4423403850631,23.3770582771053));
#57925=CARTESIAN_POINT('Ctrl Pts',(55.2969559773223,31.4338072720591,23.3728318425636));
#57926=CARTESIAN_POINT('Ctrl Pts',(55.3775325749835,31.4212433592736,23.368605408022));
#57927=CARTESIAN_POINT('Ctrl Pts',(55.4580847301207,31.4086832576907,23.3643802555489));
#57928=CARTESIAN_POINT('Ctrl Pts',(55.5380362429751,31.3920948561298,23.3601551030759));
#57929=CARTESIAN_POINT('Ctrl Pts',(55.6169601720937,31.3715628593925,23.3559299506029));
#57930=CARTESIAN_POINT('Ctrl Pts',(55.695884056456,31.3510308742986,23.3517048005259));
#57931=CARTESIAN_POINT('Ctrl Pts',(55.7737799107425,31.3265554162657,23.3474796504489));
#57932=CARTESIAN_POINT('Ctrl Pts',(55.8502340217815,31.298271602358,23.3432545003718));
#57933=CARTESIAN_POINT('Ctrl Pts',(55.9267645865935,31.2699595047615,23.3390251251634));
#57934=CARTESIAN_POINT('Ctrl Pts',(56.0018500929309,31.237831604185,23.334795749955));
#57935=CARTESIAN_POINT('Ctrl Pts',(56.075095441174,31.2020717614026,23.3305663747466));
#57936=CARTESIAN_POINT('Ctrl Pts',(56.1483757047791,31.1662948722427,23.3263349834352));
#57937=CARTESIAN_POINT('Ctrl Pts',(56.2198136567177,31.1268828150247,23.3221035921238));
#57938=CARTESIAN_POINT('Ctrl Pts',(56.2890397269056,31.0840649779839,23.3178722008124));
#57939=CARTESIAN_POINT('Ctrl Pts',(56.3583912791156,31.0411695275706,23.3136331395071));
#57940=CARTESIAN_POINT('Ctrl Pts',(56.4255225550726,30.9948562234326,23.3093940782018));
#57941=CARTESIAN_POINT('Ctrl Pts',(56.4900939366215,30.9453972113797,23.3051550168964));
#57942=CARTESIAN_POINT('Ctrl Pts',(56.5533916522134,30.896913774859,23.300999570777));
#57943=CARTESIAN_POINT('Ctrl Pts',(56.6142292897565,30.8454079401431,23.2968441246576));
#57944=CARTESIAN_POINT('Ctrl Pts',(56.6723214501742,30.7911703484837,23.2926886785382));
#57945=CARTESIAN_POINT('Ctrl Pts',(56.7314235911169,30.7359897911831,23.2884609865319));
#57946=CARTESIAN_POINT('Ctrl Pts',(56.7879040576757,30.6777759052241,23.2842332945255));
#57947=CARTESIAN_POINT('Ctrl Pts',(56.8414349319838,30.6168078553959,23.2800056025192));
#57948=CARTESIAN_POINT('Ctrl Pts',(56.8948884835476,30.5559278709502,23.2757840172083));
#57949=CARTESIAN_POINT('Ctrl Pts',(56.9454005994851,30.4923019703519,23.2715624318975));
#57950=CARTESIAN_POINT('Ctrl Pts',(56.9926786911212,30.4262474834164,23.2673408465866));
#57951=CARTESIAN_POINT('Ctrl Pts',(57.0399740251992,30.3601689062392,23.2631177216527));
#57952=CARTESIAN_POINT('Ctrl Pts',(57.0840326507937,30.2916603080827,23.2588945967188));
#57953=CARTESIAN_POINT('Ctrl Pts',(57.1246007636182,30.2210740539512,23.2546714717848));
#57954=CARTESIAN_POINT('Ctrl Pts',(57.1650804025972,30.1506417393774,23.2504575569442));
#57955=CARTESIAN_POINT('Ctrl Pts',(57.2020844836243,30.0781412129691,23.2462436421036));
#57956=CARTESIAN_POINT('Ctrl Pts',(57.2354040962635,30.0039515807091,23.2420297272629));
#57957=CARTESIAN_POINT('Ctrl Pts',(57.2687125107127,29.9297868824005,23.2378172286518));
#57958=CARTESIAN_POINT('Ctrl Pts',(57.2983387250494,29.8539346300981,23.2336047300407));
#57959=CARTESIAN_POINT('Ctrl Pts',(57.3241207737503,29.7767965493117,23.2293922314296));
#57960=CARTESIAN_POINT('Ctrl Pts',(57.3499020921784,29.6996606534499,23.2251798521369));
#57961=CARTESIAN_POINT('Ctrl Pts',(57.3718393148471,29.6212394436475,23.2209674728442));
#57962=CARTESIAN_POINT('Ctrl Pts',(57.3898199049781,29.5419511710207,23.2167550935515));
#57963=CARTESIAN_POINT('Ctrl Pts',(57.4078789979708,29.4623167275363,23.2125243231032));
#57964=CARTESIAN_POINT('Ctrl Pts',(57.4219467125659,29.3818080914518,23.208293552655));
#57965=CARTESIAN_POINT('Ctrl Pts',(57.4319609652375,29.3008589595823,23.2040627822068));
#57966=CARTESIAN_POINT('Ctrl Pts',(57.4419460760183,29.2201453930455,23.1998443234761));
#57967=CARTESIAN_POINT('Ctrl Pts',(57.4479012922646,29.1389943615875,23.1956258647454));
#57968=CARTESIAN_POINT('Ctrl Pts',(57.4498173277825,29.0578386591885,23.1914074060148));
#57969=CARTESIAN_POINT('Ctrl Pts',(57.4517417513241,28.9763276732072,23.1871704797078));
#57970=CARTESIAN_POINT('Ctrl Pts',(57.4495915665513,28.8948124482751,23.1829335534008));
#57971=CARTESIAN_POINT('Ctrl Pts',(57.443410061242,28.8137272896495,23.1786966270938));
#57972=CARTESIAN_POINT('Ctrl Pts',(57.4372285559327,28.7326421310238,23.1744597007868));
#57973=CARTESIAN_POINT('Ctrl Pts',(57.4270158514712,28.6519874962646,23.1702227744797));
#57974=CARTESIAN_POINT('Ctrl Pts',(57.4128667311383,28.572186503525,23.1659858481727));
#57975=CARTESIAN_POINT('Ctrl Pts',(57.3987289132656,28.4924492566242,23.1617523063652));
#57976=CARTESIAN_POINT('Ctrl Pts',(57.3806080574253,28.4132657080739,23.1575187645578));
#57977=CARTESIAN_POINT('Ctrl Pts',(57.3585610360867,28.3350638458819,23.1532852227503));
#57978=CARTESIAN_POINT('Ctrl Pts',(57.3365454407038,28.2569734530904,23.1490577154585));
#57979=CARTESIAN_POINT('Ctrl Pts',(57.3106149200503,28.1798624106211,23.1448302081668));
#57980=CARTESIAN_POINT('Ctrl Pts',(57.2808775707241,28.1041497014747,23.140602700875));
#57981=CARTESIAN_POINT('Ctrl Pts',(57.2511744714117,28.0285241944964,23.1363800626179));
#57982=CARTESIAN_POINT('Ctrl Pts',(57.2176734265239,27.9542942498791,23.1321574243607));
#57983=CARTESIAN_POINT('Ctrl Pts',(57.1805322388255,27.8818634227239,23.1279347861036));
#57984=CARTESIAN_POINT('Ctrl Pts',(57.1434145361545,27.8094783948568,23.123714817895));
#57985=CARTESIAN_POINT('Ctrl Pts',(57.1026614712074,27.7388906381866,23.1194948496864));
#57986=CARTESIAN_POINT('Ctrl Pts',(57.0584783653688,27.6704823922533,23.1152748814779));
#57987=CARTESIAN_POINT('Ctrl Pts',(57.014309704517,27.6020965113436,23.111056292923));
#57988=CARTESIAN_POINT('Ctrl Pts',(56.9667134815588,27.5358891157875,23.1068377043681));
#57989=CARTESIAN_POINT('Ctrl Pts',(56.9159395072919,27.4722153115056,23.1026191158132));
#57990=CARTESIAN_POINT('Ctrl Pts',(56.8651666276668,27.4085428799743,23.0984006182073));
#57991=CARTESIAN_POINT('Ctrl Pts',(56.8112164233434,27.3474042934087,23.0941821206015));
#57992=CARTESIAN_POINT('Ctrl Pts',(56.7543794388078,27.289122145012,23.0899636229956));
#57993=CARTESIAN_POINT('Ctrl Pts',(56.69747662169,27.2307724901429,23.0857402392299));
#57994=CARTESIAN_POINT('Ctrl Pts',(56.6376806661255,27.1752862200568,23.0815168554642));
#57995=CARTESIAN_POINT('Ctrl Pts',(56.5753193042457,27.1229492975226,23.0772934716985));
#57996=CARTESIAN_POINT('Ctrl Pts',(56.5129402173685,27.0705974992418,23.0730688875186));
#57997=CARTESIAN_POINT('Ctrl Pts',(56.4479946467122,27.0213971071168,23.0688443033387));
#57998=CARTESIAN_POINT('Ctrl Pts',(56.3808414053864,26.9755921203546,23.0646197191588));
#57999=CARTESIAN_POINT('Ctrl Pts',(56.3135666438222,26.9297042450705,23.0603874901881));
#58000=CARTESIAN_POINT('Ctrl Pts',(56.2440766249951,26.8872242972987,23.0561552612175));
#58001=CARTESIAN_POINT('Ctrl Pts',(56.1727570784822,26.8483515424517,23.0519230322469));
#58002=CARTESIAN_POINT('Ctrl Pts',(56.1017558713171,26.8096522986271,23.0477096941003));
#58003=CARTESIAN_POINT('Ctrl Pts',(56.0289418817796,26.7745282251677,23.0434963559538));
#58004=CARTESIAN_POINT('Ctrl Pts',(55.9547139357488,26.7431279276647,23.0392830178073));
#58005=CARTESIAN_POINT('Ctrl Pts',(55.8801328412964,26.7115782394525,23.0350496341955));
#58006=CARTESIAN_POINT('Ctrl Pts',(55.8038480783036,26.6836710384964,23.0308162505837));
#58007=CARTESIAN_POINT('Ctrl Pts',(55.726249631041,26.6595915477394,23.0265828669719));
#58008=CARTESIAN_POINT('Ctrl Pts',(55.6487615440981,26.6355463027746,23.0223555040678));
#58009=CARTESIAN_POINT('Ctrl Pts',(55.569963923485,26.6153180923391,23.0181281411637));
#58010=CARTESIAN_POINT('Ctrl Pts',(55.4902670770494,26.5990442646393,23.0139007782596));
#58011=CARTESIAN_POINT('Ctrl Pts',(55.4106616146491,26.5827890972519,23.0096782626424));
#58012=CARTESIAN_POINT('Ctrl Pts',(55.3301594283528,26.5704793932409,23.0054557470252));
#58013=CARTESIAN_POINT('Ctrl Pts',(55.2491849369823,26.5622024043861,23.001233231408));
#58014=CARTESIAN_POINT('Ctrl Pts',(55.1682613941383,26.5539306233488,22.9970133725651));
#58015=CARTESIAN_POINT('Ctrl Pts',(55.0868665968571,26.5496865675813,22.9927935137223));
#58016=CARTESIAN_POINT('Ctrl Pts',(55.0054329419913,26.549506022627,22.9885736548794));
#58017=CARTESIAN_POINT('Ctrl Pts',(54.9240256515744,26.5493255361249,22.9843551622315));
#58018=CARTESIAN_POINT('Ctrl Pts',(54.8425799925547,26.5532059487735,22.9801366695836));
#58019=CARTESIAN_POINT('Ctrl Pts',(54.7615298097258,26.5611309550633,22.9759181769358));
#58020=CARTESIAN_POINT('Ctrl Pts',(54.6804811119383,26.5690558161471,22.9716997615812));
#58021=CARTESIAN_POINT('Ctrl Pts',(54.5998283379637,26.5810250771506,22.9674813462267));
#58022=CARTESIAN_POINT('Ctrl Pts',(54.5200002233569,26.5969705652193,22.9632629308721));
#58023=CARTESIAN_POINT('Ctrl Pts',(54.440074715967,26.6129355072795,22.9590393689196));
#58024=CARTESIAN_POINT('Ctrl Pts',(54.3609763361036,26.6328862828714,22.954815806967));
#58025=CARTESIAN_POINT('Ctrl Pts',(54.2831233980475,26.6567035638714,22.9505922450145));
#58026=CARTESIAN_POINT('Ctrl Pts',(54.2052524953077,26.6805263407452,22.9463677084687));
#58027=CARTESIAN_POINT('Ctrl Pts',(54.1286280413679,26.708217233255,22.9421431719228));
#58028=CARTESIAN_POINT('Ctrl Pts',(54.0536499864002,26.7396080203293,22.9379186353769));
#58029=CARTESIAN_POINT('Ctrl Pts',(53.9785358691495,26.7710557721003,22.9336864325868));
#58030=CARTESIAN_POINT('Ctrl Pts',(53.9050745417714,26.8062166354433,22.9294542297966));
#58031=CARTESIAN_POINT('Ctrl Pts',(53.83364307309,26.8448754632159,22.9252220270064));
#58032=CARTESIAN_POINT('Ctrl Pts',(53.7625197352201,26.8833675300888,22.9210080804849));
#58033=CARTESIAN_POINT('Ctrl Pts',(53.6934091171587,26.9253271307111,22.9167941339634));
#58034=CARTESIAN_POINT('Ctrl Pts',(53.6266530602894,26.970500447601,22.9125801874418));
#58035=CARTESIAN_POINT('Ctrl Pts',(53.559831201844,27.015718291918,22.9083620872249));
#58036=CARTESIAN_POINT('Ctrl Pts',(53.4951162351161,27.0643270129538,22.904143987008));
#58037=CARTESIAN_POINT('Ctrl Pts',(53.4328743933687,27.1161030858775,22.8999258867911));
#58038=CARTESIAN_POINT('Ctrl Pts',(53.3707216263246,27.1678050617274,22.8957138231248));
#58039=CARTESIAN_POINT('Ctrl Pts',(53.3110353128802,27.2226650915625,22.8915017594585));
#58040=CARTESIAN_POINT('Ctrl Pts',(53.2541527620657,27.2804164248874,22.8872896957922));
#58041=CARTESIAN_POINT('Ctrl Pts',(53.1973355303895,27.338101441437,22.8830824689056));
#58042=CARTESIAN_POINT('Ctrl Pts',(53.1433159903921,27.3986708321606,22.878875242019));
#58043=CARTESIAN_POINT('Ctrl Pts',(53.0923972278155,27.4618186343756,22.8746680151324));
#58044=CARTESIAN_POINT('Ctrl Pts',(53.0415102841336,27.5249269758267,22.8704634173221));
#58045=CARTESIAN_POINT('Ctrl Pts',(52.9937205652041,27.5906101674105,22.8662588195117));
#58046=CARTESIAN_POINT('Ctrl Pts',(52.9492923969959,27.6585274594755,22.8620542217014));
#58047=CARTESIAN_POINT('Ctrl Pts',(52.9048781562321,27.7264234606716,22.8578509419581));
#58048=CARTESIAN_POINT('Ctrl Pts',(52.863823629782,27.7965517801551,22.8536476622147));
#58049=CARTESIAN_POINT('Ctrl Pts',(52.8263502659314,27.8685420539925,22.8494443824714));
#58050=CARTESIAN_POINT('Ctrl Pts',(52.7888769797546,27.9405321786104,22.8452411114405));
#58051=CARTESIAN_POINT('Ctrl Pts',(52.7549850561409,28.0143838338902,22.8410378404096));
#58052=CARTESIAN_POINT('Ctrl Pts',(52.7248496557592,28.0897027072979,22.8368345693787));
#58053=CARTESIAN_POINT('Ctrl Pts',(52.6946846212127,28.1650956468162,22.8326271649889));
#58054=CARTESIAN_POINT('Ctrl Pts',(52.6682836619809,28.2419582504506,22.8284197605991));
#58055=CARTESIAN_POINT('Ctrl Pts',(52.6457732464847,28.3198774793959,22.8242123562093));
#58056=CARTESIAN_POINT('Ctrl Pts',(52.6232517664169,28.3978350080738,22.8200028837489));
#58057=CARTESIAN_POINT('Ctrl Pts',(52.6046247459021,28.4768497402581,22.8157934112885));
#58058=CARTESIAN_POINT('Ctrl Pts',(52.5899677282388,28.5564972389382,22.8115839388282));
#58059=CARTESIAN_POINT('Ctrl Pts',(52.5752850185252,28.6362843504363,22.8073670876513));
#58060=CARTESIAN_POINT('Ctrl Pts',(52.564586274865,28.716705979306,22.8031502364744));
#58061=CARTESIAN_POINT('Ctrl Pts',(52.5578952153805,28.7973316232398,22.7989333852976));
#58062=CARTESIAN_POINT('Ctrl Pts',(52.552285608312,28.8649260278568,22.7953980889483));
#58063=CARTESIAN_POINT('Ctrl Pts',(52.5494919509591,28.9326636235578,22.791862792599));
#58064=CARTESIAN_POINT('Ctrl Pts',(52.5495000174313,29.0002922856895,22.7883274962497));
#58065=CARTESIAN_POINT('',(52.5495008948029,28.9979058586013,21.9883275169164));
#58066=CARTESIAN_POINT('Ctrl Pts',(52.5495000174314,29.0002922864085,22.7883274962121));
#58067=CARTESIAN_POINT('Ctrl Pts',(52.5495018809271,29.015915647263,22.7875107831668));
#58068=CARTESIAN_POINT('Ctrl Pts',(52.5496531545866,29.0315379897785,22.7866940701216));
#58069=CARTESIAN_POINT('Ctrl Pts',(52.54995379109,29.0471574406191,22.7858773570764));
#58070=CARTESIAN_POINT('Ctrl Pts',(52.551511902383,29.1281084976825,22.7816445716218));
#58071=CARTESIAN_POINT('Ctrl Pts',(52.5570892279648,29.2091326985126,22.7774117861671));
#58072=CARTESIAN_POINT('Ctrl Pts',(52.566696269008,29.2897985554489,22.7731790007125));
#58073=CARTESIAN_POINT('Ctrl Pts',(52.5762896098424,29.3703493781018,22.7689522514603));
#58074=CARTESIAN_POINT('Ctrl Pts',(52.589901198119,29.4505424143979,22.7647255022081));
#58075=CARTESIAN_POINT('Ctrl Pts',(52.6074895335361,29.5299470896805,22.7604987529559));
#58076=CARTESIAN_POINT('Ctrl Pts',(52.6250576127034,29.6092603156642,22.7562768715941));
#58077=CARTESIAN_POINT('Ctrl Pts',(52.6465932365051,29.6877865339608,22.7520549902323));
#58078=CARTESIAN_POINT('Ctrl Pts',(52.6720034019218,29.7651026658798,22.7478331088705));
#58079=CARTESIAN_POINT('Ctrl Pts',(52.6973975034608,29.8423699198451,22.7436138965108));
#58080=CARTESIAN_POINT('Ctrl Pts',(52.726661139605,29.9184281659353,22.7393946841512));
#58081=CARTESIAN_POINT('Ctrl Pts',(52.7596510489301,29.9928679808715,22.7351754717915));
#58082=CARTESIAN_POINT('Ctrl Pts',(52.7926301873071,30.0672834917891,22.7309576369717));
#58083=CARTESIAN_POINT('Ctrl Pts',(52.8293329947074,30.1400811965917,22.726739802152));
#58084=CARTESIAN_POINT('Ctrl Pts',(52.8695680384666,30.2108715486281,22.7225219673322));
#58085=CARTESIAN_POINT('Ctrl Pts',(52.9098022449982,30.2816604276293,22.7183042202789));
#58086=CARTESIAN_POINT('Ctrl Pts',(52.9535683112031,30.3504416336603,22.7140864732257));
#58087=CARTESIAN_POINT('Ctrl Pts',(53.000629506976,30.4168513971568,22.7098687261724));
#58088=CARTESIAN_POINT('Ctrl Pts',(53.0477662369107,30.4833677496537,22.7056442095506));
#58089=CARTESIAN_POINT('Ctrl Pts',(53.0982084066648,30.5475046644456,22.7014196929288));
#58090=CARTESIAN_POINT('Ctrl Pts',(53.151676470778,30.6089283331847,22.697195176307));
#58091=CARTESIAN_POINT('Ctrl Pts',(53.2051360931266,30.6703423040945,22.6929713266698));
#58092=CARTESIAN_POINT('Ctrl Pts',(53.2616203165558,30.7290435639711,22.6887474770326));
#58093=CARTESIAN_POINT('Ctrl Pts',(53.3208127308396,30.7847353767687,22.6845236273954));
#58094=CARTESIAN_POINT('Ctrl Pts',(53.3801125017213,30.8405281971637,22.6802921170109));
#58095=CARTESIAN_POINT('Ctrl Pts',(53.4421299247691,30.8933003605444,22.6760606066264));
#58096=CARTESIAN_POINT('Ctrl Pts',(53.5065150453206,30.9427951359179,22.671829096242));
#58097=CARTESIAN_POINT('Ctrl Pts',(53.5706974853756,30.992134104708,22.6676109063983));
#58098=CARTESIAN_POINT('Ctrl Pts',(53.6372323159481,31.0382161003672,22.6633927165546));
#58099=CARTESIAN_POINT('Ctrl Pts',(53.7057472873696,31.0808316043949,22.6591745267109));
#58100=CARTESIAN_POINT('Ctrl Pts',(53.7744978327295,31.1235936326335,22.6549418335321));
#58101=CARTESIAN_POINT('Ctrl Pts',(53.8454977274284,31.1630242160109,22.6507091403532));
#58102=CARTESIAN_POINT('Ctrl Pts',(53.9183907616251,31.1988796477893,22.6464764471744));
#58103=CARTESIAN_POINT('Ctrl Pts',(53.9911798559339,31.2346839524663,22.642249789492));
#58104=CARTESIAN_POINT('Ctrl Pts',(54.065856314865,31.2669230272973,22.6380231318097));
#58105=CARTESIAN_POINT('Ctrl Pts',(54.1420363842115,31.2953972823856,22.6337964741274));
#58106=CARTESIAN_POINT('Ctrl Pts',(54.2181300849763,31.3238392550009,22.6295746083865));
#58107=CARTESIAN_POINT('Ctrl Pts',(54.2957235755163,31.3485247284311,22.6253527426456));
#58108=CARTESIAN_POINT('Ctrl Pts',(54.3744113291554,31.3693013875214,22.6211308769047));
#58109=CARTESIAN_POINT('Ctrl Pts',(54.4530479677455,31.3900645502302,22.6169117536601));
#58110=CARTESIAN_POINT('Ctrl Pts',(54.532777010114,31.4069238218743,22.6126926304155));
#58111=CARTESIAN_POINT('Ctrl Pts',(54.6131770446963,31.4197764878703,22.6084735071709));
#58112=CARTESIAN_POINT('Ctrl Pts',(54.6935508500271,31.4326249608855,22.6042557603491));
#58113=CARTESIAN_POINT('Ctrl Pts',(54.7745947544948,31.4414693507897,22.6000380135274));
#58114=CARTESIAN_POINT('Ctrl Pts',(54.8558777954438,31.4462581711982,22.5958202667056));
#58115=CARTESIAN_POINT('Ctrl Pts',(54.9371591689845,31.4510468933707,22.5916026064051));
#58116=CARTESIAN_POINT('Ctrl Pts',(55.0186792054603,31.4517801853135,22.5873849461045));
#58117=CARTESIAN_POINT('Ctrl Pts',(55.1000039053973,31.4484585904004,22.583167285804));
#58118=CARTESIAN_POINT('Ctrl Pts',(55.1814630420402,31.4451315046058,22.5789426533491));
#58119=CARTESIAN_POINT('Ctrl Pts',(55.2627257296209,31.4377361405835,22.5747180208942));
#58120=CARTESIAN_POINT('Ctrl Pts',(55.34335973163,31.4263252759461,22.5704933884393));
#58121=CARTESIAN_POINT('Ctrl Pts',(55.4239772125173,31.4149167492838,22.5662696215705));
#58122=CARTESIAN_POINT('Ctrl Pts',(55.5039658117012,31.3994944760461,22.5620458547017));
#58123=CARTESIAN_POINT('Ctrl Pts',(55.582904383817,31.3801623325578,22.5578220878329));
#58124=CARTESIAN_POINT('Ctrl Pts',(55.6619861864785,31.3607951117506,22.553590657126));
#58125=CARTESIAN_POINT('Ctrl Pts',(55.7400137081264,31.3375039762578,22.5493592264192));
#58126=CARTESIAN_POINT('Ctrl Pts',(55.8165811004963,31.3104427186823,22.5451277957123));
#58127=CARTESIAN_POINT('Ctrl Pts',(55.8929181279475,31.2834628791128,22.5409090959234));
#58128=CARTESIAN_POINT('Ctrl Pts',(55.9678034109459,31.25273582221,22.5366903961344));
#58129=CARTESIAN_POINT('Ctrl Pts',(56.0408584123792,31.2184598295618,22.5324716963455));
#58130=CARTESIAN_POINT('Ctrl Pts',(56.1141528359076,31.1840715047009,22.5282391706731));
#58131=CARTESIAN_POINT('Ctrl Pts',(56.1858775852503,31.1459830025043,22.5240066450006));
#58132=CARTESIAN_POINT('Ctrl Pts',(56.2556343272889,31.1043603983476,22.5197741193282));
#58133=CARTESIAN_POINT('Ctrl Pts',(56.3252915428871,31.0627971798432,22.5155476324729));
#58134=CARTESIAN_POINT('Ctrl Pts',(56.392985932358,31.0177101101498,22.5113211456177));
#58135=CARTESIAN_POINT('Ctrl Pts',(56.458341168815,30.9693123889671,22.5070946587624));
#58136=CARTESIAN_POINT('Ctrl Pts',(56.5236256017779,30.9209671001212,22.5028727507298));
#58137=CARTESIAN_POINT('Ctrl Pts',(56.5865755447787,30.8693185603639,22.4986508426972));
#58138=CARTESIAN_POINT('Ctrl Pts',(56.6468424163714,30.8146240121965,22.4944289346646));
#58139=CARTESIAN_POINT('Ctrl Pts',(56.707066999848,30.7599678421519,22.4902099890645));
#58140=CARTESIAN_POINT('Ctrl Pts',(56.7646119089447,30.7022702212389,22.4859910434643));
#58141=CARTESIAN_POINT('Ctrl Pts',(56.8191615721865,30.6418286829873,22.4817720978642));
#58142=CARTESIAN_POINT('Ctrl Pts',(56.873693410549,30.5814068948692,22.4775545308646));
#58143=CARTESIAN_POINT('Ctrl Pts',(56.9252316357471,30.5182433146465,22.473336963865));
#58144=CARTESIAN_POINT('Ctrl Pts',(56.9734984458387,30.4526713786236,22.4691193968655));
#58145=CARTESIAN_POINT('Ctrl Pts',(57.0217642435996,30.3871008178829,22.4649019183236));
#58146=CARTESIAN_POINT('Ctrl Pts',(57.0667584882196,30.319122376608,22.4606844397818));
#58147=CARTESIAN_POINT('Ctrl Pts',(57.1082453667274,30.2491003657322,22.45646696124));
#58148=CARTESIAN_POINT('Ctrl Pts',(57.1498046716092,30.1789561128242,22.4522421199683));
#58149=CARTESIAN_POINT('Ctrl Pts',(57.1878441206886,30.1067615537844,22.4480172786966));
#58150=CARTESIAN_POINT('Ctrl Pts',(57.2221726240576,30.0329080689436,22.443792437425));
#58151=CARTESIAN_POINT('Ctrl Pts',(57.2564908969921,29.9590765936043,22.4395688552225));
#58152=CARTESIAN_POINT('Ctrl Pts',(57.2871002806282,29.883587621269,22.4353452730201));
#58153=CARTESIAN_POINT('Ctrl Pts',(57.3138586410326,29.8068509399628,22.4311216908177));
#58154=CARTESIAN_POINT('Ctrl Pts',(57.3406655535197,29.7299750227078,22.4268904450772));
#58155=CARTESIAN_POINT('Ctrl Pts',(57.3636073471398,29.6518473191553,22.4226591993367));
#58156=CARTESIAN_POINT('Ctrl Pts',(57.3825920866213,29.5728919608175,22.4184279535963));
#58157=CARTESIAN_POINT('Ctrl Pts',(57.4015250041914,29.4941521238776,22.4142082577242));
#58158=CARTESIAN_POINT('Ctrl Pts',(57.4165224394577,29.4145896078156,22.4099885618521));
#58159=CARTESIAN_POINT('Ctrl Pts',(57.4275446176907,29.3346302125048,22.40576886598));
#58160=CARTESIAN_POINT('Ctrl Pts',(57.4386006142479,29.2544254852183,22.4015362232076));
#58161=CARTESIAN_POINT('Ctrl Pts',(57.4456980206086,29.1735231071443,22.3973035804351));
#58162=CARTESIAN_POINT('Ctrl Pts',(57.4487593107478,29.0923476476475,22.3930709376626));
#58163=CARTESIAN_POINT('Ctrl Pts',(57.451816234469,29.0112879713552,22.3888443320466));
#58164=CARTESIAN_POINT('Ctrl Pts',(57.450848458447,28.9299564476022,22.3846177264305));
#58165=CARTESIAN_POINT('Ctrl Pts',(57.4458299664352,28.8487848377715,22.3803911208145));
#58166=CARTESIAN_POINT('Ctrl Pts',(57.4408170871408,28.7677040108521,22.3761692422645));
#58167=CARTESIAN_POINT('Ctrl Pts',(57.4317625226274,28.6867832037761,22.3719473637145));
#58168=CARTESIAN_POINT('Ctrl Pts',(57.4186923018831,28.6064548325652,22.3677254851645));
#58169=CARTESIAN_POINT('Ctrl Pts',(57.4056307836308,28.5261799460671,22.3635064176507));
#58170=CARTESIAN_POINT('Ctrl Pts',(57.3885589933099,28.4464971693967,22.359287350137));
#58171=CARTESIAN_POINT('Ctrl Pts',(57.3675547293458,28.3678332074902,22.3550682826232));
#58172=CARTESIAN_POINT('Ctrl Pts',(57.3465573240663,28.2891949323345,22.3508505927941));
#58173=CARTESIAN_POINT('Ctrl Pts',(57.3216301150387,28.2115752597305,22.3466329029651));
#58174=CARTESIAN_POINT('Ctrl Pts',(57.292901578214,28.1353887563629,22.342415213136));
#58175=CARTESIAN_POINT('Ctrl Pts',(57.2641736388151,28.0592038373356,22.3381976110161));
#58176=CARTESIAN_POINT('Ctrl Pts',(57.2316446937954,27.9844524625377,22.3339800088962));
#58177=CARTESIAN_POINT('Ctrl Pts',(57.1954919758804,27.9115307841539,22.3297624067764));
#58178=CARTESIAN_POINT('Ctrl Pts',(57.1592784364919,27.8384864260882,22.3255377091795));
#58179=CARTESIAN_POINT('Ctrl Pts',(57.1194291343123,27.7672783414038,22.3213130115827));
#58180=CARTESIAN_POINT('Ctrl Pts',(57.07616831138,27.6982798331357,22.3170883139859));
#58181=CARTESIAN_POINT('Ctrl Pts',(57.0329176387413,27.6292975139981,22.3128646076306));
#58182=CARTESIAN_POINT('Ctrl Pts',(56.9862573303634,27.5625241045296,22.3086409012752));
#58183=CARTESIAN_POINT('Ctrl Pts',(56.9364537618731,27.498301935099,22.3044171949198));
#58184=CARTESIAN_POINT('Ctrl Pts',(56.8865598367488,27.4339632499399,22.300185825662));
#58185=CARTESIAN_POINT('Ctrl Pts',(56.8335115583894,27.3721854084049,22.2959544564041));
#58186=CARTESIAN_POINT('Ctrl Pts',(56.777614662308,27.3132764416338,22.2917230871462));
#58187=CARTESIAN_POINT('Ctrl Pts',(56.7218809386956,27.2545394400742,22.287504069969));
#58188=CARTESIAN_POINT('Ctrl Pts',(56.663315592898,27.1986548403543,22.2832850527918));
#58189=CARTESIAN_POINT('Ctrl Pts',(56.6022539625235,27.1458876815096,22.2790660356146));
#58190=CARTESIAN_POINT('Ctrl Pts',(56.5409954399236,27.0929503758269,22.2748334142857));
#58191=CARTESIAN_POINT('Ctrl Pts',(56.4769966705314,27.042953795681,22.2706007929569));
#58192=CARTESIAN_POINT('Ctrl Pts',(56.4105715839815,26.9961941070892,22.266368171628));
#58193=CARTESIAN_POINT('Ctrl Pts',(56.3442412430922,26.9495011143471,22.2621415875138));
#58194=CARTESIAN_POINT('Ctrl Pts',(56.2754918353231,26.9060361084803,22.2579150033995));
#58195=CARTESIAN_POINT('Ctrl Pts',(56.2046713653864,26.8660559633819,22.2536884192853));
#58196=CARTESIAN_POINT('Ctrl Pts',(56.1339296517423,26.8261202784234,22.2494665353671));
#58197=CARTESIAN_POINT('Ctrl Pts',(56.0611218548132,26.7896619810227,22.2452446514489));
#58198=CARTESIAN_POINT('Ctrl Pts',(55.98662486943,26.7568946487019,22.2410227675307));
#58199=CARTESIAN_POINT('Ctrl Pts',(55.912177959732,26.7241493420591,22.2368037214956));
#58200=CARTESIAN_POINT('Ctrl Pts',(55.8360445407491,26.6950902596719,22.2325846754605));
#58201=CARTESIAN_POINT('Ctrl Pts',(55.7586248930801,26.6698844402907,22.2283656294253));
#58202=CARTESIAN_POINT('Ctrl Pts',(55.6812305249085,26.6446868512551,22.2241479610167));
#58203=CARTESIAN_POINT('Ctrl Pts',(55.602551203505,26.6233401702427,22.2199302926081));
#58204=CARTESIAN_POINT('Ctrl Pts',(55.5230046165781,26.6059623183755,22.2157126241996));
#58205=CARTESIAN_POINT('Ctrl Pts',(55.443459682209,26.5885848275282,22.2114950434119));
#58206=CARTESIAN_POINT('Ctrl Pts',(55.3630479722324,26.5751760998911,22.2072774626241));
#58207=CARTESIAN_POINT('Ctrl Pts',(55.2821982710643,26.565803133309,22.2030598818364));
#58208=CARTESIAN_POINT('Ctrl Pts',(55.201211654988,26.5564142940788,22.1988351587875));
#58209=CARTESIAN_POINT('Ctrl Pts',(55.119786027606,26.5510749435566,22.1946104357385));
#58210=CARTESIAN_POINT('Ctrl Pts',(55.0383566131692,26.5498002081001,22.1903857126896));
#58211=CARTESIAN_POINT('Ctrl Pts',(54.9569471977203,26.5485257857175,22.1861620272287));
#58212=CARTESIAN_POINT('Ctrl Pts',(54.8755344622266,26.5513139449561,22.1819383417678));
#58213=CARTESIAN_POINT('Ctrl Pts',(54.7945505732901,26.5581276071292,22.1777146563068));
#58214=CARTESIAN_POINT('Ctrl Pts',(54.7134197495079,26.5649536318155,22.1734833075122));
#58215=CARTESIAN_POINT('Ctrl Pts',(54.632719788992,26.5758196935741,22.1692519587175));
#58216=CARTESIAN_POINT('Ctrl Pts',(54.5528755146421,26.5906370251468,22.1650206099228));
#58217=CARTESIAN_POINT('Ctrl Pts',(54.4732617129635,26.6054115860886,22.1608014750316));
#58218=CARTESIAN_POINT('Ctrl Pts',(54.3944990878205,26.6241144503633,22.1565823401403));
#58219=CARTESIAN_POINT('Ctrl Pts',(54.3169925537467,26.6466086006865,22.1523632052491));
#58220=CARTESIAN_POINT('Ctrl Pts',(54.239238611905,26.6691745543434,22.1481306025031));
#58221=CARTESIAN_POINT('Ctrl Pts',(54.1624596057763,26.6956399943221,22.1438979997571));
#58222=CARTESIAN_POINT('Ctrl Pts',(54.0870748679564,26.7259028267721,22.1396653970111));
#58223=CARTESIAN_POINT('Ctrl Pts',(54.011797663029,26.7561224906709,22.13543883188));
#58224=CARTESIAN_POINT('Ctrl Pts',(53.9379112038061,26.7901286169372,22.1312122667489));
#58225=CARTESIAN_POINT('Ctrl Pts',(53.8658204147616,26.8277691378612,22.1269857016178));
#58226=CARTESIAN_POINT('Ctrl Pts',(53.7938093911539,26.8653680111262,22.1227638130039));
#58227=CARTESIAN_POINT('Ctrl Pts',(53.7235904996973,26.9065930749595,22.1185419243899));
#58228=CARTESIAN_POINT('Ctrl Pts',(53.6555480816002,26.9512444535496,22.114320035776));
#58229=CARTESIAN_POINT('Ctrl Pts',(53.5875517955472,26.9958655589746,22.1101010095582));
#58230=CARTESIAN_POINT('Ctrl Pts',(53.5217294394126,27.0439081110724,22.1058819833403));
#58231=CARTESIAN_POINT('Ctrl Pts',(53.4584390414731,27.0951272847916,22.1016629571225));
#58232=CARTESIAN_POINT('Ctrl Pts',(53.3951693136296,27.146329730772,22.0974453088021));
#58233=CARTESIAN_POINT('Ctrl Pts',(53.3344302626156,27.2007064460319,22.0932276604817));
#58234=CARTESIAN_POINT('Ctrl Pts',(53.2765481923684,27.2579712640799,22.0890100121613));
#58235=CARTESIAN_POINT('Ctrl Pts',(53.2186673279599,27.3152348891483,22.0847924517058));
#58236=CARTESIAN_POINT('Ctrl Pts',(53.1636436553973,27.3753861698215,22.0805748912503));
#58237=CARTESIAN_POINT('Ctrl Pts',(53.111766804186,27.4381019085018,22.0763573307949));
#58238=CARTESIAN_POINT('Ctrl Pts',(53.0598015653069,27.5009245021229,22.0721325844689));
#58239=CARTESIAN_POINT('Ctrl Pts',(53.0109941727395,27.5663199359595,22.067907838143));
#58240=CARTESIAN_POINT('Ctrl Pts',(52.965594258439,27.6339313601785,22.0636830918171));
#58241=CARTESIAN_POINT('Ctrl Pts',(52.9202059671091,27.7015254749906,22.0594594270813));
#58242=CARTESIAN_POINT('Ctrl Pts',(52.8782236315398,27.7713340352223,22.0552357623456));
#58243=CARTESIAN_POINT('Ctrl Pts',(52.8398514202671,27.8429743462318,22.0510120976099));
#58244=CARTESIAN_POINT('Ctrl Pts',(52.8014095878862,27.9147446387481,22.0467807696144));
#58245=CARTESIAN_POINT('Ctrl Pts',(52.7665911691204,27.988352902704,22.042549441619));
#58246=CARTESIAN_POINT('Ctrl Pts',(52.7355529769454,28.0633944641531,22.0383181136236));
#58247=CARTESIAN_POINT('Ctrl Pts',(52.7046034083988,28.1382217587587,22.034098867377));
#58248=CARTESIAN_POINT('Ctrl Pts',(52.6774125823483,28.2144737199589,22.0298796211303));
#58249=CARTESIAN_POINT('Ctrl Pts',(52.654086009428,28.2917360669646,22.0256603748837));
#58250=CARTESIAN_POINT('Ctrl Pts',(52.6254336649508,28.3866384510008,22.02047781775));
#58251=CARTESIAN_POINT('Ctrl Pts',(52.6025235371786,28.4833492873121,22.0152952606162));
#58252=CARTESIAN_POINT('Ctrl Pts',(52.5855453264011,28.5812412638087,22.0101127034825));
#58253=CARTESIAN_POINT('Ctrl Pts',(52.5688012110521,28.6777835065506,22.0050016034033));
#58254=CARTESIAN_POINT('Ctrl Pts',(52.5578265961228,28.7754745670536,21.9998905033241));
#58255=CARTESIAN_POINT('Ctrl Pts',(52.5527573617204,28.8736919662633,21.9947794032449));
#58256=CARTESIAN_POINT('Ctrl Pts',(52.5506243490207,28.9150195008028,21.9926287744687));
#58257=CARTESIAN_POINT('Ctrl Pts',(52.5495363306197,28.9564399683349,21.9904781456926));
#58258=CARTESIAN_POINT('Ctrl Pts',(52.5495008948029,28.9979058586013,21.9883275169164));
#58259=CARTESIAN_POINT('',(52.5526951386847,29.0013429706744,21.1883274962121));
#58260=CARTESIAN_POINT('Ctrl Pts',(52.5509293928096,28.9979074783278,21.9883274962121));
#58261=CARTESIAN_POINT('Ctrl Pts',(52.555637109855,29.5719524683613,21.9585375123141));
#58262=CARTESIAN_POINT('Ctrl Pts',(53.0429452071781,30.9670398873744,21.8865132516278));
#58263=CARTESIAN_POINT('Ctrl Pts',(55.3643553567281,31.8709715157123,21.7722547141527));
#58264=CARTESIAN_POINT('Ctrl Pts',(57.6065987423142,30.257328552056,21.6455518837873));
#58265=CARTESIAN_POINT('Ctrl Pts',(57.4737133360388,27.498009992113,21.5188490534219));
#58266=CARTESIAN_POINT('Ctrl Pts',(55.0867844397265,26.1073022273406,21.3921462230564));
#58267=CARTESIAN_POINT('Ctrl Pts',(52.9424797866962,27.1899851156092,21.2819723706532));
#58268=CARTESIAN_POINT('Ctrl Pts',(52.5551788087165,28.5051077036468,21.2140327950384));
#58269=CARTESIAN_POINT('Ctrl Pts',(52.5526951386847,29.0013429706744,21.1883274962121));
#58270=CARTESIAN_POINT('',(52.546116949762,29.0010979606402,20.3883274962121));
#58271=CARTESIAN_POINT('Ctrl Pts',(52.5526951386847,29.0013429706744,21.1883274962121));
#58272=CARTESIAN_POINT('Ctrl Pts',(52.5510980933635,29.3204313363915,21.1717985182499));
#58273=CARTESIAN_POINT('Ctrl Pts',(52.7571740168711,30.4528613238408,21.1130352634992));
#58274=CARTESIAN_POINT('Ctrl Pts',(54.4641895190608,31.8439653680504,21.0120377319602));
#58275=CARTESIAN_POINT('Ctrl Pts',(57.0938942397928,30.9977083845063,20.8853349015945));
#58276=CARTESIAN_POINT('Ctrl Pts',(57.8156459017858,28.3311427450632,20.7586320712293));
#58277=CARTESIAN_POINT('Ctrl Pts',(55.9717855603786,26.2740387563892,20.6319292408637));
#58278=CARTESIAN_POINT('Ctrl Pts',(53.3128323054721,26.6898183773978,20.5084943825248));
#58279=CARTESIAN_POINT('Ctrl Pts',(52.5503076068562,28.2540245866119,20.4272938009741));
#58280=CARTESIAN_POINT('Ctrl Pts',(52.546116949762,29.0010979606402,20.3883274962121));
#58281=CARTESIAN_POINT('',(52.5495689100241,28.9977886599613,19.5883274962121));
#58282=CARTESIAN_POINT('Ctrl Pts',(52.546116949762,29.0010979606402,20.3883274962121));
#58283=CARTESIAN_POINT('Ctrl Pts',(52.5457654935425,29.0637524746597,20.3850595241856));
#58284=CARTESIAN_POINT('Ctrl Pts',(52.5762972871919,29.9357868722756,20.3395572753712));
#58285=CARTESIAN_POINT('Ctrl Pts',(53.6159095712962,31.541559670917,20.2518207497671));
#58286=CARTESIAN_POINT('Ctrl Pts',(56.3784244236166,31.5446371025649,20.125117919402));
#58287=CARTESIAN_POINT('Ctrl Pts',(57.8849211638169,29.2290453097147,19.9984150890365));
#58288=CARTESIAN_POINT('Ctrl Pts',(56.7626823916054,26.704747799967,19.871712258671));
#58289=CARTESIAN_POINT('Ctrl Pts',(54.0342902665226,26.2718803937405,19.7450094283056));
#58290=CARTESIAN_POINT('Ctrl Pts',(52.6562115032221,27.8024599995536,19.6505478408193));
#58291=CARTESIAN_POINT('Ctrl Pts',(52.547821720126,28.8054976079726,19.5983205301214));
#58292=CARTESIAN_POINT('Ctrl Pts',(52.5495689100241,28.9977886599613,19.5883274962121));
#58293=CARTESIAN_POINT('',(52.553285085785,29.0006607136179,18.7883274962121));
#58294=CARTESIAN_POINT('Ctrl Pts',(52.5495689100241,28.9977886599613,19.5883274962121));
#58295=CARTESIAN_POINT('Ctrl Pts',(52.5552059942539,29.6181910889828,19.5560862533329));
#58296=CARTESIAN_POINT('Ctrl Pts',(53.1089152944742,31.0602443464707,19.4816107336654));
#58297=CARTESIAN_POINT('Ctrl Pts',(55.529472822231,31.8451520883635,19.3649009372091));
#58298=CARTESIAN_POINT('Ctrl Pts',(57.6748307788521,30.1047679303366,19.2381981068439));
#58299=CARTESIAN_POINT('Ctrl Pts',(57.3828872430288,27.3577210156594,19.1114952764783));
#58300=CARTESIAN_POINT('Ctrl Pts',(54.9196606938342,26.1071160632887,18.9847924461128));
#58301=CARTESIAN_POINT('Ctrl Pts',(52.8876672972278,27.2849697601211,18.8770698526908));
#58302=CARTESIAN_POINT('Ctrl Pts',(52.5543748892619,28.5514755235239,18.8115815360572));
#58303=CARTESIAN_POINT('Ctrl Pts',(52.553285085785,29.0006607136179,18.7883274962121));
#58304=CARTESIAN_POINT('',(52.5471787931917,29.0017322249443,17.9883274962121));
#58305=CARTESIAN_POINT('Ctrl Pts',(52.553285085785,29.0006607136179,18.7883274962121));
#58306=CARTESIAN_POINT('Ctrl Pts',(52.552395574614,29.3672912602337,18.7693472592687));
#58307=CARTESIAN_POINT('Ctrl Pts',(52.8014692833217,30.5485894345094,18.7081327455369));
#58308=CARTESIAN_POINT('Ctrl Pts',(54.6292489299202,31.8701525254662,18.6046839550165));
#58309=CARTESIAN_POINT('Ctrl Pts',(57.2057191633969,30.8735086996375,18.477981124651));
#58310=CARTESIAN_POINT('Ctrl Pts',(57.7723416519745,28.1697267677909,18.3512782942857));
#58311=CARTESIAN_POINT('Ctrl Pts',(55.8128108977569,26.2224884662913,18.2245754639201));
#58312=CARTESIAN_POINT('Ctrl Pts',(53.2345306382145,26.779769950788,18.1035918645624));
#58313=CARTESIAN_POINT('Ctrl Pts',(52.5528064276185,28.3008580228539,18.0248425419929));
#58314=CARTESIAN_POINT('Ctrl Pts',(52.5471787931917,29.0017322249443,17.9883274962121));
#58315=CARTESIAN_POINT('',(52.5495008502318,28.9979586805009,17.1883274962121));
#58316=CARTESIAN_POINT('Ctrl Pts',(52.5471787931917,29.0017322249443,17.9883274962121));
#58317=CARTESIAN_POINT('Ctrl Pts',(52.5462973554,29.1115078361563,17.9826082652045));
#58318=CARTESIAN_POINT('Ctrl Pts',(52.602769458379,30.0310210786956,17.9346547574086));
#58319=CARTESIAN_POINT('Ctrl Pts',(53.7649272708013,31.6172174592488,17.8444669728237));
#58320=CARTESIAN_POINT('Ctrl Pts',(56.5230134408625,31.4608254579201,17.7177641424583));
#58321=CARTESIAN_POINT('Ctrl Pts',(57.893332219512,29.0621332674915,17.5910613120929));
#58322=CARTESIAN_POINT('Ctrl Pts',(56.6272513453282,26.6068253439157,17.4643584817274));
#58323=CARTESIAN_POINT('Ctrl Pts',(53.8784216692723,26.3321743078981,17.3376556513621));
#58324=CARTESIAN_POINT('Ctrl Pts',(52.624400967416,27.898034156911,17.2456453228568));
#58325=CARTESIAN_POINT('Ctrl Pts',(52.5468627294195,28.8530496528172,17.1958692711402));
#58326=CARTESIAN_POINT('Ctrl Pts',(52.5481572452887,28.9979575612485,17.1883274962121));
#58327=CARTESIAN_POINT('',(52.549500001991,28.9999012170075,16.3883274962515));
#58328=CARTESIAN_POINT('Ctrl Pts',(52.5495008502318,28.9979586805009,17.1883274962121));
#58329=CARTESIAN_POINT('Ctrl Pts',(52.5494314790664,29.0812351994276,17.1839909334796));
#58330=CARTESIAN_POINT('Ctrl Pts',(52.5536121190673,29.1646579537596,17.179654370747));
#58331=CARTESIAN_POINT('Ctrl Pts',(52.5620561956239,29.247750391935,17.1753178080145));
#58332=CARTESIAN_POINT('Ctrl Pts',(52.5701546732359,29.3274420249732,17.1711587320081));
#58333=CARTESIAN_POINT('Ctrl Pts',(52.5821743818546,29.4068293158971,17.1669996560017));
#58334=CARTESIAN_POINT('Ctrl Pts',(52.5980740820284,29.4854916421281,17.1628405799952));
#58335=CARTESIAN_POINT('Ctrl Pts',(52.6139649341711,29.5641101935265,17.1586838184749));
#58336=CARTESIAN_POINT('Ctrl Pts',(52.6337314001425,29.6420041114002,17.1545270569545));
#58337=CARTESIAN_POINT('Ctrl Pts',(52.6572807298755,29.7187605104534,17.1503702954342));
#58338=CARTESIAN_POINT('Ctrl Pts',(52.6808246581083,29.7954993039226,17.1462144873485));
#58339=CARTESIAN_POINT('Ctrl Pts',(52.7081495867769,29.8711006382324,17.1420586792628));
#58340=CARTESIAN_POINT('Ctrl Pts',(52.739112672509,29.9451659866872,17.1379028711772));
#58341=CARTESIAN_POINT('Ctrl Pts',(52.7700787847425,30.0192385746946,17.1337466568801));
#58342=CARTESIAN_POINT('Ctrl Pts',(52.8046835721578,30.0917744375175,17.129590442583));
#58343=CARTESIAN_POINT('Ctrl Pts',(52.8427363862768,30.1623957806642,17.1254342282859));
#58344=CARTESIAN_POINT('Ctrl Pts',(52.880828258598,30.2330896110309,17.1212737479638));
#58345=CARTESIAN_POINT('Ctrl Pts',(52.9223749893459,30.3018645791274,17.1171132676416));
#58346=CARTESIAN_POINT('Ctrl Pts',(52.9671408046875,30.3683690079921,17.1129527873195));
#58347=CARTESIAN_POINT('Ctrl Pts',(53.0119338967066,30.4349139592923,17.1087897719361));
#58348=CARTESIAN_POINT('Ctrl Pts',(53.0599496859862,30.4991852374112,17.1046267565528));
#58349=CARTESIAN_POINT('Ctrl Pts',(53.1109116253203,30.5608636592124,17.1004637411695));
#58350=CARTESIAN_POINT('Ctrl Pts',(53.1619539794875,30.6226394058027,17.0962941568017));
#58351=CARTESIAN_POINT('Ctrl Pts',(53.2159514314526,30.6818137848235,17.092124572434));
#58352=CARTESIAN_POINT('Ctrl Pts',(53.2725906863439,30.7381045173102,17.0879549880662));
#58353=CARTESIAN_POINT('Ctrl Pts',(53.2893668024256,30.7547774037091,17.0867199889211));
#58354=CARTESIAN_POINT('Ctrl Pts',(53.3063744677791,30.771197581093,17.0854849897761));
#58355=CARTESIAN_POINT('Ctrl Pts',(53.3236050203222,30.7873584201584,17.0842499906311));
#58356=CARTESIAN_POINT('Ctrl Pts',(53.3826579202126,30.8427451762758,17.0800173764596));
#58357=CARTESIAN_POINT('Ctrl Pts',(53.4445684874815,30.895305198464,17.0757847622881));
#58358=CARTESIAN_POINT('Ctrl Pts',(53.5090351101451,30.9447297877134,17.0715521481166));
#58359=CARTESIAN_POINT('Ctrl Pts',(53.5734097772245,30.994083877427,17.0673255713719));
#58360=CARTESIAN_POINT('Ctrl Pts',(53.6403328927217,31.0403111366677,17.0630989946271));
#58361=CARTESIAN_POINT('Ctrl Pts',(53.7094671982809,31.0831407388093,17.0588724178823));
#58362=CARTESIAN_POINT('Ctrl Pts',(53.7785247727665,31.1259228050521,17.0546505321483));
#58363=CARTESIAN_POINT('Ctrl Pts',(53.8497882679766,31.1653144637599,17.0504286464142));
#58364=CARTESIAN_POINT('Ctrl Pts',(53.9228897943695,31.2010869712318,17.0462067606802));
#58365=CARTESIAN_POINT('Ctrl Pts',(53.9959420160496,31.2368353512569,17.0419877224772));
#58366=CARTESIAN_POINT('Ctrl Pts',(54.0708293905801,31.2689692244317,17.0377686842742));
#58367=CARTESIAN_POINT('Ctrl Pts',(54.1471587699883,31.2973053968491,17.0335496460711));
#58368=CARTESIAN_POINT('Ctrl Pts',(54.223463223004,31.3256323157057,17.0293319856522));
#58369=CARTESIAN_POINT('Ctrl Pts',(54.3012083105334,31.3501638351956,17.0251143252332));
#58370=CARTESIAN_POINT('Ctrl Pts',(54.3799814924724,31.3707651297257,17.0208966648142));
#58371=CARTESIAN_POINT('Ctrl Pts',(54.4587530351714,31.3913659955506,17.0166790921632));
#58372=CARTESIAN_POINT('Ctrl Pts',(54.5385521800133,31.4080366826258,17.0124615195121));
#58373=CARTESIAN_POINT('Ctrl Pts',(54.6189532264553,31.4206927947121,17.0082439468611));
#58374=CARTESIAN_POINT('Ctrl Pts',(54.6994907581661,31.4333703912559,17.0040192146448));
#58375=CARTESIAN_POINT('Ctrl Pts',(54.7806317744697,31.4420197050398,16.9997944824285));
#58376=CARTESIAN_POINT('Ctrl Pts',(54.8619420234416,31.4466079058788,16.9955697502122));
#58377=CARTESIAN_POINT('Ctrl Pts',(54.9432319643261,31.4511949607665,16.9913460731671));
#58378=CARTESIAN_POINT('Ctrl Pts',(55.0246905870729,31.4517229492961,16.987122396122));
#58379=CARTESIAN_POINT('Ctrl Pts',(55.1058845752201,31.4482113280374,16.9828987190769));
#58380=CARTESIAN_POINT('Ctrl Pts',(55.1872258777314,31.4446933354664,16.9786673788007));
#58381=CARTESIAN_POINT('Ctrl Pts',(55.2683011222209,31.4371211291395,16.9744360385244));
#58382=CARTESIAN_POINT('Ctrl Pts',(55.3486822258607,31.4255661102862,16.9702046982482));
#58383=CARTESIAN_POINT('Ctrl Pts',(55.4288323127503,31.4140443007667,16.9659855189207));
#58384=CARTESIAN_POINT('Ctrl Pts',(55.5082918124677,31.3985627102043,16.9617663395931));
#58385=CARTESIAN_POINT('Ctrl Pts',(55.5866505546961,31.3792417650745,16.9575471602656));
#58386=CARTESIAN_POINT('Ctrl Pts',(55.6652588093043,31.3598592975815,16.9533145460941));
#58387=CARTESIAN_POINT('Ctrl Pts',(55.7430516446065,31.3365408703696,16.9490819319227));
#58388=CARTESIAN_POINT('Ctrl Pts',(55.8196059182785,31.3093714271903,16.9448493177512));
#58389=CARTESIAN_POINT('Ctrl Pts',(55.8960509944673,31.2822407386705,16.9406227410064));
#58390=CARTESIAN_POINT('Ctrl Pts',(55.9712605837468,31.2512700982966,16.9363961642616));
#58391=CARTESIAN_POINT('Ctrl Pts',(56.0448239061901,31.216594968652,16.9321695875168));
#58392=CARTESIAN_POINT('Ctrl Pts',(56.1183055818639,31.1819583243861,16.9279477017828));
#58393=CARTESIAN_POINT('Ctrl Pts',(56.1901442031871,31.1436255575711,16.9237258160488));
#58394=CARTESIAN_POINT('Ctrl Pts',(56.2599476148098,31.1017807349805,16.9195039303147));
#58395=CARTESIAN_POINT('Ctrl Pts',(56.329703946196,31.0599641354251,16.9152848921117));
#58396=CARTESIAN_POINT('Ctrl Pts',(56.397427396743,31.0146404229193,16.9110658539087));
#58397=CARTESIAN_POINT('Ctrl Pts',(56.4627502687065,30.9660396489896,16.9068468157057));
#58398=CARTESIAN_POINT('Ctrl Pts',(56.5280518086015,30.9174547463009,16.9026291552867));
#58399=CARTESIAN_POINT('Ctrl Pts',(56.5909539543505,30.8655951845633,16.8984114948677));
#58400=CARTESIAN_POINT('Ctrl Pts',(56.6511190236793,30.8107336136617,16.8941938344488));
#58401=CARTESIAN_POINT('Ctrl Pts',(56.7112828409957,30.7558731844087,16.8899762617977));
#58402=CARTESIAN_POINT('Ctrl Pts',(56.7687093526638,30.6980111840744,16.8857586891467));
#58403=CARTESIAN_POINT('Ctrl Pts',(56.8230960132702,30.6374587556327,16.8815411164956));
#58404=CARTESIAN_POINT('Ctrl Pts',(56.8775749982719,30.5768035360603,16.8773163842793));
#58405=CARTESIAN_POINT('Ctrl Pts',(56.9290034955704,30.513449098005,16.8730916520631));
#58406=CARTESIAN_POINT('Ctrl Pts',(56.9771175592805,30.4477418301565,16.8688669198468));
#58407=CARTESIAN_POINT('Ctrl Pts',(57.0252196059986,30.3820509733872,16.8646432428017));
#58408=CARTESIAN_POINT('Ctrl Pts',(57.0700086359976,30.3140088630182,16.8604195657566));
#58409=CARTESIAN_POINT('Ctrl Pts',(57.1112650721079,30.2439895680017,16.8561958887114));
#58410=CARTESIAN_POINT('Ctrl Pts',(57.1525963618593,30.1738432334328,16.8519645484352));
#58411=CARTESIAN_POINT('Ctrl Pts',(57.1903820326334,30.101712957807,16.847733208159));
#58412=CARTESIAN_POINT('Ctrl Pts',(57.224448928946,30.0279966986867,16.8435018678827));
#58413=CARTESIAN_POINT('Ctrl Pts',(57.2584179163805,29.9544923014329,16.8392826885552));
#58414=CARTESIAN_POINT('Ctrl Pts',(57.2886893833677,29.8794114781285,16.8350635092277));
#58415=CARTESIAN_POINT('Ctrl Pts',(57.3151410496224,29.803163850253,16.8308443299002));
#58416=CARTESIAN_POINT('Ctrl Pts',(57.3416769441076,29.7266734322744,16.8266117157287));
#58417=CARTESIAN_POINT('Ctrl Pts',(57.364467341359,29.6487242689363,16.8223791015573));
#58418=CARTESIAN_POINT('Ctrl Pts',(57.3833531353155,29.5697175461417,16.8181464873858));
#58419=CARTESIAN_POINT('Ctrl Pts',(57.4022119904603,29.4908235190188,16.813919910641));
#58420=CARTESIAN_POINT('Ctrl Pts',(57.4171771970483,29.4108753765981,16.8096933338962));
#58421=CARTESIAN_POINT('Ctrl Pts',(57.4281387555884,29.330291437385,16.8054667571514));
#58422=CARTESIAN_POINT('Ctrl Pts',(57.4390881480678,29.2497969370128,16.8012448714174));
#58423=CARTESIAN_POINT('Ctrl Pts',(57.4460426595963,29.1686684999841,16.7970229856834));
#58424=CARTESIAN_POINT('Ctrl Pts',(57.4489432003383,29.0873352821995,16.7928010999493));
#58425=CARTESIAN_POINT('Ctrl Pts',(57.4518417847555,29.0060569211481,16.7885820617463));
#58426=CARTESIAN_POINT('Ctrl Pts',(57.4506918123866,28.924574516711,16.7843630235433));
#58427=CARTESIAN_POINT('Ctrl Pts',(57.4454860813073,28.8433217432689,16.7801439853403));
#58428=CARTESIAN_POINT('Ctrl Pts',(57.44028205023,28.7620955040202,16.7759263249213));
#58429=CARTESIAN_POINT('Ctrl Pts',(57.4310249204237,28.6810992100852,16.7717086645023));
#58430=CARTESIAN_POINT('Ctrl Pts',(57.4177595629877,28.6007645486916,16.7674910040833));
#58431=CARTESIAN_POINT('Ctrl Pts',(57.4044944815989,28.5204315590319,16.7632734314323));
#58432=CARTESIAN_POINT('Ctrl Pts',(57.3872214152632,28.4407606326884,16.7590558587812));
#58433=CARTESIAN_POINT('Ctrl Pts',(57.3660366525896,28.3621749388721,16.7548382861302));
#58434=CARTESIAN_POINT('Ctrl Pts',(57.3448159275976,28.2834558414496,16.7506135539139));
#58435=CARTESIAN_POINT('Ctrl Pts',(57.3196703420827,28.2058261133501,16.7463888216976));
#58436=CARTESIAN_POINT('Ctrl Pts',(57.2907467632637,28.1296957333227,16.7421640894813));
#58437=CARTESIAN_POINT('Ctrl Pts',(57.2618304084119,28.0535843676561,16.7379404124362));
#58438=CARTESIAN_POINT('Ctrl Pts',(57.2291381537515,27.9789720196369,16.7337167353911));
#58439=CARTESIAN_POINT('Ctrl Pts',(57.1928642397683,27.9062465195734,16.729493058346));
#58440=CARTESIAN_POINT('Ctrl Pts',(57.1565245121863,27.8333890699528,16.7252617180697));
#58441=CARTESIAN_POINT('Ctrl Pts',(57.1165903669661,27.7624257158661,16.7210303777935));
#58442=CARTESIAN_POINT('Ctrl Pts',(57.0733013549653,27.6937183529197,16.7167990375172));
#58443=CARTESIAN_POINT('Ctrl Pts',(57.0301367563706,27.6252084561811,16.7125798581897));
#58444=CARTESIAN_POINT('Ctrl Pts',(56.9836368787229,27.5589419252595,16.7083606788622));
#58445=CARTESIAN_POINT('Ctrl Pts',(56.9340787533669,27.4952443302068,16.7041414995347));
#58446=CARTESIAN_POINT('Ctrl Pts',(56.8843628234641,27.4313439072617,16.6999088853632));
#58447=CARTESIAN_POINT('Ctrl Pts',(56.8313842094394,27.3697911597357,16.6956762711918));
#58448=CARTESIAN_POINT('Ctrl Pts',(56.7753928186813,27.3109379557355,16.6914436570203));
#58449=CARTESIAN_POINT('Ctrl Pts',(56.7194812943846,27.2521687003047,16.6872170802755));
#58450=CARTESIAN_POINT('Ctrl Pts',(56.6605658461699,27.196091674292,16.6829905035307));
#58451=CARTESIAN_POINT('Ctrl Pts',(56.5989374863409,27.1430268809771,16.6787639267859));
#58452=CARTESIAN_POINT('Ctrl Pts',(56.537377526855,27.090020983438,16.6745420410519));
#58453=CARTESIAN_POINT('Ctrl Pts',(56.4731109888984,27.0400209771942,16.6703201553179));
#58454=CARTESIAN_POINT('Ctrl Pts',(56.4064656907128,26.9933100611087,16.6660982695838));
#58455=CARTESIAN_POINT('Ctrl Pts',(56.3398653427142,26.9466306500875,16.6618792313808));
#58456=CARTESIAN_POINT('Ctrl Pts',(56.2708898003976,26.9032361892494,16.6576601931778));
#58457=CARTESIAN_POINT('Ctrl Pts',(56.1998989200406,26.8633688124327,16.6534411549748));
#58458=CARTESIAN_POINT('Ctrl Pts',(56.1289312227169,26.8235144548477,16.6492234945558));
#58459=CARTESIAN_POINT('Ctrl Pts',(56.0559498991074,26.78718512114,16.6450058341369));
#58460=CARTESIAN_POINT('Ctrl Pts',(55.9813414872116,26.7545781831742,16.6407881737179));
#58461=CARTESIAN_POINT('Ctrl Pts',(55.9067346278885,26.7219719237464,16.6365706010668));
#58462=CARTESIAN_POINT('Ctrl Pts',(55.8305011737406,26.6930880910062,16.6323530284158));
#58463=CARTESIAN_POINT('Ctrl Pts',(55.7530485093739,26.668076289299,16.6281354557647));
#58464=CARTESIAN_POINT('Ctrl Pts',(55.6754643647819,26.6430220286609,16.6239107235484));
#58465=CARTESIAN_POINT('Ctrl Pts',(55.5966573134268,26.6218530935813,16.6196859913322));
#58466=CARTESIAN_POINT('Ctrl Pts',(55.5170512104585,26.6046694808934,16.6154612591159));
#58467=CARTESIAN_POINT('Ctrl Pts',(55.4374649899492,26.5874901599931,16.6112375820708));
#58468=CARTESIAN_POINT('Ctrl Pts',(55.3570805803588,26.5742942255241,16.6070139050257));
#58469=CARTESIAN_POINT('Ctrl Pts',(55.2763290482109,26.5651298787995,16.6027902279805));
#58470=CARTESIAN_POINT('Ctrl Pts',(55.1954310044693,26.5559489047366,16.5985588877043));
#58471=CARTESIAN_POINT('Ctrl Pts',(55.1141649719844,26.5508141660023,16.5943275474281));
#58472=CARTESIAN_POINT('Ctrl Pts',(55.0329649296005,26.5497217375538,16.5900962071518));
#58473=CARTESIAN_POINT('Ctrl Pts',(54.9519982576119,26.5486324487644,16.5858770278243));
#58474=CARTESIAN_POINT('Ctrl Pts',(54.8710976488593,26.5515621663447,16.5816578484968));
#58475=CARTESIAN_POINT('Ctrl Pts',(54.7906870158031,26.5584557500126,16.5774386691693));
#58476=CARTESIAN_POINT('Ctrl Pts',(54.7100203366712,26.5653712844472,16.5732060549978));
#58477=CARTESIAN_POINT('Ctrl Pts',(54.6295467390401,26.5763017170233,16.5689734408263));
#58478=CARTESIAN_POINT('Ctrl Pts',(54.5496974285382,26.5912289764,16.5647408266549));
#58479=CARTESIAN_POINT('Ctrl Pts',(54.4699620155803,26.6061349434429,16.5605142499101));
#58480=CARTESIAN_POINT('Ctrl Pts',(54.3908495739733,26.6250263295152,16.5562876731653));
#58481=CARTESIAN_POINT('Ctrl Pts',(54.3127869578739,26.6478332361987,16.5520610964205));
#58482=CARTESIAN_POINT('Ctrl Pts',(54.2348109822389,26.6706148298567,16.5478392106865));
#58483=CARTESIAN_POINT('Ctrl Pts',(54.1578829605515,26.6973031794606,16.5436173249524));
#58484=CARTESIAN_POINT('Ctrl Pts',(54.0824189116775,26.7277774764885,16.5393954392184));
#58485=CARTESIAN_POINT('Ctrl Pts',(54.0070057609643,26.7582312195481,16.5351764010154));
#58486=CARTESIAN_POINT('Ctrl Pts',(53.9330550516337,26.7924656650499,16.5309573628124));
#58487=CARTESIAN_POINT('Ctrl Pts',(53.8609657977053,26.8303107743267,16.5267383246093));
#58488=CARTESIAN_POINT('Ctrl Pts',(53.788900085499,26.8681435247706,16.5225206641903));
#58489=CARTESIAN_POINT('Ctrl Pts',(53.7186950324747,26.9095843815824,16.5183030037714));
#58490=CARTESIAN_POINT('Ctrl Pts',(53.6507266307302,26.9544165563392,16.5140853433524));
#58491=CARTESIAN_POINT('Ctrl Pts',(53.5827596433824,26.9992477981553,16.5098677707014));
#58492=CARTESIAN_POINT('Ctrl Pts',(53.5170296019134,27.0474699608352,16.5056501980503));
#58493=CARTESIAN_POINT('Ctrl Pts',(53.45388377873,27.0988227646204,16.5014326253993));
#58494=CARTESIAN_POINT('Ctrl Pts',(53.3906307619834,27.1502627426593,16.497207893183));
#58495=CARTESIAN_POINT('Ctrl Pts',(53.3299711029042,27.2048437001086,16.4929831609667));
#58496=CARTESIAN_POINT('Ctrl Pts',(53.2722194284441,27.2622645349324,16.4887584287504));
#58497=CARTESIAN_POINT('Ctrl Pts',(53.2144821780702,27.3196710283005,16.4845347517053));
#58498=CARTESIAN_POINT('Ctrl Pts',(53.1596517579463,27.3799156215909,16.4803110746602));
#58499=CARTESIAN_POINT('Ctrl Pts',(53.1080032735126,27.4426629661628,16.4760873976151));
#58500=CARTESIAN_POINT('Ctrl Pts',(53.0562610806182,27.5055241564192,16.4718560573388));
#58501=CARTESIAN_POINT('Ctrl Pts',(53.007712638625,27.570896798692,16.4676247170626));
#58502=CARTESIAN_POINT('Ctrl Pts',(52.9625909135407,27.6384147237822,16.4633933767863));
#58503=CARTESIAN_POINT('Ctrl Pts',(52.9175988691131,27.7057386011304,16.4591741974588));
#58504=CARTESIAN_POINT('Ctrl Pts',(52.8760140334964,27.7751950132776,16.4549550181313));
#58505=CARTESIAN_POINT('Ctrl Pts',(52.8380209319162,27.8463983533439,16.4507358388038));
#58506=CARTESIAN_POINT('Ctrl Pts',(52.7978259282973,27.921728305167,16.4462721356239));
#58507=CARTESIAN_POINT('Ctrl Pts',(52.7615146012321,27.9992682907874,16.441808432444));
#58508=CARTESIAN_POINT('Ctrl Pts',(52.7293216506219,28.0786042741223,16.4373447292641));
#58509=CARTESIAN_POINT('Ctrl Pts',(52.6972217088438,28.1577110474281,16.4328939221938));
#58510=CARTESIAN_POINT('Ctrl Pts',(52.6692165851757,28.2386031219828,16.4284431151235));
#58511=CARTESIAN_POINT('Ctrl Pts',(52.6454942862122,28.3208438370001,16.4239923080532));
#58512=CARTESIAN_POINT('Ctrl Pts',(52.6218134302734,28.4029408769049,16.4195492765744));
#58513=CARTESIAN_POINT('Ctrl Pts',(52.6024006204135,28.4863814977593,16.4151062450956));
#58514=CARTESIAN_POINT('Ctrl Pts',(52.5873954735558,28.5707102971405,16.4106632136169));
#58515=CARTESIAN_POINT('Ctrl Pts',(52.5724246591913,28.6548461481984,16.4062303480064));
#58516=CARTESIAN_POINT('Ctrl Pts',(52.5618414865605,28.7398657476831,16.401797482396));
#58517=CARTESIAN_POINT('Ctrl Pts',(52.5557351608016,28.8253012711598,16.3973646167856));
#58518=CARTESIAN_POINT('Ctrl Pts',(52.5515855800147,28.883359360547,16.3943522432743));
#58519=CARTESIAN_POINT('Ctrl Pts',(52.5495023518216,28.9416092003001,16.3913398697629));
#58520=CARTESIAN_POINT('Ctrl Pts',(52.549500001991,28.9999012170075,16.3883274962515));
#58521=CARTESIAN_POINT('',(52.549500910706,29.0021126687846,15.5883274962626));
#58522=CARTESIAN_POINT('Ctrl Pts',(52.549500001991,28.9999012177705,16.3883274962121));
#58523=CARTESIAN_POINT('Ctrl Pts',(52.5494965672996,29.0851059289342,16.3839243475573));
#58524=CARTESIAN_POINT('Ctrl Pts',(52.5539413361584,29.1702316435544,16.3795211989024));
#58525=CARTESIAN_POINT('Ctrl Pts',(52.5627838559111,29.2548091776064,16.3751180502476));
#58526=CARTESIAN_POINT('Ctrl Pts',(52.5716489821169,29.3396029393975,16.3707036446687));
#58527=CARTESIAN_POINT('Ctrl Pts',(52.5849342869729,29.423845318605,16.3662892390898));
#58528=CARTESIAN_POINT('Ctrl Pts',(52.6025376868597,29.5070746563101,16.3618748335109));
#58529=CARTESIAN_POINT('Ctrl Pts',(52.62016388412,29.5904117805969,16.3574547110334));
#58530=CARTESIAN_POINT('Ctrl Pts',(52.6421192227754,29.6727328593025,16.3530345885559));
#58531=CARTESIAN_POINT('Ctrl Pts',(52.6682516765415,29.753591405238,16.3486144660783));
#58532=CARTESIAN_POINT('Ctrl Pts',(52.6944539806234,29.8346660807041,16.3441825289066));
#58533=CARTESIAN_POINT('Ctrl Pts',(52.7248555799906,29.9142700303812,16.3397505917348));
#58534=CARTESIAN_POINT('Ctrl Pts',(52.7592558778403,29.9919758207773,16.3353186545631));
#58535=CARTESIAN_POINT('Ctrl Pts',(52.7884552680145,30.0579334384259,16.3315567725215));
#58536=CARTESIAN_POINT('Ctrl Pts',(52.8205347695802,30.1225237429707,16.3277948904799));
#58537=CARTESIAN_POINT('Ctrl Pts',(52.8553466886114,30.1855009168913,16.3240330084383));
#58538=CARTESIAN_POINT('Ctrl Pts',(52.8945146955292,30.2563585556664,16.3198003942668));
#58539=CARTESIAN_POINT('Ctrl Pts',(52.9372709326651,30.3254047609059,16.3155677800953));
#58540=CARTESIAN_POINT('Ctrl Pts',(52.9834232843317,30.3922530660137,16.3113351659239));
#58541=CARTESIAN_POINT('Ctrl Pts',(53.0295098040021,30.459006018291,16.3071085891791));
#58542=CARTESIAN_POINT('Ctrl Pts',(53.0789825551811,30.5235669180335,16.3028820124343));
#58543=CARTESIAN_POINT('Ctrl Pts',(53.131603859933,30.5855743797699,16.2986554356895));
#58544=CARTESIAN_POINT('Ctrl Pts',(53.1841667611299,30.6475130204039,16.2944335499555));
#58545=CARTESIAN_POINT('Ctrl Pts',(53.2398709732091,30.7069035018126,16.2902116642214));
#58546=CARTESIAN_POINT('Ctrl Pts',(53.2984367340434,30.763415067971,16.2859897784874));
#58547=CARTESIAN_POINT('Ctrl Pts',(53.3569629940884,30.8198885188307,16.2817707402844));
#58548=CARTESIAN_POINT('Ctrl Pts',(53.4183466362554,30.8734865891656,16.2775517020814));
#58549=CARTESIAN_POINT('Ctrl Pts',(53.4822698611413,30.9239141029682,16.2733326638783));
#58550=CARTESIAN_POINT('Ctrl Pts',(53.5461722110325,30.9743251489833,16.2691150034594));
#58551=CARTESIAN_POINT('Ctrl Pts',(53.6126121321914,31.0215674071835,16.2648973430404));
#58552=CARTESIAN_POINT('Ctrl Pts',(53.6812385038008,31.0653857669071,16.2606796826214));
#58553=CARTESIAN_POINT('Ctrl Pts',(53.7498634473213,31.1092032147872,16.2564621099704));
#58554=CARTESIAN_POINT('Ctrl Pts',(53.8206743586554,31.1495966568427,16.2522445373193));
#58555=CARTESIAN_POINT('Ctrl Pts',(53.8932920919819,31.1863549246017,16.2480269646683));
#58556=CARTESIAN_POINT('Ctrl Pts',(53.9660330979681,31.2231755915741,16.243802232452));
#58557=CARTESIAN_POINT('Ctrl Pts',(54.0405866460044,31.2563485267905,16.2395775002357));
#58558=CARTESIAN_POINT('Ctrl Pts',(54.1165496017435,31.2857090024368,16.2353527680194));
#58559=CARTESIAN_POINT('Ctrl Pts',(54.192493584938,31.3150621449964,16.2311290909743));
#58560=CARTESIAN_POINT('Ctrl Pts',(54.2698458225861,31.3406046061649,16.2269054139292));
#58561=CARTESIAN_POINT('Ctrl Pts',(54.3481879977817,31.3622217008071,16.2226817368841));
#58562=CARTESIAN_POINT('Ctrl Pts',(54.4266723131526,31.3838780164388,16.2184503966079));
#58563=CARTESIAN_POINT('Ctrl Pts',(54.5061497007664,31.4015946311211,16.2142190563316));
#58564=CARTESIAN_POINT('Ctrl Pts',(54.5861908563781,31.4153078981064,16.2099877160554));
#58565=CARTESIAN_POINT('Ctrl Pts',(54.6660019722557,31.4289817529133,16.2057685367279));
#58566=CARTESIAN_POINT('Ctrl Pts',(54.7463731579651,31.4386752687481,16.2015493574004));
#58567=CARTESIAN_POINT('Ctrl Pts',(54.8268770843264,31.4443769566228,16.1973301780729));
#58568=CARTESIAN_POINT('Ctrl Pts',(54.9076373538314,31.4500967999921,16.1930975639015));
#58569=CARTESIAN_POINT('Ctrl Pts',(54.9888315826127,31.4518205994553,16.18886494973));
#58570=CARTESIAN_POINT('Ctrl Pts',(55.0700310048049,31.4494991137712,16.1846323355585));
#58571=CARTESIAN_POINT('Ctrl Pts',(55.1511146036455,31.4471809394685,16.1804057588137));
#58572=CARTESIAN_POINT('Ctrl Pts',(55.2322029206835,31.4408289535834,16.1761791820689));
#58573=CARTESIAN_POINT('Ctrl Pts',(55.312863424609,31.4304457878221,16.1719526053242));
#58574=CARTESIAN_POINT('Ctrl Pts',(55.3934344047154,31.4200741461724,16.1677307195901));
#58575=CARTESIAN_POINT('Ctrl Pts',(55.4735780567573,31.4056802737708,16.1635088338561));
#58576=CARTESIAN_POINT('Ctrl Pts',(55.5528646315092,31.3873187783005,16.1592869481221));
#58577=CARTESIAN_POINT('Ctrl Pts',(55.6320977299251,31.3689696670896,16.1550679099191));
#58578=CARTESIAN_POINT('Ctrl Pts',(55.7104744477495,31.3466583521943,16.1508488717161));
#58579=CARTESIAN_POINT('Ctrl Pts',(55.7875741736494,31.3204907177148,16.146629833513));
#58580=CARTESIAN_POINT('Ctrl Pts',(55.8646487215899,31.2943316286306,16.1424121730941));
#58581=CARTESIAN_POINT('Ctrl Pts',(55.940446666215,31.2643188701095,16.1381945126751));
#58582=CARTESIAN_POINT('Ctrl Pts',(56.01456286381,31.2306080887008,16.1339768522561));
#58583=CARTESIAN_POINT('Ctrl Pts',(56.088677519075,31.1968980088007,16.1297592796051));
#58584=CARTESIAN_POINT('Ctrl Pts',(56.1611100745158,31.1594902524207,16.125541706954));
#58585=CARTESIAN_POINT('Ctrl Pts',(56.2314769894,31.1185878963541,16.121324134303));
#58586=CARTESIAN_POINT('Ctrl Pts',(56.301963356054,31.0776161062527,16.1170994020867));
#58587=CARTESIAN_POINT('Ctrl Pts',(56.3703766626418,31.033138082045,16.1128746698704));
#58588=CARTESIAN_POINT('Ctrl Pts',(56.4363592646534,30.9854023050365,16.1086499376541));
#58589=CARTESIAN_POINT('Ctrl Pts',(56.5023253868182,30.937678450539,16.104426260609));
#58590=CARTESIAN_POINT('Ctrl Pts',(56.5658616681585,30.8866987786574,16.1002025835639));
#58591=CARTESIAN_POINT('Ctrl Pts',(56.6266441758287,30.8327517494856,16.0959789065188));
#58592=CARTESIAN_POINT('Ctrl Pts',(56.6875369642803,30.7787068414873,16.0917475662425));
#58593=CARTESIAN_POINT('Ctrl Pts',(56.7456656615169,30.7216841430657,16.0875162259663));
#58594=CARTESIAN_POINT('Ctrl Pts',(56.8007431654636,30.662009116111,16.08328488569));
#58595=CARTESIAN_POINT('Ctrl Pts',(56.8556623756647,30.6025055962665,16.0790657063625));
#58596=CARTESIAN_POINT('Ctrl Pts',(56.9075476795902,30.5403653759723,16.074846527035));
#58597=CARTESIAN_POINT('Ctrl Pts',(56.9561568016372,30.4759406551106,16.0706273477075));
#58598=CARTESIAN_POINT('Ctrl Pts',(57.0049207063848,30.4113107910195,16.066394733536));
#58599=CARTESIAN_POINT('Ctrl Pts',(57.0505688764742,30.3441414614153,16.0621621193645));
#58600=CARTESIAN_POINT('Ctrl Pts',(57.092826586627,30.2747655189514,16.0579295051931));
#58601=CARTESIAN_POINT('Ctrl Pts',(57.1350240201241,30.2054885347552,16.0537029284483));
#58602=CARTESIAN_POINT('Ctrl Pts',(57.1738403592937,30.1340115825381,16.0494763517035));
#58603=CARTESIAN_POINT('Ctrl Pts',(57.2090423412836,30.0606989131776,16.0452497749587));
#58604=CARTESIAN_POINT('Ctrl Pts',(57.2442052531498,29.9874676123909,16.0410278892247));
#58605=CARTESIAN_POINT('Ctrl Pts',(57.2757615786477,29.9124050595007,16.0368060034906));
#58606=CARTESIAN_POINT('Ctrl Pts',(57.3035231682552,29.8359014674657,16.0325841177566));
#58607=CARTESIAN_POINT('Ctrl Pts',(57.3312660335314,29.7594494747312,16.0283650795536));
#58608=CARTESIAN_POINT('Ctrl Pts',(57.3552190881166,29.6815588087606,16.0241460413506));
#58609=CARTESIAN_POINT('Ctrl Pts',(57.3752421691163,29.6026399323407,16.0199270031475));
#58610=CARTESIAN_POINT('Ctrl Pts',(57.3952587113078,29.5237468279485,16.0157093427286));
#58611=CARTESIAN_POINT('Ctrl Pts',(57.4113477144833,29.4438266298739,16.0114916823096));
#58612=CARTESIAN_POINT('Ctrl Pts',(57.42341917833,29.3633039169929,16.0072740218906));
#58613=CARTESIAN_POINT('Ctrl Pts',(57.4354903909741,29.2827828797592,16.0030564492396));
#58614=CARTESIAN_POINT('Ctrl Pts',(57.4435441628035,29.2016598122362,15.9988388765885));
#58615=CARTESIAN_POINT('Ctrl Pts',(57.4475420398717,29.1203669932358,15.9946213039375));
#58616=CARTESIAN_POINT('Ctrl Pts',(57.4515467035597,29.0389361751326,15.9903965717212));
#58617=CARTESIAN_POINT('Ctrl Pts',(57.4514816740545,28.9573354954365,15.9861718395049));
#58618=CARTESIAN_POINT('Ctrl Pts',(57.4473606817844,28.876000228808,15.9819471072886));
#58619=CARTESIAN_POINT('Ctrl Pts',(57.4432407187754,28.7946852765152,15.9777234302435));
#58620=CARTESIAN_POINT('Ctrl Pts',(57.4350668867047,28.7136360663957,15.9734997531984));
#58621=CARTESIAN_POINT('Ctrl Pts',(57.4229048038741,28.6332813593999,15.9692760761533));
#58622=CARTESIAN_POINT('Ctrl Pts',(57.4107206547609,28.5527808607906,15.965044735877));
#58623=CARTESIAN_POINT('Ctrl Pts',(57.3945338864326,28.472977840116,15.9608133956008));
#58624=CARTESIAN_POINT('Ctrl Pts',(57.3744612059323,28.3942903075546,15.9565820553245));
#58625=CARTESIAN_POINT('Ctrl Pts',(57.3544462146801,28.3158289243897,15.952362875997));
#58626=CARTESIAN_POINT('Ctrl Pts',(57.3305678315509,28.2384770364956,15.9481436966695));
#58627=CARTESIAN_POINT('Ctrl Pts',(57.3029895956575,28.1626296086599,15.943924517342));
#58628=CARTESIAN_POINT('Ctrl Pts',(57.2753235442751,28.0865406650506,15.9396919031705));
#58629=CARTESIAN_POINT('Ctrl Pts',(57.2438311166961,28.0116827912019,15.9354592889991));
#58630=CARTESIAN_POINT('Ctrl Pts',(57.2086419574601,27.9384676388604,15.9312266748276));
#58631=CARTESIAN_POINT('Ctrl Pts',(57.1735029922558,27.8653569210592,15.9270000980828));
#58632=CARTESIAN_POINT('Ctrl Pts',(57.134677967898,27.7938846861118,15.922773521338));
#58633=CARTESIAN_POINT('Ctrl Pts',(57.0923454387272,27.7244448992547,15.9185469445932));
#58634=CARTESIAN_POINT('Ctrl Pts',(57.0500598937618,27.6550821825201,15.9143250588592));
#58635=CARTESIAN_POINT('Ctrl Pts',(57.0042748198077,27.5877478262943,15.9101031731252));
#58636=CARTESIAN_POINT('Ctrl Pts',(56.9552151085869,27.5228120873925,15.9058812873912));
#58637=CARTESIAN_POINT('Ctrl Pts',(56.9061884866198,27.4579201456329,15.9016622491881));
#58638=CARTESIAN_POINT('Ctrl Pts',(56.8538918932527,27.3954239778184,15.8974432109851));
#58639=CARTESIAN_POINT('Ctrl Pts',(56.7985933302329,27.3356646123928,15.8932241727821));
#58640=CARTESIAN_POINT('Ctrl Pts',(56.7433128257078,27.2759247621973,15.8890065123631));
#58641=CARTESIAN_POINT('Ctrl Pts',(56.6850326136842,27.2189202801812,15.8847888519442));
#58642=CARTESIAN_POINT('Ctrl Pts',(56.6240598453912,27.1649578019598,15.8805711915252));
#58643=CARTESIAN_POINT('Ctrl Pts',(56.5630883459184,27.1109964466773,15.8763536188742));
#58644=CARTESIAN_POINT('Ctrl Pts',(56.4994247502327,27.0600772763247,15.8721360462231));
#58645=CARTESIAN_POINT('Ctrl Pts',(56.4334107303472,27.0124678799764,15.8679184735721));
#58646=CARTESIAN_POINT('Ctrl Pts',(56.3672846479743,26.9647776640175,15.8636937413558));
#58647=CARTESIAN_POINT('Ctrl Pts',(56.2988005371564,26.9204087365886,15.8594690091395));
#58648=CARTESIAN_POINT('Ctrl Pts',(56.2283309921159,26.8795865441364,15.8552442769232));
#58649=CARTESIAN_POINT('Ctrl Pts',(56.1578790475833,26.8387745474548,15.8510205998781));
#58650=CARTESIAN_POINT('Ctrl Pts',(56.0854430847041,26.8015077086641,15.846796922833));
#58651=CARTESIAN_POINT('Ctrl Pts',(56.0114184816362,26.7679644032846,15.8425732457879));
#58652=CARTESIAN_POINT('Ctrl Pts',(55.9372595719828,26.7343602385877,15.8383419055116));
#58653=CARTESIAN_POINT('Ctrl Pts',(55.8615066952888,26.704493279414,15.8341105652354));
#58654=CARTESIAN_POINT('Ctrl Pts',(55.7845740244455,26.6784931940299,15.8298792249592));
#58655=CARTESIAN_POINT('Ctrl Pts',(55.7078624594941,26.652567833363,15.8256600456316));
#58656=CARTESIAN_POINT('Ctrl Pts',(55.6299783335128,26.6304871933858,15.8214408663041));
#58657=CARTESIAN_POINT('Ctrl Pts',(55.5513419837542,26.6123291125136,15.8172216869766));
#58658=CARTESIAN_POINT('Ctrl Pts',(55.4724552376491,26.5941132121073,15.8129890728051));
#58659=CARTESIAN_POINT('Ctrl Pts',(55.3925180616294,26.5797771679544,15.8087564586337));
#58660=CARTESIAN_POINT('Ctrl Pts',(55.311946338157,26.5694363344873,15.8045238444622));
#58661=CARTESIAN_POINT('Ctrl Pts',(55.2314895426829,26.5591102512482,15.8002972677174));
#58662=CARTESIAN_POINT('Ctrl Pts',(55.1504004543862,26.5527681188034,15.7960706909726));
#58663=CARTESIAN_POINT('Ctrl Pts',(55.0691067463729,26.55047463626,15.7918441142278));
#58664=CARTESIAN_POINT('Ctrl Pts',(54.9879032649618,26.5481836992166,15.7876222284938));
#58665=CARTESIAN_POINT('Ctrl Pts',(54.9064960771127,26.5499324964694,15.7834003427598));
#58666=CARTESIAN_POINT('Ctrl Pts',(54.8253181948176,26.5557339512774,15.7791784570258));
#58667=CARTESIAN_POINT('Ctrl Pts',(54.744195064487,26.5615314931839,15.7749594188227));
#58668=CARTESIAN_POINT('Ctrl Pts',(54.663301394714,26.5713762308611,15.7707403806197));
#58669=CARTESIAN_POINT('Ctrl Pts',(54.5830691491281,26.5852290138419,15.7665213424167));
#58670=CARTESIAN_POINT('Ctrl Pts',(54.5028631044684,26.5990772730088,15.7623036819977));
#58671=CARTESIAN_POINT('Ctrl Pts',(54.4233185124632,26.6169308991426,15.7580860215788));
#58672=CARTESIAN_POINT('Ctrl Pts',(54.3448598001788,26.6386991787199,15.7538683611598));
#58673=CARTESIAN_POINT('Ctrl Pts',(54.2664027205901,26.6604670053076,15.7496507885088));
#58674=CARTESIAN_POINT('Ctrl Pts',(54.1890319231182,26.6861491980422,15.7454332158577));
#58675=CARTESIAN_POINT('Ctrl Pts',(54.1131578747488,26.7156048295271,15.7412156432066));
#58676=CARTESIAN_POINT('Ctrl Pts',(54.0371550259428,26.7451104635923,15.7369909109903));
#58677=CARTESIAN_POINT('Ctrl Pts',(53.9626544451567,26.7784021835576,15.732766178774));
#58678=CARTESIAN_POINT('Ctrl Pts',(53.8900480831524,26.8152901812171,15.7285414465578));
#58679=CARTESIAN_POINT('Ctrl Pts',(53.8174598553484,26.8521689657124,15.7243177695126));
#58680=CARTESIAN_POINT('Ctrl Pts',(53.7467652942307,26.8926419816627,15.7200940924675));
#58681=CARTESIAN_POINT('Ctrl Pts',(53.678329269874,26.9364746836716,15.7158704154224));
#58682=CARTESIAN_POINT('Ctrl Pts',(53.6097690785732,26.9803869135711,15.7116390751462));
#58683=CARTESIAN_POINT('Ctrl Pts',(53.5434759926032,27.027670740936,15.7074077348699));
#58684=CARTESIAN_POINT('Ctrl Pts',(53.4797842570331,27.0780493386053,15.7031763945937));
#58685=CARTESIAN_POINT('Ctrl Pts',(53.4162755726665,27.1282831472709,15.6989572152661));
#58686=CARTESIAN_POINT('Ctrl Pts',(53.3553535938367,27.1815935987523,15.6947380359386));
#58687=CARTESIAN_POINT('Ctrl Pts',(53.2973124453094,27.2376704788543,15.6905188566111));
#58688=CARTESIAN_POINT('Ctrl Pts',(53.2387376267668,27.2942629681442,15.6862608832632));
#58689=CARTESIAN_POINT('Ctrl Pts',(53.1828605070431,27.3539018189101,15.6820029099154));
#58690=CARTESIAN_POINT('Ctrl Pts',(53.1300199241262,27.4162939774583,15.6777449365675));
#58691=CARTESIAN_POINT('Ctrl Pts',(53.0783432331251,27.477311856524,15.6735807513742));
#58692=CARTESIAN_POINT('Ctrl Pts',(53.0295710384744,27.540962630188,15.6694165661809));
#58693=CARTESIAN_POINT('Ctrl Pts',(52.9839856291495,27.6069327702783,15.6652523809876));
#58694=CARTESIAN_POINT('Ctrl Pts',(52.9384430373197,27.6728409458896,15.6610921071331));
#58695=CARTESIAN_POINT('Ctrl Pts',(52.8960815645859,27.7410637747401,15.6569318332785));
#58696=CARTESIAN_POINT('Ctrl Pts',(52.8571433024632,27.8112546850474,15.652771559424));
#58697=CARTESIAN_POINT('Ctrl Pts',(52.8182288838058,27.881402614635,15.6486138330726));
#58698=CARTESIAN_POINT('Ctrl Pts',(52.782733747793,27.9535158159383,15.6444561067212));
#58699=CARTESIAN_POINT('Ctrl Pts',(52.7508558078707,28.0272201415473,15.6402983803698));
#58700=CARTESIAN_POINT('Ctrl Pts',(52.71765006469,28.1039944536092,15.6359674733609));
#58701=CARTESIAN_POINT('Ctrl Pts',(52.6883697254216,28.182494867485,15.631636566352));
#58702=CARTESIAN_POINT('Ctrl Pts',(52.6631838951662,28.262273260489,15.627305659343));
#58703=CARTESIAN_POINT('Ctrl Pts',(52.6390015006805,28.3388731800271,15.6231473012222));
#58704=CARTESIAN_POINT('Ctrl Pts',(52.6185936465048,28.416650678846,15.6189889431015));
#58705=CARTESIAN_POINT('Ctrl Pts',(52.602059037614,28.4951937095169,15.6148305849807));
#58706=CARTESIAN_POINT('Ctrl Pts',(52.5855195668995,28.5737598349202,15.6106710041395));
#58707=CARTESIAN_POINT('Ctrl Pts',(52.5728556877415,28.6530914674989,15.6065114232983));
#58708=CARTESIAN_POINT('Ctrl Pts',(52.5641146513142,28.7327682315704,15.6023518424571));
#58709=CARTESIAN_POINT('Ctrl Pts',(52.5553646363121,28.8125268376292,15.5981879889981));
#58710=CARTESIAN_POINT('Ctrl Pts',(52.5505455299891,28.892630804583,15.594024135539));
#58711=CARTESIAN_POINT('Ctrl Pts',(52.5496525457875,28.9726576585775,15.58986028208));
#58712=CARTESIAN_POINT('Ctrl Pts',(52.5495429715248,28.9824774107231,15.5893493534742));
#58713=CARTESIAN_POINT('Ctrl Pts',(52.5494924473865,28.9922960060854,15.5888384248684));
#58714=CARTESIAN_POINT('Ctrl Pts',(52.549500910706,29.0021126687846,15.5883274962626));
#58715=CARTESIAN_POINT('',(52.5495005156126,28.9984103405398,14.7883274961845));
#58716=CARTESIAN_POINT('Ctrl Pts',(52.5495009107069,29.0021126697551,15.5883274962121));
#58717=CARTESIAN_POINT('Ctrl Pts',(52.5496027197749,29.1202016554576,15.5821813096032));
#58718=CARTESIAN_POINT('Ctrl Pts',(52.5582439368934,29.2379333721702,15.5760351229943));
#58719=CARTESIAN_POINT('Ctrl Pts',(52.5752507941987,29.354318414658,15.5698889363854));
#58720=CARTESIAN_POINT('Ctrl Pts',(52.5808521598771,29.3926509043574,15.5678646330055));
#58721=CARTESIAN_POINT('Ctrl Pts',(52.5873606589403,29.4308375654985,15.5658403296256));
#58722=CARTESIAN_POINT('Ctrl Pts',(52.5947690610642,29.4688436630541,15.5638160262457));
#58723=CARTESIAN_POINT('Ctrl Pts',(52.6102592826036,29.5483105792856,15.5595834120742));
#58724=CARTESIAN_POINT('Ctrl Pts',(52.6297208255725,29.6271567752449,15.5553507979027));
#58725=CARTESIAN_POINT('Ctrl Pts',(52.653089674389,29.7049554408191,15.5511181837313));
#58726=CARTESIAN_POINT('Ctrl Pts',(52.6764251897368,29.7826431339017,15.5468916069865));
#58727=CARTESIAN_POINT('Ctrl Pts',(52.7036568089021,29.8592858230665,15.5426650302417));
#58728=CARTESIAN_POINT('Ctrl Pts',(52.734669450267,29.9344665592981,15.5384384534969));
#58729=CARTESIAN_POINT('Ctrl Pts',(52.7656476711912,30.0095638536182,15.5342165677629));
#58730=CARTESIAN_POINT('Ctrl Pts',(52.8003983996278,30.0832019918242,15.5299946820288));
#58731=CARTESIAN_POINT('Ctrl Pts',(52.8387570920477,30.1549802348204,15.5257727962948));
#58732=CARTESIAN_POINT('Ctrl Pts',(52.8770899127191,30.2267100656178,15.5215537580918));
#58733=CARTESIAN_POINT('Ctrl Pts',(52.9190256459222,30.2965820839802,15.5173347198887));
#58734=CARTESIAN_POINT('Ctrl Pts',(52.9643526154026,30.3642177156091,15.5131156816857));
#58735=CARTESIAN_POINT('Ctrl Pts',(53.0096647827474,30.4318312599067,15.5088980212667));
#58736=CARTESIAN_POINT('Ctrl Pts',(53.058365728613,30.4972094822384,15.5046803608478));
#58737=CARTESIAN_POINT('Ctrl Pts',(53.1101997527774,30.5600016908957,15.5004627004288));
#58738=CARTESIAN_POINT('Ctrl Pts',(53.1620326982953,30.6227925928708,15.4962451277777));
#58739=CARTESIAN_POINT('Ctrl Pts',(53.2169982958419,30.6829972306607,15.4920275551267));
#58740=CARTESIAN_POINT('Ctrl Pts',(53.2748006694688,30.7402981123747,15.4878099824756));
#58741=CARTESIAN_POINT('Ctrl Pts',(53.3327011658547,30.7976962655371,15.4835852502593));
#58742=CARTESIAN_POINT('Ctrl Pts',(53.3934477415336,30.852180471496,15.479360518043));
#58743=CARTESIAN_POINT('Ctrl Pts',(53.4567074178512,30.9034700564718,15.4751357858268));
#58744=CARTESIAN_POINT('Ctrl Pts',(53.5199512944015,30.9547468313359,15.4709121087816));
#58745=CARTESIAN_POINT('Ctrl Pts',(53.585706627575,31.0028303227957,15.4666884317365));
#58746=CARTESIAN_POINT('Ctrl Pts',(53.6536106083631,31.0474828097172,15.4624647546914));
#58747=CARTESIAN_POINT('Ctrl Pts',(53.7216377907818,31.0922163119068,15.4582334144152));
#58748=CARTESIAN_POINT('Ctrl Pts',(53.7918210100753,31.1335061327748,15.4540020741389));
#58749=CARTESIAN_POINT('Ctrl Pts',(53.863771312899,31.1711597409239,15.4497707338627));
#58750=CARTESIAN_POINT('Ctrl Pts',(53.9355148292464,31.2087051319198,15.4455515545352));
#58751=CARTESIAN_POINT('Ctrl Pts',(54.0090148372316,31.2426350680789,15.4413323752077));
#58752=CARTESIAN_POINT('Ctrl Pts',(54.0838682298706,31.2728072575033,15.4371131958802));
#58753=CARTESIAN_POINT('Ctrl Pts',(54.1589599730452,31.3030755221656,15.4328805817087));
#58754=CARTESIAN_POINT('Ctrl Pts',(54.2356930309845,31.3296746216102,15.4286479675372));
#58755=CARTESIAN_POINT('Ctrl Pts',(54.313674534464,31.3524258979523,15.4244153533658));
#58756=CARTESIAN_POINT('Ctrl Pts',(54.3915448046509,31.375144721735,15.420188776621));
#58757=CARTESIAN_POINT('Ctrl Pts',(54.4706595412482,31.3940264943716,15.4159621998762));
#58758=CARTESIAN_POINT('Ctrl Pts',(54.5506063463779,31.4089407618462,15.4117356231314));
#58759=CARTESIAN_POINT('Ctrl Pts',(54.6304644198115,31.4238384762109,15.4075137373974));
#58760=CARTESIAN_POINT('Ctrl Pts',(54.7111522724174,31.4347773503387,15.4032918516633));
#58761=CARTESIAN_POINT('Ctrl Pts',(54.7922441765024,31.4416772448059,15.3990699659293));
#58762=CARTESIAN_POINT('Ctrl Pts',(54.8732813866128,31.4485724855083,15.3948509277263));
#58763=CARTESIAN_POINT('Ctrl Pts',(54.9547216452721,31.4514341176995,15.3906318895233));
#58764=CARTESIAN_POINT('Ctrl Pts',(55.0361321580848,31.4502336046084,15.3864128513202));
#58765=CARTESIAN_POINT('Ctrl Pts',(55.1175160851921,31.449033483561,15.3821951909013));
#58766=CARTESIAN_POINT('Ctrl Pts',(55.1988698216021,31.4437738585199,15.3779775304823));
#58767=CARTESIAN_POINT('Ctrl Pts',(55.2797599948554,31.4344783004329,15.3737598700633));
#58768=CARTESIAN_POINT('Ctrl Pts',(55.3606484848149,31.4251829357829,15.3695422974123));
#58769=CARTESIAN_POINT('Ctrl Pts',(55.4410729694212,31.411851859275,15.3653247247612));
#58770=CARTESIAN_POINT('Ctrl Pts',(55.5206060533622,31.3945604162774,15.3611071521102));
#58771=CARTESIAN_POINT('Ctrl Pts',(55.6002741491573,31.3772396200892,15.3568824198939));
#58772=CARTESIAN_POINT('Ctrl Pts',(55.6790473603885,31.3559451055838,15.3526576876776));
#58773=CARTESIAN_POINT('Ctrl Pts',(55.756508976961,31.3308033846246,15.3484329554613));
#58774=CARTESIAN_POINT('Ctrl Pts',(55.8339512466824,31.3056679430738,15.3442092784162));
#58775=CARTESIAN_POINT('Ctrl Pts',(55.9100821487366,31.27668740229,15.3399856013711));
#58776=CARTESIAN_POINT('Ctrl Pts',(55.9845047631225,31.2440366800454,15.335761924326));
#58777=CARTESIAN_POINT('Ctrl Pts',(56.0590624062261,31.2113267179421,15.3315305840498));
#58778=CARTESIAN_POINT('Ctrl Pts',(56.131905150775,31.1749334748291,15.3272992437735));
#58779=CARTESIAN_POINT('Ctrl Pts',(56.2026597500616,31.1350784003361,15.3230679034973));
#58780=CARTESIAN_POINT('Ctrl Pts',(56.2732109993462,31.0953378700503,15.3188487241698));
#58781=CARTESIAN_POINT('Ctrl Pts',(56.341685749369,31.0521556937388,15.3146295448422));
#58782=CARTESIAN_POINT('Ctrl Pts',(56.4077451903292,31.0057925438851,15.3104103655147));
#58783=CARTESIAN_POINT('Ctrl Pts',(56.474014979846,30.9592817630265,15.3061777513432));
#58784=CARTESIAN_POINT('Ctrl Pts',(56.5381005140958,30.9093967094343,15.3019451371718));
#58785=CARTESIAN_POINT('Ctrl Pts',(56.5996380520154,30.8563696702286,15.2977125230003));
#58786=CARTESIAN_POINT('Ctrl Pts',(56.6610878124152,30.8034182691153,15.2934859462555));
#58787=CARTESIAN_POINT('Ctrl Pts',(56.719996446032,30.7473340844447,15.2892593695107));
#58788=CARTESIAN_POINT('Ctrl Pts',(56.776030015009,30.688392026689,15.2850327927659));
#58789=CARTESIAN_POINT('Ctrl Pts',(56.8320013932129,30.6295153877923,15.2808109070319));
#58790=CARTESIAN_POINT('Ctrl Pts',(56.8851037288051,30.5677875133758,15.2765890212979));
#58791=CARTESIAN_POINT('Ctrl Pts',(56.9350380323161,30.5035218866017,15.2723671355638));
#58792=CARTESIAN_POINT('Ctrl Pts',(56.9849386566879,30.439299605,15.2681480973608));
#58793=CARTESIAN_POINT('Ctrl Pts',(57.031675208438,30.3725433363819,15.2639290591578));
#58794=CARTESIAN_POINT('Ctrl Pts',(57.074988136585,30.3036005841635,15.2597100209548));
#58795=CARTESIAN_POINT('Ctrl Pts',(57.1182869203088,30.2346803461345,15.2554923605358));
#58796=CARTESIAN_POINT('Ctrl Pts',(57.1581640538318,30.1635754355767,15.2512747001168));
#58797=CARTESIAN_POINT('Ctrl Pts',(57.1944033807436,30.090662208285,15.2470570396979));
#58798=CARTESIAN_POINT('Ctrl Pts',(57.2306419535287,30.0177504982899,15.2428394670468));
#58799=CARTESIAN_POINT('Ctrl Pts',(57.2632426645084,29.9430309629015,15.2386218943958));
#58800=CARTESIAN_POINT('Ctrl Pts',(57.292036040926,29.8669031301688,15.2344043217447));
#58801=CARTESIAN_POINT('Ctrl Pts',(57.3208782957089,29.7906460661862,15.2301795895285));
#58802=CARTESIAN_POINT('Ctrl Pts',(57.3459001194426,29.7129763584957,15.2259548573122));
#58803=CARTESIAN_POINT('Ctrl Pts',(57.3669807761582,29.6343124271978,15.2217301250959));
#58804=CARTESIAN_POINT('Ctrl Pts',(57.3880561677587,29.5556681430415,15.2175064480508));
#58805=CARTESIAN_POINT('Ctrl Pts',(57.4051922835052,29.4760305920444,15.2132827710057));
#58806=CARTESIAN_POINT('Ctrl Pts',(57.4183197652693,29.3958279460926,15.2090590939606));
#58807=CARTESIAN_POINT('Ctrl Pts',(57.4314710648882,29.3154797844192,15.2048277536843));
#58808=CARTESIAN_POINT('Ctrl Pts',(57.4405991433208,29.2345649417645,15.2005964134081));
#58809=CARTESIAN_POINT('Ctrl Pts',(57.4456865622944,29.1535170642398,15.1963650731318));
#58810=CARTESIAN_POINT('Ctrl Pts',(57.4507593599335,29.0727021197859,15.1921458938043));
#58811=CARTESIAN_POINT('Ctrl Pts',(57.4518147701902,28.9917553604263,15.1879267144768));
#58812=CARTESIAN_POINT('Ctrl Pts',(57.4488870033909,28.9111028986792,15.1837075351493));
#58813=CARTESIAN_POINT('Ctrl Pts',(57.4459499139042,28.830193620818,15.1794749209778));
#58814=CARTESIAN_POINT('Ctrl Pts',(57.4389932889958,28.7492795945812,15.1752423068064));
#58815=CARTESIAN_POINT('Ctrl Pts',(57.4280139560343,28.6687923924442,15.1710096926349));
#58816=CARTESIAN_POINT('Ctrl Pts',(57.4170502840602,28.5884199977437,15.1667831158901));
#58817=CARTESIAN_POINT('Ctrl Pts',(57.4020753627368,28.5084736744004,15.1625565391453));
#58818=CARTESIAN_POINT('Ctrl Pts',(57.383137997865,28.4293831993957,15.1583299624005));
#58819=CARTESIAN_POINT('Ctrl Pts',(57.3642216512753,28.3503805056598,15.1541080766665));
#58820=CARTESIAN_POINT('Ctrl Pts',(57.3413517072913,28.2722322223294,15.1498861909324));
#58821=CARTESIAN_POINT('Ctrl Pts',(57.3146283533897,28.1953598098003,15.1456643051984));
#58822=CARTESIAN_POINT('Ctrl Pts',(57.2879230235615,28.1185392453296,15.1414452669954));
#58823=CARTESIAN_POINT('Ctrl Pts',(57.2573695978118,28.0429932802206,15.1372262287924));
#58824=CARTESIAN_POINT('Ctrl Pts',(57.223118271009,27.9691288135242,15.1330071905893));
#58825=CARTESIAN_POINT('Ctrl Pts',(57.1888781294407,27.8952884682696,15.1287895301704));
#58826=CARTESIAN_POINT('Ctrl Pts',(57.1509426803136,27.8231289520367,15.1245718697514));
#58827=CARTESIAN_POINT('Ctrl Pts',(57.1095099446389,27.7530364706737,15.1203542093324));
#58828=CARTESIAN_POINT('Ctrl Pts',(57.0680780711636,27.6829454479088,15.1161366366814));
#58829=CARTESIAN_POINT('Ctrl Pts',(57.0231492932417,27.6149217737984,15.1119190640304));
#58830=CARTESIAN_POINT('Ctrl Pts',(56.9749664839744,27.5493251097582,15.1077014913793));
#58831=CARTESIAN_POINT('Ctrl Pts',(56.9267018816959,27.4836170917155,15.103476759163));
#58832=CARTESIAN_POINT('Ctrl Pts',(56.8751724724945,27.4203447032426,15.0992520269467));
#58833=CARTESIAN_POINT('Ctrl Pts',(56.8206635089471,27.3598370089566,15.0950272947304));
#58834=CARTESIAN_POINT('Ctrl Pts',(56.766168159585,27.2993444271018,15.0908036176853));
#58835=CARTESIAN_POINT('Ctrl Pts',(56.7086950879882,27.2416154739421,15.0865799406402));
#58836=CARTESIAN_POINT('Ctrl Pts',(56.6485656969155,27.1869414259453,15.0823562635951));
#58837=CARTESIAN_POINT('Ctrl Pts',(56.588327210044,27.1321681800548,15.0781249233189));
#58838=CARTESIAN_POINT('Ctrl Pts',(56.5254231320117,27.0804612120078,15.0738935830426));
#58839=CARTESIAN_POINT('Ctrl Pts',(56.4602077227072,27.0320712267599,15.0696622427664));
#58840=CARTESIAN_POINT('Ctrl Pts',(56.3951797436721,26.9838203152075,15.0654430634389));
#58841=CARTESIAN_POINT('Ctrl Pts',(56.3278541260386,26.9388675293988,15.0612238841113));
#58842=CARTESIAN_POINT('Ctrl Pts',(56.2586069278663,26.8974161488476,15.0570047047838));
#58843=CARTESIAN_POINT('Ctrl Pts',(56.1891392305801,26.8558327775022,15.0527720906123));
#58844=CARTESIAN_POINT('Ctrl Pts',(56.1174793119124,26.8176185088514,15.0485394764409));
#58845=CARTESIAN_POINT('Ctrl Pts',(56.0439874585597,26.7830109525823,15.0443068622694));
#58846=CARTESIAN_POINT('Ctrl Pts',(55.9706004344353,26.7484527607427,15.0400802855246));
#58847=CARTESIAN_POINT('Ctrl Pts',(55.895387082334,26.7174912596412,15.0358537087798));
#58848=CARTESIAN_POINT('Ctrl Pts',(55.8187344799474,26.6903194806759,15.031627132035));
#58849=CARTESIAN_POINT('Ctrl Pts',(55.7421669530735,26.6631778592389,15.027405246301));
#58850=CARTESIAN_POINT('Ctrl Pts',(55.6641637855931,26.6398177567488,15.023183360567));
#58851=CARTESIAN_POINT('Ctrl Pts',(55.5851330512618,26.6203845768022,15.0189614748329));
#58852=CARTESIAN_POINT('Ctrl Pts',(55.5061556207098,26.6009645039328,15.0147424366299));
#58853=CARTESIAN_POINT('Ctrl Pts',(55.4261524497351,26.5854662039199,15.0105233984269));
#58854=CARTESIAN_POINT('Ctrl Pts',(55.3455466217338,26.5739852056905,15.0063043602239));
#58855=CARTESIAN_POINT('Ctrl Pts',(55.2649671166572,26.5625079567366,15.0020866998049));
#58856=CARTESIAN_POINT('Ctrl Pts',(55.1837858049525,26.5550454696606,14.9978690393859));
#58857=CARTESIAN_POINT('Ctrl Pts',(55.1024344486264,26.5516418902181,14.993651378967));
#58858=CARTESIAN_POINT('Ctrl Pts',(55.0210847851912,26.5482383816029,14.9894338063159));
#58859=CARTESIAN_POINT('Ctrl Pts',(54.939565548361,26.5488936309297,14.9852162336649));
#58860=CARTESIAN_POINT('Ctrl Pts',(54.8583106515168,26.5535997100788,14.9809986610138));
#58861=CARTESIAN_POINT('Ctrl Pts',(54.7769178199451,26.5583137780603,14.9767739287975));
#58862=CARTESIAN_POINT('Ctrl Pts',(54.6957906923802,26.5670924071531,14.9725491965812));
#58863=CARTESIAN_POINT('Ctrl Pts',(54.6153605882569,26.579875463342,14.968324464365));
#58864=CARTESIAN_POINT('Ctrl Pts',(54.5349505723956,26.5926553268287,14.9641007873199));
#58865=CARTESIAN_POINT('Ctrl Pts',(54.4552376836173,26.6094375005358,14.9598771102747));
#58866=CARTESIAN_POINT('Ctrl Pts',(54.3766412238928,26.6301109548652,14.9556534332296));
#58867=CARTESIAN_POINT('Ctrl Pts',(54.2979021626316,26.6508219180895,14.9514220929534));
#58868=CARTESIAN_POINT('Ctrl Pts',(54.2202840226028,26.6754381305557,14.9471907526771));
#58869=CARTESIAN_POINT('Ctrl Pts',(54.1441899608165,26.7037989141121,14.9429594124009));
#58870=CARTESIAN_POINT('Ctrl Pts',(54.0683145947448,26.7320781882619,14.9387402330734));
#58871=CARTESIAN_POINT('Ctrl Pts',(53.9939549434447,26.7640802819455,14.9345210537459));
#58872=CARTESIAN_POINT('Ctrl Pts',(53.9214862492111,26.7996004137068,14.9303018744184));
#58873=CARTESIAN_POINT('Ctrl Pts',(53.848786797874,26.8352336497928,14.9260692602469));
#58874=CARTESIAN_POINT('Ctrl Pts',(53.7777199877831,26.8745399187011,14.9218366460755));
#58875=CARTESIAN_POINT('Ctrl Pts',(53.7086812723065,26.9173463577666,14.917604031904));
#58876=CARTESIAN_POINT('Ctrl Pts',(53.6397410340751,26.9600917374661,14.9133774551592));
#58877=CARTESIAN_POINT('Ctrl Pts',(53.572823536347,27.0063271284838,14.9091508784144));
#58878=CARTESIAN_POINT('Ctrl Pts',(53.5083014241358,27.0558329267358,14.9049243016696));
#58879=CARTESIAN_POINT('Ctrl Pts',(53.4438509239977,27.1052837792844,14.9007024159356));
#58880=CARTESIAN_POINT('Ctrl Pts',(53.3817908934466,27.1579975453547,14.8964805302015));
#58881=CARTESIAN_POINT('Ctrl Pts',(53.3224654563689,27.2137110802213,14.8922586444675));
#58882=CARTESIAN_POINT('Ctrl Pts',(53.2631800324587,27.2693870380363,14.8880396062645));
#58883=CARTESIAN_POINT('Ctrl Pts',(53.2066258766436,27.3280584291,14.8838205680615));
#58884=CARTESIAN_POINT('Ctrl Pts',(53.1531134479394,27.3894223664108,14.8796015298584));
#58885=CARTESIAN_POINT('Ctrl Pts',(53.0996184944434,27.450766264497,14.8753838694395));
#58886=CARTESIAN_POINT('Ctrl Pts',(53.0491636004792,27.5148006127681,14.8711662090205));
#58887=CARTESIAN_POINT('Ctrl Pts',(53.0020208482047,27.5811872713458,14.8669485486015));
#58888=CARTESIAN_POINT('Ctrl Pts',(52.954879076953,27.6475725484422,14.8627309759505));
#58889=CARTESIAN_POINT('Ctrl Pts',(52.9110495783621,27.7163096590762,14.8585134032994));
#58890=CARTESIAN_POINT('Ctrl Pts',(52.8707619249197,27.7870303096827,14.8542958306484));
#58891=CARTESIAN_POINT('Ctrl Pts',(52.8304058809345,27.8578710125452,14.8500710984321));
#58892=CARTESIAN_POINT('Ctrl Pts',(52.7936039428232,27.93070158653,14.8458463662158));
#58893=CARTESIAN_POINT('Ctrl Pts',(52.7605404793052,28.0051274930076,14.8416216339995));
#58894=CARTESIAN_POINT('Ctrl Pts',(52.7274852737339,28.0795348108345,14.8373979569544));
#58895=CARTESIAN_POINT('Ctrl Pts',(52.6981668234897,28.1555362217884,14.8331742799093));
#58896=CARTESIAN_POINT('Ctrl Pts',(52.6727202624752,28.2327195601955,14.8289506028642));
#58897=CARTESIAN_POINT('Ctrl Pts',(52.6472275324766,28.3100429362417,14.8247192625879));
#58898=CARTESIAN_POINT('Ctrl Pts',(52.625620854484,28.3885520761161,14.8204879223117));
#58899=CARTESIAN_POINT('Ctrl Pts',(52.6079849266118,28.4678213282329,14.8162565820354));
#58900=CARTESIAN_POINT('Ctrl Pts',(52.5903996847164,28.5468627590806,14.8120374027079));
#58901=CARTESIAN_POINT('Ctrl Pts',(52.5767623941067,28.6266594760962,14.8078182233804));
#58902=CARTESIAN_POINT('Ctrl Pts',(52.5671055611392,28.7067852333864,14.8035990440529));
#58903=CARTESIAN_POINT('Ctrl Pts',(52.5554544180134,28.8034584045383,14.798508528106));
#58904=CARTESIAN_POINT('Ctrl Pts',(52.5495638106476,28.9008395066439,14.793418012159));
#58905=CARTESIAN_POINT('Ctrl Pts',(52.549500515613,28.9984103400116,14.7883274962121));
#58906=CARTESIAN_POINT('',(52.5495001466462,28.9991522304455,13.9883274962515));
#58907=CARTESIAN_POINT('Ctrl Pts',(52.5495005156126,28.9984103405398,14.7883274961845));
#58908=CARTESIAN_POINT('Ctrl Pts',(52.5494486476381,29.0783661096744,14.7841560024729));
#58909=CARTESIAN_POINT('Ctrl Pts',(52.5533142347253,29.1584742115312,14.7799845087613));
#58910=CARTESIAN_POINT('Ctrl Pts',(52.5611155699173,29.2383127917256,14.7758130150497));
#58911=CARTESIAN_POINT('Ctrl Pts',(52.5689063467647,29.318043318207,14.7716471670471));
#58912=CARTESIAN_POINT('Ctrl Pts',(52.5806222456023,29.3975045747558,14.7674813190444));
#58913=CARTESIAN_POINT('Ctrl Pts',(52.5962295353568,29.4762749240818,14.7633154710417));
#58914=CARTESIAN_POINT('Ctrl Pts',(52.6118251610571,29.5549864046583,14.7591527363712));
#58915=CARTESIAN_POINT('Ctrl Pts',(52.6313063172899,29.6330075345443,14.7549900017007));
#58916=CARTESIAN_POINT('Ctrl Pts',(52.654587629556,29.7099232793536,14.7508272670302));
#58917=CARTESIAN_POINT('Ctrl Pts',(52.6778591264256,29.7868065965009,14.7466662873678));
#58918=CARTESIAN_POINT('Ctrl Pts',(52.7049274619381,29.862584995857,14.7425053077053));
#58919=CARTESIAN_POINT('Ctrl Pts',(52.7356568709464,29.9368566826937,14.7383443280429));
#58920=CARTESIAN_POINT('Ctrl Pts',(52.7663833333954,30.0111212478207,14.7341837473655));
#58921=CARTESIAN_POINT('Ctrl Pts',(52.8007699881503,30.0838789456754,14.730023166688));
#58922=CARTESIAN_POINT('Ctrl Pts',(52.8386328050145,30.1547476340918,14.7258625860106));
#58923=CARTESIAN_POINT('Ctrl Pts',(52.8765298797931,30.2256804438194,14.7216982408796));
#58924=CARTESIAN_POINT('Ctrl Pts',(52.9179091736609,30.2947204068032,14.7175338957486));
#58925=CARTESIAN_POINT('Ctrl Pts',(52.9625408723203,30.3615103940237,14.7133695506176));
#58926=CARTESIAN_POINT('Ctrl Pts',(53.0071919011386,30.4283293082424,14.7092034018928));
#58927=CARTESIAN_POINT('Ctrl Pts',(53.0550978534665,30.4928959221122,14.7050372531681));
#58928=CARTESIAN_POINT('Ctrl Pts',(53.1059873434397,30.554884660285,14.7008711044433));
#58929=CARTESIAN_POINT('Ctrl Pts',(53.1569665143059,30.6169826391947,14.6966976138501));
#58930=CARTESIAN_POINT('Ctrl Pts',(53.2109394031175,30.6764933129995,14.692524123257));
#58931=CARTESIAN_POINT('Ctrl Pts',(53.2675966059561,30.7331268650348,14.6883506326638));
#58932=CARTESIAN_POINT('Ctrl Pts',(53.3194297437781,30.7849383657958,14.684532493005));
#58933=CARTESIAN_POINT('Ctrl Pts',(53.3735088997252,30.8343421090488,14.6807143533463));
#58934=CARTESIAN_POINT('Ctrl Pts',(53.4295743626424,30.8811468755868,14.6768962136875));
#58935=CARTESIAN_POINT('Ctrl Pts',(53.4917259584669,30.9330324889603,14.672663599516));
#58936=CARTESIAN_POINT('Ctrl Pts',(53.5565672853796,30.981931124894,14.6684309853445));
#58937=CARTESIAN_POINT('Ctrl Pts',(53.6237794148746,31.0275520094629,14.664198371173));
#58938=CARTESIAN_POINT('Ctrl Pts',(53.690895672578,31.0731078201237,14.6599717944283));
#58939=CARTESIAN_POINT('Ctrl Pts',(53.7603756351425,31.115394906649,14.6557452176835));
#58940=CARTESIAN_POINT('Ctrl Pts',(53.8318669732864,31.1541623620101,14.6515186409387));
#58941=CARTESIAN_POINT('Ctrl Pts',(53.9032789643233,31.1928867899848,14.6472967552046));
#58942=CARTESIAN_POINT('Ctrl Pts',(53.9766974888646,31.2280991284402,14.6430748694706));
#58943=CARTESIAN_POINT('Ctrl Pts',(54.0517420667263,31.2595922512665,14.6388529837366));
#58944=CARTESIAN_POINT('Ctrl Pts',(54.1267360293474,31.2910641329581,14.6346339455336));
#58945=CARTESIAN_POINT('Ctrl Pts',(54.2033534398501,31.3188216018119,14.6304149073305));
#58946=CARTESIAN_POINT('Ctrl Pts',(54.2811912310675,31.342704463586,14.6261958691275));
#58947=CARTESIAN_POINT('Ctrl Pts',(54.3590036033,31.3665795260882,14.6219782087085));
#58948=CARTESIAN_POINT('Ctrl Pts',(54.4380351210145,31.3865823581674,14.6177605482896));
#58949=CARTESIAN_POINT('Ctrl Pts',(54.5178661492761,31.4026021726424,14.6135428878706));
#58950=CARTESIAN_POINT('Ctrl Pts',(54.5976955162842,31.4186216537512,14.6093253152196));
#58951=CARTESIAN_POINT('Ctrl Pts',(54.6783239050611,31.4306581918046,14.6051077425685));
#58952=CARTESIAN_POINT('Ctrl Pts',(54.7593214531776,31.438652104565,14.6008901699174));
#58953=CARTESIAN_POINT('Ctrl Pts',(54.8404564991578,31.446659587439,14.5966654377012));
#58954=CARTESIAN_POINT('Ctrl Pts',(54.921961493559,31.4506106687288,14.5924407054849));
#58955=CARTESIAN_POINT('Ctrl Pts',(55.0034010134452,31.4504976398902,14.5882159732686));
#58956=CARTESIAN_POINT('Ctrl Pts',(55.0848201929573,31.4503846392818,14.5839922962235));
#58957=CARTESIAN_POINT('Ctrl Pts',(55.1661734662046,31.4462096035141,14.5797686191784));
#58958=CARTESIAN_POINT('Ctrl Pts',(55.2470293623713,31.4380169696141,14.5755449421332));
#58959=CARTESIAN_POINT('Ctrl Pts',(55.3280319594846,31.4298094714036,14.571313601857));
#58960=CARTESIAN_POINT('Ctrl Pts',(55.4085349154643,31.4175698776105,14.5670822615808));
#58961=CARTESIAN_POINT('Ctrl Pts',(55.4881149828723,31.4013941811988,14.5628509213045));
#58962=CARTESIAN_POINT('Ctrl Pts',(55.5674663357224,31.3852649740322,14.558631741977));
#58963=CARTESIAN_POINT('Ctrl Pts',(55.6458996772294,31.3652224521933,14.5544125626495));
#58964=CARTESIAN_POINT('Ctrl Pts',(55.7230124725475,31.341410518158,14.550193383322));
#58965=CARTESIAN_POINT('Ctrl Pts',(55.8003708128623,31.3175227614107,14.5459607691505));
#58966=CARTESIAN_POINT('Ctrl Pts',(55.87668789292,31.2897526774452,14.5417281549791));
#58967=CARTESIAN_POINT('Ctrl Pts',(55.9515461792811,31.2582094939787,14.5374955408076));
#58968=CARTESIAN_POINT('Ctrl Pts',(56.0262976873254,31.2267113039017,14.5332689640628));
#58969=CARTESIAN_POINT('Ctrl Pts',(56.0995941099357,31.1914508825021,14.529042387318));
#58970=CARTESIAN_POINT('Ctrl Pts',(56.1710331716213,31.1525871784814,14.5248158105732));
#58971=CARTESIAN_POINT('Ctrl Pts',(56.2423929442211,31.1137666086717,14.5205939248392));
#58972=CARTESIAN_POINT('Ctrl Pts',(56.3118990459886,31.0713509235728,14.5163720391052));
#58973=CARTESIAN_POINT('Ctrl Pts',(56.3791706005989,31.0255465199406,14.5121501533712));
#58974=CARTESIAN_POINT('Ctrl Pts',(56.4463967826319,30.9797730099582,14.5079311151681));
#58975=CARTESIAN_POINT('Ctrl Pts',(56.5113910278071,30.9306155815937,14.5037120769651));
#58976=CARTESIAN_POINT('Ctrl Pts',(56.5737995310625,30.8783251278805,14.4994930387621));
#58977=CARTESIAN_POINT('Ctrl Pts',(56.636187653976,30.8260517503232,14.4952753783431));
#58978=CARTESIAN_POINT('Ctrl Pts',(56.6959913561078,30.7706476774154,14.4910577179242));
#58979=CARTESIAN_POINT('Ctrl Pts',(56.7528892567785,30.712404596896,14.4868400575052));
#58980=CARTESIAN_POINT('Ctrl Pts',(56.8097859734253,30.6541627283931,14.4826224848542));
#58981=CARTESIAN_POINT('Ctrl Pts',(56.8637766850532,30.5930823028627,14.4784049122031));
#58982=CARTESIAN_POINT('Ctrl Pts',(56.9145773112425,30.5294914086962,14.4741873395521));
#58983=CARTESIAN_POINT('Ctrl Pts',(56.9654641743332,30.4657925654337,14.4699626073358));
#58984=CARTESIAN_POINT('Ctrl Pts',(57.0131498256613,30.3995750918099,14.4657378751195));
#58985=CARTESIAN_POINT('Ctrl Pts',(57.057390754508,30.3312000350304,14.4615131429032));
#58986=CARTESIAN_POINT('Ctrl Pts',(57.1016206337188,30.2628420556384,14.4572894658581));
#58987=CARTESIAN_POINT('Ctrl Pts',(57.1424072959396,30.1923279848682,14.453065788813));
#58988=CARTESIAN_POINT('Ctrl Pts',(57.1795531230098,30.1200439428783,14.4488421117679));
#58989=CARTESIAN_POINT('Ctrl Pts',(57.2167663456349,30.0476287522909,14.4446107714916));
#58990=CARTESIAN_POINT('Ctrl Pts',(57.2503253397301,29.9734375972048,14.4403794312154));
#58991=CARTESIAN_POINT('Ctrl Pts',(57.2800802103686,29.8978777668957,14.4361480909392));
#58992=CARTESIAN_POINT('Ctrl Pts',(57.309749564969,29.8225350969098,14.4319289116116));
#58993=CARTESIAN_POINT('Ctrl Pts',(57.3356365663843,29.7458320663347,14.4277097322841));
#58994=CARTESIAN_POINT('Ctrl Pts',(57.3576427833466,29.668184672178,14.4234905529566));
#58995=CARTESIAN_POINT('Ctrl Pts',(57.3797190731995,29.5902900307384,14.4192579387851));
#58996=CARTESIAN_POINT('Ctrl Pts',(57.3979719061172,29.511155282603,14.4150253246137));
#58997=CARTESIAN_POINT('Ctrl Pts',(57.4122655995232,29.4311901290114,14.4107927104422));
#58998=CARTESIAN_POINT('Ctrl Pts',(57.4265389043178,29.3513390382027,14.4065661336974));
#58999=CARTESIAN_POINT('Ctrl Pts',(57.4368642048842,29.2706603479988,14.4023395569526));
#59000=CARTESIAN_POINT('Ctrl Pts',(57.4431558323015,29.1895780290307,14.3981129802078));
#59001=CARTESIAN_POINT('Ctrl Pts',(57.4494404767409,29.1085857020479,14.3938910944737));
#59002=CARTESIAN_POINT('Ctrl Pts',(57.4517003078846,29.0271910972604,14.3896692087397));
#59003=CARTESIAN_POINT('Ctrl Pts',(57.44990110716,28.9458260658984,14.3854473230057));
#59004=CARTESIAN_POINT('Ctrl Pts',(57.4481031199405,28.8645159127267,14.3812282848027));
#59005=CARTESIAN_POINT('Ctrl Pts',(57.4422515483897,28.7832357566018,14.3770092465996));
#59006=CARTESIAN_POINT('Ctrl Pts',(57.4323642361525,28.7024189645048,14.3727902083966));
#59007=CARTESIAN_POINT('Ctrl Pts',(57.4224801527509,28.6216285642256,14.3685725479776));
#59008=CARTESIAN_POINT('Ctrl Pts',(57.4085630023528,28.5413016882235,14.3643548875586));
#59009=CARTESIAN_POINT('Ctrl Pts',(57.3906825000909,28.4618667137601,14.3601372271397));
#59010=CARTESIAN_POINT('Ctrl Pts',(57.3728023699155,28.3824333923088,14.3559196544886));
#59011=CARTESIAN_POINT('Ctrl Pts',(57.3509591550207,28.303892388444,14.3517020818376));
#59012=CARTESIAN_POINT('Ctrl Pts',(57.3252734106166,28.2266606075731,14.3474845091865));
#59013=CARTESIAN_POINT('Ctrl Pts',(57.2995440632262,28.1492977214387,14.3432597769703));
#59014=CARTESIAN_POINT('Ctrl Pts',(57.2699592828855,28.0732489480897,14.339035044754));
#59015=CARTESIAN_POINT('Ctrl Pts',(57.2366893576674,27.99891510485,14.3348103125377));
#59016=CARTESIAN_POINT('Ctrl Pts',(57.203427741962,27.9245998272672,14.3305866354926));
#59017=CARTESIAN_POINT('Ctrl Pts',(57.1664830523105,27.8519990290742,14.3263629584475));
#59018=CARTESIAN_POINT('Ctrl Pts',(57.1260715925566,27.7814886814954,14.3221392814024));
#59019=CARTESIAN_POINT('Ctrl Pts',(57.085586812245,27.7108504034226,14.3179079411261));
#59020=CARTESIAN_POINT('Ctrl Pts',(57.041622943151,27.6423105479224,14.3136766008499));
#59021=CARTESIAN_POINT('Ctrl Pts',(56.9944400268748,27.576216579251,14.3094452605736));
#59022=CARTESIAN_POINT('Ctrl Pts',(56.9473927151562,27.510312565845,14.3052260812461));
#59023=CARTESIAN_POINT('Ctrl Pts',(56.8971451825335,27.4468407043081,14.3010069019186));
#59024=CARTESIAN_POINT('Ctrl Pts',(56.8439927917296,27.3861100303772,14.2967877225911));
#59025=CARTESIAN_POINT('Ctrl Pts',(56.7906711514053,27.3251859759175,14.2925551084196));
#59026=CARTESIAN_POINT('Ctrl Pts',(56.7342277852616,27.266794018506,14.2883224942482));
#59027=CARTESIAN_POINT('Ctrl Pts',(56.67493249533,27.2112710137957,14.2840898800767));
#59028=CARTESIAN_POINT('Ctrl Pts',(56.6157217845621,27.1558272074384,14.2798633033319));
#59029=CARTESIAN_POINT('Ctrl Pts',(56.5536675658583,27.1032445408476,14.2756367265871));
#59030=CARTESIAN_POINT('Ctrl Pts',(56.4890788382501,27.0538256852286,14.2714101498423));
#59031=CARTESIAN_POINT('Ctrl Pts',(56.4245617966502,27.0044616788168,14.2671882641083));
#59032=CARTESIAN_POINT('Ctrl Pts',(56.3575162026761,26.9582547869718,14.2629663783743));
#59033=CARTESIAN_POINT('Ctrl Pts',(56.2882856754156,26.9154688132534,14.2587444926403));
#59034=CARTESIAN_POINT('Ctrl Pts',(56.2191018419988,26.8727116973476,14.2545254544372));
#59035=CARTESIAN_POINT('Ctrl Pts',(56.1477363962833,26.8333711606566,14.2503064162342));
#59036=CARTESIAN_POINT('Ctrl Pts',(56.0745625715205,26.7976681608152,14.2460873780312));
#59037=CARTESIAN_POINT('Ctrl Pts',(56.0014126426609,26.7619768202718,14.2418697176122));
#59038=CARTESIAN_POINT('Ctrl Pts',(55.9264559247337,26.7299208610591,14.2376520571933));
#59039=CARTESIAN_POINT('Ctrl Pts',(55.8500897043675,26.7016750132916,14.2334343967743));
#59040=CARTESIAN_POINT('Ctrl Pts',(55.7737250731538,26.6734297533096,14.2292168241233));
#59041=CARTESIAN_POINT('Ctrl Pts',(55.695951433926,26.6489946071822,14.2249992514722));
#59042=CARTESIAN_POINT('Ctrl Pts',(55.6171841278108,26.6284954137977,14.2207816788212));
#59043=CARTESIAN_POINT('Ctrl Pts',(55.5382831097919,26.607961421887,14.2165569466049));
#59044=CARTESIAN_POINT('Ctrl Pts',(55.4583855019225,26.5913768684574,14.2123322143886));
#59045=CARTESIAN_POINT('Ctrl Pts',(55.3779202248495,26.5788171168518,14.2081074821723));
#59046=CARTESIAN_POINT('Ctrl Pts',(55.2974750448233,26.5662605021759,14.2038838051272));
#59047=CARTESIAN_POINT('Ctrl Pts',(55.2164629449355,26.5577267068027,14.1996601280821));
#59048=CARTESIAN_POINT('Ctrl Pts',(55.1353170553205,26.5532389686487,14.195436451037));
#59049=CARTESIAN_POINT('Ctrl Pts',(55.0540239386093,26.5487430881641,14.1912051107608));
#59050=CARTESIAN_POINT('Ctrl Pts',(54.9725970129515,26.5483079380591,14.1869737704845));
#59051=CARTESIAN_POINT('Ctrl Pts',(54.8914693069877,26.5519045487003,14.1827424302083));
#59052=CARTESIAN_POINT('Ctrl Pts',(54.8105747635226,26.5554908226172,14.1785232508808));
#59053=CARTESIAN_POINT('Ctrl Pts',(54.7299781675619,26.5630855880005,14.1743040715532));
#59054=CARTESIAN_POINT('Ctrl Pts',(54.6500995417821,26.5746093264509,14.1700848922257));
#59055=CARTESIAN_POINT('Ctrl Pts',(54.5699665639614,26.586169759153,14.1658522780542));
#59056=CARTESIAN_POINT('Ctrl Pts',(54.4902581029698,26.6017272499,14.1616196638828));
#59057=CARTESIAN_POINT('Ctrl Pts',(54.4114036022708,26.6212388664306,14.1573870497113));
#59058=CARTESIAN_POINT('Ctrl Pts',(54.3326615801128,26.6407226514724,14.1531604729665));
#59059=CARTESIAN_POINT('Ctrl Pts',(54.2547715461571,26.6641492495008,14.1489338962217));
#59060=CARTESIAN_POINT('Ctrl Pts',(54.1781556079684,26.6914242387814,14.1447073194769));
#59061=CARTESIAN_POINT('Ctrl Pts',(54.1016247045994,26.7186689559821,14.1404854337428));
#59062=CARTESIAN_POINT('Ctrl Pts',(54.0263655226236,26.7497534224188,14.1362635480088));
#59063=CARTESIAN_POINT('Ctrl Pts',(53.9527864136307,26.7845330166027,14.1320416622748));
#59064=CARTESIAN_POINT('Ctrl Pts',(53.879256931465,26.8192891530289,14.1278226240718));
#59065=CARTESIAN_POINT('Ctrl Pts',(53.8074056906419,26.8577352693669,14.1236035858687));
#59066=CARTESIAN_POINT('Ctrl Pts',(53.7376212244823,26.8996785776643,14.1193845476657));
#59067=CARTESIAN_POINT('Ctrl Pts',(53.6678595473853,26.9416081888063,14.1151668872468));
#59068=CARTESIAN_POINT('Ctrl Pts',(53.6001637024346,26.9870324847263,14.1109492268278));
#59069=CARTESIAN_POINT('Ctrl Pts',(53.534896540819,27.035713334593,14.1067315664088));
#59070=CARTESIAN_POINT('Ctrl Pts',(53.4696307373884,27.0843931714296,14.1025139937578));
#59071=CARTESIAN_POINT('Ctrl Pts',(53.4067938884794,27.1363291487885,14.0982964211067));
#59072=CARTESIAN_POINT('Ctrl Pts',(53.3467176629704,27.1912413748468,14.0940788484557));
#59073=CARTESIAN_POINT('Ctrl Pts',(53.2865394547117,27.2462468174773,14.0898541162394));
#59074=CARTESIAN_POINT('Ctrl Pts',(53.229131590767,27.3042383023091,14.0856293840231));
#59075=CARTESIAN_POINT('Ctrl Pts',(53.1747907925554,27.3648970677479,14.0814046518068));
#59076=CARTESIAN_POINT('Ctrl Pts',(53.1204635665281,27.4255406830238,14.0771809747617));
#59077=CARTESIAN_POINT('Ctrl Pts',(53.0692021511873,27.4888498710534,14.0729572977166));
#59078=CARTESIAN_POINT('Ctrl Pts',(53.0212618354783,27.5544739620937,14.0687336206715));
#59079=CARTESIAN_POINT('Ctrl Pts',(52.973234539227,27.6202171182451,14.0645022803952));
#59080=CARTESIAN_POINT('Ctrl Pts',(52.9285406403615,27.6882831816093,14.060270940119));
#59081=CARTESIAN_POINT('Ctrl Pts',(52.8873915795634,27.7582931457465,14.0560395998428));
#59082=CARTESIAN_POINT('Ctrl Pts',(52.8463607819126,27.8281018999764,14.0518204205153));
#59083=CARTESIAN_POINT('Ctrl Pts',(52.8088546108891,27.8998429543094,14.0476012411877));
#59084=CARTESIAN_POINT('Ctrl Pts',(52.7750350251377,27.9731206932477,14.0433820618602));
#59085=CARTESIAN_POINT('Ctrl Pts',(52.7381980024279,28.0529363880121,14.0387864406765));
#59086=CARTESIAN_POINT('Ctrl Pts',(52.70561483382,28.134833249766,14.0341908194928));
#59087=CARTESIAN_POINT('Ctrl Pts',(52.6775044184427,28.2183578033098,14.029595198309));
#59088=CARTESIAN_POINT('Ctrl Pts',(52.6494634471717,28.3016760173919,14.0250109301701));
#59089=CARTESIAN_POINT('Ctrl Pts',(52.625873331223,28.38661360295,14.0204266620313));
#59090=CARTESIAN_POINT('Ctrl Pts',(52.6069054817936,28.4726965987871,14.0158423938924));
#59091=CARTESIAN_POINT('Ctrl Pts',(52.5879312268089,28.5588086653633,14.0112565776189));
#59092=CARTESIAN_POINT('Ctrl Pts',(52.5735825333524,28.646066617719,14.0066707613454));
#59093=CARTESIAN_POINT('Ctrl Pts',(52.5639823990412,28.7339765088965,14.0020849450719));
#59094=CARTESIAN_POINT('Ctrl Pts',(52.55438226473,28.8218864000741,13.9974991287985));
#59095=CARTESIAN_POINT('Ctrl Pts',(52.5495308345984,28.9104479100502,13.992913312525));
#59096=CARTESIAN_POINT('Ctrl Pts',(52.5495001466462,28.9991522304455,13.9883274962515));
#59097=CARTESIAN_POINT('',(52.5495009948596,29.0022081227281,13.1883274961606));
#59098=CARTESIAN_POINT('Ctrl Pts',(52.549500146646,28.9991522312078,13.9883274962121));
#59099=CARTESIAN_POINT('Ctrl Pts',(52.549471270417,29.0826197940372,13.9840124086693));
#59100=CARTESIAN_POINT('Ctrl Pts',(52.5537112764691,29.1660567928118,13.9796973211265));
#59101=CARTESIAN_POINT('Ctrl Pts',(52.5621845880863,29.2490105769558,13.9753822335838));
#59102=CARTESIAN_POINT('Ctrl Pts',(52.5706635607001,29.3320197822995,13.9710642631426));
#59103=CARTESIAN_POINT('Ctrl Pts',(52.5833814218345,29.4145446995457,13.9667462927015));
#59104=CARTESIAN_POINT('Ctrl Pts',(52.6002510244919,29.4961402065424,13.9624283222603));
#59105=CARTESIAN_POINT('Ctrl Pts',(52.6171497683524,29.5778766647692,13.9581028927903));
#59106=CARTESIAN_POINT('Ctrl Pts',(52.6382144862426,29.6586800814982,13.9537774633202));
#59107=CARTESIAN_POINT('Ctrl Pts',(52.6633074022456,29.7381178453335,13.9494520338502));
#59108=CARTESIAN_POINT('Ctrl Pts',(52.6884241060414,29.8176309152461,13.9451225039233));
#59109=CARTESIAN_POINT('Ctrl Pts',(52.7175764641308,29.8957753472051,13.9407929739963));
#59110=CARTESIAN_POINT('Ctrl Pts',(52.7505784092967,29.9721382397982,13.9364634440694));
#59111=CARTESIAN_POINT('Ctrl Pts',(52.7836484656787,30.0486587342979,13.9321249786222));
#59112=CARTESIAN_POINT('Ctrl Pts',(52.8205837872558,30.123389956217,13.9277865131751));
#59113=CARTESIAN_POINT('Ctrl Pts',(52.8611521724728,30.195943234724,13.9234480477279));
#59114=CARTESIAN_POINT('Ctrl Pts',(52.8822502579406,30.2336754555833,13.9211917756502));
#59115=CARTESIAN_POINT('Ctrl Pts',(52.904330240533,30.2708190947748,13.9189355035725));
#59116=CARTESIAN_POINT('Ctrl Pts',(52.9273550057654,30.3073228284835,13.9166792314947));
#59117=CARTESIAN_POINT('Ctrl Pts',(52.9705479117009,30.3758013697613,13.9124466173232));
#59118=CARTESIAN_POINT('Ctrl Pts',(53.017218500924,30.4422643697956,13.9082140031518));
#59119=CARTESIAN_POINT('Ctrl Pts',(53.0671526695653,30.506337096148,13.9039813889803));
#59120=CARTESIAN_POINT('Ctrl Pts',(53.1170156118037,30.5703184287723,13.8997548122355));
#59121=CARTESIAN_POINT('Ctrl Pts',(53.1701326044661,30.6319158960519,13.8955282354907));
#59122=CARTESIAN_POINT('Ctrl Pts',(53.2262455051986,30.6907824349016,13.8913016587459));
#59123=CARTESIAN_POINT('Ctrl Pts',(53.282296127109,30.7495836387098,13.8870797730119));
#59124=CARTESIAN_POINT('Ctrl Pts',(53.3413357311895,30.8056596021463,13.8828578872779));
#59125=CARTESIAN_POINT('Ctrl Pts',(53.4030659291315,30.8586962697814,13.8786360015438));
#59126=CARTESIAN_POINT('Ctrl Pts',(53.4647544919693,30.9116971658289,13.8744169633408));
#59127=CARTESIAN_POINT('Ctrl Pts',(53.5291296930227,30.9616625354226,13.8701979251378));
#59128=CARTESIAN_POINT('Ctrl Pts',(53.5958572239643,31.0083160394985,13.8659788869348));
#59129=CARTESIAN_POINT('Ctrl Pts',(53.662562964127,31.0549543082407,13.8617612265158));
#59130=CARTESIAN_POINT('Ctrl Pts',(53.7316191281786,31.0982825933431,13.8575435660968));
#59131=CARTESIAN_POINT('Ctrl Pts',(53.802660454684,31.1380664777369,13.8533259056779));
#59132=CARTESIAN_POINT('Ctrl Pts',(53.8737003028462,31.1778495342431,13.8491083330268));
#59133=CARTESIAN_POINT('Ctrl Pts',(53.9467248254334,31.2140881107318,13.8448907603758));
#59134=CARTESIAN_POINT('Ctrl Pts',(54.0213433192699,31.2465932767776,13.8406731877248));
#59135=CARTESIAN_POINT('Ctrl Pts',(54.0960884821692,31.2791536221591,13.8364484555085));
#59136=CARTESIAN_POINT('Ctrl Pts',(54.1724326019667,31.3079676903907,13.8322237232922));
#59137=CARTESIAN_POINT('Ctrl Pts',(54.2499637077153,31.3328942989891,13.8279989910759));
#59138=CARTESIAN_POINT('Ctrl Pts',(54.3274754492571,31.3578146819056,13.8237753140308));
#59139=CARTESIAN_POINT('Ctrl Pts',(54.4061731280681,31.3788494469736,13.8195516369857));
#59140=CARTESIAN_POINT('Ctrl Pts',(54.4856325046381,31.395908247349,13.8153279599406));
#59141=CARTESIAN_POINT('Ctrl Pts',(54.5652360483783,31.4129979983697,13.8110966196644));
#59142=CARTESIAN_POINT('Ctrl Pts',(54.6456035919012,31.4260972932283,13.8068652793881));
#59143=CARTESIAN_POINT('Ctrl Pts',(54.726302872835,31.4351673726012,13.8026339391119));
#59144=CARTESIAN_POINT('Ctrl Pts',(54.8067702225712,31.4442113844015,13.7984147597844));
#59145=CARTESIAN_POINT('Ctrl Pts',(54.8875669458817,31.4492493645495,13.7941955804569));
#59146=CARTESIAN_POINT('Ctrl Pts',(54.9682657629379,31.4502945105024,13.7899764011293));
#59147=CARTESIAN_POINT('Ctrl Pts',(55.0492215437141,31.451342984442,13.7857437869579));
#59148=CARTESIAN_POINT('Ctrl Pts',(55.130379891234,31.4483770276291,13.7815111727864));
#59149=CARTESIAN_POINT('Ctrl Pts',(55.2113099121558,31.4413722311489,13.7772785586149));
#59150=CARTESIAN_POINT('Ctrl Pts',(55.2921244940016,31.4343774263531,13.7730519818701));
#59151=CARTESIAN_POINT('Ctrl Pts',(55.3727109371319,31.4233552637546,13.7688254051253));
#59152=CARTESIAN_POINT('Ctrl Pts',(55.4526375833698,31.4083333382489,13.7645988283806));
#59153=CARTESIAN_POINT('Ctrl Pts',(55.5324755202858,31.393328085341,13.7603769426465));
#59154=CARTESIAN_POINT('Ctrl Pts',(55.6116546611306,31.374331975729,13.7561550569125));
#59155=CARTESIAN_POINT('Ctrl Pts',(55.6897491254512,31.3514243330244,13.7519331711785));
#59156=CARTESIAN_POINT('Ctrl Pts',(55.7677909174774,31.3285321408145,13.7477141329755));
#59157=CARTESIAN_POINT('Ctrl Pts',(55.8447490413464,31.3017337856434,13.7434950947724));
#59158=CARTESIAN_POINT('Ctrl Pts',(55.9202096991569,31.2711592545609,13.7392760565694));
#59159=CARTESIAN_POINT('Ctrl Pts',(55.9956457142676,31.2405947080055,13.7350583961504));
#59160=CARTESIAN_POINT('Ctrl Pts',(56.0695848042591,31.2062566088348,13.7308407357315));
#59161=CARTESIAN_POINT('Ctrl Pts',(56.1416314855606,31.1683237307138,13.7266230753125));
#59162=CARTESIAN_POINT('Ctrl Pts',(56.213676667598,31.1303916419617,13.7224055026615));
#59163=CARTESIAN_POINT('Ctrl Pts',(56.2838291087358,31.0888651404542,13.7181879300104));
#59164=CARTESIAN_POINT('Ctrl Pts',(56.351717630243,31.043969103996,13.7139703573594));
#59165=CARTESIAN_POINT('Ctrl Pts',(56.419721396309,30.9989968540072,13.7097456251431));
#59166=CARTESIAN_POINT('Ctrl Pts',(56.4854531640172,30.9506438823338,13.7055208929268));
#59167=CARTESIAN_POINT('Ctrl Pts',(56.5485702286235,30.8991789007413,13.7012961607105));
#59168=CARTESIAN_POINT('Ctrl Pts',(56.6116715290809,30.8477267730678,13.6970724836654));
#59169=CARTESIAN_POINT('Ctrl Pts',(56.6721591004684,30.7931645178053,13.6928488066203));
#59170=CARTESIAN_POINT('Ctrl Pts',(56.7297262012426,30.7357988128625,13.6886251295752));
#59171=CARTESIAN_POINT('Ctrl Pts',(56.7873977489227,30.6783290264165,13.6843937892989));
#59172=CARTESIAN_POINT('Ctrl Pts',(56.8421379234027,30.6180459701271,13.6801624490227));
#59173=CARTESIAN_POINT('Ctrl Pts',(56.8936788884007,30.5552911359696,13.6759311087465));
#59174=CARTESIAN_POINT('Ctrl Pts',(56.9450717237301,30.492716660344,13.6717119294189));
#59175=CARTESIAN_POINT('Ctrl Pts',(56.9932835098872,30.4276850109937,13.6674927500914));
#59176=CARTESIAN_POINT('Ctrl Pts',(57.0380927057488,30.3605617857244,13.6632735707639));
#59177=CARTESIAN_POINT('Ctrl Pts',(57.083044584466,30.2932248245629,13.6590409565924));
#59178=CARTESIAN_POINT('Ctrl Pts',(57.1247393348929,30.223532485968,13.6548083424209));
#59179=CARTESIAN_POINT('Ctrl Pts',(57.1629219035332,30.1518329259126,13.6505757282495));
#59180=CARTESIAN_POINT('Ctrl Pts',(57.2010500083245,30.0802356385473,13.6463491515047));
#59181=CARTESIAN_POINT('Ctrl Pts',(57.2356756648905,30.0066372228569,13.6421225747599));
#59182=CARTESIAN_POINT('Ctrl Pts',(57.2665870254661,29.9314147872933,13.6378959980151));
#59183=CARTESIAN_POINT('Ctrl Pts',(57.297464078011,29.8562758399226,13.6336741122811));
#59184=CARTESIAN_POINT('Ctrl Pts',(57.324634850161,29.7795168817087,13.629452226547));
#59185=CARTESIAN_POINT('Ctrl Pts',(57.3479340309009,29.7015383357576,13.625230340813));
#59186=CARTESIAN_POINT('Ctrl Pts',(57.3712174970659,29.6236123839176,13.62101130261));
#59187=CARTESIAN_POINT('Ctrl Pts',(57.3906344253783,29.5444689220006,13.616792264407));
#59188=CARTESIAN_POINT('Ctrl Pts',(57.4060685803433,29.4645258191797,13.6125732262039));
#59189=CARTESIAN_POINT('Ctrl Pts',(57.4214976950761,29.3846088228616,13.608355565785));
#59190=CARTESIAN_POINT('Ctrl Pts',(57.4329465314363,29.3038931600108,13.604137905366));
#59191=CARTESIAN_POINT('Ctrl Pts',(57.4403497477094,29.2228078967508,13.599920244947));
#59192=CARTESIAN_POINT('Ctrl Pts',(57.4477528099245,29.1417243208446,13.595702672296));
#59193=CARTESIAN_POINT('Ctrl Pts',(57.4511103783708,29.0602716225518,13.5914850996449));
#59194=CARTESIAN_POINT('Ctrl Pts',(57.4504090162236,28.978883579614,13.5872675269939));
#59195=CARTESIAN_POINT('Ctrl Pts',(57.449706463475,28.8973573759256,13.5830427947776));
#59196=CARTESIAN_POINT('Ctrl Pts',(57.4449311983527,28.8158965141655,13.5788180625613));
#59197=CARTESIAN_POINT('Ctrl Pts',(57.4361220543256,28.7349347506204,13.574593330345));
#59198=CARTESIAN_POINT('Ctrl Pts',(57.4273151104745,28.6539932081249,13.5703696532999));
#59199=CARTESIAN_POINT('Ctrl Pts',(57.4144763969283,28.5735509715438,13.5661459762548));
#59200=CARTESIAN_POINT('Ctrl Pts',(57.39769617251,28.4940322991229,13.5619222992097));
#59201=CARTESIAN_POINT('Ctrl Pts',(57.3808855028808,28.414369351948,13.5576909589334));
#59202=CARTESIAN_POINT('Ctrl Pts',(57.360119149602,28.3356337681933,13.5534596186572));
#59203=CARTESIAN_POINT('Ctrl Pts',(57.3355377544693,28.2582361241957,13.549228278381));
#59204=CARTESIAN_POINT('Ctrl Pts',(57.3110270067123,28.1810609224311,13.5450090990535));
#59205=CARTESIAN_POINT('Ctrl Pts',(57.2827233539127,28.1052163776052,13.5407899197259));
#59206=CARTESIAN_POINT('Ctrl Pts',(57.2508128615668,28.0310873557408,13.5365707403984));
#59207=CARTESIAN_POINT('Ctrl Pts',(57.2188007588242,27.9567222899056,13.5323381262269));
#59208=CARTESIAN_POINT('Ctrl Pts',(57.1830397228031,27.8838071160754,13.5281055120555));
#59209=CARTESIAN_POINT('Ctrl Pts',(57.1436829441875,27.8127453159495,13.523872897884));
#59210=CARTESIAN_POINT('Ctrl Pts',(57.1043823043211,27.7417848788093,13.5196463211392));
#59211=CARTESIAN_POINT('Ctrl Pts',(57.0614963318947,27.6726729677245,13.5154197443944));
#59212=CARTESIAN_POINT('Ctrl Pts',(57.0152260248969,27.6057925840901,13.5111931676496));
#59213=CARTESIAN_POINT('Ctrl Pts',(56.9690070725819,27.538986429937,13.5069712819156));
#59214=CARTESIAN_POINT('Ctrl Pts',(56.9194115122677,27.4744072620696,13.5027493961816));
#59215=CARTESIAN_POINT('Ctrl Pts',(56.8666852335074,27.4124117381999,13.4985275104476));
#59216=CARTESIAN_POINT('Ctrl Pts',(56.8139945169869,27.3504580283884,13.4943084722445));
#59217=CARTESIAN_POINT('Ctrl Pts',(56.7581775759748,27.291084854603,13.4900894340415));
#59218=CARTESIAN_POINT('Ctrl Pts',(56.6995216509783,27.2346172064235,13.4858703958385));
#59219=CARTESIAN_POINT('Ctrl Pts',(56.6408848808684,27.1781679985193,13.4816527354195));
#59220=CARTESIAN_POINT('Ctrl Pts',(56.5794113023675,27.1246227538218,13.4774350750006));
#59221=CARTESIAN_POINT('Ctrl Pts',(56.5154252548821,27.074269866553,13.4732174145816));
#59222=CARTESIAN_POINT('Ctrl Pts',(56.4514405389221,27.0239180271089,13.4689998419305));
#59223=CARTESIAN_POINT('Ctrl Pts',(56.3849438237229,26.9767586993703,13.4647822692795));
#59224=CARTESIAN_POINT('Ctrl Pts',(56.316291657979,26.9330393034373,13.4605646966285));
#59225=CARTESIAN_POINT('Ctrl Pts',(56.2475229513475,26.8892456913867,13.4563399644122));
#59226=CARTESIAN_POINT('Ctrl Pts',(56.1765918672738,26.8489039454176,13.4521152321959));
#59227=CARTESIAN_POINT('Ctrl Pts',(56.1038833924458,26.8122176283089,13.4478904999796));
#59228=CARTESIAN_POINT('Ctrl Pts',(56.0311930773219,26.7755404739926,13.4436668229345));
#59229=CARTESIAN_POINT('Ctrl Pts',(55.9567266939224,26.7425170923501,13.4394431458894));
#59230=CARTESIAN_POINT('Ctrl Pts',(55.8808892577429,26.7133027385347,13.4352194688443));
#59231=CARTESIAN_POINT('Ctrl Pts',(55.8049142258629,26.6840353796378,13.430988128568));
#59232=CARTESIAN_POINT('Ctrl Pts',(55.7275636124464,26.6585910053715,13.4267567882918));
#59233=CARTESIAN_POINT('Ctrl Pts',(55.6492583847897,26.6370751599384,13.4225254480155));
#59234=CARTESIAN_POINT('Ctrl Pts',(55.5711782077782,26.6156211514354,13.418306268688));
#59235=CARTESIAN_POINT('Ctrl Pts',(55.4921493588124,26.5980731380775,13.4140870893605));
#59236=CARTESIAN_POINT('Ctrl Pts',(55.4125959674281,26.5844845648057,13.409867910033));
#59237=CARTESIAN_POINT('Ctrl Pts',(55.3327892596243,26.57085272237,13.4056352958615));
#59238=CARTESIAN_POINT('Ctrl Pts',(55.2521578355119,26.5611549021207,13.40140268169));
#59239=CARTESIAN_POINT('Ctrl Pts',(55.1711235428509,26.5554822596099,13.3971700675186));
#59240=CARTESIAN_POINT('Ctrl Pts',(55.0902048379992,26.5498177085909,13.3929434907738));
#59241=CARTESIAN_POINT('Ctrl Pts',(55.0088848655,26.5481669640471,13.3887169140289));
#59242=CARTESIAN_POINT('Ctrl Pts',(54.9275943200526,26.550569930063,13.3844903372841));
#59243=CARTESIAN_POINT('Ctrl Pts',(54.8463939976978,26.5529702290649,13.3802684515501));
#59244=CARTESIAN_POINT('Ctrl Pts',(54.7652234995034,26.5594152851691,13.3760465658161));
#59245=CARTESIAN_POINT('Ctrl Pts',(54.6845158614266,26.5698930047612,13.3718246800821));
#59246=CARTESIAN_POINT('Ctrl Pts',(54.6038626581489,26.5803636574564,13.367605641879));
#59247=CARTESIAN_POINT('Ctrl Pts',(54.5236721544562,26.5948615120148,13.363386603676));
#59248=CARTESIAN_POINT('Ctrl Pts',(54.4443733337705,26.6133225484421,13.359167565473));
#59249=CARTESIAN_POINT('Ctrl Pts',(54.3651004091885,26.6317775561681,13.354949905054));
#59250=CARTESIAN_POINT('Ctrl Pts',(54.2867190414284,26.6541930702489,13.350732244635));
#59251=CARTESIAN_POINT('Ctrl Pts',(54.2096477134736,26.6804540286551,13.3465145842161));
#59252=CARTESIAN_POINT('Ctrl Pts',(54.132577989344,26.7067144405806,13.342297011565));
#59253=CARTESIAN_POINT('Ctrl Pts',(54.0568186901607,26.7368199867859,13.338079438914));
#59254=CARTESIAN_POINT('Ctrl Pts',(53.982771463542,26.770606280933,13.3338618662629));
#59255=CARTESIAN_POINT('Ctrl Pts',(53.9085985376188,26.8044499292022,13.3296371340466));
#59256=CARTESIAN_POINT('Ctrl Pts',(53.8361439240233,26.8419866328989,13.3254124018303));
#59257=CARTESIAN_POINT('Ctrl Pts',(53.7657879634133,26.8830042752182,13.3211876696141));
#59258=CARTESIAN_POINT('Ctrl Pts',(53.695449574942,26.9240116729513,13.3169639925689));
#59259=CARTESIAN_POINT('Ctrl Pts',(53.6272091701636,26.968497998349,13.3127403155238));
#59260=CARTESIAN_POINT('Ctrl Pts',(53.5614174717795,27.0162080352268,13.3085166384787));
#59261=CARTESIAN_POINT('Ctrl Pts',(53.4955064041858,27.0640046348403,13.3042852982025));
#59262=CARTESIAN_POINT('Ctrl Pts',(53.4320532848467,27.1150363428642,13.3000539579262));
#59263=CARTESIAN_POINT('Ctrl Pts',(53.3713758218373,27.1690074996593,13.29582261765));
#59264=CARTESIAN_POINT('Ctrl Pts',(53.3108727469579,27.2228235423703,13.2916034383225));
#59265=CARTESIAN_POINT('Ctrl Pts',(53.2531296615676,27.2795617819552,13.287384258995));
#59266=CARTESIAN_POINT('Ctrl Pts',(53.1984222930922,27.3388955433288,13.2831650796675));
#59267=CARTESIAN_POINT('Ctrl Pts',(53.1441786834718,27.397726327535,13.2789816666697));
#59268=CARTESIAN_POINT('Ctrl Pts',(53.0927073678689,27.4593391010681,13.2747982536718));
#59269=CARTESIAN_POINT('Ctrl Pts',(53.0443115060476,27.5234388720333,13.2706148406739));
#59270=CARTESIAN_POINT('Ctrl Pts',(52.9959787824364,27.5874550171542,13.2664368854404));
#59271=CARTESIAN_POINT('Ctrl Pts',(52.9507138383018,27.6539513481805,13.2622589302069));
#59272=CARTESIAN_POINT('Ctrl Pts',(52.9087821854626,27.7225970478501,13.2580809749733));
#59273=CARTESIAN_POINT('Ctrl Pts',(52.8668916944516,27.7911753620887,13.2539071209918));
#59274=CARTESIAN_POINT('Ctrl Pts',(52.8283282490237,27.8618984545656,13.2497332670103));
#59275=CARTESIAN_POINT('Ctrl Pts',(52.7933153586562,27.9344047937151,13.2455594130288));
#59276=CARTESIAN_POINT('Ctrl Pts',(52.7583255353572,28.006863364495,13.241388308851));
#59277=CARTESIAN_POINT('Ctrl Pts',(52.7268818296577,28.0811024219658,13.2372172046732));
#59278=CARTESIAN_POINT('Ctrl Pts',(52.6991621075189,28.1567353662561,13.2330461004954));
#59279=CARTESIAN_POINT('Ctrl Pts',(52.6714438038877,28.2323644401648,13.2288752097664));
#59280=CARTESIAN_POINT('Ctrl Pts',(52.6474492835787,28.3093868176467,13.2247043190374));
#59281=CARTESIAN_POINT('Ctrl Pts',(52.6273080105467,28.3873965612371,13.2205334283085));
#59282=CARTESIAN_POINT('Ctrl Pts',(52.6071677410357,28.4654024180612,13.2163627453904));
#59283=CARTESIAN_POINT('Ctrl Pts',(52.5908804484917,28.5443950799622,13.2121920624724));
#59284=CARTESIAN_POINT('Ctrl Pts',(52.5785249940676,28.6239560588911,13.2080213795544));
#59285=CARTESIAN_POINT('Ctrl Pts',(52.5661601393466,28.7035775695332,13.2038475234906));
#59286=CARTESIAN_POINT('Ctrl Pts',(52.5577331587781,28.7837677880482,13.1996736674268));
#59287=CARTESIAN_POINT('Ctrl Pts',(52.5532711845619,28.8641016788011,13.195499811363));
#59288=CARTESIAN_POINT('Ctrl Pts',(52.550715379667,28.9101166805143,13.193109039646));
#59289=CARTESIAN_POINT('Ctrl Pts',(52.5494595182279,28.9561787562162,13.1907182679291));
#59290=CARTESIAN_POINT('Ctrl Pts',(52.5495009948587,29.0022081217367,13.1883274962121));
#59291=CARTESIAN_POINT('',(52.5495001658419,28.9990984507376,12.3883274961653));
#59292=CARTESIAN_POINT('Ctrl Pts',(52.5495009948596,29.0022081227281,13.1883274961606));
#59293=CARTESIAN_POINT('Ctrl Pts',(52.5495956779836,29.107284212101,13.1828698293045));
#59294=CARTESIAN_POINT('Ctrl Pts',(52.5564525380247,29.2120617946342,13.1774121624485));
#59295=CARTESIAN_POINT('Ctrl Pts',(52.5699345169715,29.3158037336601,13.1719544955924));
#59296=CARTESIAN_POINT('Ctrl Pts',(52.582691258624,29.4139650733196,13.1667904134956));
#59297=CARTESIAN_POINT('Ctrl Pts',(52.6013790218718,29.511199695907,13.1616263313989));
#59298=CARTESIAN_POINT('Ctrl Pts',(52.6258433201928,29.6069022241902,13.1564622493021));
#59299=CARTESIAN_POINT('Ctrl Pts',(52.6458948867304,29.6853424716276,13.1522296351306));
#59300=CARTESIAN_POINT('Ctrl Pts',(52.6698753221035,29.7629337919622,13.1479970209591));
#59301=CARTESIAN_POINT('Ctrl Pts',(52.6976960801471,29.8392537820171,13.1437644067877));
#59302=CARTESIAN_POINT('Ctrl Pts',(52.7254771544916,29.9154649087722,13.1395378300429));
#59303=CARTESIAN_POINT('Ctrl Pts',(52.7570875139937,29.9904078741316,13.1353112532981));
#59304=CARTESIAN_POINT('Ctrl Pts',(52.7923882008275,30.0636730673259,13.1310846765533));
#59305=CARTESIAN_POINT('Ctrl Pts',(52.8276497079867,30.1368569446398,13.1268627908193));
#59306=CARTESIAN_POINT('Ctrl Pts',(52.8665932034325,30.2083663334484,13.1226409050853));
#59307=CARTESIAN_POINT('Ctrl Pts',(52.9090312856088,30.2778106610282,13.1184190193512));
#59308=CARTESIAN_POINT('Ctrl Pts',(52.9514407446146,30.3472081505623,13.1141999811482));
#59309=CARTESIAN_POINT('Ctrl Pts',(52.9973398675489,30.4145429497611,13.1099809429452));
#59310=CARTESIAN_POINT('Ctrl Pts',(53.0464954781693,30.4794493344441,13.1057619047422));
#59311=CARTESIAN_POINT('Ctrl Pts',(53.0956350363595,30.5443345230683,13.1015442443232));
#59312=CARTESIAN_POINT('Ctrl Pts',(53.1480286900404,30.6067925020412,13.0973265839043));
#59313=CARTESIAN_POINT('Ctrl Pts',(53.2034009219129,30.6664879245337,13.0931089234853));
#59314=CARTESIAN_POINT('Ctrl Pts',(53.2587720015101,30.726182104787,13.0888913508343));
#59315=CARTESIAN_POINT('Ctrl Pts',(53.3171212192789,30.7831135030728,13.0846737781832));
#59316=CARTESIAN_POINT('Ctrl Pts',(53.3781348656214,30.8369822361381,13.0804562055322));
#59317=CARTESIAN_POINT('Ctrl Pts',(53.4392520860381,30.8909424143881,13.0762314733159));
#59318=CARTESIAN_POINT('Ctrl Pts',(53.5030424344527,30.9418292162612,13.0720067410996));
#59319=CARTESIAN_POINT('Ctrl Pts',(53.5691572857285,30.9893816569518,13.0677820088833));
#59320=CARTESIAN_POINT('Ctrl Pts',(53.6352556241266,31.0369222209214,13.0635583318382));
#59321=CARTESIAN_POINT('Ctrl Pts',(53.7036769013223,31.0811298539567,13.0593346547931));
#59322=CARTESIAN_POINT('Ctrl Pts',(53.7740451909773,31.1217881742139,13.055110977748));
#59323=CARTESIAN_POINT('Ctrl Pts',(53.8445411533833,31.1625202629204,13.0508796374718));
#59324=CARTESIAN_POINT('Ctrl Pts',(53.9169907734289,31.1996899566632,13.0466482971955));
#59325=CARTESIAN_POINT('Ctrl Pts',(53.9909946325807,31.2331274971481,13.0424169569193));
#59326=CARTESIAN_POINT('Ctrl Pts',(54.0647858032994,31.2664689375354,13.0381977775917));
#59327=CARTESIAN_POINT('Ctrl Pts',(54.140121837128,31.2960995593441,13.0339785982642));
#59328=CARTESIAN_POINT('Ctrl Pts',(54.2165920855353,31.3219005770175,13.0297594189366));
#59329=CARTESIAN_POINT('Ctrl Pts',(54.2933058329201,31.3477837511053,13.0255268047651));
#59330=CARTESIAN_POINT('Ctrl Pts',(54.3714463581967,31.3699091342994,13.0212941905937));
#59331=CARTESIAN_POINT('Ctrl Pts',(54.4506111343204,31.3881210447269,13.0170615764222));
#59332=CARTESIAN_POINT('Ctrl Pts',(54.5296629893242,31.4063069775741,13.0128349996774));
#59333=CARTESIAN_POINT('Ctrl Pts',(54.6097357444841,31.4205904213417,13.0086084229326));
#59334=CARTESIAN_POINT('Ctrl Pts',(54.6904101592007,31.4308649449268,13.0043818461878));
#59335=CARTESIAN_POINT('Ctrl Pts',(54.7709950346588,31.4411280649804,13.0001599604538));
#59336=CARTESIAN_POINT('Ctrl Pts',(54.8521797843075,31.4473910474798,12.9959380747198));
#59337=CARTESIAN_POINT('Ctrl Pts',(54.9335347643349,31.4495984614724,12.9917161889857));
#59338=CARTESIAN_POINT('Ctrl Pts',(55.0148348729512,31.4518043866327,12.9874971507827));
#59339=CARTESIAN_POINT('Ctrl Pts',(55.0963045207342,31.4499601633729,12.9832781125797));
#59340=CARTESIAN_POINT('Ctrl Pts',(55.1775099876806,31.4440622852689,12.9790590743767));
#59341=CARTESIAN_POINT('Ctrl Pts',(55.2586889358821,31.4381663331968,12.9748414139577));
#59342=CARTESIAN_POINT('Ctrl Pts',(55.3396034116048,31.4282193888435,12.9706237535387));
#59343=CARTESIAN_POINT('Ctrl Pts',(55.4198221256285,31.4142699999861,12.9664060931198));
#59344=CARTESIAN_POINT('Ctrl Pts',(55.5000391703312,31.4003209014101,12.9621885204687));
#59345=CARTESIAN_POINT('Ctrl Pts',(55.5795600246435,31.3823696046746,12.9579709478177));
#59346=CARTESIAN_POINT('Ctrl Pts',(55.6579623551695,31.3605160006193,12.9537533751666));
#59347=CARTESIAN_POINT('Ctrl Pts',(55.7364977780323,31.3386252988501,12.9495286429503));
#59348=CARTESIAN_POINT('Ctrl Pts',(55.8139104282942,31.3128191613027,12.9453039107341));
#59349=CARTESIAN_POINT('Ctrl Pts',(55.8897915935107,31.283247943198,12.9410791785178));
#59350=CARTESIAN_POINT('Ctrl Pts',(55.9656538066105,31.2536841108151,12.9368555014727));
#59351=CARTESIAN_POINT('Ctrl Pts',(56.0399848829157,31.220357288479,12.9326318244276));
#59352=CARTESIAN_POINT('Ctrl Pts',(56.1123986612753,31.183465014236,12.9284081473824));
#59353=CARTESIAN_POINT('Ctrl Pts',(56.1849438236198,31.1465058044719,12.9241768071062));
#59354=CARTESIAN_POINT('Ctrl Pts',(56.2555643319928,31.1059684467035,12.91994546683));
#59355=CARTESIAN_POINT('Ctrl Pts',(56.3239003450831,31.0620955667206,12.9157141265537));
#59356=CARTESIAN_POINT('Ctrl Pts',(56.3920399592316,31.0183487781911,12.9114949472262));
#59357=CARTESIAN_POINT('Ctrl Pts',(56.4579078698647,30.9712859468861,12.9072757678987));
#59358=CARTESIAN_POINT('Ctrl Pts',(56.5211808792693,30.9211868682004,12.9030565885712));
#59359=CARTESIAN_POINT('Ctrl Pts',(56.5846553645874,30.870928262447,12.8988239743997));
#59360=CARTESIAN_POINT('Ctrl Pts',(56.6457544591394,30.8174270950118,12.8945913602282));
#59361=CARTESIAN_POINT('Ctrl Pts',(56.7041284369947,30.7609362623974,12.8903587460568));
#59362=CARTESIAN_POINT('Ctrl Pts',(56.7624191498517,30.7045260086514,12.886132169312));
#59363=CARTESIAN_POINT('Ctrl Pts',(56.8179921352872,30.6451348798985,12.8819055925672));
#59364=CARTESIAN_POINT('Ctrl Pts',(56.8705298812866,30.5830566045514,12.8776790158224));
#59365=CARTESIAN_POINT('Ctrl Pts',(56.9230093164717,30.5210472289015,12.8734571300884));
#59366=CARTESIAN_POINT('Ctrl Pts',(56.9724599073562,30.4563569855376,12.8692352443543));
#59367=CARTESIAN_POINT('Ctrl Pts',(57.0186012586211,30.3893160938725,12.8650133586203));
#59368=CARTESIAN_POINT('Ctrl Pts',(57.0647114889755,30.3223204192099,12.8607943204173));
#59369=CARTESIAN_POINT('Ctrl Pts',(57.1075166499194,30.2529776267519,12.8565752822142));
#59370=CARTESIAN_POINT('Ctrl Pts',(57.1467776826562,30.1816496228786,12.8523562440112));
#59371=CARTESIAN_POINT('Ctrl Pts',(57.1860258941712,30.1103449121308,12.8481385835922));
#59372=CARTESIAN_POINT('Ctrl Pts',(57.221732052134,30.0370566841063,12.8439209231733));
#59373=CARTESIAN_POINT('Ctrl Pts',(57.2537020854455,29.9621731445319,12.8397032627543));
#59374=CARTESIAN_POINT('Ctrl Pts',(57.2856714534728,29.8872911632557,12.8354856901033));
#59375=CARTESIAN_POINT('Ctrl Pts',(57.3139046701088,29.8108143641371,12.8312681174522));
#59376=CARTESIAN_POINT('Ctrl Pts',(57.3382556076688,29.7331513917367,12.8270505448012));
#59377=CARTESIAN_POINT('Ctrl Pts',(57.3626478823059,29.6553565821013,12.8228258125849));
#59378=CARTESIAN_POINT('Ctrl Pts',(57.3831445523268,29.5763720160536,12.8186010803686));
#59379=CARTESIAN_POINT('Ctrl Pts',(57.3996492360996,29.4966223854064,12.8143763481523));
#59380=CARTESIAN_POINT('Ctrl Pts',(57.4161497976545,29.4168926730656,12.8101526711072));
#59381=CARTESIAN_POINT('Ctrl Pts',(57.4286603162007,29.3363987421303,12.8059289940621));
#59382=CARTESIAN_POINT('Ctrl Pts',(57.4371362651929,29.2555720541874,12.8017053170169));
#59383=CARTESIAN_POINT('Ctrl Pts',(57.4456275925285,29.1745987182919,12.7974739767407));
#59384=CARTESIAN_POINT('Ctrl Pts',(57.450069695877,29.0932918840432,12.7932426364645));
#59385=CARTESIAN_POINT('Ctrl Pts',(57.4504701979716,29.0120854810866,12.7890112961882));
#59386=CARTESIAN_POINT('Ctrl Pts',(57.4508695490159,28.9311124668059,12.7847921168607));
#59387=CARTESIAN_POINT('Ctrl Pts',(57.4472506024997,28.8502397583826,12.7805729375332));
#59388=CARTESIAN_POINT('Ctrl Pts',(57.4396721087627,28.7698907830503,12.7763537582057));
#59389=CARTESIAN_POINT('Ctrl Pts',(57.4320694833468,28.6892859579748,12.7721211440342));
#59390=CARTESIAN_POINT('Ctrl Pts',(57.4204537507425,28.608908417405,12.7678885298628));
#59391=CARTESIAN_POINT('Ctrl Pts',(57.4048466558375,28.5291891973339,12.7636559156913));
#59392=CARTESIAN_POINT('Ctrl Pts',(57.389261822988,28.449583689245,12.7594293389465));
#59393=CARTESIAN_POINT('Ctrl Pts',(57.3696970239834,28.3706350887212,12.7552027622017));
#59394=CARTESIAN_POINT('Ctrl Pts',(57.3462257918297,28.2927696388353,12.7509761854569));
#59395=CARTESIAN_POINT('Ctrl Pts',(57.3227806100257,28.2149906105821,12.7467542997229));
#59396=CARTESIAN_POINT('Ctrl Pts',(57.2954377434726,28.138292786793,12.7425324139889));
#59397=CARTESIAN_POINT('Ctrl Pts',(57.2643215411068,28.0630911418501,12.7383105282549));
#59398=CARTESIAN_POINT('Ctrl Pts',(57.2332263256545,27.9879402180846,12.7340914900518));
#59399=CARTESIAN_POINT('Ctrl Pts',(57.1983630061319,27.9142838970988,12.7298724518488));
#59400=CARTESIAN_POINT('Ctrl Pts',(57.159905014939,27.8425197295671,12.7256534136458));
#59401=CARTESIAN_POINT('Ctrl Pts',(57.121459582724,27.7707789975962,12.7214357532268));
#59402=CARTESIAN_POINT('Ctrl Pts',(57.0794220293684,27.7009296010969,12.7172180928079));
#59403=CARTESIAN_POINT('Ctrl Pts',(57.0340123391669,27.6333456713138,12.7130004323889));
#59404=CARTESIAN_POINT('Ctrl Pts',(56.9886035939239,27.5657631479268,12.7087828597379));
#59405=CARTESIAN_POINT('Ctrl Pts',(56.9398231114118,27.5004463824609,12.7045652870868));
#59406=CARTESIAN_POINT('Ctrl Pts',(56.8879341209679,27.4377404169328,12.7003477144358));
#59407=CARTESIAN_POINT('Ctrl Pts',(56.8359570460632,27.3749280045244,12.6961229822195));
#59408=CARTESIAN_POINT('Ctrl Pts',(56.7808612031716,27.3147356191941,12.6918982500032));
#59409=CARTESIAN_POINT('Ctrl Pts',(56.7229503642611,27.2574753108514,12.6876735177869));
#59410=CARTESIAN_POINT('Ctrl Pts',(56.66505398919,27.2002293038712,12.6834498407418));
#59411=CARTESIAN_POINT('Ctrl Pts',(56.6043443856516,27.145914204406,12.6792261636967));
#59412=CARTESIAN_POINT('Ctrl Pts',(56.5411592342224,27.0948022504813,12.6750024866516));
#59413=CARTESIAN_POINT('Ctrl Pts',(56.4778594427736,27.0435975615506,12.6707711463753));
#59414=CARTESIAN_POINT('Ctrl Pts',(56.4120755036895,26.9956079070793,12.6665398060991));
#59415=CARTESIAN_POINT('Ctrl Pts',(56.3441755579257,26.9510631245753,12.6623084658229));
#59416=CARTESIAN_POINT('Ctrl Pts',(56.2764707578379,26.9066463645844,12.6580892864954));
#59417=CARTESIAN_POINT('Ctrl Pts',(56.2066625324019,26.8656548605482,12.6538701071678));
#59418=CARTESIAN_POINT('Ctrl Pts',(56.1351380467958,26.8282698453268,12.6496509278403));
#59419=CARTESIAN_POINT('Ctrl Pts',(56.0633858106653,26.7907657875603,12.6454183136688));
#59420=CARTESIAN_POINT('Ctrl Pts',(55.9896394877231,26.7567517592118,12.6411856994974));
#59421=CARTESIAN_POINT('Ctrl Pts',(55.9142724797684,26.7264441764632,12.6369530853259));
#59422=CARTESIAN_POINT('Ctrl Pts',(55.8390129757738,26.6961798246356,12.6327265085811));
#59423=CARTESIAN_POINT('Ctrl Pts',(55.7621378056333,26.6696115898312,12.6284999318363));
#59424=CARTESIAN_POINT('Ctrl Pts',(55.6840445442169,26.646909837782,12.6242733550915));
#59425=CARTESIAN_POINT('Ctrl Pts',(55.6060379572776,26.6242332820488,12.6200514693575));
#59426=CARTESIAN_POINT('Ctrl Pts',(55.5268164091989,26.6054148111937,12.6158295836235));
#59427=CARTESIAN_POINT('Ctrl Pts',(55.4467956866222,26.59057603058,12.6116076978894));
#59428=CARTESIAN_POINT('Ctrl Pts',(55.3668289355414,26.5757472582636,12.6073886596864));
#59429=CARTESIAN_POINT('Ctrl Pts',(55.2860645360832,26.5648929296592,12.6031696214834));
#59430=CARTESIAN_POINT('Ctrl Pts',(55.2049303805208,26.5580839922021,12.5989505832803));
#59431=CARTESIAN_POINT('Ctrl Pts',(55.1238227204157,26.5512772782957,12.5947329228614));
#59432=CARTESIAN_POINT('Ctrl Pts',(55.0423460065726,26.5485133707775,12.5905152624424));
#59433=CARTESIAN_POINT('Ctrl Pts',(54.9609338293452,26.549811418623,12.5862976020234));
#59434=CARTESIAN_POINT('Ctrl Pts',(54.8795233462743,26.5511094394565,12.5820800293724));
#59435=CARTESIAN_POINT('Ctrl Pts',(54.7981778616191,26.5564692390106,12.5778624567213));
#59436=CARTESIAN_POINT('Ctrl Pts',(54.7173301075911,26.5658578550287,12.5736448840703));
#59437=CARTESIAN_POINT('Ctrl Pts',(54.6363451099832,26.5752624087471,12.569420151854));
#59438=CARTESIAN_POINT('Ctrl Pts',(54.5558599973781,26.5887094085851,12.5651954196377));
#59439=CARTESIAN_POINT('Ctrl Pts',(54.4763018988166,26.6061139231749,12.5609706874214));
#59440=CARTESIAN_POINT('Ctrl Pts',(54.3967636707247,26.6235140908047,12.5567470103763));
#59441=CARTESIAN_POINT('Ctrl Pts',(54.3181524379497,26.6448696538575,12.5525233333312));
#59442=CARTESIAN_POINT('Ctrl Pts',(54.2408803941934,26.6700455639476,12.5482996562861));
#59443=CARTESIAN_POINT('Ctrl Pts',(54.1634681518555,26.6952671519662,12.5440683160098));
#59444=CARTESIAN_POINT('Ctrl Pts',(54.0874003895536,26.7243227730418,12.5398369757336));
#59445=CARTESIAN_POINT('Ctrl Pts',(54.0130703170206,26.7570287449782,12.5356056354573));
#59446=CARTESIAN_POINT('Ctrl Pts',(53.9389538704648,26.7896407193577,12.5313864561298));
#59447=CARTESIAN_POINT('Ctrl Pts',(53.8665655085587,26.8258818120867,12.5271672768023));
#59448=CARTESIAN_POINT('Ctrl Pts',(53.7962680270324,26.8655259225619,12.5229480974748));
#59449=CARTESIAN_POINT('Ctrl Pts',(53.7257467020468,26.9052962690647,12.5187154833033));
#59450=CARTESIAN_POINT('Ctrl Pts',(53.6570673193136,26.9486392807201,12.5144828691319));
#59451=CARTESIAN_POINT('Ctrl Pts',(53.5906146944258,26.9953595558226,12.5102502549604));
#59452=CARTESIAN_POINT('Ctrl Pts',(53.5242568579679,27.0420131888395,12.5060236782156));
#59453=CARTESIAN_POINT('Ctrl Pts',(53.46011984776,27.0920342524662,12.5017971014708));
#59454=CARTESIAN_POINT('Ctrl Pts',(53.3985630109559,27.1451819981138,12.497570524726));
#59455=CARTESIAN_POINT('Ctrl Pts',(53.3370744951124,27.198270755918,12.493348638992));
#59456=CARTESIAN_POINT('Ctrl Pts',(53.2781608123703,27.2544789982947,12.489126753258));
#59457=CARTESIAN_POINT('Ctrl Pts',(53.2221503229588,27.3135241549774,12.4849048675239));
#59458=CARTESIAN_POINT('Ctrl Pts',(53.1661776108856,27.372529487533,12.4806858293209));
#59459=CARTESIAN_POINT('Ctrl Pts',(53.1131045220431,27.4343675980315,12.4764667911179));
#59460=CARTESIAN_POINT('Ctrl Pts',(53.0632235138284,27.4987181834802,12.4722477529149));
#59461=CARTESIAN_POINT('Ctrl Pts',(53.0133587949325,27.563047754374,12.4680300924959));
#59462=CARTESIAN_POINT('Ctrl Pts',(52.966684370872,27.6298878039107,12.4638124320769));
#59463=CARTESIAN_POINT('Ctrl Pts',(52.9234523512287,27.698885050281,12.459594771658));
#59464=CARTESIAN_POINT('Ctrl Pts',(52.8802212312274,27.7678808608447,12.4553771990069));
#59465=CARTESIAN_POINT('Ctrl Pts',(52.840432618875,27.8390333847079,12.4511596263559));
#59466=CARTESIAN_POINT('Ctrl Pts',(52.8042944443639,27.9119616904958,12.4469420537048));
#59467=CARTESIAN_POINT('Ctrl Pts',(52.7680949232823,27.9850137961579,12.4427173214885));
#59468=CARTESIAN_POINT('Ctrl Pts',(52.7355584457849,28.0598472965956,12.4384925892723));
#59469=CARTESIAN_POINT('Ctrl Pts',(52.7068462986919,28.136057668489,12.434267857056));
#59470=CARTESIAN_POINT('Ctrl Pts',(52.6781413227587,28.2122490060427,12.4300441800109));
#59471=CARTESIAN_POINT('Ctrl Pts',(52.6532588892888,28.2898160769963,12.4258205029657));
#59472=CARTESIAN_POINT('Ctrl Pts',(52.6323101148727,28.368339602424,12.4215968259206));
#59473=CARTESIAN_POINT('Ctrl Pts',(52.6113233320345,28.44700559706,12.4173654856444));
#59474=CARTESIAN_POINT('Ctrl Pts',(52.5942845688628,28.5266310586114,12.4131341453681));
#59475=CARTESIAN_POINT('Ctrl Pts',(52.5812538117933,28.6067861560991,12.4089028050919));
#59476=CARTESIAN_POINT('Ctrl Pts',(52.568260505356,28.6867108863821,12.4046836257644));
#59477=CARTESIAN_POINT('Ctrl Pts',(52.55925216562,28.7671617506215,12.4004644464369));
#59478=CARTESIAN_POINT('Ctrl Pts',(52.5542366399835,28.8477113372554,12.3962452671094));
#59479=CARTESIAN_POINT('Ctrl Pts',(52.5510992381463,28.8980981639606,12.3936060101436));
#59480=CARTESIAN_POINT('Ctrl Pts',(52.5495187507328,28.9485829339407,12.3909667531778));
#59481=CARTESIAN_POINT('Ctrl Pts',(52.5495001658422,28.9990984498427,12.3883274962121));
#59482=CARTESIAN_POINT('',(52.5495004573641,28.9985028222904,11.5883274962406));
#59483=CARTESIAN_POINT('Ctrl Pts',(52.5495001658419,28.9990984507376,12.3883274961653));
#59484=CARTESIAN_POINT('Ctrl Pts',(52.5494706380201,29.079357983368,12.3841342195694));
#59485=CARTESIAN_POINT('Ctrl Pts',(52.5533883882208,29.1597762288156,12.3799409429735));
#59486=CARTESIAN_POINT('Ctrl Pts',(52.561273989113,29.2399285181527,12.3757476663776));
#59487=CARTESIAN_POINT('Ctrl Pts',(52.5691487625614,29.3199707531757,12.3715601474236));
#59488=CARTESIAN_POINT('Ctrl Pts',(52.5809805248543,29.3997472893288,12.3673726284697));
#59489=CARTESIAN_POINT('Ctrl Pts',(52.5967378291866,29.4788331529219,12.3631851095157));
#59490=CARTESIAN_POINT('Ctrl Pts',(52.6124785576057,29.5578358220559,12.3590019956267));
#59491=CARTESIAN_POINT('Ctrl Pts',(52.6321365331142,29.6361487992951,12.3548188817378));
#59492=CARTESIAN_POINT('Ctrl Pts',(52.6556286436803,29.7133534843733,12.3506357678489));
#59493=CARTESIAN_POINT('Ctrl Pts',(52.6791077142574,29.7905153147137,12.3464549759207));
#59494=CARTESIAN_POINT('Ctrl Pts',(52.7064165592587,29.8665696211731,12.3422741839925));
#59495=CARTESIAN_POINT('Ctrl Pts',(52.7374215575929,29.941110536523,12.3380933920643));
#59496=CARTESIAN_POINT('Ctrl Pts',(52.7684192578951,30.0156339062507,12.3339135842211));
#59497=CARTESIAN_POINT('Ctrl Pts',(52.8031112019664,30.0886441548573,12.3297337763779));
#59498=CARTESIAN_POINT('Ctrl Pts',(52.8413152866402,30.159754525021,12.3255539685347));
#59499=CARTESIAN_POINT('Ctrl Pts',(52.8795225924527,30.2308708907836,12.3213738082753));
#59500=CARTESIAN_POINT('Ctrl Pts',(52.9212424003766,30.3000866437562,12.3171936480158));
#59501=CARTESIAN_POINT('Ctrl Pts',(52.9662469752236,30.3670401911476,12.3130134877564));
#59502=CARTESIAN_POINT('Ctrl Pts',(53.0112979745108,30.4340628044276,12.3088290154553));
#59503=CARTESIAN_POINT('Ctrl Pts',(53.0596402376615,30.4988181613851,12.3046445431542));
#59504=CARTESIAN_POINT('Ctrl Pts',(53.1110034996619,30.5609748465977,12.3004600708532));
#59505=CARTESIAN_POINT('Ctrl Pts',(53.1623967487656,30.6231678203726,12.2962731555569));
#59506=CARTESIAN_POINT('Ctrl Pts',(53.2168141858928,30.6827587546492,12.2920862402606));
#59507=CARTESIAN_POINT('Ctrl Pts',(53.2739479068017,30.739452333801,12.2878993249643));
#59508=CARTESIAN_POINT('Ctrl Pts',(53.331175189797,30.7962387542637,12.2837055531825));
#59509=CARTESIAN_POINT('Ctrl Pts',(53.3911272805342,30.8501180359065,12.2795117814007));
#59510=CARTESIAN_POINT('Ctrl Pts',(53.4534628821636,30.900834867408,12.2753180096189));
#59511=CARTESIAN_POINT('Ctrl Pts',(53.4820786349711,30.9241169129084,12.2733928186606));
#59512=CARTESIAN_POINT('Ctrl Pts',(53.5111962723062,30.946733117978,12.2714676277022));
#59513=CARTESIAN_POINT('Ctrl Pts',(53.5407808827152,30.9686619358718,12.2695424367439));
#59514=CARTESIAN_POINT('Ctrl Pts',(53.6058239064903,31.016873374316,12.2653098225724));
#59515=CARTESIAN_POINT('Ctrl Pts',(53.6733797551386,31.0619475530149,12.261077208401));
#59516=CARTESIAN_POINT('Ctrl Pts',(53.7431132472199,31.1036125928236,12.2568445942295));
#59517=CARTESIAN_POINT('Ctrl Pts',(53.8127472710226,31.1452182013652,12.2526180174847));
#59518=CARTESIAN_POINT('Ctrl Pts',(53.8845523734627,31.1834240929048,12.2483914407399));
#59519=CARTESIAN_POINT('Ctrl Pts',(53.9581623293075,31.2180001167552,12.2441648639951));
#59520=CARTESIAN_POINT('Ctrl Pts',(54.0316905866251,31.2525377652229,12.2399429782611));
#59521=CARTESIAN_POINT('Ctrl Pts',(54.1070192986825,31.2834533545764,12.2357210925271));
#59522=CARTESIAN_POINT('Ctrl Pts',(54.1837566635088,31.3105620670378,12.231499206793));
#59523=CARTESIAN_POINT('Ctrl Pts',(54.2604422713623,31.3376524955132,12.22728016859));
#59524=CARTESIAN_POINT('Ctrl Pts',(54.3385342081279,31.3609409922764,12.223061130387));
#59525=CARTESIAN_POINT('Ctrl Pts',(54.4176208316246,31.3802908969793,12.218842092184));
#59526=CARTESIAN_POINT('Ctrl Pts',(54.4966816283134,31.3996344827087,12.214624431765));
#59527=CARTESIAN_POINT('Ctrl Pts',(54.576736015751,31.4150419203746,12.210406771346));
#59528=CARTESIAN_POINT('Ctrl Pts',(54.6573586636032,31.4264268306694,12.2061891109271));
#59529=CARTESIAN_POINT('Ctrl Pts',(54.7379796337285,31.4378115040484,12.201971538276));
#59530=CARTESIAN_POINT('Ctrl Pts',(54.8191683806081,31.4451737526953,12.197753965625));
#59531=CARTESIAN_POINT('Ctrl Pts',(54.9004923134657,31.4484788074069,12.193536392974));
#59532=CARTESIAN_POINT('Ctrl Pts',(54.9819542982437,31.4517894726335,12.1893116607577));
#59533=CARTESIAN_POINT('Ctrl Pts',(55.0635514615379,31.4510291450554,12.1850869285414));
#59534=CARTESIAN_POINT('Ctrl Pts',(55.1448486614833,31.4462152634767,12.1808621963251));
#59535=CARTESIAN_POINT('Ctrl Pts',(55.2261255566005,31.4414025842154,12.17663851928));
#59536=CARTESIAN_POINT('Ctrl Pts',(55.307102177115,31.432538447385,12.1724148422349));
#59537=CARTESIAN_POINT('Ctrl Pts',(55.3873503367598,31.4196921222776,12.1681911651898));
#59538=CARTESIAN_POINT('Ctrl Pts',(55.467744094704,31.406822489432,12.1639598249135));
#59539=CARTESIAN_POINT('Ctrl Pts',(55.5474062946451,31.3899563257236,12.1597284846373));
#59540=CARTESIAN_POINT('Ctrl Pts',(55.6259199360131,31.3692138957261,12.155497144361));
#59541=CARTESIAN_POINT('Ctrl Pts',(55.7042079277511,31.3485310798487,12.1512779650335));
#59542=CARTESIAN_POINT('Ctrl Pts',(55.7813535454311,31.3239944660964,12.147058785706));
#59543=CARTESIAN_POINT('Ctrl Pts',(55.8569632320824,31.295770953048,12.1428396063785));
#59544=CARTESIAN_POINT('Ctrl Pts',(55.9328136774842,31.2674575697986,12.138606992207));
#59545=CARTESIAN_POINT('Ctrl Pts',(56.0074004941536,31.2353284389188,12.1343743780356));
#59546=CARTESIAN_POINT('Ctrl Pts',(56.0803131499589,31.1995167078306,12.1301417638641));
#59547=CARTESIAN_POINT('Ctrl Pts',(56.1531218027069,31.1637560588142,12.1259151871193));
#59548=CARTESIAN_POINT('Ctrl Pts',(56.2242606240282,31.1243234455889,12.1216886103745));
#59549=CARTESIAN_POINT('Ctrl Pts',(56.2933371844084,31.0814007728995,12.1174620336297));
#59550=CARTESIAN_POINT('Ctrl Pts',(56.3623370778054,31.0385257394064,12.1132401478957));
#59551=CARTESIAN_POINT('Ctrl Pts',(56.4292788656544,30.9921685871546,12.1090182621617));
#59552=CARTESIAN_POINT('Ctrl Pts',(56.4937942208316,30.9425573545742,12.1047963764276));
#59553=CARTESIAN_POINT('Ctrl Pts',(56.5582660624024,30.8929795832316,12.1005773382246));
#59554=CARTESIAN_POINT('Ctrl Pts',(56.6203143543339,30.8401523730299,12.0963583000216));
#59555=CARTESIAN_POINT('Ctrl Pts',(56.679600364143,30.7843466218117,12.0921392618185));
#59556=CARTESIAN_POINT('Ctrl Pts',(56.7388670133027,30.7285590947172,12.0879216013996));
#59557=CARTESIAN_POINT('Ctrl Pts',(56.7953728337728,30.6697952764575,12.0837039409806));
#59558=CARTESIAN_POINT('Ctrl Pts',(56.8488138182338,30.6083649198823,12.0794862805616));
#59559=CARTESIAN_POINT('Ctrl Pts',(56.902253690608,30.5469358416496,12.0752687079106));
#59560=CARTESIAN_POINT('Ctrl Pts',(56.9526285497644,30.4828406866846,12.0710511352595));
#59561=CARTESIAN_POINT('Ctrl Pts',(56.9996737276507,30.4164233946612,12.0668335626085));
#59562=CARTESIAN_POINT('Ctrl Pts',(57.0467987673553,30.3498933555733,12.0626088303922));
#59563=CARTESIAN_POINT('Ctrl Pts',(57.0905825468881,30.2810336735705,12.0583840981759));
#59564=CARTESIAN_POINT('Ctrl Pts',(57.1308028027755,30.2102188503258,12.0541593659596));
#59565=CARTESIAN_POINT('Ctrl Pts',(57.1710130132322,30.1394217138259,12.0499356889145));
#59566=CARTESIAN_POINT('Ctrl Pts',(57.2076612891364,30.0666708384707,12.0457120118694));
#59567=CARTESIAN_POINT('Ctrl Pts',(57.2405726303686,29.9923631079616,12.0414883348243));
#59568=CARTESIAN_POINT('Ctrl Pts',(57.2735436843137,29.9179205571743,12.037256994548));
#59569=CARTESIAN_POINT('Ctrl Pts',(57.3027640865823,29.8419159410713,12.0330256542718));
#59570=CARTESIAN_POINT('Ctrl Pts',(57.3281077026861,29.7647645223816,12.0287943139956));
#59571=CARTESIAN_POINT('Ctrl Pts',(57.3533784807775,29.687834838269,12.024575134668));
#59572=CARTESIAN_POINT('Ctrl Pts',(57.3747946866316,29.609765395665,12.0203559553405));
#59573=CARTESIAN_POINT('Ctrl Pts',(57.392282066255,29.5309771798061,12.016136776013));
#59574=CARTESIAN_POINT('Ctrl Pts',(57.4098251297444,29.4519380840238,12.0119041618415));
#59575=CARTESIAN_POINT('Ctrl Pts',(57.4234795273592,29.3718816558138,12.00767154767));
#59576=CARTESIAN_POINT('Ctrl Pts',(57.4331334524926,29.2912247454487,12.0034389334986));
#59577=CARTESIAN_POINT('Ctrl Pts',(57.4427736072081,29.210682884593,11.9992123567538));
#59578=CARTESIAN_POINT('Ctrl Pts',(57.4484245681362,29.1295427001877,11.994985780009));
#59579=CARTESIAN_POINT('Ctrl Pts',(57.4500252826214,29.0482324010992,11.9907592032642));
#59580=CARTESIAN_POINT('Ctrl Pts',(57.451624220499,28.9670123470269,11.9865373175302));
#59581=CARTESIAN_POINT('Ctrl Pts',(57.4491818349971,28.8856230155492,11.9823154317961));
#59582=CARTESIAN_POINT('Ctrl Pts',(57.4426888929207,28.8044975130547,11.9780935460621));
#59583=CARTESIAN_POINT('Ctrl Pts',(57.4362003301324,28.7234267271958,11.9738745078591));
#59584=CARTESIAN_POINT('Ctrl Pts',(57.4256666736764,28.6426198787795,11.9696554696561));
#59585=CARTESIAN_POINT('Ctrl Pts',(57.4111307532604,28.5625085821617,11.965436431453));
#59586=CARTESIAN_POINT('Ctrl Pts',(57.3965995797459,28.4824234469727,11.9612187710341));
#59587=CARTESIAN_POINT('Ctrl Pts',(57.3780688207534,28.4030338692272,11.9570011106151));
#59588=CARTESIAN_POINT('Ctrl Pts',(57.3556328029574,28.324763487635,11.9527834501961));
#59589=CARTESIAN_POINT('Ctrl Pts',(57.3331972520466,28.24649473482,11.9485658775451));
#59590=CARTESIAN_POINT('Ctrl Pts',(57.3068567330474,28.1693455780917,11.944348304894));
#59591=CARTESIAN_POINT('Ctrl Pts',(57.2767556657342,28.0937252687251,11.940130732243));
#59592=CARTESIAN_POINT('Ctrl Pts',(57.2466035001772,28.0179765896579,11.9359060000267));
#59593=CARTESIAN_POINT('Ctrl Pts',(57.2126781866408,27.943762384433,11.9316812678104));
#59594=CARTESIAN_POINT('Ctrl Pts',(57.175172866162,27.8714729722719,11.9274565355941));
#59595=CARTESIAN_POINT('Ctrl Pts',(57.1376769130302,27.7992016151496,11.923232858549));
#59596=CARTESIAN_POINT('Ctrl Pts',(57.0966029944165,27.7288544815802,11.9190091815039));
#59597=CARTESIAN_POINT('Ctrl Pts',(57.052188756176,27.6607944298858,11.9147855044588));
#59598=CARTESIAN_POINT('Ctrl Pts',(57.007693934934,27.5926108933933,11.9105541641825));
#59599=CARTESIAN_POINT('Ctrl Pts',(56.9598469561017,27.5267231085291,11.9063228239063));
#59600=CARTESIAN_POINT('Ctrl Pts',(56.9089274848149,27.4634629494482,11.9020914836301));
#59601=CARTESIAN_POINT('Ctrl Pts',(56.8581543570125,27.4003846012124,11.8978723043025));
#59602=CARTESIAN_POINT('Ctrl Pts',(56.8043267388008,27.3399190799684,11.893653124975));
#59603=CARTESIAN_POINT('Ctrl Pts',(56.7477573392823,27.2823578565414,11.8894339456475));
#59604=CARTESIAN_POINT('Ctrl Pts',(56.6910078096964,27.2246133448501,11.885201331476));
#59605=CARTESIAN_POINT('Ctrl Pts',(56.6312879231681,27.1695769076014,11.8809687173046));
#59606=CARTESIAN_POINT('Ctrl Pts',(56.5688864766152,27.1175692646225,11.8767361031331));
#59607=CARTESIAN_POINT('Ctrl Pts',(56.5065740398665,27.0656358056629,11.8725095263883));
#59608=CARTESIAN_POINT('Ctrl Pts',(56.441587993916,27.0167228552666,11.8682829496435));
#59609=CARTESIAN_POINT('Ctrl Pts',(56.3742542940485,26.9711147431929,11.8640563728987));
#59610=CARTESIAN_POINT('Ctrl Pts',(56.3069953267909,26.9255572508424,11.8598344871647));
#59611=CARTESIAN_POINT('Ctrl Pts',(56.2373942656691,26.8832975677387,11.8556126014307));
#59612=CARTESIAN_POINT('Ctrl Pts',(56.165809384689,26.8445792223858,11.8513907156966));
#59613=CARTESIAN_POINT('Ctrl Pts',(56.0942727854914,26.8058869913562,11.8471716774936));
#59614=CARTESIAN_POINT('Ctrl Pts',(56.0207554314249,26.7707315746989,11.8429526392906));
#59615=CARTESIAN_POINT('Ctrl Pts',(55.9456426880273,26.7393120169779,11.8387336010876));
#59616=CARTESIAN_POINT('Ctrl Pts',(55.8705544737131,26.707902719739,11.8345159406686));
#59617=CARTESIAN_POINT('Ctrl Pts',(55.7938723329707,26.6802270377313,11.8302982802497));
#59618=CARTESIAN_POINT('Ctrl Pts',(55.7160029761548,26.6564364766157,11.8260806198307));
#59619=CARTESIAN_POINT('Ctrl Pts',(55.6381352397707,26.6326464105726,11.8218630471797));
#59620=CARTESIAN_POINT('Ctrl Pts',(55.5590807810528,26.6127414392866,11.8176454745286));
#59621=CARTESIAN_POINT('Ctrl Pts',(55.4792615125366,26.5968232165317,11.8134279018775));
#59622=CARTESIAN_POINT('Ctrl Pts',(55.3993067463523,26.5808779717043,11.8092031696613));
#59623=CARTESIAN_POINT('Ctrl Pts',(55.3185850307356,26.5689331073856,11.804978437445));
#59624=CARTESIAN_POINT('Ctrl Pts',(55.2375289214324,26.5610391021004,11.8007537052287));
#59625=CARTESIAN_POINT('Ctrl Pts',(55.1564930567426,26.5531470684259,11.7965300281836));
#59626=CARTESIAN_POINT('Ctrl Pts',(55.0751234320191,26.549303871314,11.7923063511385));
#59627=CARTESIAN_POINT('Ctrl Pts',(54.9938537965713,26.5495077077894,11.7880826740934));
#59628=CARTESIAN_POINT('Ctrl Pts',(54.9124367095087,26.5497119140958,11.7838513338171));
#59629=CARTESIAN_POINT('Ctrl Pts',(54.8311204395328,26.5539778037926,11.7796199935409));
#59630=CARTESIAN_POINT('Ctrl Pts',(54.7503356209827,26.5622514592662,11.7753886532646));
#59631=CARTESIAN_POINT('Ctrl Pts',(54.669782979467,26.5705013361038,11.7711694739371));
#59632=CARTESIAN_POINT('Ctrl Pts',(54.5897591761054,26.5827358216747,11.7669502946096));
#59633=CARTESIAN_POINT('Ctrl Pts',(54.5106789430665,26.598851284647,11.7627311152821));
#59634=CARTESIAN_POINT('Ctrl Pts',(54.4313469002539,26.615018062985,11.7584985011107));
#59635=CARTESIAN_POINT('Ctrl Pts',(54.352669393887,26.6351507295708,11.7542658869392));
#59636=CARTESIAN_POINT('Ctrl Pts',(54.2750726731228,26.6591816343965,11.7500332727677));
#59637=CARTESIAN_POINT('Ctrl Pts',(54.197586636795,26.6831782613928,11.7458066960229));
#59638=CARTESIAN_POINT('Ctrl Pts',(54.1211787642444,26.7110619465329,11.7415801192782));
#59639=CARTESIAN_POINT('Ctrl Pts',(54.0462650087663,26.7427140596512,11.7373535425334));
#59640=CARTESIAN_POINT('Ctrl Pts',(53.9714343988815,26.7743310425893,11.7331316567994));
#59641=CARTESIAN_POINT('Ctrl Pts',(53.8980950368,26.8097079629586,11.7289097710654));
#59642=CARTESIAN_POINT('Ctrl Pts',(53.8266462450325,26.8486768685984,11.7246878853313));
#59643=CARTESIAN_POINT('Ctrl Pts',(53.7552456432594,26.8876194909198,11.7204688471283));
#59644=CARTESIAN_POINT('Ctrl Pts',(53.6857334860588,26.9301490649902,11.7162498089253));
#59645=CARTESIAN_POINT('Ctrl Pts',(53.6184865303419,26.9760506964963,11.7120307707223));
#59646=CARTESIAN_POINT('Ctrl Pts',(53.5512615350292,27.0219373382029,11.7078131103033));
#59647=CARTESIAN_POINT('Ctrl Pts',(53.4863006555292,27.0711935887503,11.7035954498844));
#59648=CARTESIAN_POINT('Ctrl Pts',(53.4239523920575,27.1235607690366,11.6993777894654));
#59649=CARTESIAN_POINT('Ctrl Pts',(53.3616054260292,27.1759268595818,11.6951602168144));
#59650=CARTESIAN_POINT('Ctrl Pts',(53.3018713228988,27.2314034514767,11.6909426441633));
#59651=CARTESIAN_POINT('Ctrl Pts',(53.2450650419408,27.2896919742392,11.6867250715122));
#59652=CARTESIAN_POINT('Ctrl Pts',(53.1881623291467,27.3480794450261,11.682500339296));
#59653=CARTESIAN_POINT('Ctrl Pts',(53.1341977085533,27.4092880627194,11.6782756070797));
#59654=CARTESIAN_POINT('Ctrl Pts',(53.0834490065173,27.4729824691968,11.6740508748634));
#59655=CARTESIAN_POINT('Ctrl Pts',(53.032712979502,27.5366609673279,11.6698271978183));
#59656=CARTESIAN_POINT('Ctrl Pts',(52.9851915195056,27.6028236216844,11.6656035207732));
#59657=CARTESIAN_POINT('Ctrl Pts',(52.9411192476209,27.6711056108619,11.661379843728));
#59658=CARTESIAN_POINT('Ctrl Pts',(52.8969670131816,27.7395114875099,11.6571485034518));
#59659=CARTESIAN_POINT('Ctrl Pts',(52.8562767061392,27.8100439799548,11.6529171631756));
#59660=CARTESIAN_POINT('Ctrl Pts',(52.8192375367207,27.8823125084568,11.6486858228993));
#59661=CARTESIAN_POINT('Ctrl Pts',(52.7823048185469,27.9543733358971,11.6444666435718));
#59662=CARTESIAN_POINT('Ctrl Pts',(52.7490023906174,28.0281597847597,11.6402474642442));
#59663=CARTESIAN_POINT('Ctrl Pts',(52.7194691048837,28.1032675502581,11.6360282849167));
#59664=CARTESIAN_POINT('Ctrl Pts',(52.6860019559815,28.1883797451664,11.631247106687));
#59665=CARTESIAN_POINT('Ctrl Pts',(52.65726976131,28.2754529496787,11.6264659284574));
#59666=CARTESIAN_POINT('Ctrl Pts',(52.6334774315741,28.3639802022492,11.6216847502278));
#59667=CARTESIAN_POINT('Ctrl Pts',(52.6097729953872,28.4521804177246,11.6169212346115));
#59668=CARTESIAN_POINT('Ctrl Pts',(52.5909721282548,28.5418237490575,11.6121577189953));
#59669=CARTESIAN_POINT('Ctrl Pts',(52.5772307427071,28.6323869209124,11.6073942033791));
#59670=CARTESIAN_POINT('Ctrl Pts',(52.5635760436512,28.722378781845,11.602660738041));
#59671=CARTESIAN_POINT('Ctrl Pts',(52.554917305081,28.8132786888873,11.5979272727028));
#59672=CARTESIAN_POINT('Ctrl Pts',(52.5513594669747,28.9045547799749,11.5931938073647));
#59673=CARTESIAN_POINT('Ctrl Pts',(52.5501402370929,28.9358340384533,11.5915717036567));
#59674=CARTESIAN_POINT('Ctrl Pts',(52.5495196084685,28.9671573297734,11.5899495999486));
#59675=CARTESIAN_POINT('Ctrl Pts',(52.5495004573641,28.9985028222904,11.5883274962406));
#59676=CARTESIAN_POINT('',(52.5495008325386,29.0020199680429,10.7883274961659));
#59677=CARTESIAN_POINT('Ctrl Pts',(52.5495004573637,28.9985028228412,11.5883274962121));
#59678=CARTESIAN_POINT('Ctrl Pts',(52.5494502760639,29.0806368920414,11.5840771250261));
#59679=CARTESIAN_POINT('Ctrl Pts',(52.5535337966699,29.162786480375,11.5798267538401));
#59680=CARTESIAN_POINT('Ctrl Pts',(52.5617291806368,29.2445110660934,11.575576382654));
#59681=CARTESIAN_POINT('Ctrl Pts',(52.5699256911786,29.3262468860455,11.5713254271926));
#59682=CARTESIAN_POINT('Ctrl Pts',(52.5822351423506,29.4075571352908,11.5670744717312));
#59683=CARTESIAN_POINT('Ctrl Pts',(52.598583889012,29.4880070818006,11.5628235162698));
#59684=CARTESIAN_POINT('Ctrl Pts',(52.6157295688845,29.5723786276551,11.5583653444599));
#59685=CARTESIAN_POINT('Ctrl Pts',(52.6373182619213,29.6558033196536,11.5539071726501));
#59686=CARTESIAN_POINT('Ctrl Pts',(52.6632053716463,29.7377947647533,11.5494490008402));
#59687=CARTESIAN_POINT('Ctrl Pts',(52.6879344924561,29.816118547237,11.5451902531295));
#59688=CARTESIAN_POINT('Ctrl Pts',(52.7165854932329,29.8931341456156,11.5409315054189));
#59689=CARTESIAN_POINT('Ctrl Pts',(52.7489826375331,29.9684374444808,11.5366727577082));
#59690=CARTESIAN_POINT('Ctrl Pts',(52.781406914166,30.0438038092182,11.5324104433326));
#59691=CARTESIAN_POINT('Ctrl Pts',(52.817583379001,30.1174546134316,11.528148128957));
#59692=CARTESIAN_POINT('Ctrl Pts',(52.8572903621785,30.1890103691671,11.5238858145813));
#59693=CARTESIAN_POINT('Ctrl Pts',(52.8970653766748,30.260688723802,11.5196161974381));
#59694=CARTESIAN_POINT('Ctrl Pts',(52.9403827378663,30.3302644848842,11.515346580295));
#59695=CARTESIAN_POINT('Ctrl Pts',(52.9869778522888,30.3973875921963,11.5110769631518));
#59696=CARTESIAN_POINT('Ctrl Pts',(52.9933493637473,30.4065661434816,11.5104931269516));
#59697=CARTESIAN_POINT('Ctrl Pts',(52.9997821040668,30.4156988867582,11.5099092907514));
#59698=CARTESIAN_POINT('Ctrl Pts',(53.0062753409067,30.4247849780663,11.5093254545513));
#59699=CARTESIAN_POINT('Ctrl Pts',(53.0533491027925,30.4906560542727,11.5050928403798));
#59700=CARTESIAN_POINT('Ctrl Pts',(53.1037784033861,30.5543142031118,11.5008602262083));
#59701=CARTESIAN_POINT('Ctrl Pts',(53.1573278646467,30.6153976759896,11.4966276120368));
#59702=CARTESIAN_POINT('Ctrl Pts',(53.2108009426289,30.6763940190287,11.492401035292));
#59703=CARTESIAN_POINT('Ctrl Pts',(53.2673850380899,30.734822633813,11.4881744585472));
#59704=CARTESIAN_POINT('Ctrl Pts',(53.3268024051304,30.7903519370567,11.4839478818025));
#59705=CARTESIAN_POINT('Ctrl Pts',(53.3861538257739,30.8458196092039,11.4797259960684));
#59706=CARTESIAN_POINT('Ctrl Pts',(53.4483319319848,30.898394048177,11.4755041103344));
#59707=CARTESIAN_POINT('Ctrl Pts',(53.5130207043615,30.9477789464779,11.4712822246004));
#59708=CARTESIAN_POINT('Ctrl Pts',(53.5776658461673,30.9971305361963,11.4670631863973));
#59709=CARTESIAN_POINT('Ctrl Pts',(53.6448179226719,31.0432965766419,11.4628441481943));
#59710=CARTESIAN_POINT('Ctrl Pts',(53.7141272315008,31.0860204872513,11.4586251099913));
#59711=CARTESIAN_POINT('Ctrl Pts',(53.7834139064364,31.1287304457891,11.4544074495723));
#59712=CARTESIAN_POINT('Ctrl Pts',(53.8548560195054,31.1680002632532,11.4501897891534));
#59713=CARTESIAN_POINT('Ctrl Pts',(53.9280753867571,31.2036169979205,11.4459721287344));
#59714=CARTESIAN_POINT('Ctrl Pts',(54.0012932303415,31.239232991417,11.4417545560833));
#59715=CARTESIAN_POINT('Ctrl Pts',(54.0762878363156,31.2711958511109,11.4375369834323));
#59716=CARTESIAN_POINT('Ctrl Pts',(54.1526582470961,31.2993395146837,11.4333194107812));
#59717=CARTESIAN_POINT('Ctrl Pts',(54.2291583009165,31.327530953698,11.4290946785649));
#59718=CARTESIAN_POINT('Ctrl Pts',(54.3070383941571,31.3518900635452,11.4248699463486));
#59719=CARTESIAN_POINT('Ctrl Pts',(54.3858790931439,31.3722996778995,11.4206452141324));
#59720=CARTESIAN_POINT('Ctrl Pts',(54.4647001008393,31.3927041947387,11.4164215370872));
#59721=CARTESIAN_POINT('Ctrl Pts',(54.5444807736633,31.409161115333,11.4121978600421));
#59722=CARTESIAN_POINT('Ctrl Pts',(54.6247923642888,31.4216047324252,11.407974182997));
#59723=CARTESIAN_POINT('Ctrl Pts',(54.7052496682997,31.4340709266019,11.4037428427208));
#59724=CARTESIAN_POINT('Ctrl Pts',(54.7862393517869,31.4425092170877,11.3995115024445));
#59725=CARTESIAN_POINT('Ctrl Pts',(54.8673276357942,31.4469058612411,11.3952801621683));
#59726=CARTESIAN_POINT('Ctrl Pts',(54.9481828706022,31.4512898693594,11.3910609828408));
#59727=CARTESIAN_POINT('Ctrl Pts',(55.0291356843062,31.4516555127718,11.3868418035132));
#59728=CARTESIAN_POINT('Ctrl Pts',(55.109760271355,31.4480406313687,11.3826226241857));
#59729=CARTESIAN_POINT('Ctrl Pts',(55.1906415857582,31.4444142393462,11.3783900100142));
#59730=CARTESIAN_POINT('Ctrl Pts',(55.2714933988372,31.436768417361,11.3741573958427));
#59731=CARTESIAN_POINT('Ctrl Pts',(55.3518841267503,31.4251036702255,11.3699247816713));
#59732=CARTESIAN_POINT('Ctrl Pts',(55.4321601848385,31.4134555617565,11.3656982049265));
#59733=CARTESIAN_POINT('Ctrl Pts',(55.511976008113,31.3977999800111,11.3614716281817));
#59734=CARTESIAN_POINT('Ctrl Pts',(55.5909022510574,31.3781893910484,11.3572450514369));
#59735=CARTESIAN_POINT('Ctrl Pts',(55.6697408950114,31.3586005675686,11.3530231657028));
#59736=CARTESIAN_POINT('Ctrl Pts',(55.7476914718922,31.3350655704522,11.3488012799688));
#59737=CARTESIAN_POINT('Ctrl Pts',(55.8243333902782,31.3076881747048,11.3445793942348));
#59738=CARTESIAN_POINT('Ctrl Pts',(55.9009236160669,31.2803292441618,11.3403603560318));
#59739=CARTESIAN_POINT('Ctrl Pts',(55.9762065000338,31.2491332179575,11.3361413178288));
#59740=CARTESIAN_POINT('Ctrl Pts',(56.0497764376747,31.2142537526,11.3319222796257));
#59741=CARTESIAN_POINT('Ctrl Pts',(56.1233223500562,31.1793856776042,11.3277046192068));
#59742=CARTESIAN_POINT('Ctrl Pts',(56.195156007577,31.1408367511517,11.3234869587878));
#59743=CARTESIAN_POINT('Ctrl Pts',(56.2648929057,31.0988082778352,11.3192692983688));
#59744=CARTESIAN_POINT('Ctrl Pts',(56.3346283526245,31.0567806791155,11.3150517257178));
#59745=CARTESIAN_POINT('Ctrl Pts',(56.4022667296338,31.0112739182926,11.3108341530667));
#59746=CARTESIAN_POINT('Ctrl Pts',(56.4674504578341,30.9625339242424,11.3066165804157));
#59747=CARTESIAN_POINT('Ctrl Pts',(56.5327448390552,30.913711191329,11.3023918481994));
#59748=CARTESIAN_POINT('Ctrl Pts',(56.5955758604643,30.8616445234465,11.2981671159831));
#59749=CARTESIAN_POINT('Ctrl Pts',(56.6556168999613,30.8066219666999,11.2939423837669));
#59750=CARTESIAN_POINT('Ctrl Pts',(56.715642943579,30.7516131524138,11.2897187067217));
#59751=CARTESIAN_POINT('Ctrl Pts',(56.7728800863489,30.6936502722294,11.2854950296766));
#59752=CARTESIAN_POINT('Ctrl Pts',(56.8270398009749,30.6330571991371,11.2812713526315));
#59753=CARTESIAN_POINT('Ctrl Pts',(56.8812977803136,30.5723541889642,11.2770400123553));
#59754=CARTESIAN_POINT('Ctrl Pts',(56.9324668802389,30.5090118114391,11.272808672079));
#59755=CARTESIAN_POINT('Ctrl Pts',(56.9802994234629,30.4433864497883,11.2685773318028));
#59756=CARTESIAN_POINT('Ctrl Pts',(57.0279944950895,30.377949696618,11.2643581524753));
#59757=CARTESIAN_POINT('Ctrl Pts',(57.0723719830576,30.3102434908223,11.2601389731478));
#59758=CARTESIAN_POINT('Ctrl Pts',(57.1132318195364,30.2406456089065,11.2559197938203));
#59759=CARTESIAN_POINT('Ctrl Pts',(57.1542217631962,30.1708261112182,11.2516871796488));
#59760=CARTESIAN_POINT('Ctrl Pts',(57.1918240470589,30.0988431790726,11.2474545654774));
#59761=CARTESIAN_POINT('Ctrl Pts',(57.2258041399824,30.0250591107039,11.2432219513059));
#59762=CARTESIAN_POINT('Ctrl Pts',(57.2597357634939,29.9513802883808,11.2389953745611));
#59763=CARTESIAN_POINT('Ctrl Pts',(57.2900552651194,29.8759058509472,11.2347687978163));
#59764=CARTESIAN_POINT('Ctrl Pts',(57.3165729186675,29.7990245068183,11.2305422210715));
#59765=CARTESIAN_POINT('Ctrl Pts',(57.3430611406908,29.7222284920788,11.2263203353375));
#59766=CARTESIAN_POINT('Ctrl Pts',(57.3657557482853,29.6440291102945,11.2220984496035));
#59767=CARTESIAN_POINT('Ctrl Pts',(57.3845148202347,29.564835659357,11.2178765638694));
#59768=CARTESIAN_POINT('Ctrl Pts',(57.4032612397717,29.4856956219463,11.2136575256664));
#59769=CARTESIAN_POINT('Ctrl Pts',(57.4180772887261,29.4055632978649,11.2094384874634));
#59770=CARTESIAN_POINT('Ctrl Pts',(57.4288710466342,29.3248625691302,11.2052194492604));
#59771=CARTESIAN_POINT('Ctrl Pts',(57.4396612796946,29.2441881943112,11.2010017888414));
#59772=CARTESIAN_POINT('Ctrl Pts',(57.446431768768,29.1629462435645,11.1967841284224));
#59773=CARTESIAN_POINT('Ctrl Pts',(57.4491420486453,29.0815688393782,11.1925664680035));
#59774=CARTESIAN_POINT('Ctrl Pts',(57.4518522721227,29.0001931286248,11.1883488953524));
#59775=CARTESIAN_POINT('Ctrl Pts',(57.4505024401052,28.9186824343659,11.1841313227014));
#59776=CARTESIAN_POINT('Ctrl Pts',(57.4451041776997,28.8374705866766,11.1799137500503));
#59777=CARTESIAN_POINT('Ctrl Pts',(57.4396967514422,28.756120877338,11.175689017834));
#59778=CARTESIAN_POINT('Ctrl Pts',(57.4302271756289,28.6750714955413,11.1714642856177));
#59779=CARTESIAN_POINT('Ctrl Pts',(57.4167592572644,28.5947532326757,11.1672395534014));
#59780=CARTESIAN_POINT('Ctrl Pts',(57.4032947026538,28.5144550301386,11.1630158763563));
#59781=CARTESIAN_POINT('Ctrl Pts',(57.3858339231741,28.4348880321328,11.1587921993112));
#59782=CARTESIAN_POINT('Ctrl Pts',(57.3644915171676,28.3564705793497,11.1545685222661));
#59783=CARTESIAN_POINT('Ctrl Pts',(57.3431103885532,28.2779108498114,11.1503371819898));
#59784=CARTESIAN_POINT('Ctrl Pts',(57.3178337035763,28.2005052765348,11.1461058417136));
#59785=CARTESIAN_POINT('Ctrl Pts',(57.2888255697627,28.1246556327933,11.1418745014374));
#59786=CARTESIAN_POINT('Ctrl Pts',(57.2599008058519,28.0490239823041,11.1376553221098));
#59787=CARTESIAN_POINT('Ctrl Pts',(57.2272662726081,27.9749397128427,11.1334361427823));
#59788=CARTESIAN_POINT('Ctrl Pts',(57.1911299414055,27.9027763081868,11.1292169634548));
#59789=CARTESIAN_POINT('Ctrl Pts',(57.1548785437568,27.8303831185404,11.1249843492833));
#59790=CARTESIAN_POINT('Ctrl Pts',(57.1149681579824,27.7596538079307,11.1207517351119));
#59791=CARTESIAN_POINT('Ctrl Pts',(57.0715750100384,27.6909823424474,11.1165191209404));
#59792=CARTESIAN_POINT('Ctrl Pts',(57.0282437583455,27.6224088303617,11.1122925441956));
#59793=CARTESIAN_POINT('Ctrl Pts',(56.9814398573322,27.5558877229245,11.1080659674508));
#59794=CARTESIAN_POINT('Ctrl Pts',(56.9313860783316,27.4917897804263,11.103839390706));
#59795=CARTESIAN_POINT('Ctrl Pts',(56.8813878532297,27.4277629792217,11.099617504972));
#59796=CARTESIAN_POINT('Ctrl Pts',(56.8281472016935,27.3661543633525,11.095395619238));
#59797=CARTESIAN_POINT('Ctrl Pts',(56.7719301910955,27.3073058020173,11.091173733504));
#59798=CARTESIAN_POINT('Ctrl Pts',(56.7157510971278,27.2484969322118,11.0869546953009));
#59799=CARTESIAN_POINT('Ctrl Pts',(56.6565999511539,27.1924447547406,11.0827356570979));
#59800=CARTESIAN_POINT('Ctrl Pts',(56.5947822745287,27.1394571365193,11.0785166188949));
#59801=CARTESIAN_POINT('Ctrl Pts',(56.5329847853029,27.0864868221223,11.0742989584759));
#59802=CARTESIAN_POINT('Ctrl Pts',(56.468522847203,27.0365793815965,11.070081298057));
#59803=CARTESIAN_POINT('Ctrl Pts',(56.4017369061809,26.9900040060114,11.065863637638));
#59804=CARTESIAN_POINT('Ctrl Pts',(56.334952354949,26.9434295996422,11.061646064987));
#59805=CARTESIAN_POINT('Ctrl Pts',(56.2658442786624,26.9001873851175,11.0574284923359));
#59806=CARTESIAN_POINT('Ctrl Pts',(56.1947829136503,26.8605037884471,11.0532109196849));
#59807=CARTESIAN_POINT('Ctrl Pts',(56.1236009180002,26.8207528266538,11.0489861874686));
#59808=CARTESIAN_POINT('Ctrl Pts',(56.0504594071755,26.7845727969416,11.0447614552523));
#59809=CARTESIAN_POINT('Ctrl Pts',(55.9757544764458,26.7521446995645,11.040536723036));
#59810=CARTESIAN_POINT('Ctrl Pts',(55.9010682040559,26.7197247014448,11.0363130459909));
#59811=CARTESIAN_POINT('Ctrl Pts',(55.8248197364326,26.6910549058961,11.0320893689458));
#59812=CARTESIAN_POINT('Ctrl Pts',(55.7474223757313,26.6662669299476,11.0278656919007));
#59813=CARTESIAN_POINT('Ctrl Pts',(55.6698845890796,26.6414339799192,11.0236343516245));
#59814=CARTESIAN_POINT('Ctrl Pts',(55.5911941937921,26.6204970444419,11.0194030113482));
#59815=CARTESIAN_POINT('Ctrl Pts',(55.5117775476953,26.6035371916771,11.015171671072));
#59816=CARTESIAN_POINT('Ctrl Pts',(55.4325891464803,26.5866260818368,11.0109524917445));
#59817=CARTESIAN_POINT('Ctrl Pts',(55.3526791260918,26.5736692155802,11.0067333124169));
#59818=CARTESIAN_POINT('Ctrl Pts',(55.2724739939285,26.5646954661413,11.0025141330894));
#59819=CARTESIAN_POINT('Ctrl Pts',(55.1920134700522,26.5556931422063,10.9982815189179));
#59820=CARTESIAN_POINT('Ctrl Pts',(55.1109566938016,26.5506658869071,10.9940489047465));
#59821=CARTESIAN_POINT('Ctrl Pts',(55.029730071424,26.5496803529227,10.989816290575));
#59822=CARTESIAN_POINT('Ctrl Pts',(54.9486193111962,26.54869622471,10.9855897138302));
#59823=CARTESIAN_POINT('Ctrl Pts',(54.8673396466744,26.5517423730987,10.9813631370854));
#59824=CARTESIAN_POINT('Ctrl Pts',(54.7863233578371,26.5588337740756,10.9771365603406));
#59825=CARTESIAN_POINT('Ctrl Pts',(54.7053969876991,26.5659173044185,10.9729146746066));
#59826=CARTESIAN_POINT('Ctrl Pts',(54.6247338728599,26.5770371258987,10.9686927888725));
#59827=CARTESIAN_POINT('Ctrl Pts',(54.5447656291199,26.5921561683595,10.9644709031385));
#59828=CARTESIAN_POINT('Ctrl Pts',(54.4648513214803,26.6072650134949,10.9602518649355));
#59829=CARTESIAN_POINT('Ctrl Pts',(54.3856314094065,26.6263676363598,10.9560328267325));
#59830=CARTESIAN_POINT('Ctrl Pts',(54.3075304655059,26.6493753609312,10.9518137885294));
#59831=CARTESIAN_POINT('Ctrl Pts',(54.2294550265261,26.6723755720185,10.9475961281105));
#59832=CARTESIAN_POINT('Ctrl Pts',(54.1524982753025,26.6992782210437,10.9433784676915));
#59833=CARTESIAN_POINT('Ctrl Pts',(54.0770713551459,26.7299442811887,10.9391608072725));
#59834=CARTESIAN_POINT('Ctrl Pts',(54.0016460045951,26.7606097031846,10.9349432346215));
#59835=CARTESIAN_POINT('Ctrl Pts',(53.9277508517128,26.7950382045397,10.9307256619704));
#59836=CARTESIAN_POINT('Ctrl Pts',(53.8557773853043,26.8330424881832,10.9265080893194));
#59837=CARTESIAN_POINT('Ctrl Pts',(53.7836817399151,26.8711112862218,10.9222833571031));
#59838=CARTESIAN_POINT('Ctrl Pts',(53.7135147207998,26.9127677933263,10.9180586248868));
#59839=CARTESIAN_POINT('Ctrl Pts',(53.6456437901219,26.9577782914765,10.9138338926705));
#59840=CARTESIAN_POINT('Ctrl Pts',(53.5777898109206,27.0027775477829,10.9096102156254));
#59841=CARTESIAN_POINT('Ctrl Pts',(53.512231135899,27.0511288261646,10.9053865385803));
#59842=CARTESIAN_POINT('Ctrl Pts',(53.4493031707684,27.1025570907637,10.9011628615351));
#59843=CARTESIAN_POINT('Ctrl Pts',(53.3862610322444,27.1540786642673,10.8969315212589));
#59844=CARTESIAN_POINT('Ctrl Pts',(53.3258594879415,27.2086880684349,10.8927001809826));
#59845=CARTESIAN_POINT('Ctrl Pts',(53.2683986494233,27.2660717971378,10.8884688407064));
#59846=CARTESIAN_POINT('Ctrl Pts',(53.2111029543979,27.3232906039629,10.8842496613789));
#59847=CARTESIAN_POINT('Ctrl Pts',(53.1567313285859,27.3832674165504,10.8800304820514));
#59848=CARTESIAN_POINT('Ctrl Pts',(53.1055401825562,27.4456601883466,10.8758113027239));
#59849=CARTESIAN_POINT('Ctrl Pts',(53.0544250736637,27.50796028459,10.8715983903848));
#59850=CARTESIAN_POINT('Ctrl Pts',(53.0062851429247,27.5729079792855,10.8673854780457));
#59851=CARTESIAN_POINT('Ctrl Pts',(52.9614081126638,27.6401862749307,10.8631725657066));
#59852=CARTESIAN_POINT('Ctrl Pts',(52.9165921463314,27.7073730253686,10.8589653858542));
#59853=CARTESIAN_POINT('Ctrl Pts',(52.8750305270319,27.7768836970744,10.8547582060018));
#59854=CARTESIAN_POINT('Ctrl Pts',(52.8369711761229,27.8483678725058,10.8505510261493));
#59855=CARTESIAN_POINT('Ctrl Pts',(52.7989517092293,27.919777136624,10.8463482551799));
#59856=CARTESIAN_POINT('Ctrl Pts',(52.76442744343,27.9931553871588,10.8421454842105));
#59857=CARTESIAN_POINT('Ctrl Pts',(52.7336025250028,28.0681240772901,10.8379427132411));
#59858=CARTESIAN_POINT('Ctrl Pts',(52.7027967376404,28.1430462391272,10.8337425506642));
#59859=CARTESIAN_POINT('Ctrl Pts',(52.6756859210305,28.2195564499582,10.8295423880872));
#59860=CARTESIAN_POINT('Ctrl Pts',(52.6524272465736,28.2972536607209,10.8253422255102));
#59861=CARTESIAN_POINT('Ctrl Pts',(52.6291779684574,28.3749194823579,10.8211437597693));
#59862=CARTESIAN_POINT('Ctrl Pts',(52.6097778731808,28.4537709017236,10.8169452940285));
#59863=CARTESIAN_POINT('Ctrl Pts',(52.594334617116,28.5333906177609,10.8127468282876));
#59864=CARTESIAN_POINT('Ctrl Pts',(52.5788858380369,28.613038808417,10.8085468610378));
#59865=CARTESIAN_POINT('Ctrl Pts',(52.567396821711,28.6934553850803,10.804346893788));
#59866=CARTESIAN_POINT('Ctrl Pts',(52.5599241172339,28.77421263024,10.8001469265382));
#59867=CARTESIAN_POINT('Ctrl Pts',(52.5529142919454,28.8499675568645,10.7962071164295));
#59868=CARTESIAN_POINT('Ctrl Pts',(52.5494381866502,28.9260218523768,10.7922673063208));
#59869=CARTESIAN_POINT('Ctrl Pts',(52.5495008325378,29.0020199671524,10.7883274962121));
#59870=CARTESIAN_POINT('',(52.5495000009021,28.9999335093135,9.98832749618066));
#59871=CARTESIAN_POINT('Ctrl Pts',(52.5495008325386,29.0020199680429,10.7883274961659));
#59872=CARTESIAN_POINT('Ctrl Pts',(52.5495806928346,29.0989014953011,10.7833050713127));
#59873=CARTESIAN_POINT('Ctrl Pts',(52.5554097972367,29.195537660279,10.7782826464595));
#59874=CARTESIAN_POINT('Ctrl Pts',(52.5668780804804,29.2913210853217,10.7732602216063));
#59875=CARTESIAN_POINT('Ctrl Pts',(52.578489456825,29.3882996279791,10.7681751304994));
#59876=CARTESIAN_POINT('Ctrl Pts',(52.5958815310451,29.4844039715165,10.7630900393925));
#59877=CARTESIAN_POINT('Ctrl Pts',(52.6188909492805,29.5790249896004,10.7580049482857));
#59878=CARTESIAN_POINT('Ctrl Pts',(52.6323094394725,29.6342054896082,10.75503945631));
#59879=CARTESIAN_POINT('Ctrl Pts',(52.6476374345984,29.6888819236266,10.7520739643342));
#59880=CARTESIAN_POINT('Ctrl Pts',(52.6648351019657,29.7429368405111,10.7491084723585));
#59881=CARTESIAN_POINT('Ctrl Pts',(52.6893811439755,29.8200888305072,10.744875858187));
#59882=CARTESIAN_POINT('Ctrl Pts',(52.717800499929,29.8961665176382,10.7406432440155));
#59883=CARTESIAN_POINT('Ctrl Pts',(52.7499803883688,29.970753314326,10.736410629844));
#59884=CARTESIAN_POINT('Ctrl Pts',(52.7821143752193,30.0452337199517,10.7321840530992));
#59885=CARTESIAN_POINT('Ctrl Pts',(52.8179980583693,30.1182270358674,10.7279574763544));
#59886=CARTESIAN_POINT('Ctrl Pts',(52.8574690671919,30.189332355551,10.7237308996096));
#59887=CARTESIAN_POINT('Ctrl Pts',(52.8968962677652,30.2603587565634,10.7195090138756));
#59888=CARTESIAN_POINT('Ctrl Pts',(52.9399026584179,30.3295009208941,10.7152871281416));
#59889=CARTESIAN_POINT('Ctrl Pts',(52.9862786045282,30.3963797447038,10.7110652424076));
#59890=CARTESIAN_POINT('Ctrl Pts',(53.032623271501,30.4632134608209,10.7068462042045));
#59891=CARTESIAN_POINT('Ctrl Pts',(53.0823327161962,30.5277864875226,10.7026271660015));
#59892=CARTESIAN_POINT('Ctrl Pts',(53.1351530399975,30.5897471703921,10.6984081277985));
#59893=CARTESIAN_POINT('Ctrl Pts',(53.1879561146069,30.6516876191615,10.6941904673795));
#59894=CARTESIAN_POINT('Ctrl Pts',(53.2438677496658,30.7110170650421,10.6899728069605));
#59895=CARTESIAN_POINT('Ctrl Pts',(53.3025935296144,30.7674166244248,10.6857551465415));
#59896=CARTESIAN_POINT('Ctrl Pts',(53.3613180875018,30.823815010154,10.6815375738905));
#59897=CARTESIAN_POINT('Ctrl Pts',(53.4228563379765,30.8772833096742,10.6773200012394));
#59898=CARTESIAN_POINT('Ctrl Pts',(53.4868777839744,30.9275402484436,10.6731024285884));
#59899=CARTESIAN_POINT('Ctrl Pts',(53.551007909954,30.9778825011745,10.6688776963721));
#59900=CARTESIAN_POINT('Ctrl Pts',(53.6176292980807,31.0250021976902,10.6646529641558));
#59901=CARTESIAN_POINT('Ctrl Pts',(53.6863788393578,31.0686589125114,10.6604282319395));
#59902=CARTESIAN_POINT('Ctrl Pts',(53.7551112097162,31.1123047236105,10.6562045548944));
#59903=CARTESIAN_POINT('Ctrl Pts',(53.8259702543295,31.152489071163,10.6519808778493));
#59904=CARTESIAN_POINT('Ctrl Pts',(53.8985681831979,31.1890176342222,10.6477572008042));
#59905=CARTESIAN_POINT('Ctrl Pts',(53.9712978301646,31.2256124729031,10.6435258605279));
#59906=CARTESIAN_POINT('Ctrl Pts',(54.0457722403259,31.2585380831304,10.6392945202517));
#59907=CARTESIAN_POINT('Ctrl Pts',(54.1215828619718,31.2876480458363,10.6350631799754));
#59908=CARTESIAN_POINT('Ctrl Pts',(54.1971756025148,31.3166743459808,10.630844000648));
#59909=CARTESIAN_POINT('Ctrl Pts',(54.2740964257098,31.3419068389321,10.6266248213205));
#59910=CARTESIAN_POINT('Ctrl Pts',(54.351928510941,31.3632506416097,10.622405641993));
#59911=CARTESIAN_POINT('Ctrl Pts',(54.4300084315551,31.3846624078977,10.6181730278216));
#59912=CARTESIAN_POINT('Ctrl Pts',(54.5092958350579,31.40224028939,10.6139404136501));
#59913=CARTESIAN_POINT('Ctrl Pts',(54.5893798789632,31.415852099405,10.6097077994786));
#59914=CARTESIAN_POINT('Ctrl Pts',(54.6693496904995,31.4294444934512,10.6054812227338));
#59915=CARTESIAN_POINT('Ctrl Pts',(54.7501134313602,31.439081974809,10.601254645989));
#59916=CARTESIAN_POINT('Ctrl Pts',(54.8312464163408,31.4446824902228,10.5970280692442));
#59917=CARTESIAN_POINT('Ctrl Pts',(54.912289353103,31.4502767897131,10.5928061835102));
#59918=CARTESIAN_POINT('Ctrl Pts',(54.9937002585672,31.4518429943024,10.5885842977762));
#59919=CARTESIAN_POINT('Ctrl Pts',(55.075047005612,31.4493505663642,10.5843624120422));
#59920=CARTESIAN_POINT('Ctrl Pts',(55.1563388867985,31.4468598194914,10.5801433738391));
#59921=CARTESIAN_POINT('Ctrl Pts',(55.237566232377,31.44031589104,10.5759243356361));
#59922=CARTESIAN_POINT('Ctrl Pts',(55.3182958431399,31.4297403166264,10.5717052974331));
#59923=CARTESIAN_POINT('Ctrl Pts',(55.3989990905552,31.4191681958099,10.5674876370141));
#59924=CARTESIAN_POINT('Ctrl Pts',(55.4792044656936,31.4045671039895,10.5632699765952));
#59925=CARTESIAN_POINT('Ctrl Pts',(55.558484200871,31.3860104038703,10.5590523161762));
#59926=CARTESIAN_POINT('Ctrl Pts',(55.6377622862671,31.3674540899091,10.5548347435252));
#59927=CARTESIAN_POINT('Ctrl Pts',(55.7161143179457,31.3449424383288,10.5506171708741));
#59928=CARTESIAN_POINT('Ctrl Pts',(55.7931244328572,31.3185995523171,10.5463995982231));
#59929=CARTESIAN_POINT('Ctrl Pts',(55.8702652767418,31.2922119477844,10.5421748660068));
#59930=CARTESIAN_POINT('Ctrl Pts',(55.9460592042979,31.2619802475128,10.5379501337905));
#59931=CARTESIAN_POINT('Ctrl Pts',(56.0201068637376,31.2280781486643,10.5337254015742));
#59932=CARTESIAN_POINT('Ctrl Pts',(56.0941360289977,31.1941845172206,10.5295017245291));
#59933=CARTESIAN_POINT('Ctrl Pts',(56.1664193944902,31.1566225542158,10.525278047484));
#59934=CARTESIAN_POINT('Ctrl Pts',(56.2365828457144,31.1156117592047,10.5210543704389));
#59935=CARTESIAN_POINT('Ctrl Pts',(56.3068735980408,31.0745265562315,10.5168230301626));
#59936=CARTESIAN_POINT('Ctrl Pts',(56.3750363594652,31.0299802709464,10.5125916898864));
#59937=CARTESIAN_POINT('Ctrl Pts',(56.4407258940992,30.9822358961718,10.5083603496102));
#59938=CARTESIAN_POINT('Ctrl Pts',(56.5062266358189,30.9346287395965,10.5041411702826));
#59939=CARTESIAN_POINT('Ctrl Pts',(56.5692680456235,30.8838422020938,10.4999219909551));
#59940=CARTESIAN_POINT('Ctrl Pts',(56.6295436157121,30.8301742688859,10.4957028116276));
#59941=CARTESIAN_POINT('Ctrl Pts',(56.6900111171732,30.7763354445514,10.4914701974561));
#59942=CARTESIAN_POINT('Ctrl Pts',(56.747920014007,30.7193965831343,10.4872375832847));
#59943=CARTESIAN_POINT('Ctrl Pts',(56.8029357617094,30.6596303471404,10.4830049691132));
#59944=CARTESIAN_POINT('Ctrl Pts',(56.8578730346133,30.5999493620705,10.4787783923684));
#59945=CARTESIAN_POINT('Ctrl Pts',(56.9099250427466,30.5374493513981,10.4745518156236));
#59946=CARTESIAN_POINT('Ctrl Pts',(56.9587917588003,30.4724418819282,10.4703252388788));
#59947=CARTESIAN_POINT('Ctrl Pts',(57.0076042384578,30.4075065632217,10.4661033531448));
#59948=CARTESIAN_POINT('Ctrl Pts',(57.0532381729521,30.3400696849732,10.4618814674108));
#59949=CARTESIAN_POINT('Ctrl Pts',(57.0954326961982,30.2704771016053,10.4576595816767));
#59950=CARTESIAN_POINT('Ctrl Pts',(57.137598760547,30.2009314562767,10.4534405434737));
#59951=CARTESIAN_POINT('Ctrl Pts',(57.1763297806992,30.129233389725,10.4492215052707));
#59952=CARTESIAN_POINT('Ctrl Pts',(57.2114079872756,30.0557580043807,10.4450024670676));
#59953=CARTESIAN_POINT('Ctrl Pts',(57.2464747385885,29.9823066134184,10.4407848066487));
#59954=CARTESIAN_POINT('Ctrl Pts',(57.277890845314,29.9070794752191,10.4365671462297));
#59955=CARTESIAN_POINT('Ctrl Pts',(57.3054849688676,29.8304753508235,10.4323494858107));
#59956=CARTESIAN_POINT('Ctrl Pts',(57.333078518198,29.7538728205307,10.4281319131597));
#59957=CARTESIAN_POINT('Ctrl Pts',(57.3568500861601,29.6758937984692,10.4239143405086));
#59958=CARTESIAN_POINT('Ctrl Pts',(57.3766773774591,29.5969546829317,10.4196967678576));
#59959=CARTESIAN_POINT('Ctrl Pts',(57.396538326693,29.5178815638347,10.4154720356413));
#59960=CARTESIAN_POINT('Ctrl Pts',(57.4124414891092,29.4378455433135,10.411247303425));
#59961=CARTESIAN_POINT('Ctrl Pts',(57.424315158834,29.3572761685977,10.4070225712087));
#59962=CARTESIAN_POINT('Ctrl Pts',(57.4361858629852,29.2767269169283,10.4027988941636));
#59963=CARTESIAN_POINT('Ctrl Pts',(57.4440290632794,29.1956450434864,10.3985752171185));
#59964=CARTESIAN_POINT('Ctrl Pts',(57.4478252132447,29.1144638606878,10.3943515400734));
#59965=CARTESIAN_POINT('Ctrl Pts',(57.4516282507571,29.0331353867587,10.3901201997971));
#59966=CARTESIAN_POINT('Ctrl Pts',(57.4513695651493,28.9517077092808,10.3858888595209));
#59967=CARTESIAN_POINT('Ctrl Pts',(57.4470818147394,28.870613594331,10.3816575192447));
#59968=CARTESIAN_POINT('Ctrl Pts',(57.4428063874019,28.789752545339,10.3774383399172));
#59969=CARTESIAN_POINT('Ctrl Pts',(57.4345251528575,28.7092235884595,10.3732191605896));
#59970=CARTESIAN_POINT('Ctrl Pts',(57.4223212055342,28.6294460535637,10.3689999812621));
#59971=CARTESIAN_POINT('Ctrl Pts',(57.4100783980166,28.5494144885236,10.3647673670906));
#59972=CARTESIAN_POINT('Ctrl Pts',(57.3938422947662,28.4698414829047,10.3605347529192));
#59973=CARTESIAN_POINT('Ctrl Pts',(57.3736594856737,28.3911560987647,10.3563021387477));
#59974=CARTESIAN_POINT('Ctrl Pts',(57.3535054654632,28.3125829519369,10.3520755620029));
#59975=CARTESIAN_POINT('Ctrl Pts',(57.3294160349933,28.2348953581758,10.3478489852581));
#59976=CARTESIAN_POINT('Ctrl Pts',(57.301489209251,28.1585146051766,10.3436224085133));
#59977=CARTESIAN_POINT('Ctrl Pts',(57.2735933790515,28.0822186259686,10.3394005227793));
#59978=CARTESIAN_POINT('Ctrl Pts',(57.2418687750507,28.0072270395985,10.3351786370453));
#59979=CARTESIAN_POINT('Ctrl Pts',(57.2064634929563,27.9339469505456,10.3309567513112));
#59980=CARTESIAN_POINT('Ctrl Pts',(57.1710820906267,27.8607162866402,10.3267377131082));
#59981=CARTESIAN_POINT('Ctrl Pts',(57.1320251422449,27.7891952446147,10.3225186749052));
#59982=CARTESIAN_POINT('Ctrl Pts',(57.089488739367,27.7197707009841,10.3182996367022));
#59983=CARTESIAN_POINT('Ctrl Pts',(57.0469662273274,27.6503688288784,10.3140819762832));
#59984=CARTESIAN_POINT('Ctrl Pts',(57.000966759851,27.5830624913214,10.3098643158642));
#59985=CARTESIAN_POINT('Ctrl Pts',(56.9517315508951,27.5182124972721,10.3056466554453));
#59986=CARTESIAN_POINT('Ctrl Pts',(56.9024973665053,27.4533638527268,10.3014290827942));
#59987=CARTESIAN_POINT('Ctrl Pts',(56.8500278563562,27.3909718193431,10.2972115101432));
#59988=CARTESIAN_POINT('Ctrl Pts',(56.7946057281832,27.3313656690658,10.2929939374921));
#59989=CARTESIAN_POINT('Ctrl Pts',(56.7390895178508,27.2716583340179,10.2887692052759));
#59990=CARTESIAN_POINT('Ctrl Pts',(56.6806109791777,27.2147466860857,10.2845444730596));
#59991=CARTESIAN_POINT('Ctrl Pts',(56.6194913904811,27.1609247198231,10.2803197408433));
#59992=CARTESIAN_POINT('Ctrl Pts',(56.5583870670427,27.1071161961611,10.2760960637982));
#59993=CARTESIAN_POINT('Ctrl Pts',(56.4946433906778,27.0563960846154,10.2718723867531));
#59994=CARTESIAN_POINT('Ctrl Pts',(56.4286131936573,27.0090166768884,10.267648709708));
#59995=CARTESIAN_POINT('Ctrl Pts',(56.3624631947068,26.9615513063029,10.2634173694317));
#59996=CARTESIAN_POINT('Ctrl Pts',(56.2940187759755,26.9174390050455,10.2591860291555));
#59997=CARTESIAN_POINT('Ctrl Pts',(56.2236607317809,26.8768879766962,10.2549546888792));
#59998=CARTESIAN_POINT('Ctrl Pts',(56.1535048978822,26.8364534927382,10.2507355095517));
#59999=CARTESIAN_POINT('Ctrl Pts',(56.0814468665521,26.7995599721353,10.2465163302242));
#60000=CARTESIAN_POINT('Ctrl Pts',(56.0078836189387,26.7663659967051,10.2422971508967));
#60001=CARTESIAN_POINT('Ctrl Pts',(55.9340861289105,26.7330663239707,10.2380645367252));
#60002=CARTESIAN_POINT('Ctrl Pts',(55.8584993366765,26.7033659685561,10.2338319225538));
#60003=CARTESIAN_POINT('Ctrl Pts',(55.7815085138889,26.6774594314159,10.2295993083823));
#60004=CARTESIAN_POINT('Ctrl Pts',(55.7046275112808,26.6515898475183,10.2253727316375));
#60005=CARTESIAN_POINT('Ctrl Pts',(55.626346892407,26.62950348083,10.2211461548927));
#60006=CARTESIAN_POINT('Ctrl Pts',(55.5470734034523,26.6113474632682,10.2169195781479));
#60007=CARTESIAN_POINT('Ctrl Pts',(55.4678878988907,26.5932115967835,10.2126976924139));
#60008=CARTESIAN_POINT('Ctrl Pts',(55.3877121644035,26.5789975148659,10.2084758066798));
#60009=CARTESIAN_POINT('Ctrl Pts',(55.3069683129208,26.5688026191067,10.2042539209458));
#60010=CARTESIAN_POINT('Ctrl Pts',(55.2262789206621,26.5586145994885,10.2000348827428));
#60011=CARTESIAN_POINT('Ctrl Pts',(55.1450226321312,26.5524404401531,10.1958158445398));
#60012=CARTESIAN_POINT('Ctrl Pts',(55.0636307215102,26.5503262704433,10.1915968063367));
#60013=CARTESIAN_POINT('Ctrl Pts',(54.9822653905197,26.5482127911443,10.1873791459178));
#60014=CARTESIAN_POINT('Ctrl Pts',(54.9007649894306,26.550156680478,10.1831614854988));
#60015=CARTESIAN_POINT('Ctrl Pts',(54.8195634909725,26.5561520267803,10.1789438250798));
#60016=CARTESIAN_POINT('Ctrl Pts',(54.7383636822869,26.5621472483217,10.1747262524288));
#60017=CARTESIAN_POINT('Ctrl Pts',(54.6574632270658,26.572193723826,10.1705086797777));
#60018=CARTESIAN_POINT('Ctrl Pts',(54.5772922332422,26.5862335668249,10.1662911071267));
#60019=CARTESIAN_POINT('Ctrl Pts',(54.4969851446769,26.6002972432419,10.1620663749104));
#60020=CARTESIAN_POINT('Ctrl Pts',(54.4174104550551,26.6183677697227,10.1578416426941));
#60021=CARTESIAN_POINT('Ctrl Pts',(54.3389896786002,26.6403357007822,10.1536169104778));
#60022=CARTESIAN_POINT('Ctrl Pts',(54.2605884885567,26.6622981451206,10.1493932334327));
#60023=CARTESIAN_POINT('Ctrl Pts',(54.1833410706479,26.6881558793239,10.1451695563876));
#60024=CARTESIAN_POINT('Ctrl Pts',(54.107651135691,26.7177502865886,10.1409458793425));
#60025=CARTESIAN_POINT('Ctrl Pts',(54.0318238726525,26.7473983884849,10.1367145390662));
#60026=CARTESIAN_POINT('Ctrl Pts',(53.9575601647771,26.7807965212213,10.13248319879));
#60027=CARTESIAN_POINT('Ctrl Pts',(53.8852419632136,26.8177386111146,10.1282518585138));
#60028=CARTESIAN_POINT('Ctrl Pts',(53.8131316054736,26.8545745287712,10.1240326791862));
#60029=CARTESIAN_POINT('Ctrl Pts',(53.7429559393099,26.8949337609263,10.1198134998587));
#60030=CARTESIAN_POINT('Ctrl Pts',(53.6750641040087,26.9385696418473,10.1155943205312));
#60031=CARTESIAN_POINT('Ctrl Pts',(53.6069560853829,26.9823444695174,10.1113617063597));
#60032=CARTESIAN_POINT('Ctrl Pts',(53.5408931673629,27.0295796802682,10.1071290921883));
#60033=CARTESIAN_POINT('Ctrl Pts',(53.4772482444542,27.0800579849948,10.1028964780168));
#60034=CARTESIAN_POINT('Ctrl Pts',(53.413694105052,27.1304642871594,10.098669901272));
#60035=CARTESIAN_POINT('Ctrl Pts',(53.3525514714623,27.1841042092555,10.0944433245272));
#60036=CARTESIAN_POINT('Ctrl Pts',(53.2941651945998,27.2407166610562,10.0902167477824));
#60037=CARTESIAN_POINT('Ctrl Pts',(53.2358437197436,27.297266279591,10.0859948620484));
#60038=CARTESIAN_POINT('Ctrl Pts',(53.180272854749,27.3567815506487,10.0817729763144));
#60039=CARTESIAN_POINT('Ctrl Pts',(53.1277641011473,27.4189614207594,10.0775510905803));
#60040=CARTESIAN_POINT('Ctrl Pts',(53.0752907630715,27.481099352476,10.0733320523773));
#60041=CARTESIAN_POINT('Ctrl Pts',(53.0258757334726,27.5458979598612,10.0691130141743));
#60042=CARTESIAN_POINT('Ctrl Pts',(52.9797924928195,27.6130205921026,10.0648939759713));
#60043=CARTESIAN_POINT('Ctrl Pts',(52.9337243012726,27.6801213045395,10.0606763155523));
#60044=CARTESIAN_POINT('Ctrl Pts',(52.8909860006212,27.7495441519376,10.0564586551333));
#60045=CARTESIAN_POINT('Ctrl Pts',(52.8518088871162,27.8209218887084,10.0522409947144));
#60046=CARTESIAN_POINT('Ctrl Pts',(52.812632588872,27.8922981401356,10.0480234220633));
#60047=CARTESIAN_POINT('Ctrl Pts',(52.777017552922,27.9656287922486,10.0438058494123));
#60048=CARTESIAN_POINT('Ctrl Pts',(52.7451493737418,28.0405215462227,10.0395882767612));
#60049=CARTESIAN_POINT('Ctrl Pts',(52.7132270965467,28.1155414348316,10.035363544545));
#60050=CARTESIAN_POINT('Ctrl Pts',(52.685064584843,28.1921283011353,10.0311388123287));
#60051=CARTESIAN_POINT('Ctrl Pts',(52.6607995056797,28.2698689861594,10.0269140801124));
#60052=CARTESIAN_POINT('Ctrl Pts',(52.6365404869745,28.3475902546322,10.0226904030673));
#60053=CARTESIAN_POINT('Ctrl Pts',(52.6161770501565,28.4264643088748,10.0184667260222));
#60054=CARTESIAN_POINT('Ctrl Pts',(52.5997959239436,28.5060661549535,10.014243048977));
#60055=CARTESIAN_POINT('Ctrl Pts',(52.5833850766241,28.5858124266921,10.0100117087008));
#60056=CARTESIAN_POINT('Ctrl Pts',(52.5709710504681,28.6662886687285,10.0057803684246));
#60057=CARTESIAN_POINT('Ctrl Pts',(52.562588920185,28.7470623041239,10.0015490281483));
#60058=CARTESIAN_POINT('Ctrl Pts',(52.5542308802965,28.8276037946254,9.99732984882081));
#60059=CARTESIAN_POINT('Ctrl Pts',(52.5498815331473,28.9084405122791,9.99311066949331));
#60060=CARTESIAN_POINT('Ctrl Pts',(52.5495240410073,28.9891453052202,9.9888914901658));
#60061=CARTESIAN_POINT('Ctrl Pts',(52.5495081118901,28.9927413454074,9.98870349218122));
#60062=CARTESIAN_POINT('Ctrl Pts',(52.5495000984775,28.9963374206841,9.98851549419664));
#60063=CARTESIAN_POINT('Ctrl Pts',(52.5495000009021,28.999933508713,9.98832749621206));
#60064=CARTESIAN_POINT('',(52.5495007901279,28.9980321543788,9.18832749626153));
#60065=CARTESIAN_POINT('Ctrl Pts',(52.5495000009021,28.9999335093135,9.98832749618066));
#60066=CARTESIAN_POINT('Ctrl Pts',(52.5494978058378,29.0808321322443,9.98409823984876));
#60067=CARTESIAN_POINT('Ctrl Pts',(52.5535059878827,29.1618824777843,9.97986898351686));
#60068=CARTESIAN_POINT('Ctrl Pts',(52.5615436641983,29.2426539684173,9.97563972718495));
#60069=CARTESIAN_POINT('Ctrl Pts',(52.569569873288,29.3233102236385,9.97141650466635));
#60070=CARTESIAN_POINT('Ctrl Pts',(52.5816141135454,29.4036879548487,9.96719328214775));
#60071=CARTESIAN_POINT('Ctrl Pts',(52.5976434925847,29.4833564536443,9.96297005962915));
#60072=CARTESIAN_POINT('Ctrl Pts',(52.613654441598,29.5629333523532,9.95875169282585));
#60073=CARTESIAN_POINT('Ctrl Pts',(52.633641331911,29.6418021853624,9.95453332602254));
#60074=CARTESIAN_POINT('Ctrl Pts',(52.6575196292917,29.7195387153213,9.95031495921924));
#60075=CARTESIAN_POINT('Ctrl Pts',(52.6813828891315,29.7972262901045,9.94609924896478));
#60076=CARTESIAN_POINT('Ctrl Pts',(52.7091325551766,29.8737825336235,9.94188353871032));
#60077=CARTESIAN_POINT('Ctrl Pts',(52.7406335763444,29.9487958756537,9.93766782845585));
#60078=CARTESIAN_POINT('Ctrl Pts',(52.7721244336861,30.0237850145779,9.93345347840319));
#60079=CARTESIAN_POINT('Ctrl Pts',(52.8073640624274,30.0972318118537,9.92923912835052));
#60080=CARTESIAN_POINT('Ctrl Pts',(52.8461688640155,30.1687436364163,9.92502477829785));
#60081=CARTESIAN_POINT('Ctrl Pts',(52.8849730622045,30.2402543489988,9.92081049377664));
#60082=CARTESIAN_POINT('Ctrl Pts',(52.9273420999318,30.3098297402525,9.91659620925541));
#60083=CARTESIAN_POINT('Ctrl Pts',(52.9730465961936,30.3771020836516,9.9123819247342));
#60084=CARTESIAN_POINT('Ctrl Pts',(53.0187960794113,30.4444406432481,9.90816349209086));
#60085=CARTESIAN_POINT('Ctrl Pts',(53.067887317589,30.5094712406044,9.90394505944751));
#60086=CARTESIAN_POINT('Ctrl Pts',(53.1200480822684,30.5718559212018,9.89972662680417));
#60087=CARTESIAN_POINT('Ctrl Pts',(53.1722334319942,30.6342700057062,9.89550620587781));
#60088=CARTESIAN_POINT('Ctrl Pts',(53.227490874146,30.6940353467502,9.89128578495145));
#60089=CARTESIAN_POINT('Ctrl Pts',(53.2855101318628,30.7508497200088,9.88706536402509));
#60090=CARTESIAN_POINT('Ctrl Pts',(53.3436339422809,30.8077664747253,9.88283733775483));
#60091=CARTESIAN_POINT('Ctrl Pts',(53.4045291642281,30.8617213258825,9.87860931148456));
#60092=CARTESIAN_POINT('Ctrl Pts',(53.467851266408,30.9124514394233,9.87438128521429));
#60093=CARTESIAN_POINT('Ctrl Pts',(53.5287199099901,30.961215979666,9.87031707674297));
#60094=CARTESIAN_POINT('Ctrl Pts',(53.5918304998814,31.0070008999972,9.86625286827166));
#60095=CARTESIAN_POINT('Ctrl Pts',(53.6568537203743,31.0496117489729,9.86218865980035));
#60096=CARTESIAN_POINT('Ctrl Pts',(53.7245712615576,31.0939882332272,9.85795604562887));
#60097=CARTESIAN_POINT('Ctrl Pts',(53.7946163414348,31.1350876378089,9.85372343145738));
#60098=CARTESIAN_POINT('Ctrl Pts',(53.8666386434207,31.1726578850369,9.8494908172859));
#60099=CARTESIAN_POINT('Ctrl Pts',(53.9385582123553,31.2101745418348,9.84526424054112));
#60100=CARTESIAN_POINT('Ctrl Pts',(54.0124489934216,31.2441718264052,9.84103766379634));
#60101=CARTESIAN_POINT('Ctrl Pts',(54.0879320867521,31.274441111927,9.83681108705155));
#60102=CARTESIAN_POINT('Ctrl Pts',(54.1633314025899,31.304676802047,9.83258920131752));
#60103=CARTESIAN_POINT('Ctrl Pts',(54.2403190901064,31.3311925425831,9.8283673155835));
#60104=CARTESIAN_POINT('Ctrl Pts',(54.3184933321552,31.3538264404333,9.82414542984947));
#60105=CARTESIAN_POINT('Ctrl Pts',(54.3966148481019,31.3764450724214,9.81992639164645));
#60106=CARTESIAN_POINT('Ctrl Pts',(54.4759208840565,31.3951869328009,9.81570735344342));
#60107=CARTESIAN_POINT('Ctrl Pts',(54.5559925955995,31.4099393508629,9.8114883152404));
#60108=CARTESIAN_POINT('Ctrl Pts',(54.6360381586408,31.4246869513231,9.80727065482143));
#60109=CARTESIAN_POINT('Ctrl Pts',(54.716848444194,31.4354476126523,9.80305299440246));
#60110=CARTESIAN_POINT('Ctrl Pts',(54.7979938449502,31.442159651481,9.7988353339835));
#60111=CARTESIAN_POINT('Ctrl Pts',(54.8791375571012,31.4488715506348,9.79461776133245));
#60112=CARTESIAN_POINT('Ctrl Pts',(54.9606159075262,31.4515349576749,9.7904001886814));
#60113=CARTESIAN_POINT('Ctrl Pts',(55.0419950197388,31.4501401323837,9.78618261603036));
#60114=CARTESIAN_POINT('Ctrl Pts',(55.1235122775416,31.4487429392986,9.78195788381407));
#60115=CARTESIAN_POINT('Ctrl Pts',(55.2049294931523,31.4432737384524,9.77773315159778));
#60116=CARTESIAN_POINT('Ctrl Pts',(55.2858132569215,31.4337750578408,9.77350841938149));
#60117=CARTESIAN_POINT('Ctrl Pts',(55.3666768191224,31.4242787496243,9.76928474233638));
#60118=CARTESIAN_POINT('Ctrl Pts',(55.447006739762,31.4107550725452,9.76506106529126));
#60119=CARTESIAN_POINT('Ctrl Pts',(55.5263795450707,31.393297897156,9.76083738824615));
#60120=CARTESIAN_POINT('Ctrl Pts',(55.6058963604791,31.3758090483295,9.75660604796991));
#60121=CARTESIAN_POINT('Ctrl Pts',(55.6844521406715,31.3543725613023,9.75237470769367));
#60122=CARTESIAN_POINT('Ctrl Pts',(55.761637522592,31.3291325711904,9.74814336741743));
#60123=CARTESIAN_POINT('Ctrl Pts',(55.8386010723243,31.303965121268,9.74392418808991));
#60124=CARTESIAN_POINT('Ctrl Pts',(55.9142016949616,31.2750162422132,9.7397050087624));
#60125=CARTESIAN_POINT('Ctrl Pts',(55.9880561238729,31.2424752721217,9.73548582943489));
#60126=CARTESIAN_POINT('Ctrl Pts',(56.0621457223876,31.2098306840463,9.7312532152634));
#60127=CARTESIAN_POINT('Ctrl Pts',(56.1347535377424,31.1734496529806,9.72702060109192));
#60128=CARTESIAN_POINT('Ctrl Pts',(56.2054774081875,31.1334888020212,9.72278798692043));
#60129=CARTESIAN_POINT('Ctrl Pts',(56.2761003976719,31.0935849514636,9.71856141017565));
#60130=CARTESIAN_POINT('Ctrl Pts',(56.3448443784209,31.0501116493631,9.71433483343087));
#60131=CARTESIAN_POINT('Ctrl Pts',(56.4113280756007,31.0032731498778,9.71010825668609));
#60132=CARTESIAN_POINT('Ctrl Pts',(56.4777379835754,30.956486635703,9.70588637095206));
#60133=CARTESIAN_POINT('Ctrl Pts',(56.5418922148169,30.9063426117408,9.70166448521803));
#60134=CARTESIAN_POINT('Ctrl Pts',(56.6034362197288,30.8530899976153,9.69744259948401));
#60135=CARTESIAN_POINT('Ctrl Pts',(56.6649387151179,30.7998733007266,9.69322356128098));
#60136=CARTESIAN_POINT('Ctrl Pts',(56.7238341303281,30.7435524809836,9.68900452307796));
#60137=CARTESIAN_POINT('Ctrl Pts',(56.7797999350869,30.6844175376268,9.68478548487493));
#60138=CARTESIAN_POINT('Ctrl Pts',(56.8357474634543,30.6253019055865,9.68056782445596));
#60139=CARTESIAN_POINT('Ctrl Pts',(56.8887669622505,30.5633743121338,9.67635016403699));
#60140=CARTESIAN_POINT('Ctrl Pts',(56.9385728113438,30.4989615422414,9.67213250361803));
#60141=CARTESIAN_POINT('Ctrl Pts',(56.9883776239961,30.4345501127544,9.66791493096698));
#60142=CARTESIAN_POINT('Ctrl Pts',(57.0349686366767,30.3676539778703,9.66369735831594));
#60143=CARTESIAN_POINT('Ctrl Pts',(57.0781014763362,30.2986317815491,9.6594797856649));
#60144=CARTESIAN_POINT('Ctrl Pts',(57.1213075364012,30.2294924161929,9.65525505344861));
#60145=CARTESIAN_POINT('Ctrl Pts',(57.1610434305799,30.1582201644429,9.65103032123232));
#60146=CARTESIAN_POINT('Ctrl Pts',(57.1971088838655,30.0852017335222,9.64680558901603));
#60147=CARTESIAN_POINT('Ctrl Pts',(57.2331653294258,30.0122015397203,9.64258191197092));
#60148=CARTESIAN_POINT('Ctrl Pts',(57.2655530014879,29.9374564750665,9.63835823492581));
#60149=CARTESIAN_POINT('Ctrl Pts',(57.2941201015777,29.8613728632464,9.6341345578807));
#60150=CARTESIAN_POINT('Ctrl Pts',(57.3227390324036,29.7851512090768,9.62990321760446));
#60151=CARTESIAN_POINT('Ctrl Pts',(57.3475233963717,29.7075865980716,9.62567187732821));
#60152=CARTESIAN_POINT('Ctrl Pts',(57.3683712400756,29.6291008815624,9.62144053705197));
#60153=CARTESIAN_POINT('Ctrl Pts',(57.3891591666985,29.5508407344265,9.61722135772446));
#60154=CARTESIAN_POINT('Ctrl Pts',(57.4060331565599,29.4716652318527,9.61300217839695));
#60155=CARTESIAN_POINT('Ctrl Pts',(57.4189433805684,29.3919989433716,9.60878299906944));
#60156=CARTESIAN_POINT('Ctrl Pts',(57.4318947137196,29.3120789789805,9.60455038489796));
#60157=CARTESIAN_POINT('Ctrl Pts',(57.4409051402828,29.231367849109,9.60031777072648));
#60158=CARTESIAN_POINT('Ctrl Pts',(57.4458871024818,29.1502881629185,9.596085156555));
#60159=CARTESIAN_POINT('Ctrl Pts',(57.4508619583795,29.0693241292871,9.59185857981021));
#60160=CARTESIAN_POINT('Ctrl Pts',(57.4518197344045,28.9879930432876,9.58763200306542));
#60161=CARTESIAN_POINT('Ctrl Pts',(57.4487241977703,28.9067259239975,9.58340542632063));
#60162=CARTESIAN_POINT('Ctrl Pts',(57.4456320968234,28.8255490017993,9.5791835405866));
#60163=CARTESIAN_POINT('Ctrl Pts',(57.4384956397333,28.7444363671145,9.57496165485257));
#60164=CARTESIAN_POINT('Ctrl Pts',(57.4273306094741,28.663820937133,9.57073976911855));
#60165=CARTESIAN_POINT('Ctrl Pts',(57.4161731096816,28.583259879759,9.56652073091552));
#60166=CARTESIAN_POINT('Ctrl Pts',(57.4009924967785,28.5031958200244,9.5623016927125));
#60167=CARTESIAN_POINT('Ctrl Pts',(57.3818564437034,28.4240571802786,9.55808265450948));
#60168=CARTESIAN_POINT('Ctrl Pts',(57.3627266397655,28.3449443843274,9.55386499409051));
#60169=CARTESIAN_POINT('Ctrl Pts',(57.3396440699972,28.2667568593869,9.54964733367155));
#60170=CARTESIAN_POINT('Ctrl Pts',(57.3127273580472,28.1899120928318,9.54542967325259));
#60171=CARTESIAN_POINT('Ctrl Pts',(57.2858112062238,28.1130689253872,9.54121210060154));
#60172=CARTESIAN_POINT('Ctrl Pts',(57.2550612255348,28.0375688988133,9.5369945279505));
#60173=CARTESIAN_POINT('Ctrl Pts',(57.2206452186966,27.9638122454497,9.53277695529945));
#60174=CARTESIAN_POINT('Ctrl Pts',(57.1861707887636,27.8899303860456,9.52855222308317));
#60175=CARTESIAN_POINT('Ctrl Pts',(57.14801807881,27.8177982442578,9.52432749086688));
#60176=CARTESIAN_POINT('Ctrl Pts',(57.1064024387348,27.7477943395385,9.52010275865059));
#60177=CARTESIAN_POINT('Ctrl Pts',(57.0647971926022,27.6778079190285,9.51587908160548));
#60178=CARTESIAN_POINT('Ctrl Pts',(57.01973102153,27.6099490491839,9.51165540456037));
#60179=CARTESIAN_POINT('Ctrl Pts',(56.9714621208644,27.5445662653363,9.50743172751526));
#60180=CARTESIAN_POINT('Ctrl Pts',(56.9231056434881,27.4790648541933,9.50320038723902));
#60181=CARTESIAN_POINT('Ctrl Pts',(56.8715351187498,27.4160488676827,9.49896904696278));
#60182=CARTESIAN_POINT('Ctrl Pts',(56.8170489026719,27.3558334830989,9.49473770668654));
#60183=CARTESIAN_POINT('Ctrl Pts',(56.7627192809676,27.2957911586229,9.49051852735902));
#60184=CARTESIAN_POINT('Ctrl Pts',(56.7054910857013,27.2385336228024,9.48629934803151));
#60185=CARTESIAN_POINT('Ctrl Pts',(56.6456933295085,27.1843338095312,9.48208016870399));
#60186=CARTESIAN_POINT('Ctrl Pts',(56.5857051634132,27.1299614115042,9.47784755453251));
#60187=CARTESIAN_POINT('Ctrl Pts',(56.5229079150301,27.0784640342167,9.47361494036103));
#60188=CARTESIAN_POINT('Ctrl Pts',(56.4576084130609,27.0301451921083,9.46938232618954));
#60189=CARTESIAN_POINT('Ctrl Pts',(56.3924020546999,26.9818952722912,9.46515574944476));
#60190=CARTESIAN_POINT('Ctrl Pts',(56.3247009020312,26.9368151568067,9.46092917269997));
#60191=CARTESIAN_POINT('Ctrl Pts',(56.2548467795724,26.8951698857635,9.45670259595518));
#60192=CARTESIAN_POINT('Ctrl Pts',(56.1850701871006,26.8535708361487,9.45248071022115));
#60193=CARTESIAN_POINT('Ctrl Pts',(56.1131457698716,26.8153992926695,9.44825882448713));
#60194=CARTESIAN_POINT('Ctrl Pts',(56.0394452620096,26.7808776966364,9.4440369387531));
#60195=CARTESIAN_POINT('Ctrl Pts',(55.9657944628546,26.7463793843492,9.43981790055008));
#60196=CARTESIAN_POINT('Ctrl Pts',(55.8903703718364,26.7155263267475,9.43559886234706));
#60197=CARTESIAN_POINT('Ctrl Pts',(55.813569201632,26.6884949915356,9.43137982414403));
#60198=CARTESIAN_POINT('Ctrl Pts',(55.7367931118897,26.6614724837724,9.42716216372507));
#60199=CARTESIAN_POINT('Ctrl Pts',(55.6586412739084,26.63826937399,9.4229445033061));
#60200=CARTESIAN_POINT('Ctrl Pts',(55.57952846544,26.6190134381428,9.41872684288714));
#60201=CARTESIAN_POINT('Ctrl Pts',(55.5004173032792,26.5997579030042,9.41450927023609));
#60202=CARTESIAN_POINT('Ctrl Pts',(55.4203456620391,26.5844494872086,9.41029169758504));
#60203=CARTESIAN_POINT('Ctrl Pts',(55.3397406186372,26.5731653204126,9.40607412493399));
#60204=CARTESIAN_POINT('Ctrl Pts',(55.2589987436701,26.561861998113,9.40184939271771));
#60205=CARTESIAN_POINT('Ctrl Pts',(55.1777221173716,26.5545966575692,9.39762466050142));
#60206=CARTESIAN_POINT('Ctrl Pts',(55.0963454880657,26.5513947241482,9.39339992828513));
#60207=CARTESIAN_POINT('Ctrl Pts',(55.0149891834263,26.5481935904436,9.38917625124002));
#60208=CARTESIAN_POINT('Ctrl Pts',(54.9335333916301,26.5490538081861,9.3849525741949));
#60209=CARTESIAN_POINT('Ctrl Pts',(54.8524110346605,26.5539485395213,9.38072889714979));
#60210=CARTESIAN_POINT('Ctrl Pts',(54.771141493291,26.5588521516154,9.37649755687354));
#60211=CARTESIAN_POINT('Ctrl Pts',(54.6902070588287,26.5678048548927,9.3722662165973));
#60212=CARTESIAN_POINT('Ctrl Pts',(54.6100345351985,26.5807279635679,9.36803487632105));
#60213=CARTESIAN_POINT('Ctrl Pts',(54.530092428856,26.5936139309943,9.36381569699355));
#60214=CARTESIAN_POINT('Ctrl Pts',(54.4509082877067,26.6104473362374,9.35959651766604));
#60215=CARTESIAN_POINT('Ctrl Pts',(54.3728901703299,26.6311007806301,9.35537733833854));
#60216=CARTESIAN_POINT('Ctrl Pts',(54.2946236252016,26.6518199903724,9.35114472416706));
#60217=CARTESIAN_POINT('Ctrl Pts',(54.2172394533364,26.6764606928121,9.34691210999558));
#60218=CARTESIAN_POINT('Ctrl Pts',(54.1411592880959,26.7049307457996,9.3426794958241));
#60219=CARTESIAN_POINT('Ctrl Pts',(54.0651876440677,26.7333601889296,9.33845291907931));
#60220=CARTESIAN_POINT('Ctrl Pts',(53.9905167438469,26.7656079724965,9.33422634233453));
#60221=CARTESIAN_POINT('Ctrl Pts',(53.9175549993061,26.8015316535204,9.32999976558974));
#60222=CARTESIAN_POINT('Ctrl Pts',(53.8446742338529,26.8374154634183,9.32577787985571));
#60223=CARTESIAN_POINT('Ctrl Pts',(53.7734992694838,26.8769668600102,9.32155599412169));
#60224=CARTESIAN_POINT('Ctrl Pts',(53.7044190679385,26.9199951205637,9.31733410838766));
#60225=CARTESIAN_POINT('Ctrl Pts',(53.6353854588469,26.9629943598899,9.31311507018463));
#60226=CARTESIAN_POINT('Ctrl Pts',(53.5684441998257,27.0094655607562,9.30889603198161));
#60227=CARTESIAN_POINT('Ctrl Pts',(53.503959014938,27.0591724391346,9.30467699377858));
#60228=CARTESIAN_POINT('Ctrl Pts',(53.4394948885609,27.1088630850585,9.30045933335962));
#60229=CARTESIAN_POINT('Ctrl Pts',(53.3774856111131,27.1617870266523,9.29624167294066));
#60230=CARTESIAN_POINT('Ctrl Pts',(53.318264169631,27.217665899206,9.2920240125217));
#60231=CARTESIAN_POINT('Ctrl Pts',(53.2590439605247,27.2735436089417,9.28780643987066));
#60232=CARTESIAN_POINT('Ctrl Pts',(53.2026118091136,27.3323758077121,9.28358886721961));
#60233=CARTESIAN_POINT('Ctrl Pts',(53.1492649147178,27.3938462420722,9.27937129456856));
#60234=CARTESIAN_POINT('Ctrl Pts',(53.095827460988,27.4554210259295,9.27514656235227));
#60235=CARTESIAN_POINT('Ctrl Pts',(53.0454860491666,27.5196426532177,9.27092183013599));
#60236=CARTESIAN_POINT('Ctrl Pts',(52.9984986840313,27.586160287665,9.2666970979197));
#60237=CARTESIAN_POINT('Ctrl Pts',(52.9515230544833,27.6526613086354,9.26247342087459));
#60238=CARTESIAN_POINT('Ctrl Pts',(52.907900028098,27.7214567849452,9.25824974382948));
#60239=CARTESIAN_POINT('Ctrl Pts',(52.867842775683,27.7921689601633,9.25402606678437));
#60240=CARTESIAN_POINT('Ctrl Pts',(52.8277128453667,27.8630094320616,9.24979472650813));
#60241=CARTESIAN_POINT('Ctrl Pts',(52.7911618273533,27.935773136337,9.24556338623189));
#60242=CARTESIAN_POINT('Ctrl Pts',(52.7583560704221,28.0100592224852,9.24133204595565));
#60243=CARTESIAN_POINT('Ctrl Pts',(52.7256445978314,28.0841318090742,9.23711286662813));
#60244=CARTESIAN_POINT('Ctrl Pts',(52.6966569725273,28.1597175836678,9.23289368730061));
#60245=CARTESIAN_POINT('Ctrl Pts',(52.6715084767136,28.2364049004982,9.22867450797309));
#60246=CARTESIAN_POINT('Ctrl Pts',(52.6414535836778,28.328053686239,9.22363217922602));
#60247=CARTESIAN_POINT('Ctrl Pts',(52.6167895085714,28.4215518952709,9.21858985047894));
#60248=CARTESIAN_POINT('Ctrl Pts',(52.5977094991824,28.5163155990923,9.21354752173187));
#60249=CARTESIAN_POINT('Ctrl Pts',(52.5788396119689,28.6100356998838,9.20856072257414));
#60250=CARTESIAN_POINT('Ctrl Pts',(52.5654315328359,28.7049935042304,9.20357392341642));
#60251=CARTESIAN_POINT('Ctrl Pts',(52.5576258895964,28.8006035235255,9.1985871242587));
#60252=CARTESIAN_POINT('Ctrl Pts',(52.5522728903824,28.8661715161226,9.19516724825964));
#60253=CARTESIAN_POINT('Ctrl Pts',(52.5495537797068,28.9320458190386,9.19174737226059));
#60254=CARTESIAN_POINT('Ctrl Pts',(52.5495007901279,28.9980321543788,9.18832749626153));
#60255=CARTESIAN_POINT('',(52.5495005111529,29.0015827696721,8.38832749618323));
#60256=CARTESIAN_POINT('Ctrl Pts',(52.5495007901272,28.9980321553333,9.18832749621206));
#60257=CARTESIAN_POINT('Ctrl Pts',(52.5494356333114,29.0791700257587,9.18412236109965));
#60258=CARTESIAN_POINT('Ctrl Pts',(52.5534045814512,29.1603656797671,9.17991722598724));
#60259=CARTESIAN_POINT('Ctrl Pts',(52.5613981666387,29.241187371823,9.17571209087484));
#60260=CARTESIAN_POINT('Ctrl Pts',(52.5693897025857,29.3219883443796,9.17150803379349));
#60261=CARTESIAN_POINT('Ctrl Pts',(52.5814037806911,29.402415080424,9.16730397671214));
#60262=CARTESIAN_POINT('Ctrl Pts',(52.5973789763346,29.4820399015032,9.16309991963079));
#60263=CARTESIAN_POINT('Ctrl Pts',(52.613355033272,29.5616690155106,9.15889563589004));
#60264=CARTESIAN_POINT('Ctrl Pts',(52.6332925383797,29.6404956706803,9.15469135214927));
#60265=CARTESIAN_POINT('Ctrl Pts',(52.6570790391625,29.7181027929679,9.15048706840852));
#60266=CARTESIAN_POINT('Ctrl Pts',(52.6808909100591,29.7957926891591,9.14627830047911));
#60267=CARTESIAN_POINT('Ctrl Pts',(52.7085598373744,29.8722600070486,9.1420695325497));
#60268=CARTESIAN_POINT('Ctrl Pts',(52.7399237536216,29.947103801363,9.13786076462029));
#60269=CARTESIAN_POINT('Ctrl Pts',(52.771304532971,30.0219878361418,9.13364973380753));
#60270=CARTESIAN_POINT('Ctrl Pts',(52.806384054545,30.095246187559,9.12943870299477));
#60271=CARTESIAN_POINT('Ctrl Pts',(52.8449535347726,30.1665011713286,9.12522767218202));
#60272=CARTESIAN_POINT('Ctrl Pts',(52.883593346088,30.237886087897,9.12100896259382));
#60273=CARTESIAN_POINT('Ctrl Pts',(52.9257355850283,30.3072599395976,9.11679025300563));
#60274=CARTESIAN_POINT('Ctrl Pts',(52.9711273947103,30.3742729719765,9.11257154341743));
#60275=CARTESIAN_POINT('Ctrl Pts',(53.0091443191936,30.4303982820091,9.10903825481416));
#60276=CARTESIAN_POINT('Ctrl Pts',(53.0494398132988,30.4848680186467,9.1055049662109));
#60277=CARTESIAN_POINT('Ctrl Pts',(53.0918445043536,30.5374956437123,9.10197167760763));
#60278=CARTESIAN_POINT('Ctrl Pts',(53.1426421369415,30.6005395828511,9.09773906343615));
#60279=CARTESIAN_POINT('Ctrl Pts',(53.1966619733455,30.6611805883413,9.09350644926467));
#60280=CARTESIAN_POINT('Ctrl Pts',(53.2536481463105,30.7190711018208,9.08927383509319));
#60281=CARTESIAN_POINT('Ctrl Pts',(53.3105530338507,30.7768790399185,9.0850472583484));
#60282=CARTESIAN_POINT('Ctrl Pts',(53.3704155310609,30.8319439499115,9.08082068160361));
#60283=CARTESIAN_POINT('Ctrl Pts',(53.4329392147453,30.8839508341029,9.07659410485882));
#60284=CARTESIAN_POINT('Ctrl Pts',(53.4953935043809,30.9358999966751,9.07237221912479));
#60285=CARTESIAN_POINT('Ctrl Pts',(53.5605027563299,30.9847975818501,9.06815033339076));
#60286=CARTESIAN_POINT('Ctrl Pts',(53.6279343739839,31.0303660182108,9.06392844765674));
#60287=CARTESIAN_POINT('Ctrl Pts',(53.6953205111029,31.0759037200742,9.05970940945372));
#60288=CARTESIAN_POINT('Ctrl Pts',(53.7650255190825,31.1181164732636,9.05549037125071));
#60289=CARTESIAN_POINT('Ctrl Pts',(53.8366854677165,31.1567683113812,9.05127133304769));
#60290=CARTESIAN_POINT('Ctrl Pts',(53.908322014824,31.1954075272177,9.04705367262872));
#60291=CARTESIAN_POINT('Ctrl Pts',(53.9819118261865,31.2304879169971,9.04283601220975));
#60292=CARTESIAN_POINT('Ctrl Pts',(54.057065056535,31.2618187244765,9.03861835179079));
#60293=CARTESIAN_POINT('Ctrl Pts',(54.132216722973,31.2931488799736,9.03440077913975));
#60294=CARTESIAN_POINT('Ctrl Pts',(54.2089313144798,31.3207294306384,9.03018320648871));
#60295=CARTESIAN_POINT('Ctrl Pts',(54.2867989562092,31.3444177360564,9.02596563383767));
#60296=CARTESIAN_POINT('Ctrl Pts',(54.3647987826116,31.3681462536965,9.02174090162138));
#60297=CARTESIAN_POINT('Ctrl Pts',(54.4439551286935,31.3879691705021,9.01751616940509));
#60298=CARTESIAN_POINT('Ctrl Pts',(54.5238424968138,31.4037937270405,9.0132914371888));
#60299=CARTESIAN_POINT('Ctrl Pts',(54.603709912226,31.41961433123,9.00906776014369));
#60300=CARTESIAN_POINT('Ctrl Pts',(54.6843075202604,31.4314385255299,9.00484408309858));
#60301=CARTESIAN_POINT('Ctrl Pts',(54.7652034955927,31.4392254613951,9.00062040605347));
#60302=CARTESIAN_POINT('Ctrl Pts',(54.8462462445892,31.4470265254923,8.99638906577723));
#60303=CARTESIAN_POINT('Ctrl Pts',(54.9275879773352,31.450775670937,8.99215772550099));
#60304=CARTESIAN_POINT('Ctrl Pts',(55.0087948448896,31.4504842175993,8.98792638522476));
#60305=CARTESIAN_POINT('Ctrl Pts',(55.0897683224335,31.4501936019038,8.98370720589723));
#60306=CARTESIAN_POINT('Ctrl Pts',(55.1706072587814,31.4458856892045,8.97948802656971));
#60307=CARTESIAN_POINT('Ctrl Pts',(55.2508887426691,31.4376228356335,8.97526884724219));
#60308=CARTESIAN_POINT('Ctrl Pts',(55.3314258613909,31.4293336712234,8.97103623307072));
#60309=CARTESIAN_POINT('Ctrl Pts',(55.4117015091039,31.4170334819488,8.96680361889926));
#60310=CARTESIAN_POINT('Ctrl Pts',(55.4912848507461,31.4007476846656,8.96257100472779));
#60311=CARTESIAN_POINT('Ctrl Pts',(55.5707546742239,31.3844851175431,8.95834442798302));
#60312=CARTESIAN_POINT('Ctrl Pts',(55.6495337016168,31.3642483261047,8.95411785123825));
#60313=CARTESIAN_POINT('Ctrl Pts',(55.7271963318837,31.3401144726049,8.94989127449347));
#60314=CARTESIAN_POINT('Ctrl Pts',(55.8047727656244,31.3160074048878,8.94566938875944));
#60315=CARTESIAN_POINT('Ctrl Pts',(55.8812348228851,31.2880120066089,8.94144750302541));
#60316=CARTESIAN_POINT('Ctrl Pts',(55.9561686038967,31.2562561580907,8.93722561729138));
#60317=CARTESIAN_POINT('Ctrl Pts',(56.0310518443965,31.2245217279077,8.93300657908837));
#60318=CARTESIAN_POINT('Ctrl Pts',(56.1044084292349,31.1890320656087,8.92878754088536));
#60319=CARTESIAN_POINT('Ctrl Pts',(56.1758422999468,31.1499639847346,8.92456850268235));
#60320=CARTESIAN_POINT('Ctrl Pts',(56.247252842961,31.1109086620713,8.92035084226339));
#60321=CARTESIAN_POINT('Ctrl Pts',(56.3167415115339,31.0682774643003,8.91613318184443));
#60322=CARTESIAN_POINT('Ctrl Pts',(56.3839360624377,31.0222935556156,8.91191552142547));
#60323=CARTESIAN_POINT('Ctrl Pts',(56.4511292150484,30.9763106038386,8.90769794877443));
#60324=CARTESIAN_POINT('Ctrl Pts',(56.5160279622005,30.9269753431916,8.90348037612339));
#60325=CARTESIAN_POINT('Ctrl Pts',(56.5782895173192,30.8745539334787,8.89926280347235));
#60326=CARTESIAN_POINT('Ctrl Pts',(56.6406567649069,30.8220435354934,8.89503807125605));
#60327=CARTESIAN_POINT('Ctrl Pts',(56.7003775062325,30.7664368073819,8.89081333903975));
#60328=CARTESIAN_POINT('Ctrl Pts',(56.7571422910847,30.7080401689894,8.88658860682345));
#60329=CARTESIAN_POINT('Ctrl Pts',(56.8138928983363,30.6496581157702,8.88236492977835));
#60330=CARTESIAN_POINT('Ctrl Pts',(56.8676887336057,30.5884879097927,8.87814125273325));
#60331=CARTESIAN_POINT('Ctrl Pts',(56.918260446048,30.5248695390517,8.87391757568816));
#60332=CARTESIAN_POINT('Ctrl Pts',(56.9689239133089,30.4611357422793,8.86968623541193));
#60333=CARTESIAN_POINT('Ctrl Pts',(57.016351295979,30.3949452826139,8.8654548951357));
#60334=CARTESIAN_POINT('Ctrl Pts',(57.0603159017376,30.3266682460385,8.86122355485947));
#60335=CARTESIAN_POINT('Ctrl Pts',(57.1041541524224,30.2585874389039,8.85700437553189));
#60336=CARTESIAN_POINT('Ctrl Pts',(57.1445493486987,30.1884324685906,8.85278519620431));
#60337=CARTESIAN_POINT('Ctrl Pts',(57.1813235632301,30.1165920304647,8.84856601687674));
#60338=CARTESIAN_POINT('Ctrl Pts',(57.2182148753756,30.0445228357491,8.84433340270522));
#60339=CARTESIAN_POINT('Ctrl Pts',(57.2515992936489,29.9704893643416,8.84010078853371));
#60340=CARTESIAN_POINT('Ctrl Pts',(57.2812635913947,29.8948668485181,8.83586817436219));
#60341=CARTESIAN_POINT('Ctrl Pts',(57.3108855758052,29.8193522011129,8.83164159761737));
#60342=CARTESIAN_POINT('Ctrl Pts',(57.3367978106545,29.7422534399687,8.82741502087254));
#60343=CARTESIAN_POINT('Ctrl Pts',(57.3588333240383,29.6639695771694,8.82318844412772));
#60344=CARTESIAN_POINT('Ctrl Pts',(57.3808443805536,29.5857726003937,8.8189665583937));
#60345=CARTESIAN_POINT('Ctrl Pts',(57.3989871398471,29.5063935804293,8.81474467265968));
#60346=CARTESIAN_POINT('Ctrl Pts',(57.4131435437912,29.426249324995,8.81052278692566));
#60347=CARTESIAN_POINT('Ctrl Pts',(57.4272903996801,29.3461591243747,8.8063037487226));
#60348=CARTESIAN_POINT('Ctrl Pts',(57.4374561595622,29.265305169645,8.80208471051954));
#60349=CARTESIAN_POINT('Ctrl Pts',(57.4435735245486,29.1841159420724,8.79786567231648));
#60350=CARTESIAN_POINT('Ctrl Pts',(57.4496888918266,29.1029532279416,8.79364801189748));
#60351=CARTESIAN_POINT('Ctrl Pts',(57.4517584548587,29.0214559212844,8.78943035147848));
#60352=CARTESIAN_POINT('Ctrl Pts',(57.4497667598874,28.940057759878,8.78521269105948));
#60353=CARTESIAN_POINT('Ctrl Pts',(57.4477751063625,28.8586612923366,8.78099511840841));
#60354=CARTESIAN_POINT('Ctrl Pts',(57.4417223754058,28.7773644303241,8.77677754575734));
#60355=CARTESIAN_POINT('Ctrl Pts',(57.4316452152877,28.696599609479,8.77255997310626));
#60356=CARTESIAN_POINT('Ctrl Pts',(57.4215509486275,28.615697685839,8.76833524089001));
#60357=CARTESIAN_POINT('Ctrl Pts',(57.4074186420021,28.535330073799,8.76411050867376));
#60358=CARTESIAN_POINT('Ctrl Pts',(57.3893368631636,28.4559231632135,8.75988577645752));
#60359=CARTESIAN_POINT('Ctrl Pts',(57.3712596004387,28.3765360853354,8.75566209941237));
#60360=CARTESIAN_POINT('Ctrl Pts',(57.3492349845927,28.2981096721276,8.75143842236722));
#60361=CARTESIAN_POINT('Ctrl Pts',(57.3234015713157,28.2210549516122,8.74721474532208));
#60362=CARTESIAN_POINT('Ctrl Pts',(57.2975212871689,28.1438604268158,8.7429834050458));
#60363=CARTESIAN_POINT('Ctrl Pts',(57.2678185651516,28.0680430021525,8.73875206476953));
#60364=CARTESIAN_POINT('Ctrl Pts',(57.2344804312408,27.9939943079674,8.73452072449325));
#60365=CARTESIAN_POINT('Ctrl Pts',(57.2012381117335,27.9201584310769,8.73030154516593));
#60366=CARTESIAN_POINT('Ctrl Pts',(57.1643815302306,27.8480814989764,8.7260823658386));
#60367=CARTESIAN_POINT('Ctrl Pts',(57.1241398704255,27.7781243676753,8.72186318651128));
#60368=CARTESIAN_POINT('Ctrl Pts',(57.0837700718557,27.7079444766663,8.71763057233982));
#60369=CARTESIAN_POINT('Ctrl Pts',(57.0398434325917,27.6396369028923,8.71339795816837));
#60370=CARTESIAN_POINT('Ctrl Pts',(56.9925586261697,27.5735847830044,8.70916534399691));
#60371=CARTESIAN_POINT('Ctrl Pts',(56.9453412670842,27.5076268802634,8.70493876725215));
#60372=CARTESIAN_POINT('Ctrl Pts',(56.8947755227792,27.443918416245,8.70071219050739));
#60373=CARTESIAN_POINT('Ctrl Pts',(56.8411051950176,27.382816673695,8.69648561376262));
#60374=CARTESIAN_POINT('Ctrl Pts',(56.7874944351046,27.3217827470032,8.69226372802859));
#60375=CARTESIAN_POINT('Ctrl Pts',(56.7307862434185,27.2633501403435,8.68804184229456));
#60376=CARTESIAN_POINT('Ctrl Pts',(56.6712659778491,27.2078447943094,8.68381995656052));
#60377=CARTESIAN_POINT('Ctrl Pts',(56.6117858568535,27.1523768849103,8.67960091835753));
#60378=CARTESIAN_POINT('Ctrl Pts',(56.5494977677676,27.0998326309214,8.67538188015453));
#60379=CARTESIAN_POINT('Ctrl Pts',(56.4847244939177,27.0505017498954,8.67116284195153));
#60380=CARTESIAN_POINT('Ctrl Pts',(56.4199723726575,27.0011869785367,8.6669451815326));
#60381=CARTESIAN_POINT('Ctrl Pts',(56.3527370476518,26.9550837774033,8.66272752111366));
#60382=CARTESIAN_POINT('Ctrl Pts',(56.2833739360523,26.9124412366926,8.65850986069472));
#60383=CARTESIAN_POINT('Ctrl Pts',(56.2140122678729,26.8697995833571,8.65429228804371));
#60384=CARTESIAN_POINT('Ctrl Pts',(56.1425232974958,26.8306186895519,8.65007471539269));
#60385=CARTESIAN_POINT('Ctrl Pts',(56.0692897141918,26.7951032320937,8.64585714274168));
#60386=CARTESIAN_POINT('Ctrl Pts',(55.995931812787,26.7595274851614,8.64163241052536));
#60387=CARTESIAN_POINT('Ctrl Pts',(55.9208237932188,26.7276298276872,8.63740767830904));
#60388=CARTESIAN_POINT('Ctrl Pts',(55.8443715384095,26.6995680937867,8.63318294609272));
#60389=CARTESIAN_POINT('Ctrl Pts',(55.7679383783536,26.671513368599,8.62895926904763));
#60390=CARTESIAN_POINT('Ctrl Pts',(55.6901621058367,26.6472927694118,8.62473559200254));
#60391=CARTESIAN_POINT('Ctrl Pts',(55.6114629313621,26.6270138362034,8.62051191495746));
#60392=CARTESIAN_POINT('Ctrl Pts',(55.5326209689902,26.6066981098997,8.61628057468124));
#60393=CARTESIAN_POINT('Ctrl Pts',(55.4528532146922,26.5903384353346,8.61204923440502));
#60394=CARTESIAN_POINT('Ctrl Pts',(55.3725899949738,26.5779911342761,8.6078178941288));
#60395=CARTESIAN_POINT('Ctrl Pts',(55.2925574532021,26.5656793195844,8.60359871480114));
#60396=CARTESIAN_POINT('Ctrl Pts',(55.2120327515495,26.5573568099956,8.59937953547349));
#60397=CARTESIAN_POINT('Ctrl Pts',(55.1314433529275,26.5530278107483,8.59516035614583));
#60398=CARTESIAN_POINT('Ctrl Pts',(55.0505973390032,26.5486850269653,8.59092774197442));
#60399=CARTESIAN_POINT('Ctrl Pts',(54.9693855250677,26.5483451018986,8.58669512780302));
#60400=CARTESIAN_POINT('Ctrl Pts',(54.8882374538426,26.552049963076,8.58246251363161));
#60401=CARTESIAN_POINT('Ctrl Pts',(54.807205132722,26.5557495396167,8.57823593688691));
#60402=CARTESIAN_POINT('Ctrl Pts',(54.7262368339361,26.5634824224046,8.57400936014221));
#60403=CARTESIAN_POINT('Ctrl Pts',(54.6457649811417,26.5752386093856,8.56978278339751));
#60404=CARTESIAN_POINT('Ctrl Pts',(54.5653824427835,26.5869817483606,8.56556089766346));
#60405=CARTESIAN_POINT('Ctrl Pts',(54.4854957129381,26.6027392519697,8.56133901192941));
#60406=CARTESIAN_POINT('Ctrl Pts',(54.4065335478631,26.6224491971384,8.55711712619536));
#60407=CARTESIAN_POINT('Ctrl Pts',(54.3276246403217,26.6421458485597,8.55289808799242));
#60408=CARTESIAN_POINT('Ctrl Pts',(54.2496395086022,26.6657895348154,8.54867904978947));
#60409=CARTESIAN_POINT('Ctrl Pts',(54.1729968985998,26.6932672195778,8.54446001158653));
#60410=CARTESIAN_POINT('Ctrl Pts',(54.0963793172795,26.7207359311301,8.54024235116764));
#60411=CARTESIAN_POINT('Ctrl Pts',(54.0211038239627,26.7520359980488,8.53602469074875));
#60412=CARTESIAN_POINT('Ctrl Pts',(53.9475728511745,26.7870048923653,8.53180703032986));
#60413=CARTESIAN_POINT('Ctrl Pts',(53.8740434085379,26.8219730589925,8.52758945767888));
#60414=CARTESIAN_POINT('Ctrl Pts',(53.8022588332697,26.860609700648,8.5233718850279));
#60415=CARTESIAN_POINT('Ctrl Pts',(53.7325991497947,26.9027052341412,8.51915431237692));
#60416=CARTESIAN_POINT('Ctrl Pts',(53.662821215112,26.9448722271562,8.51492958016054));
#60417=CARTESIAN_POINT('Ctrl Pts',(53.5951757889163,26.9905096183042,8.51070484794416));
#60418=CARTESIAN_POINT('Ctrl Pts',(53.5300162294356,27.0393628677704,8.50648011572778));
#60419=CARTESIAN_POINT('Ctrl Pts',(53.4648729442408,27.0882039156235,8.50225643868274));
#60420=CARTESIAN_POINT('Ctrl Pts',(53.4022146291533,27.1402589013781,8.49803276163769));
#60421=CARTESIAN_POINT('Ctrl Pts',(53.3423602543571,27.1952338867141,8.49380908459265));
#60422=CARTESIAN_POINT('Ctrl Pts',(53.2823972827381,27.2503086159496,8.48957774431648));
#60423=CARTESIAN_POINT('Ctrl Pts',(53.2252487452473,27.3083136005641,8.48534640404031));
#60424=CARTESIAN_POINT('Ctrl Pts',(53.1711961561012,27.3689185334445,8.48111506376414));
#60425=CARTESIAN_POINT('Ctrl Pts',(53.1172989150709,27.429349286655,8.47689588443622));
#60426=CARTESIAN_POINT('Ctrl Pts',(53.0664800715651,27.4923646569045,8.4726767051083));
#60427=CARTESIAN_POINT('Ctrl Pts',(53.0189758641979,27.557608366854,8.46845752578038));
#60428=CARTESIAN_POINT('Ctrl Pts',(52.9710150013666,27.6234792611793,8.46419778770196));
#60429=CARTESIAN_POINT('Ctrl Pts',(52.9262542749234,27.691866689358,8.45993804962353));
#60430=CARTESIAN_POINT('Ctrl Pts',(52.8849658519662,27.7624294756859,8.45567831154511));
#60431=CARTESIAN_POINT('Ctrl Pts',(52.8437376019429,27.8328894251997,8.45142478152501));
#60432=CARTESIAN_POINT('Ctrl Pts',(52.8059718335822,27.9055180461353,8.4471712515049));
#60433=CARTESIAN_POINT('Ctrl Pts',(52.7718988642993,27.9799433451571,8.4429177214848));
#60434=CARTESIAN_POINT('Ctrl Pts',(52.7378655894756,28.054281939907,8.4386691467585));
#60435=CARTESIAN_POINT('Ctrl Pts',(52.7075167558013,28.130412641639,8.4344205720322));
#60436=CARTESIAN_POINT('Ctrl Pts',(52.6810372815973,28.2079380323115,8.4301719973059));
#60437=CARTESIAN_POINT('Ctrl Pts',(52.6545822678531,28.2853918087714,8.4259273472078));
#60438=CARTESIAN_POINT('Ctrl Pts',(52.6319896538309,28.3642372819011,8.42168269710969));
#60439=CARTESIAN_POINT('Ctrl Pts',(52.6133961035504,28.4440574746867,8.41743804701158));
#60440=CARTESIAN_POINT('Ctrl Pts',(52.594812424493,28.5238352913302,8.41319565037704));
#60441=CARTESIAN_POINT('Ctrl Pts',(52.5802236919809,28.6045863549805,8.40895325374249));
#60442=CARTESIAN_POINT('Ctrl Pts',(52.5697162820903,28.685880117689,8.40471085710795));
#60443=CARTESIAN_POINT('Ctrl Pts',(52.5592102493312,28.7671632258017,8.40046901649419));
#60444=CARTESIAN_POINT('Ctrl Pts',(52.5527845372909,28.8489884393477,8.39622717588043));
#60445=CARTESIAN_POINT('Ctrl Pts',(52.5504739432897,28.9309178206984,8.39198533526666));
#60446=CARTESIAN_POINT('Ctrl Pts',(52.5498097834161,28.9544676990108,8.3907660555818));
#60447=CARTESIAN_POINT('Ctrl Pts',(52.5494852960204,28.9780261599311,8.38954677589693));
#60448=CARTESIAN_POINT('Ctrl Pts',(52.5495005111525,29.0015827691152,8.38832749621206));
#60449=CARTESIAN_POINT('',(52.5495001241791,29.000780129339,7.58832749625521));
#60450=CARTESIAN_POINT('Ctrl Pts',(52.5495005111528,29.0015827696721,8.38832749618324));
#60451=CARTESIAN_POINT('Ctrl Pts',(52.54956003669,29.093742292839,8.38355735997699));
#60452=CARTESIAN_POINT('Ctrl Pts',(52.5548225910511,29.185703809808,8.37878722377074));
#60453=CARTESIAN_POINT('Ctrl Pts',(52.5651971369812,29.2769210505458,8.3740170875645));
#60454=CARTESIAN_POINT('Ctrl Pts',(52.5756211608251,29.3685733212895,8.36922420179507));
#60455=CARTESIAN_POINT('Ctrl Pts',(52.5912059224144,29.4594739912179,8.36443131602564));
#60456=CARTESIAN_POINT('Ctrl Pts',(52.6118095392283,29.5490870359779,8.3596384302562));
#60457=CARTESIAN_POINT('Ctrl Pts',(52.6325284203184,29.6392014093562,8.35481873130564));
#60458=CARTESIAN_POINT('Ctrl Pts',(52.6583223494864,29.7280135082775,8.34999903235508));
#60459=CARTESIAN_POINT('Ctrl Pts',(52.6889989463192,29.8149996195619,8.34517933340452));
#60460=CARTESIAN_POINT('Ctrl Pts',(52.696264700189,29.8356022854357,8.34403778740799));
#60461=CARTESIAN_POINT('Ctrl Pts',(52.7038041549949,29.8561026184683,8.34289624141145));
#60462=CARTESIAN_POINT('Ctrl Pts',(52.7116143735494,29.8764938531754,8.34175469541492));
#60463=CARTESIAN_POINT('Ctrl Pts',(52.7405730329762,29.9521002932589,8.33752208124372));
#60464=CARTESIAN_POINT('Ctrl Pts',(52.7733365344255,30.0264106373841,8.33328946707252));
#60465=CARTESIAN_POINT('Ctrl Pts',(52.8097682372598,30.0990155028406,8.32905685290132));
#60466=CARTESIAN_POINT('Ctrl Pts',(52.8461479736908,30.1715168042739,8.3248302761568));
#60467=CARTESIAN_POINT('Ctrl Pts',(52.8861853127835,30.2423170469457,8.32060369941229));
#60468=CARTESIAN_POINT('Ctrl Pts',(52.9296950125962,30.3110253655558,8.31637712266778));
#60469=CARTESIAN_POINT('Ctrl Pts',(52.9731564216839,30.3796574258942,8.31215523693368));
#60470=CARTESIAN_POINT('Ctrl Pts',(53.0200822864821,30.4462017850736,8.30793335119959));
#60471=CARTESIAN_POINT('Ctrl Pts',(53.0702414384091,30.5102920724041,8.30371146546549));
#60472=CARTESIAN_POINT('Ctrl Pts',(53.1203667595396,30.5743391328181,8.29949242726274));
#60473=CARTESIAN_POINT('Ctrl Pts',(53.173720751063,30.6359350438601,8.29527338905999));
#60474=CARTESIAN_POINT('Ctrl Pts',(53.2300296387102,30.6947433936014,8.29105435085723));
#60475=CARTESIAN_POINT('Ctrl Pts',(53.2863201379277,30.7535325386799,8.28683669043854));
#60476=CARTESIAN_POINT('Ctrl Pts',(53.3455632958838,30.8095355950081,8.28261903001984));
#60477=CARTESIAN_POINT('Ctrl Pts',(53.4074467805978,30.8624512056351,8.27840136960114));
#60478=CARTESIAN_POINT('Ctrl Pts',(53.4693289775399,30.9153657151083,8.27418379695036));
#60479=CARTESIAN_POINT('Ctrl Pts',(53.5338510381637,30.9651926056109,8.26996622429957));
#60480=CARTESIAN_POINT('Ctrl Pts',(53.6006667801059,31.0116701493289,8.26574865164879));
#60481=CARTESIAN_POINT('Ctrl Pts',(53.6675959455129,31.0582265912808,8.26152391943218));
#60482=CARTESIAN_POINT('Ctrl Pts',(53.7368261991617,31.1014220440101,8.25729918721557));
#60483=CARTESIAN_POINT('Ctrl Pts',(53.8079811591194,31.1410374431536,8.25307445499896));
#60484=CARTESIAN_POINT('Ctrl Pts',(53.8791183473698,31.1806429479302,8.24885077795411));
#60485=CARTESIAN_POINT('Ctrl Pts',(53.9521788531332,31.2166700001067,8.24462710090925));
#60486=CARTESIAN_POINT('Ctrl Pts',(54.0267643159805,31.2489469876702,8.2404034238644));
#60487=CARTESIAN_POINT('Ctrl Pts',(54.1014851030099,31.2812825370068,8.23617208358841));
#60488=CARTESIAN_POINT('Ctrl Pts',(54.1777359402165,31.3098542608292,8.23194074331241));
#60489=CARTESIAN_POINT('Ctrl Pts',(54.2551005051838,31.3345395675856,8.22770940303642));
#60490=CARTESIAN_POINT('Ctrl Pts',(54.332242723019,31.3591539283325,8.22349022370744));
#60491=CARTESIAN_POINT('Ctrl Pts',(54.4104918140557,31.3799041451524,8.21927104437846));
#60492=CARTESIAN_POINT('Ctrl Pts',(54.4894261756389,31.3967195538647,8.21505186504948));
#60493=CARTESIAN_POINT('Ctrl Pts',(54.5686118824718,31.4135885067245,8.21081925087842));
#60494=CARTESIAN_POINT('Ctrl Pts',(54.6487817503826,31.4265602664254,8.20658663670737));
#60495=CARTESIAN_POINT('Ctrl Pts',(54.7295179915529,31.4355265823034,8.20235402253631));
#60496=CARTESIAN_POINT('Ctrl Pts',(54.8101390700559,31.4444801085737,8.19812744579195));
#60497=CARTESIAN_POINT('Ctrl Pts',(54.8913244593947,31.4494394876987,8.19390086904759));
#60498=CARTESIAN_POINT('Ctrl Pts',(54.9726454460324,31.4503473179077,8.18967429230322));
#60499=CARTESIAN_POINT('Ctrl Pts',(55.053876175802,31.4512541405303,8.18545240656909));
#60500=CARTESIAN_POINT('Ctrl Pts',(55.1352417416545,31.4481183441097,8.18123052083496));
#60501=CARTESIAN_POINT('Ctrl Pts',(55.2163089742501,31.4409343861847,8.17700863510082));
#60502=CARTESIAN_POINT('Ctrl Pts',(55.2973215295009,31.4337552736175,8.17278959689824));
#60503=CARTESIAN_POINT('Ctrl Pts',(55.3780356895875,31.4225334631796,8.16857055869565));
#60504=CARTESIAN_POINT('Ctrl Pts',(55.4580202207648,31.4073154607094,8.16435152049306));
#60505=CARTESIAN_POINT('Ctrl Pts',(55.5379786319102,31.392102427884,8.16013386007453));
#60506=CARTESIAN_POINT('Ctrl Pts',(55.6172074313242,31.3728958814592,8.15591619965601));
#60507=CARTESIAN_POINT('Ctrl Pts',(55.6952837994118,31.3497937544124,8.15169853923748));
#60508=CARTESIAN_POINT('Ctrl Pts',(55.7733585427597,31.3266921081121,8.14748096658687));
#60509=CARTESIAN_POINT('Ctrl Pts',(55.8502804573394,31.299695175302,8.14326339393626));
#60510=CARTESIAN_POINT('Ctrl Pts',(55.9256415373002,31.2689508576487,8.13904582128565));
#60511=CARTESIAN_POINT('Ctrl Pts',(56.0011305469222,31.2381543497912,8.13482108906885));
#60512=CARTESIAN_POINT('Ctrl Pts',(56.0750529882894,31.2035979058228,8.13059635685204));
#60513=CARTESIAN_POINT('Ctrl Pts',(56.1470202020595,31.1654779855882,8.12637162463524));
#60514=CARTESIAN_POINT('Ctrl Pts',(56.2189694412471,31.1273675862121,8.12214794759057));
#60515=CARTESIAN_POINT('Ctrl Pts',(56.2889640397234,31.0856957471054,8.11792427054589));
#60516=CARTESIAN_POINT('Ctrl Pts',(56.3566431772644,31.0407031973273,8.11370059350122));
#60517=CARTESIAN_POINT('Ctrl Pts',(56.4244451084916,30.9956290152879,8.10946925322541));
#60518=CARTESIAN_POINT('Ctrl Pts',(56.4899228084764,30.9472223589163,8.10523791294961));
#60519=CARTESIAN_POINT('Ctrl Pts',(56.5527467980732,30.8957657110185,8.1010065726738));
#60520=CARTESIAN_POINT('Ctrl Pts',(56.6153902304262,30.8444569504258,8.09678739334387));
#60521=CARTESIAN_POINT('Ctrl Pts',(56.6753949040331,30.7901160735973,8.09256821401394));
#60522=CARTESIAN_POINT('Ctrl Pts',(56.7324720231711,30.7330582618393,8.08834903468401));
#60523=CARTESIAN_POINT('Ctrl Pts',(56.7897308890671,30.6758187648024,8.08411642051055));
#60524=CARTESIAN_POINT('Ctrl Pts',(56.8442564691055,30.6156320935251,8.07988380633709));
#60525=CARTESIAN_POINT('Ctrl Pts',(56.8957305158735,30.5527897672209,8.07565119216363));
#60526=CARTESIAN_POINT('Ctrl Pts',(56.947131139747,30.4900370795945,8.07142461541686));
#60527=CARTESIAN_POINT('Ctrl Pts',(56.9954885835029,30.4246366168747,8.06719803867008));
#60528=CARTESIAN_POINT('Ctrl Pts',(57.0405213050927,30.3569167452216,8.06297146192331));
#60529=CARTESIAN_POINT('Ctrl Pts',(57.0855040455498,30.2892720348241,8.05874957618978));
#60530=CARTESIAN_POINT('Ctrl Pts',(57.1271691400413,30.2193134154538,8.05452769045625));
#60531=CARTESIAN_POINT('Ctrl Pts',(57.1652761216738,30.14740122316,8.05030580472271));
#60532=CARTESIAN_POINT('Ctrl Pts',(57.2033574013513,30.0755375333677,8.04608676651771));
#60533=CARTESIAN_POINT('Ctrl Pts',(57.2378851174962,30.0017232969852,8.04186772831271));
#60534=CARTESIAN_POINT('Ctrl Pts',(57.26866351638,29.9263455615732,8.03764869010771));
#60535=CARTESIAN_POINT('Ctrl Pts',(57.2994318641608,29.8509924417816,8.03343102968677));
#60536=CARTESIAN_POINT('Ctrl Pts',(57.3264531507695,29.7740772666921,8.02921336926582));
#60537=CARTESIAN_POINT('Ctrl Pts',(57.3495793415295,29.69600802284,8.02499570884488));
#60538=CARTESIAN_POINT('Ctrl Pts',(57.3727050510423,29.6179404035795,8.02077813619187));
#60539=CARTESIAN_POINT('Ctrl Pts',(57.3919356950475,29.5387192090555,8.01656056353886));
#60540=CARTESIAN_POINT('Ctrl Pts',(57.4071732184801,29.4587672026555,8.01234299088585));
#60541=CARTESIAN_POINT('Ctrl Pts',(57.4224366084445,29.3786794733389,8.00811825867191));
#60542=CARTESIAN_POINT('Ctrl Pts',(57.4336932281304,29.2978589087463,8.00389352645796));
#60543=CARTESIAN_POINT('Ctrl Pts',(57.4408962865524,29.2167384790355,7.99966879424403));
#60544=CARTESIAN_POINT('Ctrl Pts',(57.4480975459424,29.1356383099208,7.99544511719699));
#60545=CARTESIAN_POINT('Ctrl Pts',(57.451247271857,29.0542388920839,7.99122144014996));
#60546=CARTESIAN_POINT('Ctrl Pts',(57.4503509630831,28.9729739437261,7.98699776310293));
#60547=CARTESIAN_POINT('Ctrl Pts',(57.4494530280908,28.8915615522583,7.9827664228248));
#60548=CARTESIAN_POINT('Ctrl Pts',(57.4444944161923,28.8102845828779,7.97853508254668));
#60549=CARTESIAN_POINT('Ctrl Pts',(57.435532712379,28.7295731948718,7.97430374226855));
#60550=CARTESIAN_POINT('Ctrl Pts',(57.426596764692,28.6490937731021,7.97008456295189));
#60551=CARTESIAN_POINT('Ctrl Pts',(57.4136808590501,28.5691771222106,7.96586538363523));
#60552=CARTESIAN_POINT('Ctrl Pts',(57.3968921568583,28.4902370762884,7.96164620431857));
#60553=CARTESIAN_POINT('Ctrl Pts',(57.3800499955182,28.4110456668256,7.95741359014969));
#60554=CARTESIAN_POINT('Ctrl Pts',(57.3592476670589,28.3325425624581,7.95318097598081));
#60555=CARTESIAN_POINT('Ctrl Pts',(57.3345564510021,28.2551534204384,7.94894836181193));
#60556=CARTESIAN_POINT('Ctrl Pts',(57.3099004546465,28.1778746667632,7.94472178506973));
#60557=CARTESIAN_POINT('Ctrl Pts',(57.2813667280436,28.1017071584427,7.94049520832754));
#60558=CARTESIAN_POINT('Ctrl Pts',(57.2490774412937,28.0270658228514,7.93626863158534));
#60559=CARTESIAN_POINT('Ctrl Pts',(57.2168239918883,27.9525073304422,7.93204674585066));
#60560=CARTESIAN_POINT('Ctrl Pts',(57.1808234481206,27.8794720692538,7.92782486011599));
#60561=CARTESIAN_POINT('Ctrl Pts',(57.1412471585885,27.8083579162195,7.92360297438131));
#60562=CARTESIAN_POINT('Ctrl Pts',(57.1016975620664,27.73729172753,7.91938393618084));
#60563=CARTESIAN_POINT('Ctrl Pts',(57.0585772350112,27.6681444784381,7.91516489798036));
#60564=CARTESIAN_POINT('Ctrl Pts',(57.012104274193,27.6012910811129,7.91094585977989));
#60565=CARTESIAN_POINT('Ctrl Pts',(56.9656464897493,27.5344595156696,7.90672819936345));
#60566=CARTESIAN_POINT('Ctrl Pts',(56.9158385107976,27.4699206954975,7.90251053894701));
#60567=CARTESIAN_POINT('Ctrl Pts',(56.8629419765386,27.4080209040159,7.89829287853057));
#60568=CARTESIAN_POINT('Ctrl Pts',(56.8100465430362,27.3461224006452,7.89407530588203));
#60569=CARTESIAN_POINT('Ctrl Pts',(56.7540629847037,27.2868631691755,7.88985773323349));
#60570=CARTESIAN_POINT('Ctrl Pts',(56.6952925448785,27.2305556133975,7.88564016058495));
#60571=CARTESIAN_POINT('Ctrl Pts',(56.6364223388707,27.1741524723232,7.88141542836563));
#60572=CARTESIAN_POINT('Ctrl Pts',(56.5747561231674,27.1207113551315,7.87719069614631));
#60573=CARTESIAN_POINT('Ctrl Pts',(56.5106316110116,27.0705072205855,7.87296596392699));
#60574=CARTESIAN_POINT('Ctrl Pts',(56.4465231147079,27.0203156251134,7.8687422868843));
#60575=CARTESIAN_POINT('Ctrl Pts',(56.3799579429414,26.9733596468785,7.86451860984161));
#60576=CARTESIAN_POINT('Ctrl Pts',(56.3113029030241,26.9298707898973,7.86029493279892));
#60577=CARTESIAN_POINT('Ctrl Pts',(56.2425232987904,26.88630302888,7.85606359252503));
#60578=CARTESIAN_POINT('Ctrl Pts',(56.1716466542426,26.8462151899789,7.85183225225114));
#60579=CARTESIAN_POINT('Ctrl Pts',(56.0990651471578,26.8097931485125,7.84760091197725));
#60580=CARTESIAN_POINT('Ctrl Pts',(56.0266922403633,26.7734757845145,7.84338173263587));
#60581=CARTESIAN_POINT('Ctrl Pts',(55.9526247076398,26.7408032826157,7.83916255329449));
#60582=CARTESIAN_POINT('Ctrl Pts',(55.8772680222262,26.7119110447408,7.83494337395311));
#60583=CARTESIAN_POINT('Ctrl Pts',(55.8016713839619,26.6829268073995,7.83071075978369));
#60584=CARTESIAN_POINT('Ctrl Pts',(55.7244961952023,26.6576391719911,7.82647814561427));
#60585=CARTESIAN_POINT('Ctrl Pts',(55.6461383126182,26.6362200756063,7.82224553144485));
#60586=CARTESIAN_POINT('Ctrl Pts',(55.567892200197,26.6148315315514,7.81801895470215));
#60587=CARTESIAN_POINT('Ctrl Pts',(55.4884671889393,26.59730068832,7.81379237795946));
#60588=CARTESIAN_POINT('Ctrl Pts',(55.4082778398956,26.5837509533473,7.80956580121676));
#60589=CARTESIAN_POINT('Ctrl Pts',(55.3281774916941,26.570216257003,7.80534391548222));
#60590=CARTESIAN_POINT('Ctrl Pts',(55.2473149470752,26.5606539662429,7.80112202974767));
#60591=CARTESIAN_POINT('Ctrl Pts',(55.1661172375628,26.5551369540638,7.79690014401313));
#60592=CARTESIAN_POINT('Ctrl Pts',(55.0849742934391,26.5496236629418,7.79268110581226));
#60593=CARTESIAN_POINT('Ctrl Pts',(55.0034970956777,26.5481502629355,7.7884620676114));
#60594=CARTESIAN_POINT('Ctrl Pts',(54.9221188621217,26.5507379114593,7.78424302941054));
#60595=CARTESIAN_POINT('Ctrl Pts',(54.8407672037304,26.5533247149514,7.78002536899375));
#60596=CARTESIAN_POINT('Ctrl Pts',(54.7595149093206,26.559969918488,7.77580770857697));
#60597=CARTESIAN_POINT('Ctrl Pts',(54.678794886752,26.5706425694799,7.77159004816019));
#60598=CARTESIAN_POINT('Ctrl Pts',(54.5980765439369,26.5813149983779,7.76737247551134));
#60599=CARTESIAN_POINT('Ctrl Pts',(54.5178909113262,26.5960146460401,7.76315490286249));
#60600=CARTESIAN_POINT('Ctrl Pts',(54.4386640382166,26.614658894831,7.75893733021364));
#60601=CARTESIAN_POINT('Ctrl Pts',(54.3593026729739,26.6333347932971,7.75471259799481));
#60602=CARTESIAN_POINT('Ctrl Pts',(54.2809037781545,26.6559685834207,7.75048786577598));
#60603=CARTESIAN_POINT('Ctrl Pts',(54.2038818474671,26.6824266705868,7.74626313355715));
#60604=CARTESIAN_POINT('Ctrl Pts',(54.1268791539015,26.7088781495383,7.74203945651425));
#60605=CARTESIAN_POINT('Ctrl Pts',(54.0512531615973,26.7391518224769,7.73781577947137));
#60606=CARTESIAN_POINT('Ctrl Pts',(53.9773977521605,26.7730660331493,7.73359210242848));
#60607=CARTESIAN_POINT('Ctrl Pts',(53.9034083431144,26.8070417760914,7.72936076215445));
#60608=CARTESIAN_POINT('Ctrl Pts',(53.8311963500906,26.8446710417584,7.72512942188042));
#60609=CARTESIAN_POINT('Ctrl Pts',(53.7611311918934,26.8857260522107,7.72089808160639));
#60610=CARTESIAN_POINT('Ctrl Pts',(53.6912674019958,26.9266630699565,7.71667890226682));
#60611=CARTESIAN_POINT('Ctrl Pts',(53.6235384586531,26.971005848546,7.71245972292724));
#60612=CARTESIAN_POINT('Ctrl Pts',(53.5582786803735,27.0184879797149,7.70824054358767));
#60613=CARTESIAN_POINT('Ctrl Pts',(53.493336088166,27.0657393305918,7.70404187098223));
#60614=CARTESIAN_POINT('Ctrl Pts',(53.4305885577082,27.1162817178861,7.69984319837678));
#60615=CARTESIAN_POINT('Ctrl Pts',(53.3703926384257,27.1698824909031,7.69564452577134));
#60616=CARTESIAN_POINT('Ctrl Pts',(53.3102828322357,27.2234065854944,7.69145185956444));
#60617=CARTESIAN_POINT('Ctrl Pts',(53.2527177405871,27.2799800682008,7.68725919335755));
#60618=CARTESIAN_POINT('Ctrl Pts',(53.1980236960905,27.3393279522589,7.68306652715065));
#60619=CARTESIAN_POINT('Ctrl Pts',(53.1433919473746,27.3986082398757,7.67887863633415));
#60620=CARTESIAN_POINT('Ctrl Pts',(53.0916250678718,27.4606563049205,7.67469074551765));
#60621=CARTESIAN_POINT('Ctrl Pts',(53.0430139528752,27.5251590386218,7.67050285470115));
#60622=CARTESIAN_POINT('Ctrl Pts',(52.9944325484566,27.5896223489628,7.66631752347739));
#60623=CARTESIAN_POINT('Ctrl Pts',(52.9490033651089,27.6565369742822,7.66213219225362));
#60624=CARTESIAN_POINT('Ctrl Pts',(52.9069774212357,27.7255563038005,7.65794686102986));
#60625=CARTESIAN_POINT('Ctrl Pts',(52.864963787464,27.7945554164032,7.65376275575959));
#60626=CARTESIAN_POINT('Ctrl Pts',(52.8263516595754,27.8656576054518,7.64957865048931));
#60627=CARTESIAN_POINT('Ctrl Pts',(52.791348199437,27.9384881188277,7.64539454521904));
#60628=CARTESIAN_POINT('Ctrl Pts',(52.7563438519329,28.0113204785156,7.64121033387833));
#60629=CARTESIAN_POINT('Ctrl Pts',(52.724948556607,28.0858808223611,7.63702612253763));
#60630=CARTESIAN_POINT('Ctrl Pts',(52.6973223782933,28.1617720951368,7.63284191119692));
#60631=CARTESIAN_POINT('Ctrl Pts',(52.6696696439529,28.2377363193953,7.62865367772811));
#60632=CARTESIAN_POINT('Ctrl Pts',(52.6457934207092,28.3150335811986,7.6244654442593));
#60633=CARTESIAN_POINT('Ctrl Pts',(52.6258044213698,28.3932499654614,7.62027721079048));
#60634=CARTESIAN_POINT('Ctrl Pts',(52.6058048288362,28.4715078005907,7.61608675776233));
#60635=CARTESIAN_POINT('Ctrl Pts',(52.5896966540588,28.5506852641807,7.61189630473417));
#60636=CARTESIAN_POINT('Ctrl Pts',(52.5775393163813,28.6303589764087,7.60770585170601));
#60637=CARTESIAN_POINT('Ctrl Pts',(52.5653624033685,28.7101609765624,7.60350865135165));
#60638=CARTESIAN_POINT('Ctrl Pts',(52.5571490730172,28.7904603501842,7.59931145099729));
#60639=CARTESIAN_POINT('Ctrl Pts',(52.5529067564705,28.8708299281092,7.59511425064293));
#60640=CARTESIAN_POINT('Ctrl Pts',(52.5506201878051,28.9141483737054,7.59285199918035));
#60641=CARTESIAN_POINT('Ctrl Pts',(52.5494863416593,28.9574872273925,7.59058974771779));
#60642=CARTESIAN_POINT('Ctrl Pts',(52.5495001241791,29.000780129339,7.58832749625521));
#60643=CARTESIAN_POINT('',(52.5495009849895,28.9978028581341,6.78832749625012));
#60644=CARTESIAN_POINT('Ctrl Pts',(52.5495001241794,29.000780130165,7.58832749621205));
#60645=CARTESIAN_POINT('Ctrl Pts',(52.5495139128642,29.0440923516512,7.58606423521544));
#60646=CARTESIAN_POINT('Ctrl Pts',(52.5506759352354,29.0873847550339,7.58380097421883));
#60647=CARTESIAN_POINT('Ctrl Pts',(52.5529834801352,29.1306154719347,7.58153771322222));
#60648=CARTESIAN_POINT('Ctrl Pts',(52.5572989113675,29.2114629501035,7.5773050990735));
#60649=CARTESIAN_POINT('Ctrl Pts',(52.5656333752337,29.2922466793995,7.57307248492477));
#60650=CARTESIAN_POINT('Ctrl Pts',(52.5779826895163,29.3725350959535,7.56883987077604));
#60651=CARTESIAN_POINT('Ctrl Pts',(52.5903143886615,29.4527089886203,7.56461329405396));
#60652=CARTESIAN_POINT('Ctrl Pts',(52.6066494940107,29.5323885164452,7.56038671733188));
#60653=CARTESIAN_POINT('Ctrl Pts',(52.626931883058,29.6111447965527,7.5561601406098));
#60654=CARTESIAN_POINT('Ctrl Pts',(52.6471917611382,29.6898136668373,7.55193825487009));
#60655=CARTESIAN_POINT('Ctrl Pts',(52.6713901026035,29.7675608778629,7.54771636913039));
#60656=CARTESIAN_POINT('Ctrl Pts',(52.6994195524536,29.8439667377138,7.54349448339068));
#60657=CARTESIAN_POINT('Ctrl Pts',(52.7274300971225,29.9203210636733,7.53927544521007));
#60658=CARTESIAN_POINT('Ctrl Pts',(52.759266458567,29.9953354002865,7.53505640702946));
#60659=CARTESIAN_POINT('Ctrl Pts',(52.7947715297969,30.0686054670483,7.53083736884884));
#60660=CARTESIAN_POINT('Ctrl Pts',(52.8302650063662,30.1418516064803,7.52661970845213));
#60661=CARTESIAN_POINT('Ctrl Pts',(52.8694246110104,30.21335418955,7.52240204805542));
#60662=CARTESIAN_POINT('Ctrl Pts',(52.9120457701724,30.282730440952,7.51818438765871));
#60663=CARTESIAN_POINT('Ctrl Pts',(52.954666042406,30.3521052486634,7.51396681502973));
#60664=CARTESIAN_POINT('Ctrl Pts',(53.0007474817649,30.4193534174791,7.50974924240076));
#60665=CARTESIAN_POINT('Ctrl Pts',(53.0500411214562,30.4841194769924,7.50553166977178));
#60666=CARTESIAN_POINT('Ctrl Pts',(53.0994184404249,30.5489954812591,7.50130693752886));
#60667=CARTESIAN_POINT('Ctrl Pts',(53.1520185869289,30.6113805742921,7.49708220528594));
#60668=CARTESIAN_POINT('Ctrl Pts',(53.2075507422407,30.6709506002148,7.49285747304302));
#60669=CARTESIAN_POINT('Ctrl Pts',(53.2630690271832,30.7305057472218,7.4886337960193));
#60670=CARTESIAN_POINT('Ctrl Pts',(53.3215175071784,30.7872469237406,7.48441011899559));
#60671=CARTESIAN_POINT('Ctrl Pts',(53.3825698625209,30.8408883726002,7.48018644197187));
#60672=CARTESIAN_POINT('Ctrl Pts',(53.443732988252,30.8946271458644,7.47595510171645));
#60673=CARTESIAN_POINT('Ctrl Pts',(53.5075090658685,30.9452546624414,7.47172376146103));
#60674=CARTESIAN_POINT('Ctrl Pts',(53.5735396146827,30.9925262906974,7.46749242120561));
#60675=CARTESIAN_POINT('Ctrl Pts',(53.6393803927309,31.0396620610321,7.46327324175599));
#60676=CARTESIAN_POINT('Ctrl Pts',(53.7074622727845,31.0834610304722,7.45905406230637));
#60677=CARTESIAN_POINT('Ctrl Pts',(53.7774057872843,31.1237263573808,7.45483488285675));
#60678=CARTESIAN_POINT('Ctrl Pts',(53.8475720159899,31.164119897182,7.45060226869189));
#60679=CARTESIAN_POINT('Ctrl Pts',(53.9198727351502,31.2011074660635,7.44636965452703));
#60680=CARTESIAN_POINT('Ctrl Pts',(53.9939436613002,31.2344576284553,7.44213704036217));
#60681=CARTESIAN_POINT('Ctrl Pts',(54.0679089322243,31.2677602199697,7.43791046362427));
#60682=CARTESIAN_POINT('Ctrl Pts',(54.143638975022,31.2974355207267,7.43368388688636));
#60683=CARTESIAN_POINT('Ctrl Pts',(54.2207434787784,31.3232971235151,7.42945731014846));
#60684=CARTESIAN_POINT('Ctrl Pts',(54.2977624056204,31.3491300229715,7.42523542441274));
#60685=CARTESIAN_POINT('Ctrl Pts',(54.3761523240618,31.3711574879541,7.42101353867703));
#60686=CARTESIAN_POINT('Ctrl Pts',(54.4555027417914,31.3892410899286,7.41679165294131));
#60687=CARTESIAN_POINT('Ctrl Pts',(54.5347996399532,31.4073124950353,7.41257261474574));
#60688=CARTESIAN_POINT('Ctrl Pts',(54.6150552989914,31.4214452172141,7.40835357655017));
#60689=CARTESIAN_POINT('Ctrl Pts',(54.6958450690456,31.4315509511372,7.4041345383546));
#60690=CARTESIAN_POINT('Ctrl Pts',(54.7766084561026,31.4416533848955,7.39991687794328));
#60691=CARTESIAN_POINT('Ctrl Pts',(54.8579051471828,31.4477313844269,7.39569921753196));
#60692=CARTESIAN_POINT('Ctrl Pts',(54.9393026906921,31.4497481680048,7.39148155712065));
#60693=CARTESIAN_POINT('Ctrl Pts',(55.0206985403457,31.4517649096141,7.38726398447743));
#60694=CARTESIAN_POINT('Ctrl Pts',(55.1021947738211,31.4497205929703,7.38304641183422));
#60695=CARTESIAN_POINT('Ctrl Pts',(55.1833576758483,31.4436305393221,7.378828839191));
#60696=CARTESIAN_POINT('Ctrl Pts',(55.264658356755,31.4375301474437,7.37460410696603));
#60697=CARTESIAN_POINT('Ctrl Pts',(55.3456241083945,31.4273703124783,7.37037937474106));
#60698=CARTESIAN_POINT('Ctrl Pts',(55.4258246986973,31.4132185097872,7.36615464251609));
#60699=CARTESIAN_POINT('Ctrl Pts',(55.5060052577411,31.3990702417137,7.36193096547917));
#60700=CARTESIAN_POINT('Ctrl Pts',(55.5854205879014,31.3809321242811,7.35770728844226));
#60701=CARTESIAN_POINT('Ctrl Pts',(55.6636533401404,31.3589223162539,7.35348361140535));
#60702=CARTESIAN_POINT('Ctrl Pts',(55.7420280340206,31.3368725747182,7.34925227113746));
#60703=CARTESIAN_POINT('Ctrl Pts',(55.8192154204152,31.310937252548,7.34502093086957));
#60704=CARTESIAN_POINT('Ctrl Pts',(55.8948151389593,31.281283874727,7.34078959060168));
#60705=CARTESIAN_POINT('Ctrl Pts',(55.9701975834504,31.2517157208949,7.33657041123156));
#60706=CARTESIAN_POINT('Ctrl Pts',(56.0440010929758,31.2184511171995,7.33235123186144));
#60707=CARTESIAN_POINT('Ctrl Pts',(56.1158539693795,31.1817012098406,7.32813205249133));
#60708=CARTESIAN_POINT('Ctrl Pts',(56.1879356429818,31.1448342817545,7.32389943821827));
#60709=CARTESIAN_POINT('Ctrl Pts',(56.2583223204356,31.1043226757462,7.31966682394521));
#60710=CARTESIAN_POINT('Ctrl Pts',(56.3266215515227,31.0603459682867,7.31543420967216));
#60711=CARTESIAN_POINT('Ctrl Pts',(56.3948233601778,31.016431989466,7.31120763282544));
#60712=CARTESIAN_POINT('Ctrl Pts',(56.4609432489158,30.9690629753186,7.30698105597871));
#60713=CARTESIAN_POINT('Ctrl Pts',(56.5246123690791,30.9184648482709,7.30275447913199));
#60714=CARTESIAN_POINT('Ctrl Pts',(56.5882108219746,30.8679228808087,7.2985325934234));
#60715=CARTESIAN_POINT('Ctrl Pts',(56.6493635493592,30.8141592094933,7.29431070771481));
#60716=CARTESIAN_POINT('Ctrl Pts',(56.707730961565,30.7574428050187,7.29008882200622));
#60717=CARTESIAN_POINT('Ctrl Pts',(56.7660590085238,30.7007646522876,7.28586978370114));
#60718=CARTESIAN_POINT('Ctrl Pts',(56.8216051389128,30.6411380444694,7.28165074539606));
#60719=CARTESIAN_POINT('Ctrl Pts',(56.8740641002604,30.5788711151057,7.27743170709098));
#60720=CARTESIAN_POINT('Ctrl Pts',(56.926505930422,30.5166245198532,7.27321404657014));
#60721=CARTESIAN_POINT('Ctrl Pts',(56.9758622945986,30.4517396703964,7.2689963860493));
#60722=CARTESIAN_POINT('Ctrl Pts',(57.0218669123456,30.3845592940579,7.26477872552846));
#60723=CARTESIAN_POINT('Ctrl Pts',(57.0678705727504,30.3173803157227,7.26056115277585));
#60724=CARTESIAN_POINT('Ctrl Pts',(57.1105223638987,30.2479062894376,7.25634358002325));
#60725=CARTESIAN_POINT('Ctrl Pts',(57.1495990226901,30.1765093674297,7.25212600727065));
#60726=CARTESIAN_POINT('Ctrl Pts',(57.1887420142307,30.1049912489257,7.24790127517525));
#60727=CARTESIAN_POINT('Ctrl Pts',(57.2242975069586,30.0315441136056,7.24367654307985));
#60728=CARTESIAN_POINT('Ctrl Pts',(57.2560878822445,29.9565655845731,7.23945181098445));
#60729=CARTESIAN_POINT('Ctrl Pts',(57.2878703192107,29.8816057782994,7.2352281338396));
#60730=CARTESIAN_POINT('Ctrl Pts',(57.3158893784778,29.8051157880412,7.23100445669475));
#60731=CARTESIAN_POINT('Ctrl Pts',(57.3400169694353,29.7275100224429,7.2267807795499));
#60732=CARTESIAN_POINT('Ctrl Pts',(57.364188336291,29.6497634528124,7.2225494391758));
#60733=CARTESIAN_POINT('Ctrl Pts',(57.3844540087452,29.5708975133715,7.21831809880169));
#60734=CARTESIAN_POINT('Ctrl Pts',(57.4007365544642,29.4913392372477,7.21408675842759));
#60735=CARTESIAN_POINT('Ctrl Pts',(57.41697230132,29.412009625422,7.20986757966034));
#60736=CARTESIAN_POINT('Ctrl Pts',(57.4292478004427,29.3319921139886,7.2056484008931));
#60737=CARTESIAN_POINT('Ctrl Pts',(57.4375378138133,29.2517134407027,7.20142922212585));
#60738=CARTESIAN_POINT('Ctrl Pts',(57.4458542252345,29.1711791344779,7.19719660814569));
#60739=CARTESIAN_POINT('Ctrl Pts',(57.4501906321446,29.0900824681324,7.19296399416552));
#60740=CARTESIAN_POINT('Ctrl Pts',(57.4504840175798,29.0088504003319,7.18873138018536));
#60741=CARTESIAN_POINT('Ctrl Pts',(57.4507769845281,28.9277342024496,7.18450480363166));
#60742=CARTESIAN_POINT('Ctrl Pts',(57.4470383823237,28.8464834473939,7.18027822707797));
#60743=CARTESIAN_POINT('Ctrl Pts',(57.4392569188675,28.7655305270256,7.17605165052427));
#60744=CARTESIAN_POINT('Ctrl Pts',(57.4314840914952,28.6846674504533,7.17182976474244));
#60745=CARTESIAN_POINT('Ctrl Pts',(57.4196773625136,28.6041020118625,7.16760787896062));
#60746=CARTESIAN_POINT('Ctrl Pts',(57.4038774784267,28.5242654955621,7.16338599317879));
#60747=CARTESIAN_POINT('Ctrl Pts',(57.3880882517584,28.4444828309965,7.15916695516493));
#60748=CARTESIAN_POINT('Ctrl Pts',(57.3683113094349,28.3654285667424,7.15494791715107));
#60749=CARTESIAN_POINT('Ctrl Pts',(57.3446389419345,28.2875265043777,7.1507288791372));
#60750=CARTESIAN_POINT('Ctrl Pts',(57.3209743049602,28.2096498819664,7.14651121890626));
#60751=CARTESIAN_POINT('Ctrl Pts',(57.2934169040895,28.1329251583408,7.14229355867531));
#60752=CARTESIAN_POINT('Ctrl Pts',(57.2621092643398,28.057762277242,7.13807589844436));
#60753=CARTESIAN_POINT('Ctrl Pts',(57.2308022760799,27.9826009602296,7.13385832597994));
#60754=CARTESIAN_POINT('Ctrl Pts',(57.1957453838109,27.9090018495065,7.12964075351552));
#60755=CARTESIAN_POINT('Ctrl Pts',(57.1571292135792,27.8373548237217,7.1254231810511));
#60756=CARTESIAN_POINT('Ctrl Pts',(57.1184474864727,27.7655861661161,7.12119844861021));
#60757=CARTESIAN_POINT('Ctrl Pts',(57.0761946134957,27.6957766350037,7.11697371616932));
#60758=CARTESIAN_POINT('Ctrl Pts',(57.0306074353041,27.6282916878259,7.11274898372843));
#60759=CARTESIAN_POINT('Ctrl Pts',(56.9850316473682,27.5608236022051,7.10852530686467));
#60760=CARTESIAN_POINT('Ctrl Pts',(56.9361235170756,27.4956792990654,7.10430163000091));
#60761=CARTESIAN_POINT('Ctrl Pts',(56.8841609282059,27.4331918283905,7.10007795313715));
#60762=CARTESIAN_POINT('Ctrl Pts',(56.8321040609197,27.3705909834609,7.09584661303768));
#60763=CARTESIAN_POINT('Ctrl Pts',(56.7769819752198,27.3106569473758,7.09161527293821));
#60764=CARTESIAN_POINT('Ctrl Pts',(56.7191107230254,27.2536871494548,7.08738393283874));
#60765=CARTESIAN_POINT('Ctrl Pts',(56.6614057773356,27.1968810675,7.08316475247929));
#60766=CARTESIAN_POINT('Ctrl Pts',(56.6009678400075,27.1430224503848,7.07894557211985));
#60767=CARTESIAN_POINT('Ctrl Pts',(56.5381411302798,27.0923647850436,7.07472639176041));
#60768=CARTESIAN_POINT('Ctrl Pts',(56.4751143809048,27.041545826177,7.07049377757077));
#60769=CARTESIAN_POINT('Ctrl Pts',(56.4094491918281,26.9937592464748,7.06626116338113));
#60770=CARTESIAN_POINT('Ctrl Pts',(56.3414694002919,26.9492903428129,7.06202854919149));
#60771=CARTESIAN_POINT('Ctrl Pts',(56.2735865755749,26.904884869886,7.0578019724304));
#60772=CARTESIAN_POINT('Ctrl Pts',(56.2033960912588,26.8637879261263,7.05357539566932));
#60773=CARTESIAN_POINT('Ctrl Pts',(56.1312545011445,26.8262443781234,7.04934881890823));
#60774=CARTESIAN_POINT('Ctrl Pts',(56.0591929801929,26.7887424992942,7.04512693317851));
#60775=CARTESIAN_POINT('Ctrl Pts',(55.9851850663174,26.7547863931242,7.04090504744879));
#60776=CARTESIAN_POINT('Ctrl Pts',(55.9096147140627,26.7245766719222,7.03668316171907));
#60777=CARTESIAN_POINT('Ctrl Pts',(55.8340953313802,26.6943873261256,7.03246412350433));
#60778=CARTESIAN_POINT('Ctrl Pts',(55.7570160335231,26.6679395188327,7.02824508528959));
#60779=CARTESIAN_POINT('Ctrl Pts',(55.6787825589831,26.6453865523997,7.02402604707484));
#60780=CARTESIAN_POINT('Ctrl Pts',(55.6005746326758,26.6228409509526,7.0198083866459));
#60781=CARTESIAN_POINT('Ctrl Pts',(55.5212137242396,26.604187793001,7.01559072621695));
#60782=CARTESIAN_POINT('Ctrl Pts',(55.4411212955882,26.5895306986857,7.011373065788));
#60783=CARTESIAN_POINT('Ctrl Pts',(55.3610305336629,26.574873909385,7.00715549312872));
#60784=CARTESIAN_POINT('Ctrl Pts',(55.2802087389603,26.56421310085,7.00293792046943));
#60785=CARTESIAN_POINT('Ctrl Pts',(55.1990867285295,26.5576006214127,6.99872034781014));
#60786=CARTESIAN_POINT('Ctrl Pts',(55.1178270094009,26.5509769169587,6.99449561560887));
#60787=CARTESIAN_POINT('Ctrl Pts',(55.0362665203414,26.5484153292952,6.99027088340761));
#60788=CARTESIAN_POINT('Ctrl Pts',(54.9548407524154,26.5499161458518,6.98604615120634));
#60789=CARTESIAN_POINT('Ctrl Pts',(54.8734353210632,26.5514165875706,6.98182247415728));
#60790=CARTESIAN_POINT('Ctrl Pts',(54.7921650071736,26.5569773515209,6.97759879710821));
#60791=CARTESIAN_POINT('Ctrl Pts',(54.7114604616645,26.5665466544811,6.97337512005915));
#60792=CARTESIAN_POINT('Ctrl Pts',(54.6306094898613,26.5761333195064,6.96914377978153));
#60793=CARTESIAN_POINT('Ctrl Pts',(54.5503267972118,26.5897429803003,6.9649124395039));
#60794=CARTESIAN_POINT('Ctrl Pts',(54.4710339338915,26.607272445324,6.96068109922628));
#60795=CARTESIAN_POINT('Ctrl Pts',(54.3919689606695,26.6247515301327,6.95646191994917));
#60796=CARTESIAN_POINT('Ctrl Pts',(54.3138885519046,26.6461277175504,6.95224274067206));
#60797=CARTESIAN_POINT('Ctrl Pts',(54.2371927317533,26.6712502664498,6.94802356139495));
#60798=CARTESIAN_POINT('Ctrl Pts',(54.1602526807823,26.6964528158069,6.9437909465276));
#60799=CARTESIAN_POINT('Ctrl Pts',(54.0844198979967,26.7255193857952,6.93955833166025));
#60800=CARTESIAN_POINT('Ctrl Pts',(54.0101099949605,26.7583336492861,6.93532571679289));
#60801=CARTESIAN_POINT('Ctrl Pts',(53.9359060879517,26.791101106343,6.93109913934912));
#60802=CARTESIAN_POINT('Ctrl Pts',(53.863221167765,26.8276054534984,6.92687256190536));
#60803=CARTESIAN_POINT('Ctrl Pts',(53.7924547429285,26.867680909872,6.92264598446159));
#60804=CARTESIAN_POINT('Ctrl Pts',(53.7217668752385,26.9077118788563,6.91842409890192));
#60805=CARTESIAN_POINT('Ctrl Pts',(53.6529936733689,26.9513058523189,6.91420221334225));
#60806=CARTESIAN_POINT('Ctrl Pts',(53.58651244099,26.9982499730176,6.90998032778258));
#60807=CARTESIAN_POINT('Ctrl Pts',(53.520076034353,27.0451624410985,6.90576128887821));
#60808=CARTESIAN_POINT('Ctrl Pts',(53.4559289064382,27.0954203028341,6.90154224997385));
#60809=CARTESIAN_POINT('Ctrl Pts',(53.3944205355582,27.1487666723606,6.89732321106948));
#60810=CARTESIAN_POINT('Ctrl Pts',(53.3329322510764,27.202095620902,6.89310554994986));
#60811=CARTESIAN_POINT('Ctrl Pts',(53.2740813629766,27.2585107700868,6.88888788883023));
#60812=CARTESIAN_POINT('Ctrl Pts',(53.2181842347152,27.3177149978132,6.88467022771061));
#60813=CARTESIAN_POINT('Ctrl Pts',(53.1622882696734,27.3769179934993,6.88045265436053));
#60814=CARTESIAN_POINT('Ctrl Pts',(53.1093462603175,27.4389096137375,6.87623508101046));
#60815=CARTESIAN_POINT('Ctrl Pts',(53.0596366549587,27.5033569766908,6.87201750766039));
#60816=CARTESIAN_POINT('Ctrl Pts',(53.0098426828071,27.5679137192554,6.86779277627448));
#60817=CARTESIAN_POINT('Ctrl Pts',(52.963292376095,27.634934173688,6.86356804488858));
#60818=CARTESIAN_POINT('Ctrl Pts',(52.9202230574265,27.7040531958682,6.85934331350267));
#60819=CARTESIAN_POINT('Ctrl Pts',(52.8771644802957,27.7731549796846,6.85511963576964));
#60820=CARTESIAN_POINT('Ctrl Pts',(52.8375853630188,27.8443538668529,6.85089595803661));
#60821=CARTESIAN_POINT('Ctrl Pts',(52.8016767153071,27.9172604255977,6.84667228030358));
#60822=CARTESIAN_POINT('Ctrl Pts',(52.7657029168312,27.990299262173,6.84244093935153));
#60823=CARTESIAN_POINT('Ctrl Pts',(52.7334130814668,28.0650515344894,6.83820959839948));
#60824=CARTESIAN_POINT('Ctrl Pts',(52.7049501418823,28.1411074579705,6.83397825744744));
#60825=CARTESIAN_POINT('Ctrl Pts',(52.6765690357659,28.2169447139463,6.82975908197479));
#60826=CARTESIAN_POINT('Ctrl Pts',(52.6519929084458,28.2940776758606,6.82553990650215));
#60827=CARTESIAN_POINT('Ctrl Pts',(52.6313130877515,28.3720887309958,6.82132073102951));
#60828=CARTESIAN_POINT('Ctrl Pts',(52.6043609741696,28.4737609287255,6.81582185856627));
#60829=CARTESIAN_POINT('Ctrl Pts',(52.583942728695,28.577232327224,6.81032298610304));
#60830=CARTESIAN_POINT('Ctrl Pts',(52.570251424349,28.6817672092287,6.80482411363981));
#60831=CARTESIAN_POINT('Ctrl Pts',(52.5565601200031,28.7863020912335,6.79932524117658));
#60832=CARTESIAN_POINT('Ctrl Pts',(52.5495959378341,28.8919007970249,6.79382636871335));
#60833=CARTESIAN_POINT('Ctrl Pts',(52.5495009849895,28.9978028581341,6.78832749625011));
#60834=CARTESIAN_POINT('',(52.5495001872432,29.0009579555037,5.9883274961685));
#60835=CARTESIAN_POINT('Ctrl Pts',(52.5495009849888,28.9978028588672,6.78832749621205));
#60836=CARTESIAN_POINT('Ctrl Pts',(52.5494288600355,29.078244722314,6.78415062238013));
#60837=CARTESIAN_POINT('Ctrl Pts',(52.5533219557559,29.1587813112267,6.77997374854822));
#60838=CARTESIAN_POINT('Ctrl Pts',(52.5611815322018,29.2389868848418,6.7757968747163));
#60839=CARTESIAN_POINT('Ctrl Pts',(52.5690366754036,29.3191472179931,6.77162235687663));
#60840=CARTESIAN_POINT('Ctrl Pts',(52.5808538141535,29.3989764342918,6.76744783903695));
#60841=CARTESIAN_POINT('Ctrl Pts',(52.5965821798488,29.4780512857214,6.76327332119728));
#60842=CARTESIAN_POINT('Ctrl Pts',(52.6123067321063,29.5571069649721,6.75909981549485));
#60843=CARTESIAN_POINT('Ctrl Pts',(52.6319405357407,29.6354081765147,6.75492630979243));
#60844=CARTESIAN_POINT('Ctrl Pts',(52.6553815221646,29.7125408362983,6.75075280409001));
#60845=CARTESIAN_POINT('Ctrl Pts',(52.6788243637717,29.7896796005698,6.74657896808502));
#60846=CARTESIAN_POINT('Ctrl Pts',(52.7060748458035,29.8656491754188,6.74240513208003));
#60847=CARTESIAN_POINT('Ctrl Pts',(52.7369812040606,29.94005115777,6.73823129607504));
#60848=CARTESIAN_POINT('Ctrl Pts',(52.7679195171146,30.0145300660479,6.73405314464468));
#60849=CARTESIAN_POINT('Ctrl Pts',(52.8025210667272,30.0874377078138,6.72987499321432));
#60850=CARTESIAN_POINT('Ctrl Pts',(52.8405864519799,30.1583969003011,6.72569684178396));
#60851=CARTESIAN_POINT('Ctrl Pts',(52.8786740011369,30.2293974094004,6.7215162575883));
#60852=CARTESIAN_POINT('Ctrl Pts',(52.9202291526092,30.2984468056787,6.71733567339264));
#60853=CARTESIAN_POINT('Ctrl Pts',(52.965008511472,30.365195916936,6.71315508919698));
#60854=CARTESIAN_POINT('Ctrl Pts',(53.0098618370269,30.4320552845945,6.70896759949861));
#60855=CARTESIAN_POINT('Ctrl Pts',(53.0579497132379,30.4966064052028,6.70478010980025));
#60856=CARTESIAN_POINT('Ctrl Pts',(53.1089881508435,30.558532783213,6.70059262010189));
#60857=CARTESIAN_POINT('Ctrl Pts',(53.133262068887,30.5879850136314,6.69860104695594));
#60858=CARTESIAN_POINT('Ctrl Pts',(53.158202847914,30.6168440727045,6.69660947381));
#60859=CARTESIAN_POINT('Ctrl Pts',(53.1837771558477,30.6450789739035,6.69461790066405));
#60860=CARTESIAN_POINT('Ctrl Pts',(53.2381292618132,30.7050855377514,6.69038528584816));
#60861=CARTESIAN_POINT('Ctrl Pts',(53.2955594916946,30.7625071746051,6.68615267103227));
#60862=CARTESIAN_POINT('Ctrl Pts',(53.3557923422701,30.8170116753236,6.68192005621637));
#60863=CARTESIAN_POINT('Ctrl Pts',(53.4159392761671,30.8714384303332,6.67769347884023));
#60864=CARTESIAN_POINT('Ctrl Pts',(53.4788805492502,30.9229560044402,6.67346690146409));
#60865=CARTESIAN_POINT('Ctrl Pts',(53.5443020495218,30.9712670359374,6.66924032408795));
#60866=CARTESIAN_POINT('Ctrl Pts',(53.6096509272737,31.0195244387526,6.66501843851339));
#60867=CARTESIAN_POINT('Ctrl Pts',(53.6774741897334,31.0645820970959,6.66079655293884));
#60868=CARTESIAN_POINT('Ctrl Pts',(53.7474237724054,31.1061821013542,6.65657466736428));
#60869=CARTESIAN_POINT('Ctrl Pts',(53.8173261887602,31.1477540551379,6.65235562856574));
#60870=CARTESIAN_POINT('Ctrl Pts',(53.8893516795222,31.1858727484733,6.64813658976719));
#60871=CARTESIAN_POINT('Ctrl Pts',(53.9631233002723,31.2203236159537,6.64391755096865));
#60872=CARTESIAN_POINT('Ctrl Pts',(54.0368708296467,31.2547632329183,6.63969988996888));
#60873=CARTESIAN_POINT('Ctrl Pts',(54.1123629359801,31.2855372063541,6.63548222896912));
#60874=CARTESIAN_POINT('Ctrl Pts',(54.1891994127194,31.3124776015489,6.63126456796936));
#60875=CARTESIAN_POINT('Ctrl Pts',(54.2660342902399,31.3394174360258,6.62704699475293));
#60876=CARTESIAN_POINT('Ctrl Pts',(54.3442130437623,31.362523698306,6.62282942153651));
#60877=CARTESIAN_POINT('Ctrl Pts',(54.4233182479969,31.3816776454648,6.61861184832009));
#60878=CARTESIAN_POINT('Ctrl Pts',(54.5025577137125,31.4008641017023,6.6143871168183));
#60879=CARTESIAN_POINT('Ctrl Pts',(54.5827263223072,31.4160847116326,6.61016238531651));
#60880=CARTESIAN_POINT('Ctrl Pts',(54.6633939314659,31.4272714320047,6.60593765381472));
#60881=CARTESIAN_POINT('Ctrl Pts',(54.7440414166564,31.4384553616506,6.60171397624726));
#60882=CARTESIAN_POINT('Ctrl Pts',(54.8251871872543,31.4456073943768,6.59749029867979));
#60883=CARTESIAN_POINT('Ctrl Pts',(54.9063977799338,31.4487116764533,6.59326662111233));
#60884=CARTESIAN_POINT('Ctrl Pts',(54.9877557165144,31.4518215907634,6.58903528034344));
#60885=CARTESIAN_POINT('Ctrl Pts',(55.0691782443495,31.4508690831215,6.58480393957455));
#60886=CARTESIAN_POINT('Ctrl Pts',(55.1502328912408,31.4458904980374,6.58057259880565));
#60887=CARTESIAN_POINT('Ctrl Pts',(55.2310545156928,31.4409262257913,6.57635342263664));
#60888=CARTESIAN_POINT('Ctrl Pts',(55.3115099283703,31.4319591272632,6.57213424646762));
#60889=CARTESIAN_POINT('Ctrl Pts',(55.3911805236031,31.4190758665147,6.56791507029861));
#60890=CARTESIAN_POINT('Ctrl Pts',(55.4711049550331,31.4061515587787,6.56368245153347));
#60891=CARTESIAN_POINT('Ctrl Pts',(55.5505368141948,31.3892379989933,6.55944983276834));
#60892=CARTESIAN_POINT('Ctrl Pts',(55.629047450847,31.3683854320154,6.55521721400321));
#60893=CARTESIAN_POINT('Ctrl Pts',(55.707446100048,31.347562609107,6.55099063263896));
#60894=CARTESIAN_POINT('Ctrl Pts',(55.7849256913231,31.3228120565172,6.54676405127471));
#60895=CARTESIAN_POINT('Ctrl Pts',(55.8610657867765,31.294235376077,6.54253746991046));
#60896=CARTESIAN_POINT('Ctrl Pts',(55.9371212716691,31.2656904514277,6.53831558532807));
#60897=CARTESIAN_POINT('Ctrl Pts',(56.0118397857047,31.233328009683,6.53409370074568));
#60898=CARTESIAN_POINT('Ctrl Pts',(56.0848155021396,31.1972996100481,6.52987181616329));
#60899=CARTESIAN_POINT('Ctrl Pts',(56.1577420989467,31.1612954609677,6.5256527733125));
#60900=CARTESIAN_POINT('Ctrl Pts',(56.2289278124649,31.1216304597929,6.5214337304617));
#60901=CARTESIAN_POINT('Ctrl Pts',(56.2979874505031,31.0785039880492,6.51721468761091));
#60902=CARTESIAN_POINT('Ctrl Pts',(56.3670245362098,31.0353915998211,6.51299702254395));
#60903=CARTESIAN_POINT('Ctrl Pts',(56.4339365315444,30.9888202317808,6.50877935747699));
#60904=CARTESIAN_POINT('Ctrl Pts',(56.4983646954293,30.9390341640856,6.50456169241003));
#60905=CARTESIAN_POINT('Ctrl Pts',(56.5627915184957,30.8892491324913,6.50034411511716));
#60906=CARTESIAN_POINT('Ctrl Pts',(56.6247342460189,30.8362498192367,6.49612653782428));
#60907=CARTESIAN_POINT('Ctrl Pts',(56.683866026361,30.780321728022,6.4919089605314));
#60908=CARTESIAN_POINT('Ctrl Pts',(56.7430980439055,30.7242988303367,6.48768423381488));
#60909=CARTESIAN_POINT('Ctrl Pts',(56.7995092414239,30.6653375423788,6.48345950709836));
#60910=CARTESIAN_POINT('Ctrl Pts',(56.8528083740854,30.6037616340713,6.47923478038184));
#60911=CARTESIAN_POINT('Ctrl Pts',(56.9060943218714,30.5422009581071,6.47501109875729));
#60912=CARTESIAN_POINT('Ctrl Pts',(56.956269473905,30.4780273355217,6.47078741713273));
#60913=CARTESIAN_POINT('Ctrl Pts',(57.0030845534015,30.411595736011,6.46656373550818));
#60914=CARTESIAN_POINT('Ctrl Pts',(57.0499845709571,30.3450436075769,6.4623323907263));
#60915=CARTESIAN_POINT('Ctrl Pts',(57.0935120837138,30.2762257088127,6.45810104594442));
#60916=CARTESIAN_POINT('Ctrl Pts',(57.1334621396473,30.20552459481,6.45386970116254));
#60917=CARTESIAN_POINT('Ctrl Pts',(57.1732970944237,30.1350271796465,6.44965054741941));
#60918=CARTESIAN_POINT('Ctrl Pts',(57.2095750493838,30.0626578305374,6.44543139367628));
#60919=CARTESIAN_POINT('Ctrl Pts',(57.2421408135098,29.9888148574904,6.44121223993315));
#60920=CARTESIAN_POINT('Ctrl Pts',(57.2748103779279,29.9147365169531,6.43697963803664));
#60921=CARTESIAN_POINT('Ctrl Pts',(57.3038655318623,29.8388996131088,6.43274703614012));
#60922=CARTESIAN_POINT('Ctrl Pts',(57.3291150640083,29.7616910585072,6.42851443424361));
#60923=CARTESIAN_POINT('Ctrl Pts',(57.3543285799335,29.6845926350686,6.42428786977873));
#60924=CARTESIAN_POINT('Ctrl Pts',(57.3757471123381,29.6061268846802,6.42006130531384));
#60925=CARTESIAN_POINT('Ctrl Pts',(57.3932270001455,29.5267017901758,6.41583474084896));
#60926=CARTESIAN_POINT('Ctrl Pts',(57.4106875507256,29.4473645601437,6.41161285204557));
#60927=CARTESIAN_POINT('Ctrl Pts',(57.4242180148205,29.3670705461218,6.40739096324219));
#60928=CARTESIAN_POINT('Ctrl Pts',(57.4337245898435,29.2862426781441,6.40316907443881));
#60929=CARTESIAN_POINT('Ctrl Pts',(57.4432247185924,29.2054696184003,6.39895004843849));
#60930=CARTESIAN_POINT('Ctrl Pts',(57.4487063234812,29.1241638838749,6.39473102243817));
#60931=CARTESIAN_POINT('Ctrl Pts',(57.4501269514733,29.0427571241308,6.39051199643785));
#60932=CARTESIAN_POINT('Ctrl Pts',(57.4515471155577,28.9613769478611,6.38629434816551));
#60933=CARTESIAN_POINT('Ctrl Pts',(57.4489089282322,28.8798962760132,6.38207669989316));
#60934=CARTESIAN_POINT('Ctrl Pts',(57.4422219985723,28.7987490131965,6.37785905162082));
#60935=CARTESIAN_POINT('Ctrl Pts',(57.4355352079506,28.7176034376365,6.37364149104405));
#60936=CARTESIAN_POINT('Ctrl Pts',(57.4247998816956,28.6367917202094,6.36942393046728));
#60937=CARTESIAN_POINT('Ctrl Pts',(57.4100775688688,28.556743457989,6.36520636989052));
#60938=CARTESIAN_POINT('Ctrl Pts',(57.3953301713377,28.4765588050395,6.36098162319695));
#60939=CARTESIAN_POINT('Ctrl Pts',(57.3765822798807,28.3971406692574,6.35675687650338));
#60940=CARTESIAN_POINT('Ctrl Pts',(57.3539469297499,28.3189096227952,6.35253212980982));
#60941=CARTESIAN_POINT('Ctrl Pts',(57.3313173736756,28.2406986014307,6.34830846454068));
#60942=CARTESIAN_POINT('Ctrl Pts',(57.3048025207277,28.1636744955753,6.34408479927155));
#60943=CARTESIAN_POINT('Ctrl Pts',(57.2745644219918,28.0882396475998,6.33986113400242));
#60944=CARTESIAN_POINT('Ctrl Pts',(57.2442714586458,28.0126679291299,6.33562980523069));
#60945=CARTESIAN_POINT('Ctrl Pts',(57.2102419435187,27.9386916545432,6.33139847645896));
#60946=CARTESIAN_POINT('Ctrl Pts',(57.1726851973896,27.86669100284,6.32716714768723));
#60947=CARTESIAN_POINT('Ctrl Pts',(57.135235696081,27.7948959519343,6.32294790164739));
#60948=CARTESIAN_POINT('Ctrl Pts',(57.0942793833322,27.7250656066502,6.31872865560755));
#60949=CARTESIAN_POINT('Ctrl Pts',(57.0500659050149,27.6575470082363,6.31450940956771));
#60950=CARTESIAN_POINT('Ctrl Pts',(57.0057122524442,27.5898143490996,6.31027678684532));
#60951=CARTESIAN_POINT('Ctrl Pts',(56.9579157577534,27.5241562099011,6.30604416412293));
#60952=CARTESIAN_POINT('Ctrl Pts',(56.9068968804013,27.4609436210731,6.30181154140054));
#60953=CARTESIAN_POINT('Ctrl Pts',(56.8559507776077,27.397821200208,6.2975849561934));
#60954=CARTESIAN_POINT('Ctrl Pts',(56.8017917107017,27.3371377598075,6.29335837098627));
#60955=CARTESIAN_POINT('Ctrl Pts',(56.7446836997035,27.2792359144877,6.28913178577912));
#60956=CARTESIAN_POINT('Ctrl Pts',(56.6876392149322,27.2213984784462,6.28490990217175));
#60957=CARTESIAN_POINT('Ctrl Pts',(56.6276526288117,27.1663368182792,6.28068801856439));
#60958=CARTESIAN_POINT('Ctrl Pts',(56.5650276366769,27.1143598576511,6.27646613495702));
#60959=CARTESIAN_POINT('Ctrl Pts',(56.5024447301628,27.0624178268901,6.27224708856505));
#60960=CARTESIAN_POINT('Ctrl Pts',(56.4372272955657,27.0135566745421,6.26802804217309));
#60961=CARTESIAN_POINT('Ctrl Pts',(56.3697143025282,26.9680470036318,6.26380899578113));
#60962=CARTESIAN_POINT('Ctrl Pts',(56.3022233586583,26.9225521957918,6.25959132729372));
#60963=CARTESIAN_POINT('Ctrl Pts',(56.2324387301324,26.8804069551102,6.25537365880631));
#60964=CARTESIAN_POINT('Ctrl Pts',(56.1607296208659,26.8418394412731,6.2511559903189));
#60965=CARTESIAN_POINT('Ctrl Pts',(56.0890220060584,26.803272731205,6.24693840973012));
#60966=CARTESIAN_POINT('Ctrl Pts',(56.0153903999367,26.7682838187407,6.24272082914134));
#60967=CARTESIAN_POINT('Ctrl Pts',(55.9402286694053,26.7370549500201,6.23850324855256));
#60968=CARTESIAN_POINT('Ctrl Pts',(55.8649396634547,26.7057731997689,6.2342785261067));
#60969=CARTESIAN_POINT('Ctrl Pts',(55.788115780296,26.6782644114158,6.23005380366084));
#60970=CARTESIAN_POINT('Ctrl Pts',(55.7101713327564,26.6546627261456,6.22582908121498));
#60971=CARTESIAN_POINT('Ctrl Pts',(55.6322460333196,26.631066838947,6.22160539662906));
#60972=CARTESIAN_POINT('Ctrl Pts',(55.5532011774512,26.6113762274964,6.21738171204314));
#60973=CARTESIAN_POINT('Ctrl Pts',(55.4734624837417,26.5956739974602,6.21315802745723));
#60974=CARTESIAN_POINT('Ctrl Pts',(55.393579121926,26.5799432792236,6.20892667993601));
#60975=CARTESIAN_POINT('Ctrl Pts',(55.3129998676101,26.5682154704624,6.2046953324148));
#60976=CARTESIAN_POINT('Ctrl Pts',(55.2321575821357,26.56052196012,6.20046398489359));
#60977=CARTESIAN_POINT('Ctrl Pts',(55.1515486193776,26.552850654379,6.19624484966314));
#60978=CARTESIAN_POINT('Ctrl Pts',(55.0706786002372,26.5491903285429,6.19202571443269));
#60979=CARTESIAN_POINT('Ctrl Pts',(54.9899745035598,26.5495205082635,6.18780657920225));
#60980=CARTESIAN_POINT('Ctrl Pts',(54.9090120275628,26.5498517450756,6.18357393614091));
#60981=CARTESIAN_POINT('Ctrl Pts',(54.8279154383746,26.554200339424,6.17934129307957));
#60982=CARTESIAN_POINT('Ctrl Pts',(54.7471159881272,26.5625833498273,6.17510865001823));
#60983=CARTESIAN_POINT('Ctrl Pts',(54.6664317859521,26.570954403147,6.17088204417561));
#60984=CARTESIAN_POINT('Ctrl Pts',(54.586044339172,26.5833483958408,6.16665543833299));
#60985=CARTESIAN_POINT('Ctrl Pts',(54.5063847778751,26.5997303771271,6.16242883249037));
#60986=CARTESIAN_POINT('Ctrl Pts',(54.426814313883,26.616094035561,6.1582069540048));
#60987=CARTESIAN_POINT('Ctrl Pts',(54.3479705703504,26.6364367260928,6.15398507551924));
#60988=CARTESIAN_POINT('Ctrl Pts',(54.270278007529,26.660671877717,6.14976319703367));
#60989=CARTESIAN_POINT('Ctrl Pts',(54.192637171885,26.6848908937428,6.14554412944595));
#60990=CARTESIAN_POINT('Ctrl Pts',(54.1161464371773,26.712997086288,6.14132506185822));
#60991=CARTESIAN_POINT('Ctrl Pts',(54.041217330246,26.7448534322179,6.1371059942705));
#60992=CARTESIAN_POINT('Ctrl Pts',(53.9663126915176,26.7766993754142,6.1328883044251));
#60993=CARTESIAN_POINT('Ctrl Pts',(53.8929690950125,26.8122928583612,6.12867061457969));
#60994=CARTESIAN_POINT('Ctrl Pts',(53.8215789243146,26.8514483905709,6.12445292473428));
#60995=CARTESIAN_POINT('Ctrl Pts',(53.7501902391895,26.890603107985,6.12023532265566));
#60996=CARTESIAN_POINT('Ctrl Pts',(53.6807553057858,26.9333195028628,6.11601772057704));
#60997=CARTESIAN_POINT('Ctrl Pts',(53.6136414206032,26.9793664015134,6.11180011849842));
#60998=CARTESIAN_POINT('Ctrl Pts',(53.5464146278028,27.025490766185,6.10757542102661));
#60999=CARTESIAN_POINT('Ctrl Pts',(53.4815170806266,27.0749565805098,6.10335072355481));
#61000=CARTESIAN_POINT('Ctrl Pts',(53.4192868435943,27.1274893412411,6.09912602608301));
#61001=CARTESIAN_POINT('Ctrl Pts',(53.3570712084832,27.1800097755009,6.09490231990905));
#61002=CARTESIAN_POINT('Ctrl Pts',(53.297521958275,27.2355953835484,6.09067861373509));
#61003=CARTESIAN_POINT('Ctrl Pts',(53.2409405682616,27.2939343020821,6.08645490756113));
#61004=CARTESIAN_POINT('Ctrl Pts',(53.1842565259842,27.3523790614596,6.08222353856728));
#61005=CARTESIAN_POINT('Ctrl Pts',(53.13055141174,27.4135867638002,6.07799216957343));
#61006=CARTESIAN_POINT('Ctrl Pts',(53.080087208073,27.4772113996372,6.07376080057958));
#61007=CARTESIAN_POINT('Ctrl Pts',(53.0297703139504,27.5406503094458,6.06954178333199));
#61008=CARTESIAN_POINT('Ctrl Pts',(52.9826756319443,27.6064916426494,6.06532276608439));
#61009=CARTESIAN_POINT('Ctrl Pts',(52.9390184174073,27.6743661266346,6.0611037488368));
#61010=CARTESIAN_POINT('Ctrl Pts',(52.8942488691094,27.7439699715248,6.05677723606133));
#61011=CARTESIAN_POINT('Ctrl Pts',(52.8529333346666,27.8159616604484,6.05245072328586));
#61012=CARTESIAN_POINT('Ctrl Pts',(52.8153283562073,27.8899729468124,6.04812421051039));
#61013=CARTESIAN_POINT('Ctrl Pts',(52.7777843730217,27.963864186873,6.04380471533846));
#61014=CARTESIAN_POINT('Ctrl Pts',(52.7439391787127,28.0397681264347,6.03948522016654));
#61015=CARTESIAN_POINT('Ctrl Pts',(52.7140055440341,28.1172884971333,6.03516572499462));
#61016=CARTESIAN_POINT('Ctrl Pts',(52.6841225849363,28.1946776311863,6.03085354243036));
#61017=CARTESIAN_POINT('Ctrl Pts',(52.6581381619751,28.2736773444822,6.0265413598661));
#61018=CARTESIAN_POINT('Ctrl Pts',(52.636218034592,28.353869154109,6.02222917730185));
#61019=CARTESIAN_POINT('Ctrl Pts',(52.614319784242,28.4339809295804,6.01792129844256));
#61020=CARTESIAN_POINT('Ctrl Pts',(52.5964778819453,28.5152820169277,6.01361341958326));
#61021=CARTESIAN_POINT('Ctrl Pts',(52.5828089271904,28.5973369056775,6.00930554072397));
#61022=CARTESIAN_POINT('Ctrl Pts',(52.5691514667886,28.6793227936964,6.0050012844007));
#61023=CARTESIAN_POINT('Ctrl Pts',(52.5596600446458,28.7620607920093,6.00069702807742));
#61024=CARTESIAN_POINT('Ctrl Pts',(52.5544003556719,28.845104455641,5.99639277175415));
#61025=CARTESIAN_POINT('Ctrl Pts',(52.5511151702141,28.8969732709803,5.99370434657345));
#61026=CARTESIAN_POINT('Ctrl Pts',(52.549479860527,28.9489611166896,5.99101592139276));
#61027=CARTESIAN_POINT('Ctrl Pts',(52.5495001872428,29.0009579546612,5.98832749621206));
#61028=CARTESIAN_POINT('Ctrl Pts',(52.5495001872432,29.0009579555037,5.9883274961685));
#61029=CARTESIAN_POINT('Ctrl Pts',(52.5495348804631,29.0897050095589,5.98373895147723));
#61030=CARTESIAN_POINT('Ctrl Pts',(52.5543948630893,29.1783029161916,5.97915040678597));
#61031=CARTESIAN_POINT('Ctrl Pts',(52.5640065805463,29.2662448316463,5.97456186209471));
#61032=CARTESIAN_POINT('Ctrl Pts',(52.5736441829486,29.354423580079,5.96996096017084));
#61033=CARTESIAN_POINT('Ctrl Pts',(52.5880590237614,29.4419424892432,5.96536005824698));
#61034=CARTESIAN_POINT('Ctrl Pts',(52.6071265666039,29.5283057653925,5.96075915632312));
#61035=CARTESIAN_POINT('Ctrl Pts',(52.6262757077358,29.6150386274747,5.95613856514353));
#61036=CARTESIAN_POINT('Ctrl Pts',(52.6501173215307,29.700605641685,5.95151797396394));
#61037=CARTESIAN_POINT('Ctrl Pts',(52.6784764616596,29.7845245126389,5.94689738278434));
#61038=CARTESIAN_POINT('Ctrl Pts',(52.7040423808818,29.8601778316844,5.94273189468001));
#61039=CARTESIAN_POINT('Ctrl Pts',(52.7332790280157,29.9344918007638,5.93856640657567));
#61040=CARTESIAN_POINT('Ctrl Pts',(52.7660259964594,30.0071297838435,5.93440091847134));
#61041=CARTESIAN_POINT('Ctrl Pts',(52.7993013887138,30.0809398949598,5.9301682136687));
#61042=CARTESIAN_POINT('Ctrl Pts',(52.8363005913983,30.1532363580626,5.92593550886607));
#61043=CARTESIAN_POINT('Ctrl Pts',(52.8768635501333,30.2236183495059,5.92170280406344));
#61044=CARTESIAN_POINT('Ctrl Pts',(52.9173686453212,30.2938999401942,5.91747613726498));
#61045=CARTESIAN_POINT('Ctrl Pts',(52.9614271695572,30.3622720842524,5.91324947046653));
#61046=CARTESIAN_POINT('Ctrl Pts',(53.0088316173746,30.4283552506408,5.90902280366807));
#61047=CARTESIAN_POINT('Ctrl Pts',(53.0561821895524,30.4943633128349,5.90480094051965));
#61048=CARTESIAN_POINT('Ctrl Pts',(53.1068708588622,30.5580871916842,5.90057907737122));
#61049=CARTESIAN_POINT('Ctrl Pts',(53.1606457045262,30.6191744889672,5.8963572142228));
#61050=CARTESIAN_POINT('Ctrl Pts',(53.2143856893116,30.6802221848933,5.89213808800196));
#61051=CARTESIAN_POINT('Ctrl Pts',(53.2712075719737,30.7386363451589,5.88791896178113));
#61052=CARTESIAN_POINT('Ctrl Pts',(53.3308186070495,30.7940969113813,5.8836998355603));
#61053=CARTESIAN_POINT('Ctrl Pts',(53.3904101622112,30.8495393539951,5.87948208808111));
#61054=CARTESIAN_POINT('Ctrl Pts',(53.4527887198652,30.9020298031947,5.87526434060193));
#61055=CARTESIAN_POINT('Ctrl Pts',(53.5176250644263,30.9512854225825,5.87104659312274));
#61056=CARTESIAN_POINT('Ctrl Pts',(53.5824600433415,31.0005400045007,5.86682893448183));
#61057=CARTESIAN_POINT('Ctrl Pts',(53.6497523356319,31.046559612006,5.86261127584092));
#61058=CARTESIAN_POINT('Ctrl Pts',(53.71914121885,31.0891029253608,5.85839361720001));
#61059=CARTESIAN_POINT('Ctrl Pts',(53.7886447524352,31.1317165324899,5.8541689897755));
#61060=CARTESIAN_POINT('Ctrl Pts',(53.8602514094746,31.1708421100769,5.84994436235099));
#61061=CARTESIAN_POINT('Ctrl Pts',(53.9335728330193,31.2062826989136,5.84571973492648));
#61062=CARTESIAN_POINT('Ctrl Pts',(54.0068791943299,31.24171600728,5.84149597535647));
#61063=CARTESIAN_POINT('Ctrl Pts',(54.0818991803267,31.2734656782613,5.83727221578646));
#61064=CARTESIAN_POINT('Ctrl Pts',(54.1582251784986,31.3013833665616,5.83304845621645));
#61065=CARTESIAN_POINT('Ctrl Pts',(54.2346896069915,31.3293516883897,5.82881703613224));
#61066=CARTESIAN_POINT('Ctrl Pts',(54.3124643364177,31.3534740002599,5.82458561604803));
#61067=CARTESIAN_POINT('Ctrl Pts',(54.3911266505643,31.3736519320126,5.82035419596382));
#61068=CARTESIAN_POINT('Ctrl Pts',(54.4695525463929,31.3937692193164,5.81613549334452));
#61069=CARTESIAN_POINT('Ctrl Pts',(54.5488602366159,31.409965794223,5.81191679072521));
#61070=CARTESIAN_POINT('Ctrl Pts',(54.6286248968841,31.4221954468593,5.8076980881059));
#61071=CARTESIAN_POINT('Ctrl Pts',(54.7086557912035,31.4344659189505,5.80346530453539));
#61072=CARTESIAN_POINT('Ctrl Pts',(54.7894442047976,31.442788526944,5.79923252096488));
#61073=CARTESIAN_POINT('Ctrl Pts',(54.8705667614793,31.4470793380612,5.79499973739437));
#61074=CARTESIAN_POINT('Ctrl Pts',(54.9515736403356,31.4513640306373,5.79077298961981));
#61075=CARTESIAN_POINT('Ctrl Pts',(55.0329132559281,31.4516283206803,5.78654624184525));
#61076=CARTESIAN_POINT('Ctrl Pts',(55.1141542634911,31.4478396708377,5.78231949407068));
#61077=CARTESIAN_POINT('Ctrl Pts',(55.1953017187549,31.4440553837783,5.77809761356678));
#61078=CARTESIAN_POINT('Ctrl Pts',(55.2763503300436,31.4362274541488,5.77387573306287));
#61079=CARTESIAN_POINT('Ctrl Pts',(55.3568673555319,31.4243753712154,5.76965385255896));
#61080=CARTESIAN_POINT('Ctrl Pts',(55.4373334866782,31.4125307799145,5.76543464068109));
#61081=CARTESIAN_POINT('Ctrl Pts',(55.5172682407257,31.3966671521891,5.76121542880322));
#61082=CARTESIAN_POINT('Ctrl Pts',(55.5962437602841,31.3768558282576,5.75699621692535));
#61083=CARTESIAN_POINT('Ctrl Pts',(55.6751935019768,31.3570509708066,5.75277838221191));
#61084=CARTESIAN_POINT('Ctrl Pts',(55.7531841807739,31.3333010890549,5.74856054749848));
#61085=CARTESIAN_POINT('Ctrl Pts',(55.8297993097425,31.3057283785283,5.74434271278505));
#61086=CARTESIAN_POINT('Ctrl Pts',(55.9064128512869,31.2781562392935,5.74012496546289));
#61087=CARTESIAN_POINT('Ctrl Pts',(55.9816504630053,31.2467615871665,5.73590721814072));
#61088=CARTESIAN_POINT('Ctrl Pts',(56.055113332537,31.211715647524,5.73168947081855));
#61089=CARTESIAN_POINT('Ctrl Pts',(56.1286941265191,31.1766134512557,5.72746495306204));
#61090=CARTESIAN_POINT('Ctrl Pts',(56.2004940578778,31.1378484432521,5.72324043530553));
#61091=CARTESIAN_POINT('Ctrl Pts',(56.2701365348185,31.0956391466374,5.71901591754902));
#61092=CARTESIAN_POINT('Ctrl Pts',(56.3397680171007,31.0534365137261,5.71479206672931));
#61093=CARTESIAN_POINT('Ctrl Pts',(56.4072423515412,31.0077909577052,5.7105682159096));
#61094=CARTESIAN_POINT('Ctrl Pts',(56.4722131888498,30.9589636486104,5.70634436508989));
#61095=CARTESIAN_POINT('Ctrl Pts',(56.5373018712743,30.9100477757823,5.70211285298382));
#61096=CARTESIAN_POINT('Ctrl Pts',(56.5998776237771,30.8579389146044,5.69788134087774));
#61097=CARTESIAN_POINT('Ctrl Pts',(56.6596277954745,30.8029381105541,5.69364982877167));
#61098=CARTESIAN_POINT('Ctrl Pts',(56.7191898600446,30.7481104615418,5.68943163842792));
#61099=CARTESIAN_POINT('Ctrl Pts',(56.7759438507384,30.6904094356497,5.68521344808418));
#61100=CARTESIAN_POINT('Ctrl Pts',(56.8296198357287,30.6301660978895,5.68099525774043));
#61101=CARTESIAN_POINT('Ctrl Pts',(56.8834703391349,30.5697268890729,5.67676335266193));
#61102=CARTESIAN_POINT('Ctrl Pts',(56.9344231637771,30.5065038715945,5.67253144758343));
#61103=CARTESIAN_POINT('Ctrl Pts',(56.9821774481714,30.4408063068853,5.66829954250492));
#61104=CARTESIAN_POINT('Ctrl Pts',(57.0298635899893,30.3752024887663,5.66407367610795));
#61105=CARTESIAN_POINT('Ctrl Pts',(57.0743599854588,30.3071315092119,5.65984780971098));
#61106=CARTESIAN_POINT('Ctrl Pts',(57.1154045371144,30.236937304133,5.65562194331401));
#61107=CARTESIAN_POINT('Ctrl Pts',(57.1564121491291,30.1668062730595,5.65139988014988));
#61108=CARTESIAN_POINT('Ctrl Pts',(57.1939738470693,30.0945562067714,5.64717781698576));
#61109=CARTESIAN_POINT('Ctrl Pts',(57.2278702471078,30.0205608321172,5.64295575382163));
#61110=CARTESIAN_POINT('Ctrl Pts',(57.2617366757566,29.9466308845941,5.63873742382978));
#61111=CARTESIAN_POINT('Ctrl Pts',(57.2919440611223,29.870959120572,5.63451909383792));
#61112=CARTESIAN_POINT('Ctrl Pts',(57.3183193406169,29.793943124488,5.63030076384607));
#61113=CARTESIAN_POINT('Ctrl Pts',(57.3446860203039,29.7169522399008,5.62608380926432));
#61114=CARTESIAN_POINT('Ctrl Pts',(57.3672229250302,29.6386184329849,5.62186685468258));
#61115=CARTESIAN_POINT('Ctrl Pts',(57.3858058396285,29.5593574399207,5.61764990010084));
#61116=CARTESIAN_POINT('Ctrl Pts',(57.4043883820968,29.4800980340881,5.61343302996522));
#61117=CARTESIAN_POINT('Ctrl Pts',(57.419016986936,29.3999119317448,5.6092161598296));
#61118=CARTESIAN_POINT('Ctrl Pts',(57.4296181882844,29.319226736283,5.60499928969398));
#61119=CARTESIAN_POINT('Ctrl Pts',(57.4402412657466,29.2383750428492,5.60077371783407));
#61120=CARTESIAN_POINT('Ctrl Pts',(57.4468202434313,29.1570226586364,5.59654814597415));
#61121=CARTESIAN_POINT('Ctrl Pts',(57.44933340943,29.0756048903831,5.59232257411424));
#61122=CARTESIAN_POINT('Ctrl Pts',(57.4518450397081,28.9942368740935,5.58809958437494));
#61123=CARTESIAN_POINT('Ctrl Pts',(57.4502958591789,28.9128040196171,5.58387659463564));
#61124=CARTESIAN_POINT('Ctrl Pts',(57.44471643472,28.8317388820619,5.57965360489633));
#61125=CARTESIAN_POINT('Ctrl Pts',(57.4391268663778,28.7505263609714,5.57542293739102));
#61126=CARTESIAN_POINT('Ctrl Pts',(57.4294924658969,28.6696833556457,5.57119226988571));
#61127=CARTESIAN_POINT('Ctrl Pts',(57.4158955933696,28.5896358544689,5.5669616023804));
#61128=CARTESIAN_POINT('Ctrl Pts',(57.4023231758288,28.5097323246766,5.56273854404527));
#61129=CARTESIAN_POINT('Ctrl Pts',(57.3848027010076,28.4306218705929,5.55851548571013));
#61130=CARTESIAN_POINT('Ctrl Pts',(57.3634655259986,28.3527126160536,5.55429242737499));
#61131=CARTESIAN_POINT('Ctrl Pts',(57.3420757069462,28.2746111402772,5.5500589497193));
#61132=CARTESIAN_POINT('Ctrl Pts',(57.3167706850182,28.1974260423424,5.5458254720636));
#61133=CARTESIAN_POINT('Ctrl Pts',(57.2876462846144,28.121578275263,5.54159199440791));
#61134=CARTESIAN_POINT('Ctrl Pts',(57.2585634435399,28.0458387398479,5.53736455775184));
#61135=CARTESIAN_POINT('Ctrl Pts',(57.2256722137725,27.9714331749786,5.53313712109577));
#61136=CARTESIAN_POINT('Ctrl Pts',(57.1891186039552,27.8987688762948,5.5289096844397));
#61137=CARTESIAN_POINT('Ctrl Pts',(57.15260717494,27.8261884281094,5.52468712600687));
#61138=CARTESIAN_POINT('Ctrl Pts',(57.1124419730094,27.7553456652756,5.52046456757404));
#61139=CARTESIAN_POINT('Ctrl Pts',(57.0688170908201,27.6866279678892,5.51624200914121));
#61140=CARTESIAN_POINT('Ctrl Pts',(57.0252198507741,27.6179538122696,5.51202212625866));
#61141=CARTESIAN_POINT('Ctrl Pts',(56.9781675304111,27.5514024400632,5.50780224337611));
#61142=CARTESIAN_POINT('Ctrl Pts',(56.9278995891057,27.4873356537797,5.50358236049356));
#61143=CARTESIAN_POINT('Ctrl Pts',(56.8776481454277,27.4232898938192,5.49936386255047));
#61144=CARTESIAN_POINT('Ctrl Pts',(56.8241834631045,27.3617274654113,5.49514536460738));
#61145=CARTESIAN_POINT('Ctrl Pts',(56.7677868187332,27.3029790768782,5.49092686666429));
#61146=CARTESIAN_POINT('Ctrl Pts',(56.7113914580959,27.2442320256109,5.48670846474516));
#61147=CARTESIAN_POINT('Ctrl Pts',(56.652064590513,27.188299221033,5.48249006282603));
#61148=CARTESIAN_POINT('Ctrl Pts',(56.5901250769412,27.135475264395,5.47827166090691));
#61149=CARTESIAN_POINT('Ctrl Pts',(56.5281106291953,27.0825874015471,5.47404815558213));
#61150=CARTESIAN_POINT('Ctrl Pts',(56.4634775713136,27.0328162076375,5.46982465025735));
#61151=CARTESIAN_POINT('Ctrl Pts',(56.3965784963801,26.986416439914,5.46560114493257));
#61152=CARTESIAN_POINT('Ctrl Pts',(56.3296640223232,26.9400059916878,5.46137666742276));
#61153=CARTESIAN_POINT('Ctrl Pts',(56.2604828922113,26.8969687536104,5.45715218991294));
#61154=CARTESIAN_POINT('Ctrl Pts',(56.1894147494465,26.8575148066325,5.45292771240313));
#61155=CARTESIAN_POINT('Ctrl Pts',(56.1182180905243,26.8179895130642,5.44869559555457));
#61156=CARTESIAN_POINT('Ctrl Pts',(56.0451280173098,26.7820606658857,5.444463478706));
#61157=CARTESIAN_POINT('Ctrl Pts',(55.9705468772094,26.7498913339265,5.44023136185744));
#61158=CARTESIAN_POINT('Ctrl Pts',(55.8962863854371,26.7178603082803,5.43601744024147));
#61159=CARTESIAN_POINT('Ctrl Pts',(55.8205480775728,26.6895566078653,5.4318035186255));
#61160=CARTESIAN_POINT('Ctrl Pts',(55.7437429055251,26.6650917061946,5.42758959700954));
#61161=CARTESIAN_POINT('Ctrl Pts',(55.6665809343043,26.6405131525855,5.42335609957976));
#61162=CARTESIAN_POINT('Ctrl Pts',(55.5880563758273,26.6197181557584,5.41912260214997));
#61163=CARTESIAN_POINT('Ctrl Pts',(55.5085745716469,26.6028554163184,5.41488910472019));
#61164=CARTESIAN_POINT('Ctrl Pts',(55.4292058827146,26.5860166752384,5.41066163223054));
#61165=CARTESIAN_POINT('Ctrl Pts',(55.3488831043022,26.5730991721212,5.4064341597409));
#61166=CARTESIAN_POINT('Ctrl Pts',(55.2680274277603,26.5642020716061,5.40220668725125));
#61167=CARTESIAN_POINT('Ctrl Pts',(55.1872645983554,26.5553151876935,5.39798406919772));
#61168=CARTESIAN_POINT('Ctrl Pts',(55.1059705462059,26.5504395813525,5.39376145114421));
#61169=CARTESIAN_POINT('Ctrl Pts',(55.0245759219857,26.5496232383451,5.38953883309069));
#61170=CARTESIAN_POINT('Ctrl Pts',(54.9432325944776,26.5488074098153,5.38531887622548));
#61171=CARTESIAN_POINT('Ctrl Pts',(54.8617892837758,26.5520457708118,5.38109891936026));
#61172=CARTESIAN_POINT('Ctrl Pts',(54.7806798685637,26.5593343264702,5.37687896249505));
#61173=CARTESIAN_POINT('Ctrl Pts',(54.6995968008861,26.5666205145185,5.37266037643814));
#61174=CARTESIAN_POINT('Ctrl Pts',(54.6188478753948,26.577954242836,5.36844179038123));
#61175=CARTESIAN_POINT('Ctrl Pts',(54.5388636393897,26.5932795120906,5.36422320432431));
#61176=CARTESIAN_POINT('Ctrl Pts',(54.4588809601898,26.6086044830556,5.36000470037754));
#61177=CARTESIAN_POINT('Ctrl Pts',(54.3796633966782,26.6279207519469,5.35578619643076));
#61178=CARTESIAN_POINT('Ctrl Pts',(54.3016316561382,26.6511211384382,5.35156769248399));
#61179=CARTESIAN_POINT('Ctrl Pts',(54.2235091569189,26.6743485092878,5.34734428199733));
#61180=CARTESIAN_POINT('Ctrl Pts',(54.146575683951,26.7014688949003,5.34312087151067));
#61181=CARTESIAN_POINT('Ctrl Pts',(54.0712368133841,26.7323251570855,5.33889746102401));
#61182=CARTESIAN_POINT('Ctrl Pts',(53.9958765090544,26.7631901978176,5.33467284898524));
#61183=CARTESIAN_POINT('Ctrl Pts',(53.9221121290926,26.7977930283744,5.33044823694648));
#61184=CARTESIAN_POINT('Ctrl Pts',(53.8503265516765,26.8359294807655,5.32622362490771));
#61185=CARTESIAN_POINT('Ctrl Pts',(53.7784108564861,26.8741350588847,5.32199135538208));
#61186=CARTESIAN_POINT('Ctrl Pts',(53.7084815316927,26.9158868203423,5.31775908585645));
#61187=CARTESIAN_POINT('Ctrl Pts',(53.6408943715873,26.9609359645129,5.31352681633082));
#61188=CARTESIAN_POINT('Ctrl Pts',(53.5736093482096,27.005783724264,5.30931346643524));
#61189=CARTESIAN_POINT('Ctrl Pts',(53.5086458998363,27.0538991039601,5.30510011653967));
#61190=CARTESIAN_POINT('Ctrl Pts',(53.4463210542274,27.1049981573985,5.30088676664409));
#61191=CARTESIAN_POINT('Ctrl Pts',(53.3846040832502,27.1555988250329,5.29671451092999));
#61192=CARTESIAN_POINT('Ctrl Pts',(53.3252305756237,27.2093254374529,5.29254225521589));
#61193=CARTESIAN_POINT('Ctrl Pts',(53.2685409160821,27.2659297330505,5.2883699995018));
#61194=CARTESIAN_POINT('Ctrl Pts',(53.2119031338706,27.3224822294356,5.28420156186472));
#61195=CARTESIAN_POINT('Ctrl Pts',(53.1579446829156,27.3819068699599,5.28003312422765));
#61196=CARTESIAN_POINT('Ctrl Pts',(53.1069740353159,27.4439142224698,5.27586468659057));
#61197=CARTESIAN_POINT('Ctrl Pts',(53.0560883838579,27.5058181745725,5.27170320003482));
#61198=CARTESIAN_POINT('Ctrl Pts',(53.0081809220524,27.5702958977824,5.26754171347906));
#61199=CARTESIAN_POINT('Ctrl Pts',(52.9635221819285,27.6370222501806,5.2633802269233));
#61200=CARTESIAN_POINT('Ctrl Pts',(52.9188903880555,27.7037083411422,5.25922125133092));
#61201=CARTESIAN_POINT('Ctrl Pts',(52.877503692765,27.7726399724987,5.25506227573853));
#61202=CARTESIAN_POINT('Ctrl Pts',(52.8395909509523,27.843460769886,5.25090330014614));
#61203=CARTESIAN_POINT('Ctrl Pts',(52.8016887096749,27.9142619523298,5.24674547644802));
#61204=CARTESIAN_POINT('Ctrl Pts',(52.7672587371688,27.9869508397116,5.24258765274991));
#61205=CARTESIAN_POINT('Ctrl Pts',(52.7364844969214,28.0611454759534,5.23842982905179));
#61206=CARTESIAN_POINT('Ctrl Pts',(52.7055816869476,28.1356500852116,5.23425463464848));
#61207=CARTESIAN_POINT('Ctrl Pts',(52.6783654327688,28.2116726133079,5.23007944024517));
#61208=CARTESIAN_POINT('Ctrl Pts',(52.6549724545473,28.2888065937679,5.22590424584186));
#61209=CARTESIAN_POINT('Ctrl Pts',(52.6316551638009,28.3656910089022,5.22174256018975));
#61210=CARTESIAN_POINT('Ctrl Pts',(52.6121365308147,28.4436792188454,5.21758087453763));
#61211=CARTESIAN_POINT('Ctrl Pts',(52.5965011928653,28.5223560592845,5.21341918888552));
#61212=CARTESIAN_POINT('Ctrl Pts',(52.5807897269088,28.6014159749789,5.2092372401066));
#61213=CARTESIAN_POINT('Ctrl Pts',(52.5689995442004,28.6811707622526,5.2050552913277));
#61214=CARTESIAN_POINT('Ctrl Pts',(52.5611638549431,28.761193577214,5.20087334254879));
#61215=CARTESIAN_POINT('Ctrl Pts',(52.5533281656857,28.8412163921755,5.19669139376987));
#61216=CARTESIAN_POINT('Ctrl Pts',(52.5494469351108,28.9215067478683,5.19250944499096));
#61217=CARTESIAN_POINT('Ctrl Pts',(52.5495005484666,29.0016395226469,5.18832749621205));
#61218=CARTESIAN_POINT('Origin',(55.,29.,3.45145488139523));
#61219=CARTESIAN_POINT('',(53.1796208058588,29.8156268460748,23.7995000000001));
#61220=CARTESIAN_POINT('Ctrl Pts',(53.0466869607994,29.4044696940301,23.0258937941419));
#61221=CARTESIAN_POINT('Ctrl Pts',(53.0269937965999,29.3093651287642,23.0326584916325));
#61222=CARTESIAN_POINT('Ctrl Pts',(53.0142625475846,29.21290049674,23.0393919029704));
#61223=CARTESIAN_POINT('Ctrl Pts',(53.0077245142915,29.1005080488077,23.0468431679078));
#61224=CARTESIAN_POINT('Ctrl Pts',(53.0070096342023,29.08516404734,23.047851829735));
#61225=CARTESIAN_POINT('Ctrl Pts',(53.0062705156584,29.0640582609184,23.0492260649345));
#61226=CARTESIAN_POINT('Ctrl Pts',(53.0060939086745,29.0583028169952,23.0495994647139));
#61227=CARTESIAN_POINT('Ctrl Pts',(53.0058343146134,29.0484516465045,23.0502361882818));
#61228=CARTESIAN_POINT('Ctrl Pts',(53.0057390190016,29.0443563211459,23.0505001779298));
#61229=CARTESIAN_POINT('Ctrl Pts',(53.0055672213574,29.0358461944791,23.0510472377948));
#61230=CARTESIAN_POINT('Ctrl Pts',(53.0054927613474,29.0314314097092,23.0513301832163));
#61231=CARTESIAN_POINT('Ctrl Pts',(53.0053480779659,29.0207497161521,23.0520127872558));
#61232=CARTESIAN_POINT('Ctrl Pts',(53.0052927287307,29.0144825850596,23.0524116274026));
#61233=CARTESIAN_POINT('Ctrl Pts',(53.0052021000396,28.992477019324,23.0538065749029));
#61234=CARTESIAN_POINT('Ctrl Pts',(53.0053235413239,28.9767380484583,23.0547944262847));
#61235=CARTESIAN_POINT('Ctrl Pts',(53.0072294407947,28.8792708253711,23.0608599701355));
#61236=CARTESIAN_POINT('Ctrl Pts',(53.0138504254682,28.7977057763332,23.0657111526208));
#61237=CARTESIAN_POINT('Ctrl Pts',(53.0284238550768,28.6961073179405,23.0717176928971));
#61238=CARTESIAN_POINT('Ctrl Pts',(53.0317117769336,28.6754930727361,23.0729344098968));
#61239=CARTESIAN_POINT('Ctrl Pts',(53.0634162678052,28.4949794853208,23.0835974444499));
#61240=CARTESIAN_POINT('Ctrl Pts',(53.110933483601,28.3390733782184,23.0929288342571));
#61241=CARTESIAN_POINT('Ctrl Pts',(53.1853969964351,28.171332104408,23.104242425343));
#61242=CARTESIAN_POINT('Ctrl Pts',(53.1942814473479,28.1521468299178,23.105555364071));
#61243=CARTESIAN_POINT('Ctrl Pts',(53.2084123863968,28.1228621667007,23.1075906217099));
#61244=CARTESIAN_POINT('Ctrl Pts',(53.2134433262879,28.1126600432109,23.1083055677231));
#61245=CARTESIAN_POINT('Ctrl Pts',(53.2217855759446,28.0961015639035,23.1094758719722));
#61246=CARTESIAN_POINT('Ctrl Pts',(53.2250444165549,28.0897189470692,23.1099294012262));
#61247=CARTESIAN_POINT('Ctrl Pts',(53.2319649715542,28.0763431305161,23.1108850256121));
#61248=CARTESIAN_POINT('Ctrl Pts',(53.2356339379979,28.0693538423847,23.111387368638));
#61249=CARTESIAN_POINT('Ctrl Pts',(53.2445224864398,28.0526628758661,23.1125943046141));
#61250=CARTESIAN_POINT('Ctrl Pts',(53.2497810989011,28.0429823838635,23.1133002642427));
#61251=CARTESIAN_POINT('Ctrl Pts',(53.2681715927985,28.0097862072837,23.1157420511611));
#61252=CARTESIAN_POINT('Ctrl Pts',(53.2816989131776,27.98649408225,23.117491853158));
#61253=CARTESIAN_POINT('Ctrl Pts',(53.3155064269025,27.9309055810656,23.1217591266877));
#61254=CARTESIAN_POINT('Ctrl Pts',(53.3362485980348,27.8989039857857,23.1242924895472));
#61255=CARTESIAN_POINT('Ctrl Pts',(53.4216929830226,27.775009081462,23.1344084990309));
#61256=CARTESIAN_POINT('Ctrl Pts',(53.4931887835824,27.6880660864639,23.1422137902668));
#61257=CARTESIAN_POINT('Ctrl Pts',(53.6473467165213,27.5299224298756,23.1576074858563));
#61258=CARTESIAN_POINT('Ctrl Pts',(53.7292996110698,27.4585318490359,23.1651655992862));
#61259=CARTESIAN_POINT('Ctrl Pts',(53.8295922485481,27.3846265671882,23.1734194324104));
#61260=CARTESIAN_POINT('Ctrl Pts',(53.8426399155792,27.3752528485534,23.174475171916));
#61261=CARTESIAN_POINT('Ctrl Pts',(53.861127967449,27.3623063885016,23.1759443698658));
#61262=CARTESIAN_POINT('Ctrl Pts',(53.8664743567736,27.3586013614416,23.1763661392876));
#61263=CARTESIAN_POINT('Ctrl Pts',(53.8751523361516,27.3526501773608,23.1770456192352));
#61264=CARTESIAN_POINT('Ctrl Pts',(53.8784727030794,27.3503878552904,23.1773043996749));
#61265=CARTESIAN_POINT('Ctrl Pts',(53.8855193801861,27.3456177332947,23.1778510190905));
#61266=CARTESIAN_POINT('Ctrl Pts',(53.8892473727873,27.3431124545434,23.1781386836943));
#61267=CARTESIAN_POINT('Ctrl Pts',(53.8985088657935,27.3369338691558,23.178849656092));
#61268=CARTESIAN_POINT('Ctrl Pts',(53.9040523658649,27.3332755295128,23.1792719759884));
#61269=CARTESIAN_POINT('Ctrl Pts',(53.9248696230127,27.3196862975788,23.1808462374057));
#61270=CARTESIAN_POINT('Ctrl Pts',(53.9402614664818,27.3099367580645,23.1819868582589));
#61271=CARTESIAN_POINT('Ctrl Pts',(53.9795955272188,27.2857703779029,23.1848488145544));
#61272=CARTESIAN_POINT('Ctrl Pts',(54.0037116932348,27.2716429037138,23.1865548134304));
#61273=CARTESIAN_POINT('Ctrl Pts',(54.1153955260518,27.209332257933,23.1942723266549));
#61274=CARTESIAN_POINT('Ctrl Pts',(54.2062160544311,27.1672626624804,23.2000480025739));
#61275=CARTESIAN_POINT('Ctrl Pts',(54.4232766365216,27.0858936953332,23.2135099583196));
#61276=CARTESIAN_POINT('Ctrl Pts',(54.5510086944361,27.0519717573984,23.221200619581));
#61277=CARTESIAN_POINT('Ctrl Pts',(54.7051792221558,27.027007086802,23.2308154270356));
#61278=CARTESIAN_POINT('Ctrl Pts',(54.7292812957294,27.023555811542,23.2323269565471));
#61279=CARTESIAN_POINT('Ctrl Pts',(54.7631637726224,27.019335417538,23.2344661364921));
#61280=CARTESIAN_POINT('Ctrl Pts',(54.7728964799116,27.018195879373,23.2350822549687));
#61281=CARTESIAN_POINT('Ctrl Pts',(54.7898217301219,27.0163405289065,23.2361567060718));
#61282=CARTESIAN_POINT('Ctrl Pts',(54.797010557825,27.0155920060299,23.2366140117171));
#61283=CARTESIAN_POINT('Ctrl Pts',(54.8120235351367,27.0141112409155,23.2375710778735));
#61284=CARTESIAN_POINT('Ctrl Pts',(54.8198482478452,27.0133861326082,23.238071052261));
#61285=CARTESIAN_POINT('Ctrl Pts',(54.8384151345723,27.0117761520964,23.2392602479254));
#61286=CARTESIAN_POINT('Ctrl Pts',(54.8491605116404,27.0109320827679,23.239950726404));
#61287=CARTESIAN_POINT('Ctrl Pts',(54.885285171777,27.0083888286327,23.2422798574794));
#61288=CARTESIAN_POINT('Ctrl Pts',(54.910689137617,27.0070880548499,23.243930776762));
#61289=CARTESIAN_POINT('Ctrl Pts',(54.9714639187638,27.0051404984673,23.2479131143175));
#61290=CARTESIAN_POINT('Ctrl Pts',(55.0068397008295,27.0049481950451,23.2502577455333));
#61291=CARTESIAN_POINT('Ctrl Pts',(55.1452925243451,27.0078779066466,23.2595387027066));
#61292=CARTESIAN_POINT('Ctrl Pts',(55.248049560848,27.018049589813,23.266664843371));
#61293=CARTESIAN_POINT('Ctrl Pts',(55.4705398563118,27.057650285062,23.2824051829382));
#61294=CARTESIAN_POINT('Ctrl Pts',(55.5892924061433,27.0903220407767,23.2910124544846));
#61295=CARTESIAN_POINT('Ctrl Pts',(55.7190341513746,27.1392835284934,23.3001951079177));
#61296=CARTESIAN_POINT('Ctrl Pts',(55.7337120060112,27.1450222030181,23.301230345357));
#61297=CARTESIAN_POINT('Ctrl Pts',(55.7543099648585,27.1533582416038,23.3026765027001));
#61298=CARTESIAN_POINT('Ctrl Pts',(55.760287375528,27.1558111766054,23.3030953751033));
#61299=CARTESIAN_POINT('Ctrl Pts',(55.7703298121838,27.1599893908685,23.303797640786));
#61300=CARTESIAN_POINT('Ctrl Pts',(55.7744011863436,27.1616991907608,23.3040819427536));
#61301=CARTESIAN_POINT('Ctrl Pts',(55.7827168361507,27.1652239309213,23.3046617376676));
#61302=CARTESIAN_POINT('Ctrl Pts',(55.7869605300156,27.1670401001385,23.3049571553129));
#61303=CARTESIAN_POINT('Ctrl Pts',(55.7977757553531,27.1717131646593,23.305708940068));
#61304=CARTESIAN_POINT('Ctrl Pts',(55.8043383341192,27.1745907976322,23.3061640769284));
#61305=CARTESIAN_POINT('Ctrl Pts',(55.8310940166077,27.1864952348645,23.3080159818504));
#61306=CARTESIAN_POINT('Ctrl Pts',(55.8511526922929,27.1958226286283,23.30939572661));
#61307=CARTESIAN_POINT('Ctrl Pts',(56.0261601913642,27.2807706915851,23.3213929464275));
#61308=CARTESIAN_POINT('Ctrl Pts',(56.1708713746678,27.3758599743514,23.3310817786555));
#61309=CARTESIAN_POINT('Ctrl Pts',(56.372195455831,27.5492087654979,23.3466972653289));
#61310=CARTESIAN_POINT('Ctrl Pts',(56.4384711079166,27.6148959523822,23.35227580554));
#61311=CARTESIAN_POINT('Ctrl Pts',(56.5100495467407,27.6965374580077,23.3590179190276));
#61312=CARTESIAN_POINT('Ctrl Pts',(56.5200570380525,27.7082218408238,23.3599784346568));
#61313=CARTESIAN_POINT('Ctrl Pts',(56.5361859839426,27.7275003759686,23.3615567948436));
#61314=CARTESIAN_POINT('Ctrl Pts',(56.5423887730352,27.7350258746334,23.3621713492577));
#61315=CARTESIAN_POINT('Ctrl Pts',(56.5534026539198,27.7485898505873,23.3632763954362));
#61316=CARTESIAN_POINT('Ctrl Pts',(56.5582343730027,27.7546113846124,23.3637660508649));
#61317=CARTESIAN_POINT('Ctrl Pts',(56.568419601323,27.7674567997589,23.3648087602921));
#61318=CARTESIAN_POINT('Ctrl Pts',(56.5737637907646,27.7742878342497,23.3653621682558));
#61319=CARTESIAN_POINT('Ctrl Pts',(56.5879892300069,27.7927174445258,23.3668524385846));
#61320=CARTESIAN_POINT('Ctrl Pts',(56.5967877644377,27.8043789145247,23.3677924956758));
#61321=CARTESIAN_POINT('Ctrl Pts',(56.6405830399055,27.8637703861967,23.3725664991025));
#61322=CARTESIAN_POINT('Ctrl Pts',(56.6735680910811,27.9129401615652,23.3764760805458));
#61323=CARTESIAN_POINT('Ctrl Pts',(56.7684776016419,28.0689997145327,23.3887640361049));
#61324=CARTESIAN_POINT('Ctrl Pts',(56.8226980836196,28.1802196279707,23.397374778849));
#61325=CARTESIAN_POINT('Ctrl Pts',(56.8841831293861,28.3431504683717,23.4095042681128));
#61326=CARTESIAN_POINT('Ctrl Pts',(56.9002673620794,28.3912457921987,23.4130254420823));
#61327=CARTESIAN_POINT('Ctrl Pts',(56.9298778868938,28.4924593881586,23.4202565067685));
#61328=CARTESIAN_POINT('Ctrl Pts',(56.9430843746261,28.5456318536107,23.4239560146763));
#61329=CARTESIAN_POINT('Ctrl Pts',(56.9558963189699,28.6081093374627,23.4281392119864));
#61330=CARTESIAN_POINT('Ctrl Pts',(56.95764608585,28.6169458109699,23.4287270780151));
#61331=CARTESIAN_POINT('Ctrl Pts',(56.96037778546,28.6312489427348,23.4296721905237));
#61332=CARTESIAN_POINT('Ctrl Pts',(56.9613968287197,28.63670826318,23.4300314166702));
#61333=CARTESIAN_POINT('Ctrl Pts',(56.9631650278105,28.6464053806947,23.4306667265646));
#61334=CARTESIAN_POINT('Ctrl Pts',(56.9639232897444,28.6506414525974,23.4309433170164));
#61335=CARTESIAN_POINT('Ctrl Pts',(56.9655277203487,28.6597750112247,23.4315376344174));
#61336=CARTESIAN_POINT('Ctrl Pts',(56.9663692987154,28.6646732268088,23.4318551013414));
#61337=CARTESIAN_POINT('Ctrl Pts',(56.9686708131002,28.6783753272465,23.4327397866297));
#61338=CARTESIAN_POINT('Ctrl Pts',(56.9700900114112,28.6871860704638,23.4333047559333));
#61339=CARTESIAN_POINT('Ctrl Pts',(56.9781906316498,28.739719938627,23.4366517527509));
#61340=CARTESIAN_POINT('Ctrl Pts',(56.9834759991016,28.7836495542177,23.4393615630364));
#61341=CARTESIAN_POINT('Ctrl Pts',(56.9963859202443,28.9325708719677,23.4483575379999));
#61342=CARTESIAN_POINT('Ctrl Pts',(56.9971640112668,29.0379823119999,23.4544142480253));
#61343=CARTESIAN_POINT('Ctrl Pts',(56.9806647011903,29.2675935326576,23.4677755473257));
#61344=CARTESIAN_POINT('Ctrl Pts',(56.9600220017781,29.3910849872229,23.4750825923943));
#61345=CARTESIAN_POINT('Ctrl Pts',(56.9217309019719,29.5353211833679,23.484266788313));
#61346=CARTESIAN_POINT('Ctrl Pts',(56.915065151186,29.5586983227218,23.4857754975631));
#61347=CARTESIAN_POINT('Ctrl Pts',(56.9051284679641,29.5912767747246,23.4879089592227));
#61348=CARTESIAN_POINT('Ctrl Pts',(56.9022144792804,29.6005853587795,23.4885221173801));
#61349=CARTESIAN_POINT('Ctrl Pts',(56.8970361774662,29.6167113612844,23.4895907140938));
#61350=CARTESIAN_POINT('Ctrl Pts',(56.8948030734968,29.6235386693897,23.490045124005));
#61351=CARTESIAN_POINT('Ctrl Pts',(56.8900687174059,29.6377527939192,23.4909954224819));
#61352=CARTESIAN_POINT('Ctrl Pts',(56.8875609284246,29.6451372887339,23.4914915198569));
#61353=CARTESIAN_POINT('Ctrl Pts',(56.8815177860186,29.6625951656407,23.4926701442732));
#61354=CARTESIAN_POINT('Ctrl Pts',(56.8779447685756,29.6726551653545,23.4933539081129));
#61355=CARTESIAN_POINT('Ctrl Pts',(56.8657054623858,29.7062577726948,23.4956535222178));
#61356=CARTESIAN_POINT('Ctrl Pts',(56.8566761286016,29.7296646984661,23.4972813705041));
#61357=CARTESIAN_POINT('Ctrl Pts',(56.8340726161987,29.785121876564,23.5012023012756));
#61358=CARTESIAN_POINT('Ctrl Pts',(56.8200966915207,29.8169984779811,23.5035082162291));
#61359=CARTESIAN_POINT('Ctrl Pts',(56.7625488991183,29.9394401404017,23.5125711797984));
#61360=CARTESIAN_POINT('Ctrl Pts',(56.7129959541922,30.0270185615008,23.519509994011));
#61361=CARTESIAN_POINT('Ctrl Pts',(56.5863504229899,30.2159991613256,23.5353575152376));
#61362=CARTESIAN_POINT('Ctrl Pts',(56.5057156092179,30.3145294081862,23.5442725769919));
#61363=CARTESIAN_POINT('Ctrl Pts',(56.4053126561713,30.4157560492814,23.5537134968081));
#61364=CARTESIAN_POINT('Ctrl Pts',(56.3942449034619,30.4266569445521,23.5547339758985));
#61365=CARTESIAN_POINT('Ctrl Pts',(56.3784386814168,30.4418652238573,23.5561616570567));
#61366=CARTESIAN_POINT('Ctrl Pts',(56.3738054175832,30.4462804705647,23.5565766220354));
#61367=CARTESIAN_POINT('Ctrl Pts',(56.3659606293862,30.4536844105377,23.5572731705885));
#61368=CARTESIAN_POINT('Ctrl Pts',(56.362760378524,30.4566849208744,23.5575556453886));
#61369=CARTESIAN_POINT('Ctrl Pts',(56.3561756278052,30.4628179981053,23.5581333839986));
#61370=CARTESIAN_POINT('Ctrl Pts',(56.3527901458667,30.4659494027158,23.558428564128));
#61371=CARTESIAN_POINT('Ctrl Pts',(56.3441132951714,30.4739194081151,23.5591804599885));
#61372=CARTESIAN_POINT('Ctrl Pts',(56.3388065881791,30.4787413212083,23.5596359397828));
#61373=CARTESIAN_POINT('Ctrl Pts',(56.31695192135,30.4983853711532,23.5614944693113));
#61374=CARTESIAN_POINT('Ctrl Pts',(56.3001821923403,30.5129598299847,23.5628803043307));
#61375=CARTESIAN_POINT('Ctrl Pts',(56.1521480754288,30.6373356444658,23.5748039478997));
#61376=CARTESIAN_POINT('Ctrl Pts',(56.0074867602964,30.7301155604524,23.5844238475882));
#61377=CARTESIAN_POINT('Ctrl Pts',(55.7655181453883,30.8445373607581,23.6001335628644));
#61378=CARTESIAN_POINT('Ctrl Pts',(55.6754310293716,30.8793949850743,23.605899824467));
#61379=CARTESIAN_POINT('Ctrl Pts',(55.5683294707553,30.9121376584505,23.612854367207));
#61380=CARTESIAN_POINT('Ctrl Pts',(55.5534236850307,30.9165048958821,23.6138241994013));
#61381=CARTESIAN_POINT('Ctrl Pts',(55.5290198806953,30.9233465175018,23.6154158610411));
#61382=CARTESIAN_POINT('Ctrl Pts',(55.5195517425197,30.9259257103851,23.6160343276561));
#61383=CARTESIAN_POINT('Ctrl Pts',(55.5025751192138,30.9304159749629,23.6171450926423));
#61384=CARTESIAN_POINT('Ctrl Pts',(55.4950737554998,30.9323533736677,23.6176365387527));
#61385=CARTESIAN_POINT('Ctrl Pts',(55.4791429887171,30.9363690069521,23.6186816677031));
#61386=CARTESIAN_POINT('Ctrl Pts',(55.4707109442223,30.9384360030261,23.6192356970079));
#61387=CARTESIAN_POINT('Ctrl Pts',(55.4480919170739,30.9438244509622,23.6207242885064));
#61388=CARTESIAN_POINT('Ctrl Pts',(55.4338817994746,30.9470455639079,23.6216620043055));
#61389=CARTESIAN_POINT('Ctrl Pts',(55.3626139068295,30.9623814701046,23.6263784521179));
#61390=CARTESIAN_POINT('Ctrl Pts',(55.3050844080902,30.9721440726963,23.6302301539382));
#61391=CARTESIAN_POINT('Ctrl Pts',(55.1336318920188,30.993557701073,23.6418458428476));
#61392=CARTESIAN_POINT('Ctrl Pts',(55.0190501218361,30.9979393475764,23.6497985991136));
#61393=CARTESIAN_POINT('Ctrl Pts',(54.8001909402524,30.9874755624655,23.6650546666023));
#61394=CARTESIAN_POINT('Ctrl Pts',(54.6961882118609,30.9742556737258,23.6723277967546));
#61395=CARTESIAN_POINT('Ctrl Pts',(54.5779959171746,30.9496659336828,23.6803221828443));
#61396=CARTESIAN_POINT('Ctrl Pts',(54.5623359725929,30.9462104039463,23.6813756071969));
#61397=CARTESIAN_POINT('Ctrl Pts',(54.5404432024905,30.9411019139186,23.6828385873551));
#61398=CARTESIAN_POINT('Ctrl Pts',(54.5341746046335,30.9396071236522,23.6832563622914));
#61399=CARTESIAN_POINT('Ctrl Pts',(54.5236203829862,30.9370362787557,23.6839577353699));
#61400=CARTESIAN_POINT('Ctrl Pts',(54.519330942291,30.9359763281572,23.6842422203313));
#61401=CARTESIAN_POINT('Ctrl Pts',(54.5106107827195,30.9337907470628,23.6848193751251));
#61402=CARTESIAN_POINT('Ctrl Pts',(54.5061804006559,30.9326641362935,23.6851119901684));
#61403=CARTESIAN_POINT('Ctrl Pts',(54.4949803460138,30.9297750245215,23.6858502565804));
#61404=CARTESIAN_POINT('Ctrl Pts',(54.4882159346453,30.9279921083906,23.6862947823126));
#61405=CARTESIAN_POINT('Ctrl Pts',(54.4621253596635,30.9209683476557,23.6880045728139));
#61406=CARTESIAN_POINT('Ctrl Pts',(54.4428684186382,30.9154720025348,23.6892564236563));
#61407=CARTESIAN_POINT('Ctrl Pts',(54.2912854644196,30.8697274444191,23.6990539728212));
#61408=CARTESIAN_POINT('Ctrl Pts',(54.1633721998504,30.8161004049785,23.7069985486325));
#61409=CARTESIAN_POINT('Ctrl Pts',(54.0258782399295,30.740819710466,23.7161584189659));
#61410=CARTESIAN_POINT('Ctrl Pts',(54.0098540500527,30.731755599347,23.7172357677195));
#61411=CARTESIAN_POINT('Ctrl Pts',(53.9038475038053,30.6698404423495,23.7244399152103));
#61412=CARTESIAN_POINT('Ctrl Pts',(53.8180171704275,30.6102266877487,23.7306586870503));
#61413=CARTESIAN_POINT('Ctrl Pts',(53.7250642332943,30.5342144919913,23.7381142867862));
#61414=CARTESIAN_POINT('Ctrl Pts',(53.7129980410297,30.5241067064651,23.7390969735459));
#61415=CARTESIAN_POINT('Ctrl Pts',(53.6935228361529,30.5073962427245,23.7407083149328));
#61416=CARTESIAN_POINT('Ctrl Pts',(53.6860411059779,30.5008790862246,23.741333555631));
#61417=CARTESIAN_POINT('Ctrl Pts',(53.6727481960419,30.4891243761616,23.742455799945));
#61418=CARTESIAN_POINT('Ctrl Pts',(53.6669185808696,30.4839079102067,23.7429519385613));
#61419=CARTESIAN_POINT('Ctrl Pts',(53.6546291352255,30.4727801836509,23.7440064174553));
#61420=CARTESIAN_POINT('Ctrl Pts',(53.6481772574697,30.4668604234792,23.7445651032287));
#61421=CARTESIAN_POINT('Ctrl Pts',(53.6310172363931,30.4509063047845,23.7460648860278));
#61422=CARTESIAN_POINT('Ctrl Pts',(53.6203806593805,30.4407960884781,23.7470091508639));
#61423=CARTESIAN_POINT('Ctrl Pts',(53.5679022930759,30.3898007086786,23.751742653849));
#61424=CARTESIAN_POINT('Ctrl Pts',(53.5277654489043,30.3472097564735,23.755604899916));
#61425=CARTESIAN_POINT('Ctrl Pts',(53.3631004050786,30.1563181795977,23.7725527284527));
#61426=CARTESIAN_POINT('Ctrl Pts',(53.2587174625726,29.992160893355,23.7863691355466));
#61427=CARTESIAN_POINT('Ctrl Pts',(53.1796208058588,29.8156268460748,23.7995000000001));
#61428=CARTESIAN_POINT('',(55.1572109533382,30.9885452669352,23.7995));
#61429=CARTESIAN_POINT('Origin',(55.,29.,23.7995));
#61430=CARTESIAN_POINT('',(53.0052505146164,29.0014328510003,23.2095451186048));
#61431=CARTESIAN_POINT('Ctrl Pts',(53.0052505146164,29.0014328510003,23.2095451186048));
#61432=CARTESIAN_POINT('Ctrl Pts',(53.0052003937452,28.9316568713932,23.213983964139));
#61433=CARTESIAN_POINT('Ctrl Pts',(53.008815721088,28.8618442511641,23.2184228096733));
#61434=CARTESIAN_POINT('Ctrl Pts',(53.0160814449356,28.7924072993311,23.2228616552075));
#61435=CARTESIAN_POINT('Ctrl Pts',(53.0233464821315,28.7229769096794,23.2273000812459));
#61436=CARTESIAN_POINT('Ctrl Pts',(53.0342611791721,28.6539226036702,23.2317385072843));
#61437=CARTESIAN_POINT('Ctrl Pts',(53.0487586209827,28.5856515436127,23.2361769333228));
#61438=CARTESIAN_POINT('Ctrl Pts',(53.0632595914515,28.5173638664694,23.2406164396682));
#61439=CARTESIAN_POINT('Ctrl Pts',(53.0813449337531,28.4498602909106,23.2450559460137));
#61440=CARTESIAN_POINT('Ctrl Pts',(53.1028970159024,28.3835360268208,23.2494954523591));
#61441=CARTESIAN_POINT('Ctrl Pts',(53.1244760897302,28.3171286986818,23.2539405187116));
#61442=CARTESIAN_POINT('Ctrl Pts',(53.1495304120609,28.2519040931028,23.2583855850641));
#61443=CARTESIAN_POINT('Ctrl Pts',(53.1778933430144,28.1882396332238,23.2628306514166));
#61444=CARTESIAN_POINT('Ctrl Pts',(53.2062775865753,28.1245273342959,23.2672790579018));
#61445=CARTESIAN_POINT('Ctrl Pts',(53.237975161805,28.0623779471762,23.271727464387));
#61446=CARTESIAN_POINT('Ctrl Pts',(53.2727736951244,28.0021438709685,23.2761758708722));
#61447=CARTESIAN_POINT('Ctrl Pts',(53.3076334738165,27.9418037828661,23.280632106547));
#61448=CARTESIAN_POINT('Ctrl Pts',(53.3456048299077,27.8833861368431,23.2850883422217));
#61449=CARTESIAN_POINT('Ctrl Pts',(53.3864329442855,27.8272131825379,23.2895445778965));
#61450=CARTESIAN_POINT('Ctrl Pts',(53.3960350471951,27.814002224937,23.2905926114437));
#61451=CARTESIAN_POINT('Ctrl Pts',(53.4057949933653,27.8009152710909,23.291640644991));
#61452=CARTESIAN_POINT('Ctrl Pts',(53.4157091669753,27.787956222369,23.2926886785382));
#61453=CARTESIAN_POINT('Ctrl Pts',(53.4579393336063,27.7327561816565,23.2971528560961));
#61454=CARTESIAN_POINT('Ctrl Pts',(53.5031392396318,27.6796594619913,23.3016170336539));
#61455=CARTESIAN_POINT('Ctrl Pts',(53.5510719652676,27.6290021470963,23.3060812112118));
#61456=CARTESIAN_POINT('Ctrl Pts',(53.5989330395069,27.5784205564024,23.310538715572));
#61457=CARTESIAN_POINT('Ctrl Pts',(53.6495184920662,27.5302714830558,23.3149962199321));
#61458=CARTESIAN_POINT('Ctrl Pts',(53.7025503019092,27.4848591341317,23.3194537242923));
#61459=CARTESIAN_POINT('Ctrl Pts',(53.7555194471414,27.4395004463438,23.3239059614783));
#61460=CARTESIAN_POINT('Ctrl Pts',(53.8109288390678,27.3968723744137,23.3283581986643));
#61461=CARTESIAN_POINT('Ctrl Pts',(53.8684639171322,27.3572420581023,23.3328104358503));
#61462=CARTESIAN_POINT('Ctrl Pts',(53.925962550079,27.3176368452857,23.3372598528037));
#61463=CARTESIAN_POINT('Ctrl Pts',(53.9855837973,27.2810258960868,23.341709269757));
#61464=CARTESIAN_POINT('Ctrl Pts',(54.0469815372319,27.2476349204224,23.3461586867104));
#61465=CARTESIAN_POINT('Ctrl Pts',(54.1083609907082,27.2142538897917,23.3506067784673));
#61466=CARTESIAN_POINT('Ctrl Pts',(54.1715154586615,27.1840911611187,23.3550548702242));
#61467=CARTESIAN_POINT('Ctrl Pts',(54.2360729823614,27.1573271928468,23.3595029619811));
#61468=CARTESIAN_POINT('Ctrl Pts',(54.300632943392,27.1305622141173,23.3639512216731));
#61469=CARTESIAN_POINT('Ctrl Pts',(54.3665956144681,27.1071964348777,23.368399481365));
#61470=CARTESIAN_POINT('Ctrl Pts',(54.4335693888397,27.0873620506639,23.372847741057));
#61471=CARTESIAN_POINT('Ctrl Pts',(54.5006111469935,27.0675075329506,23.3773005160913));
#61472=CARTESIAN_POINT('Ctrl Pts',(54.5686655890589,27.051191703632,23.3817532911256));
#61473=CARTESIAN_POINT('Ctrl Pts',(54.6373272168936,27.0384964912359,23.3862060661599));
#61474=CARTESIAN_POINT('Ctrl Pts',(54.7060278406712,27.0257940686732,23.39066137012));
#61475=CARTESIAN_POINT('Ctrl Pts',(54.7753358536369,27.0167164203056,23.3951166740801));
#61476=CARTESIAN_POINT('Ctrl Pts',(54.8448395772272,27.0112936854063,23.3995719780401));
#61477=CARTESIAN_POINT('Ctrl Pts',(54.9144593687262,27.0058618947979,23.4040347221457));
#61478=CARTESIAN_POINT('Ctrl Pts',(54.9842750363814,27.0040972136788,23.4084974662512));
#61479=CARTESIAN_POINT('Ctrl Pts',(55.0538746652478,27.0059776623758,23.4129602103568));
#61480=CARTESIAN_POINT('Ctrl Pts',(55.0873082045986,27.0068809725878,23.4151039765391));
#61481=CARTESIAN_POINT('Ctrl Pts',(55.1206919650002,27.0086246434188,23.4172477427214));
#61482=CARTESIAN_POINT('Ctrl Pts',(55.1539809403483,27.0112020131473,23.4193915089037));
#61483=CARTESIAN_POINT('Ctrl Pts',(55.223243451322,27.0165646023299,23.4238519234155));
#61484=CARTESIAN_POINT('Ctrl Pts',(55.2923578402198,27.0255599757434,23.4283123379274));
#61485=CARTESIAN_POINT('Ctrl Pts',(55.3609135802758,27.0381720386149,23.4327727524393));
#61486=CARTESIAN_POINT('Ctrl Pts',(55.429368653755,27.0507655820569,23.4372266173222));
#61487=CARTESIAN_POINT('Ctrl Pts',(55.4972662306628,27.0669651856091,23.4416804822051));
#61488=CARTESIAN_POINT('Ctrl Pts',(55.564200204765,27.0867029265054,23.446134347088));
#61489=CARTESIAN_POINT('Ctrl Pts',(55.6310579929409,27.1064182014104,23.4505831424703));
#61490=CARTESIAN_POINT('Ctrl Pts',(55.6969538910947,27.1296634772005,23.4550319378526));
#61491=CARTESIAN_POINT('Ctrl Pts',(55.7614930396604,27.15632000796,23.459480733235));
#61492=CARTESIAN_POINT('Ctrl Pts',(55.8259930789442,27.1829603854574,23.4639268327467));
#61493=CARTESIAN_POINT('Ctrl Pts',(55.8891375499583,27.213007730801,23.4683729322584));
#61494=CARTESIAN_POINT('Ctrl Pts',(55.950549236786,27.2462942918079,23.4728190317701));
#61495=CARTESIAN_POINT('Ctrl Pts',(56.0119443912701,27.2795718919005,23.4772639343688));
#61496=CARTESIAN_POINT('Ctrl Pts',(56.0716072591108,27.3160867439157,23.4817088369676));
#61497=CARTESIAN_POINT('Ctrl Pts',(56.1291845935455,27.3556248249869,23.4861537395663));
#61498=CARTESIAN_POINT('Ctrl Pts',(56.1867658175742,27.3951655770237,23.4905989424371));
#61499=CARTESIAN_POINT('Ctrl Pts',(56.2422608277492,27.4377296854861,23.4950441453079));
#61500=CARTESIAN_POINT('Ctrl Pts',(56.295346242923,27.4830604252492,23.4994893481787));
#61501=CARTESIAN_POINT('Ctrl Pts',(56.3484881889734,27.5284394379032,23.5039392847643));
#61502=CARTESIAN_POINT('Ctrl Pts',(56.3992150471316,27.5765906445625,23.50838922135));
#61503=CARTESIAN_POINT('Ctrl Pts',(56.447238100391,27.6272183555726,23.5128391579356));
#61504=CARTESIAN_POINT('Ctrl Pts',(56.495289745305,27.6778762089817,23.5172917438956));
#61505=CARTESIAN_POINT('Ctrl Pts',(56.5406340643731,27.7310131305015,23.5217443298557));
#61506=CARTESIAN_POINT('Ctrl Pts',(56.5830224948326,27.7863001428055,23.5261969158157));
#61507=CARTESIAN_POINT('Ctrl Pts',(56.6254837756589,27.841682173469,23.5306571541591));
#61508=CARTESIAN_POINT('Ctrl Pts',(56.6649787517476,27.899221268783,23.5351173925025));
#61509=CARTESIAN_POINT('Ctrl Pts',(56.7013025072247,27.9585599674437,23.5395776308459));
#61510=CARTESIAN_POINT('Ctrl Pts',(56.7189929910849,27.9874592449867,23.541749866987));
#61511=CARTESIAN_POINT('Ctrl Pts',(56.7359319909526,28.0167850081694,23.5439221031281));
#61512=CARTESIAN_POINT('Ctrl Pts',(56.7520999247469,28.0464941446421,23.5460943392691));
#61513=CARTESIAN_POINT('Ctrl Pts',(56.7849370585255,28.1068335115155,23.5505061589654));
#61514=CARTESIAN_POINT('Ctrl Pts',(56.8147250413319,28.1690028022865,23.5549179786618));
#61515=CARTESIAN_POINT('Ctrl Pts',(56.8412533880425,28.2326581442915,23.5593297983581));
#61516=CARTESIAN_POINT('Ctrl Pts',(56.8677416371924,28.2962172713323,23.5637349495949));
#61517=CARTESIAN_POINT('Ctrl Pts',(56.8909798325664,28.3612575373282,23.5681401008316));
#61518=CARTESIAN_POINT('Ctrl Pts',(56.9108030193091,28.4274099338102,23.5725452520684));
#61519=CARTESIAN_POINT('Ctrl Pts',(56.9306036107021,28.4934869268492,23.5769453821179));
#61520=CARTESIAN_POINT('Ctrl Pts',(56.9469967761192,28.5606730584504,23.5813455121674));
#61521=CARTESIAN_POINT('Ctrl Pts',(56.9598661039142,28.6285805373597,23.5857456422169));
#61522=CARTESIAN_POINT('Ctrl Pts',(56.9727276878521,28.6964471543194,23.5901431245773));
#61523=CARTESIAN_POINT('Ctrl Pts',(56.982069544642,28.765033768377,23.5945406069377));
#61524=CARTESIAN_POINT('Ctrl Pts',(56.9878258834181,28.8339403128002,23.5989380892981));
#61525=CARTESIAN_POINT('Ctrl Pts',(56.9935808038825,28.9028298792501,23.6033344881571));
#61526=CARTESIAN_POINT('Ctrl Pts',(56.9957519173905,28.9720387219498,23.6077308870161));
#61527=CARTESIAN_POINT('Ctrl Pts',(56.9943252738296,29.0411614463345,23.612127285875));
#61528=CARTESIAN_POINT('Ctrl Pts',(56.9928984748356,29.1102917016561,23.6165241637227));
#61529=CARTESIAN_POINT('Ctrl Pts',(56.987873153928,29.1793353205475,23.6209210415703));
#61530=CARTESIAN_POINT('Ctrl Pts',(56.9792874447691,29.2478886312022,23.625317919418));
#61531=CARTESIAN_POINT('Ctrl Pts',(56.9706913314874,29.3165250144432,23.629720125382));
#61532=CARTESIAN_POINT('Ctrl Pts',(56.9585262831637,29.3846694070833,23.634122331346));
#61533=CARTESIAN_POINT('Ctrl Pts',(56.9428819981594,29.4519259936409,23.63852453731));
#61534=CARTESIAN_POINT('Ctrl Pts',(56.9272273849109,29.5192269825121,23.6429296495786));
#61535=CARTESIAN_POINT('Ctrl Pts',(56.9080891071294,29.5856385203148,23.6473347618472));
#61536=CARTESIAN_POINT('Ctrl Pts',(56.8856065793176,29.6507806009204,23.6517398741159));
#61537=CARTESIAN_POINT('Ctrl Pts',(56.8630803356331,29.7160493462374,23.6561535518505));
#61538=CARTESIAN_POINT('Ctrl Pts',(56.8371970534577,29.780043246305,23.6605672295851));
#61539=CARTESIAN_POINT('Ctrl Pts',(56.8081437043812,29.8424036483816,23.6649809073197));
#61540=CARTESIAN_POINT('Ctrl Pts',(56.7909933359761,29.8792153724512,23.6675863280913));
#61541=CARTESIAN_POINT('Ctrl Pts',(56.7727391922468,29.9154583669337,23.6701917488629));
#61542=CARTESIAN_POINT('Ctrl Pts',(56.7534268006312,29.9510636242272,23.6727971696346));
#61543=CARTESIAN_POINT('Ctrl Pts',(56.7194988970924,30.0136147447188,23.6773743585389));
#61544=CARTESIAN_POINT('Ctrl Pts',(56.6821654181802,30.0744490461571,23.6819515474432));
#61545=CARTESIAN_POINT('Ctrl Pts',(56.6416212702106,30.1331845249968,23.6865287363475));
#61546=CARTESIAN_POINT('Ctrl Pts',(56.5999260677838,30.1935875129124,23.691235872333));
#61547=CARTESIAN_POINT('Ctrl Pts',(56.5548352799137,30.2517702301202,23.6959430083185));
#61548=CARTESIAN_POINT('Ctrl Pts',(56.5066120605671,30.3073437426529,23.700650144304));
#61549=CARTESIAN_POINT('Ctrl Pts',(56.4598751211621,30.3612044330623,23.7052122024227));
#61550=CARTESIAN_POINT('Ctrl Pts',(56.4101963491268,30.4126140338595,23.7097742605413));
#61551=CARTESIAN_POINT('Ctrl Pts',(56.3578584746602,30.4612487554464,23.7143363186599));
#61552=CARTESIAN_POINT('Ctrl Pts',(56.3055697505126,30.5098378043324,23.7188940925654));
#61553=CARTESIAN_POINT('Ctrl Pts',(56.2506272201341,30.5556568431123,23.7234518664708));
#61554=CARTESIAN_POINT('Ctrl Pts',(56.193351055624,30.5984182245398,23.7280096403763));
#61555=CARTESIAN_POINT('Ctrl Pts',(56.1361132473686,30.6411509698593,23.7325643620673));
#61556=CARTESIAN_POINT('Ctrl Pts',(56.0765452772435,30.6808298560183,23.7371190837583));
#61557=CARTESIAN_POINT('Ctrl Pts',(56.0149999893189,30.7172077871308,23.7416738054493));
#61558=CARTESIAN_POINT('Ctrl Pts',(55.9534793501874,30.7535711489379,23.7462267029812));
#61559=CARTESIAN_POINT('Ctrl Pts',(55.8899833615618,30.7866359535699,23.7507796005132));
#61560=CARTESIAN_POINT('Ctrl Pts',(55.824892246756,30.8161994228999,23.7553324980452));
#61561=CARTESIAN_POINT('Ctrl Pts',(55.7597915763966,30.845767232228,23.7598860639549));
#61562=CARTESIAN_POINT('Ctrl Pts',(55.6930957255118,30.8718324847587,23.7644396298647));
#61563=CARTESIAN_POINT('Ctrl Pts',(55.6252069064563,30.8942396592352,23.7689931957745));
#61564=CARTESIAN_POINT('Ctrl Pts',(55.5573127849839,30.916648583811,23.7735471173379));
#61565=CARTESIAN_POINT('Ctrl Pts',(55.4882259463757,30.9353987263845,23.7781010389013));
#61566=CARTESIAN_POINT('Ctrl Pts',(55.4183641249596,30.9503843266,23.7826549604647));
#61567=CARTESIAN_POINT('Ctrl Pts',(55.3484544890822,30.9653801831813,23.7872119987992));
#61568=CARTESIAN_POINT('Ctrl Pts',(55.2777692603935,30.9766062679254,23.7917690371337));
#61569=CARTESIAN_POINT('Ctrl Pts',(55.2067358047839,30.9840080316169,23.7963260754682));
#61570=CARTESIAN_POINT('Ctrl Pts',(55.1902444778306,30.9857264459052,23.7973840503121));
#61571=CARTESIAN_POINT('Ctrl Pts',(55.17373440234,30.9872389516035,23.7984420251561));
#61572=CARTESIAN_POINT('Ctrl Pts',(55.1572109533382,30.9885452669352,23.7995));
#61573=CARTESIAN_POINT('Ctrl Pts',(53.0052505724191,29.0015111801821,23.2106966576448));
#61574=CARTESIAN_POINT('Ctrl Pts',(53.0053532058501,29.1369867378291,23.2014815125057));
#61575=CARTESIAN_POINT('Ctrl Pts',(53.0192563134189,29.2719984182957,23.1919432329457));
#61576=CARTESIAN_POINT('Ctrl Pts',(53.0466869980277,29.4044698738173,23.182578193545));
#61577=CARTESIAN_POINT('Origin',(55.,29.,23.7995));
#61578=CARTESIAN_POINT('',(57.0818213830407,27.7073399599607,23.7995));
#61579=CARTESIAN_POINT('',(52.5495,29.,23.7995));
#61580=CARTESIAN_POINT('Origin',(55.,29.,23.7995));
#61581=CARTESIAN_POINT('Ctrl Pts',(57.0818213830407,27.7073399599607,23.7995));
#61582=CARTESIAN_POINT('Ctrl Pts',(57.1030396553067,27.7491534849406,23.7995));
#61583=CARTESIAN_POINT('Ctrl Pts',(57.1229432336361,27.7915806564359,23.7995));
#61584=CARTESIAN_POINT('Ctrl Pts',(57.1414767532722,27.834592368553,23.7995));
#61585=CARTESIAN_POINT('Ctrl Pts',(57.1752210883004,27.9129046185899,23.7995));
#61586=CARTESIAN_POINT('Ctrl Pts',(57.204426630953,27.9931545233241,23.7995));
#61587=CARTESIAN_POINT('Ctrl Pts',(57.2291348926794,28.0749451167352,23.7995));
#61588=CARTESIAN_POINT('Ctrl Pts',(57.2415707567772,28.1161109711122,23.7995));
#61589=CARTESIAN_POINT('Ctrl Pts',(57.2528665481713,28.1576672136207,23.7995));
#61590=CARTESIAN_POINT('Ctrl Pts',(57.2630226514886,28.1995631640058,23.7995));
#61591=CARTESIAN_POINT('Ctrl Pts',(57.2679451975272,28.219869647522,23.7995));
#61592=CARTESIAN_POINT('Ctrl Pts',(57.2725999564407,28.2402559300432,23.7995));
#61593=CARTESIAN_POINT('Ctrl Pts',(57.2769867024841,28.2607161878036,23.7995));
#61594=CARTESIAN_POINT('Ctrl Pts',(57.2803633605224,28.2764652859161,23.7995));
#61595=CARTESIAN_POINT('Ctrl Pts',(57.283579417055,28.2922499240532,23.7995));
#61596=CARTESIAN_POINT('Ctrl Pts',(57.2866346383619,28.3080640271147,23.7995));
#61597=CARTESIAN_POINT('Ctrl Pts',(57.3027426818727,28.3914407237968,23.7995));
#61598=CARTESIAN_POINT('Ctrl Pts',(57.3143907517678,28.4756669169532,23.7995));
#61599=CARTESIAN_POINT('Ctrl Pts',(57.3216193457988,28.560349030643,23.7995));
#61600=CARTESIAN_POINT('Ctrl Pts',(57.3272123451589,28.625870348572,23.7995));
#61601=CARTESIAN_POINT('Ctrl Pts',(57.3301584584012,28.6916648728046,23.7995));
#61602=CARTESIAN_POINT('Ctrl Pts',(57.3304553643523,28.7575465748756,23.7995));
#61603=CARTESIAN_POINT('Ctrl Pts',(57.3306021462004,28.7901166124713,23.7995));
#61604=CARTESIAN_POINT('Ctrl Pts',(57.3301011767369,28.8227078729075,23.7995));
#61605=CARTESIAN_POINT('Ctrl Pts',(57.3289505854467,28.8552972137907,23.7995));
#61606=CARTESIAN_POINT('Ctrl Pts',(57.3282547843989,28.8750050785456,23.7995));
#61607=CARTESIAN_POINT('Ctrl Pts',(57.3273209535759,28.8947175616372,23.7995));
#61608=CARTESIAN_POINT('Ctrl Pts',(57.3261507382989,28.9143980333835,23.7995));
#61609=CARTESIAN_POINT('Ctrl Pts',(57.321219325461,28.9973336546602,23.7995));
#61610=CARTESIAN_POINT('Ctrl Pts',(57.3120931008026,29.0797939101152,23.7995));
#61611=CARTESIAN_POINT('Ctrl Pts',(57.2988083985721,29.1614134126558,23.7995));
#61612=CARTESIAN_POINT('Ctrl Pts',(57.2856622806402,29.2421814710828,23.7995));
#61613=CARTESIAN_POINT('Ctrl Pts',(57.2684436947102,29.3221271630888,23.7995));
#61614=CARTESIAN_POINT('Ctrl Pts',(57.2471404962224,29.4008787730705,23.7995));
#61615=CARTESIAN_POINT('Ctrl Pts',(57.2264556547298,29.4773445005381,23.7995));
#61616=CARTESIAN_POINT('Ctrl Pts',(57.2019195046976,29.5526851565708,23.7995));
#61617=CARTESIAN_POINT('Ctrl Pts',(57.1734812055056,29.6265319791042,23.7995));
#61618=CARTESIAN_POINT('Ctrl Pts',(57.1631231693767,29.653429088901,23.7995));
#61619=CARTESIAN_POINT('Ctrl Pts',(57.1522471027555,29.6801276936848,23.7995));
#61620=CARTESIAN_POINT('Ctrl Pts',(57.1408493279597,29.7066087272485,23.7995));
#61621=CARTESIAN_POINT('Ctrl Pts',(57.1357954958359,29.7183505540957,23.7995));
#61622=CARTESIAN_POINT('Ctrl Pts',(57.1306390832675,29.7300495949142,23.7995));
#61623=CARTESIAN_POINT('Ctrl Pts',(57.125379729995,29.7417041391356,23.7995));
#61624=CARTESIAN_POINT('Ctrl Pts',(57.1196168749922,29.7544744257074,23.7995));
#61625=CARTESIAN_POINT('Ctrl Pts',(57.1137336869214,29.7671839514575,23.7995));
#61626=CARTESIAN_POINT('Ctrl Pts',(57.1077332174747,29.7798243326649,23.7995));
#61627=CARTESIAN_POINT('Ctrl Pts',(57.0742497329774,29.8503594819485,23.7995));
#61628=CARTESIAN_POINT('Ctrl Pts',(57.0370888487061,29.9188081298351,23.7995));
#61629=CARTESIAN_POINT('Ctrl Pts',(56.9962424222594,29.9848386006808,23.7995));
#61630=CARTESIAN_POINT('Ctrl Pts',(56.9810932635781,30.00932803997,23.7995));
#61631=CARTESIAN_POINT('Ctrl Pts',(56.9654367357015,30.0334845581951,23.7995));
#61632=CARTESIAN_POINT('Ctrl Pts',(56.9492709954722,30.0572900658797,23.7995));
#61633=CARTESIAN_POINT('Ctrl Pts',(56.904600395496,30.1230715454731,23.7995));
#61634=CARTESIAN_POINT('Ctrl Pts',(56.8560436870518,30.1861759538499,23.7995));
#61635=CARTESIAN_POINT('Ctrl Pts',(56.8039291296095,30.2464231547475,23.7995));
#61636=CARTESIAN_POINT('Ctrl Pts',(56.753493550458,30.3047293674193,23.7995));
#61637=CARTESIAN_POINT('Ctrl Pts',(56.6997246599247,30.3603596510879,23.7995));
#61638=CARTESIAN_POINT('Ctrl Pts',(56.6429003401567,30.4131086059567,23.7995));
#61639=CARTESIAN_POINT('Ctrl Pts',(56.631007338023,30.4241486577403,23.7995));
#61640=CARTESIAN_POINT('Ctrl Pts',(56.6189775044667,30.4350648031822,23.7995));
#61641=CARTESIAN_POINT('Ctrl Pts',(56.6068336367285,30.4458373588959,23.7995));
#61642=CARTESIAN_POINT('Ctrl Pts',(56.548571484007,30.4975204222927,23.7995));
#61643=CARTESIAN_POINT('Ctrl Pts',(56.4876029081873,30.5459827779286,23.7995));
#61644=CARTESIAN_POINT('Ctrl Pts',(56.4242546407422,30.5910801684579,23.7995));
#61645=CARTESIAN_POINT('Ctrl Pts',(56.3610994478872,30.6360401099214,23.7995));
#61646=CARTESIAN_POINT('Ctrl Pts',(56.2955780376467,30.6776559088237,23.7995));
#61647=CARTESIAN_POINT('Ctrl Pts',(56.2279927066909,30.7157377301824,23.7995));
#61648=CARTESIAN_POINT('Ctrl Pts',(56.1614582290472,30.7532274347675,23.7995));
#61649=CARTESIAN_POINT('Ctrl Pts',(56.0929225858511,30.7872924132189,23.7995));
#61650=CARTESIAN_POINT('Ctrl Pts',(56.0226677290349,30.8177021134375,23.7995));
#61651=CARTESIAN_POINT('Ctrl Pts',(55.9956814080747,30.8293830984625,23.7995));
#61652=CARTESIAN_POINT('Ctrl Pts',(55.9684414235731,30.8405242122541,23.7995));
#61653=CARTESIAN_POINT('Ctrl Pts',(55.9409639301567,30.8511103048716,23.7995));
#61654=CARTESIAN_POINT('Ctrl Pts',(55.9293858895887,30.8555709086074,23.7995));
#61655=CARTESIAN_POINT('Ctrl Pts',(55.9177654819835,30.859932941087,23.7995));
#61656=CARTESIAN_POINT('Ctrl Pts',(55.9061177979359,30.8641903960764,23.7995));
#61657=CARTESIAN_POINT('Ctrl Pts',(55.8355459925781,30.8899857630871,23.7995));
#61658=CARTESIAN_POINT('Ctrl Pts',(55.7638488209893,30.9119951518818,23.7995));
#61659=CARTESIAN_POINT('Ctrl Pts',(55.6913062742255,30.9300521964143,23.7995));
#61660=CARTESIAN_POINT('Ctrl Pts',(55.620784624429,30.9476062061325,23.7995));
#61661=CARTESIAN_POINT('Ctrl Pts',(55.5494632169023,30.9614250473839,23.7995));
#61662=CARTESIAN_POINT('Ctrl Pts',(55.4775979949367,30.9713078399483,23.7995));
#61663=CARTESIAN_POINT('Ctrl Pts',(55.4067390150588,30.9810522556797,23.7995));
#61664=CARTESIAN_POINT('Ctrl Pts',(55.3353506394514,30.9869701931208,23.7995));
#61665=CARTESIAN_POINT('Ctrl Pts',(55.263688103798,30.9888204486881,23.7995));
#61666=CARTESIAN_POINT('Ctrl Pts',(55.2282516842486,30.989735381881,23.7995));
#61667=CARTESIAN_POINT('Ctrl Pts',(55.1927484456801,30.9896549180268,23.7995));
#61668=CARTESIAN_POINT('Ctrl Pts',(55.1572109533382,30.9885452669352,23.7995));
#61669=CARTESIAN_POINT('',(53.1673064968656,29.7915239329253,23.80042507898));
#61670=CARTESIAN_POINT('Ctrl Pts',(53.1796208058588,29.8156268460748,23.7995000000001));
#61671=CARTESIAN_POINT('Ctrl Pts',(53.1759393605194,29.8074103111085,23.79980835966));
#61672=CARTESIAN_POINT('Ctrl Pts',(53.1723135457441,29.7991688506918,23.80011671932));
#61673=CARTESIAN_POINT('Ctrl Pts',(53.1687436939319,29.7909032203662,23.80042507898));
#61674=CARTESIAN_POINT('Ctrl Pts',(53.165787664683,29.7920814616361,23.7995));
#61675=CARTESIAN_POINT('Ctrl Pts',(53.1401820698082,29.7477636700476,23.7995));
#61676=CARTESIAN_POINT('Ctrl Pts',(53.1164423925447,29.7024883184289,23.7995));
#61677=CARTESIAN_POINT('Ctrl Pts',(53.0946595038619,29.6563380756085,23.7995));
#61678=CARTESIAN_POINT('Ctrl Pts',(53.0640455095737,29.5914778410146,23.7995));
#61679=CARTESIAN_POINT('Ctrl Pts',(53.037294163456,29.524890812006,23.7995));
#61680=CARTESIAN_POINT('Ctrl Pts',(53.0142981560509,29.456912722762,23.7995));
#61681=CARTESIAN_POINT('Ctrl Pts',(53.0009606170863,29.4174858606089,23.7995));
#61682=CARTESIAN_POINT('Ctrl Pts',(52.9888871151828,29.3775904012731,23.7995));
#61683=CARTESIAN_POINT('Ctrl Pts',(52.9780631887975,29.3372874974198,23.7995));
#61684=CARTESIAN_POINT('Ctrl Pts',(52.9745837243386,29.3243317070202,23.7995));
#61685=CARTESIAN_POINT('Ctrl Pts',(52.9712330997116,29.3113324732422,23.7995));
#61686=CARTESIAN_POINT('Ctrl Pts',(52.9680119647507,29.2982959373246,23.7995));
#61687=CARTESIAN_POINT('Ctrl Pts',(52.9500851274445,29.2257426723206,23.7995));
#61688=CARTESIAN_POINT('Ctrl Pts',(52.9362078481641,29.1522120659674,23.7995));
#61689=CARTESIAN_POINT('Ctrl Pts',(52.9262598407908,29.0780700769049,23.7995));
#61690=CARTESIAN_POINT('Ctrl Pts',(52.9178400915168,29.0153181171246,23.7995));
#61691=CARTESIAN_POINT('Ctrl Pts',(52.9122358150479,28.9521272587033,23.7995));
#61692=CARTESIAN_POINT('Ctrl Pts',(52.9093993969571,28.8887050743856,23.7995));
#61693=CARTESIAN_POINT('Ctrl Pts',(52.9080492667043,28.8585162210475,23.7995));
#61694=CARTESIAN_POINT('Ctrl Pts',(52.907326603863,28.8282748042801,23.7995));
#61695=CARTESIAN_POINT('Ctrl Pts',(52.9072281478651,28.7980025837903,23.7995));
#61696=CARTESIAN_POINT('Ctrl Pts',(52.9071800358105,28.7832095924427,23.7995));
#61697=CARTESIAN_POINT('Ctrl Pts',(52.9072810447628,28.7684067535663,23.7995));
#61698=CARTESIAN_POINT('Ctrl Pts',(52.9075307536315,28.7536046094758,23.7995));
#61699=CARTESIAN_POINT('Ctrl Pts',(52.9088393982126,28.6760312907818,23.7995));
#61700=CARTESIAN_POINT('Ctrl Pts',(52.9142236191172,28.5986682948975,23.7995));
#61701=CARTESIAN_POINT('Ctrl Pts',(52.9235643439375,28.5218879125633,23.7995));
#61702=CARTESIAN_POINT('Ctrl Pts',(52.9332602936395,28.4421875959892,23.7995));
#61703=CARTESIAN_POINT('Ctrl Pts',(52.9472190372289,28.3631140585917,23.7995));
#61704=CARTESIAN_POINT('Ctrl Pts',(52.9653613277415,28.2850644949545,23.7995));
#61705=CARTESIAN_POINT('Ctrl Pts',(52.9831194474831,28.2086676642516,23.7995));
#61706=CARTESIAN_POINT('Ctrl Pts',(53.0048859614684,28.1332507805631,23.7995));
#61707=CARTESIAN_POINT('Ctrl Pts',(53.0306380316024,28.0591843708784,23.7995));
#61708=CARTESIAN_POINT('Ctrl Pts',(53.0394167579217,28.0339355758613,23.7995));
#61709=CARTESIAN_POINT('Ctrl Pts',(53.0486590790892,28.0088437755125,23.7995));
#61710=CARTESIAN_POINT('Ctrl Pts',(53.0583654557726,27.983923948249,23.7995));
#61711=CARTESIAN_POINT('Ctrl Pts',(53.0630790096306,27.9718225275264,23.7995));
#61712=CARTESIAN_POINT('Ctrl Pts',(53.0679020080437,27.9597616651288,23.7995));
#61713=CARTESIAN_POINT('Ctrl Pts',(53.0728345632088,27.9477430987234,23.7995));
#61714=CARTESIAN_POINT('Ctrl Pts',(53.0780479523345,27.9350402578415,23.7995));
#61715=CARTESIAN_POINT('Ctrl Pts',(53.0833805561955,27.9223925031397,23.7995));
#61716=CARTESIAN_POINT('Ctrl Pts',(53.0888294627625,27.909807514102,23.7995));
#61717=CARTESIAN_POINT('Ctrl Pts',(53.1210151517875,27.8354702982651,23.7995));
#61718=CARTESIAN_POINT('Ctrl Pts',(53.1572806186558,27.7632594115094,23.7995));
#61719=CARTESIAN_POINT('Ctrl Pts',(53.1975435690432,27.6935631803969,23.7995));
#61720=CARTESIAN_POINT('Ctrl Pts',(53.2111784159906,27.6699609000155,23.7995));
#61721=CARTESIAN_POINT('Ctrl Pts',(53.2252721371432,27.6466469888357,23.7995));
#61722=CARTESIAN_POINT('Ctrl Pts',(53.2398228910682,27.6236366097474,23.7995));
#61723=CARTESIAN_POINT('Ctrl Pts',(53.2817577761606,27.5573213103493,23.7995));
#61724=CARTESIAN_POINT('Ctrl Pts',(53.3274848540066,27.4935254236365,23.7995));
#61725=CARTESIAN_POINT('Ctrl Pts',(53.3766655016659,27.4323469456169,23.7995));
#61726=CARTESIAN_POINT('Ctrl Pts',(53.4258461493252,27.3711684675974,23.7995));
#61727=CARTESIAN_POINT('Ctrl Pts',(53.4784810156533,27.3126068943904,23.7995000000001));
#61728=CARTESIAN_POINT('Ctrl Pts',(53.5342771578376,27.2567856770345,23.7995));
#61729=CARTESIAN_POINT('Ctrl Pts',(53.5477935777438,27.2432631827559,23.7995));
#61730=CARTESIAN_POINT('Ctrl Pts',(53.5615006180451,27.2298971458495,23.7995));
#61731=CARTESIAN_POINT('Ctrl Pts',(53.5753681819369,27.2167140140831,23.7995));
#61732=CARTESIAN_POINT('Ctrl Pts',(53.633752056695,27.1612116691885,23.7995));
#61733=CARTESIAN_POINT('Ctrl Pts',(53.6950394894952,27.108883136901,23.7995));
#61734=CARTESIAN_POINT('Ctrl Pts',(53.7588597602439,27.0598159162569,23.7995));
#61735=CARTESIAN_POINT('Ctrl Pts',(53.8246617759526,27.0092250618821,23.7995));
#61736=CARTESIAN_POINT('Ctrl Pts',(53.8931568786773,26.9621005359295,23.7995));
#61737=CARTESIAN_POINT('Ctrl Pts',(53.9639880369228,26.9185657891014,23.7995));
#61738=CARTESIAN_POINT('Ctrl Pts',(54.0348191951683,26.8750310422733,23.7995));
#61739=CARTESIAN_POINT('Ctrl Pts',(54.107987210922,26.8350855029082,23.7995));
#61740=CARTESIAN_POINT('Ctrl Pts',(54.1831732887653,26.7988889473287,23.7995));
#61741=CARTESIAN_POINT('Ctrl Pts',(54.2150841291888,26.7835262293614,23.7995));
#61742=CARTESIAN_POINT('Ctrl Pts',(54.2473588964334,26.7688393372961,23.7995));
#61743=CARTESIAN_POINT('Ctrl Pts',(54.279974752017,26.754842857782,23.7995));
#61744=CARTESIAN_POINT('Ctrl Pts',(54.2965159643313,26.7477445083702,23.7995));
#61745=CARTESIAN_POINT('Ctrl Pts',(54.313149574602,26.7408220047297,23.7995));
#61746=CARTESIAN_POINT('Ctrl Pts',(54.3298442609607,26.7340884936375,23.7995));
#61747=CARTESIAN_POINT('Ctrl Pts',(54.4093433274494,26.7020239292294,23.7995));
#61748=CARTESIAN_POINT('Ctrl Pts',(54.4903303509709,26.6741939381907,23.7995));
#61749=CARTESIAN_POINT('Ctrl Pts',(54.5724341788774,26.6507190230252,23.7995));
#61750=CARTESIAN_POINT('Ctrl Pts',(54.6544887625027,26.6272581876579,23.7995));
#61751=CARTESIAN_POINT('Ctrl Pts',(54.7376596641008,26.6081466518036,23.7995));
#61752=CARTESIAN_POINT('Ctrl Pts',(54.8216091428745,26.5935443949621,23.7995));
#61753=CARTESIAN_POINT('Ctrl Pts',(54.9045672100692,26.5791145852487,23.7995));
#61754=CARTESIAN_POINT('Ctrl Pts',(54.9882864392925,26.5690877150561,23.7995));
#61755=CARTESIAN_POINT('Ctrl Pts',(55.0724600567375,26.5636643588097,23.7995));
#61756=CARTESIAN_POINT('Ctrl Pts',(55.1197647546895,26.5606164889794,23.7995));
#61757=CARTESIAN_POINT('Ctrl Pts',(55.167213237544,26.5590234297658,23.7995));
#61758=CARTESIAN_POINT('Ctrl Pts',(55.2147522011135,26.5589281571169,23.7995));
#61759=CARTESIAN_POINT('Origin',(55.,29.,23.7995));
#61760=CARTESIAN_POINT('Ctrl Pts',(54.1264195366494,30.7893316856308,4.66531914574752));
#61761=CARTESIAN_POINT('Ctrl Pts',(53.5328852721049,30.4995587262633,4.707553422536));
#61762=CARTESIAN_POINT('Ctrl Pts',(52.6669803260193,29.287877577452,4.79202197611296));
#61763=CARTESIAN_POINT('Ctrl Pts',(53.4895592866451,27.1957792326284,4.91872480647843));
#61764=CARTESIAN_POINT('Ctrl Pts',(55.6906360859252,26.7527320219417,5.04542763684387));
#61765=CARTESIAN_POINT('Ctrl Pts',(57.2612985360137,28.3549210763986,5.17213046720934));
#61766=CARTESIAN_POINT('Ctrl Pts',(56.7720339725362,30.5461560293319,5.29883329757478));
#61767=CARTESIAN_POINT('Ctrl Pts',(54.6678069104706,31.3278986568886,5.42553612794023));
#61768=CARTESIAN_POINT('Ctrl Pts',(52.8664205998243,29.9887889527256,5.55223895830568));
#61769=CARTESIAN_POINT('Ctrl Pts',(53.009073421732,27.7485304409038,5.67894178867113));
#61770=CARTESIAN_POINT('Ctrl Pts',(54.9658935874079,26.648693626069,5.80564461903658));
#61771=CARTESIAN_POINT('Ctrl Pts',(56.9537719413826,27.6913201942627,5.93234744940203));
#61772=CARTESIAN_POINT('Ctrl Pts',(57.1613864127378,29.9264357302167,6.05905027976748));
#61773=CARTESIAN_POINT('Ctrl Pts',(55.3995439881701,31.317373277448,6.18575311013294));
#61774=CARTESIAN_POINT('Ctrl Pts',(53.2736403188764,30.5967297689046,6.31245594049839));
#61775=CARTESIAN_POINT('Ctrl Pts',(52.720791484149,28.4211457420414,6.43915877086384));
#61776=CARTESIAN_POINT('Ctrl Pts',(54.2447544488578,26.7730142754301,6.56586160122929));
#61777=CARTESIAN_POINT('Ctrl Pts',(56.4568955974548,27.1541078477562,6.69256443159474));
#61778=CARTESIAN_POINT('Ctrl Pts',(57.3415160026948,29.2171757615622,6.8192672619602));
#61779=CARTESIAN_POINT('Ctrl Pts',(56.0925507123657,31.0823532731961,6.94597009232564));
#61780=CARTESIAN_POINT('Ctrl Pts',(53.848055020457,31.0500939414026,7.0726729226911));
#61781=CARTESIAN_POINT('Ctrl Pts',(52.6532097130149,29.1497922643776,7.19937575305655));
#61782=CARTESIAN_POINT('Ctrl Pts',(53.5967559427171,27.113000143957,7.32607858342201));
#61783=CARTESIAN_POINT('Ctrl Pts',(55.8189358885639,26.7956392360687,7.45278141378746));
#61784=CARTESIAN_POINT('Ctrl Pts',(57.2949027764116,28.4868883085401,7.5794842441529));
#61785=CARTESIAN_POINT('Ctrl Pts',(56.6797579534097,30.64568392336,7.70618707451836));
#61786=CARTESIAN_POINT('Ctrl Pts',(54.5340203927282,31.3049350027155,7.83288990488381));
#61787=CARTESIAN_POINT('Ctrl Pts',(52.8128826983748,29.8639330234614,7.95959273524927));
#61788=CARTESIAN_POINT('Ctrl Pts',(53.0846427626806,27.6357166668124,8.08629556561471));
#61789=CARTESIAN_POINT('Ctrl Pts',(55.1016732529539,26.6506330831788,8.21299839598018));
#61790=CARTESIAN_POINT('Ctrl Pts',(57.0260592391414,27.8062888458497,8.3397012263456));
#61791=CARTESIAN_POINT('Ctrl Pts',(57.1043033136765,30.0496522872255,8.46640405671108));
#61792=CARTESIAN_POINT('Ctrl Pts',(55.2651096020556,31.3365742571087,8.59310688707651));
#61793=CARTESIAN_POINT('Ctrl Pts',(53.1843484485316,30.4944135316941,8.71980971744197));
#61794=CARTESIAN_POINT('Ctrl Pts',(52.758006060917,28.2905456059944,8.84651254780742));
#61795=CARTESIAN_POINT('Ctrl Pts',(54.3745649353107,26.7331313800921,8.97321537817288));
#61796=CARTESIAN_POINT('Ctrl Pts',(56.5610192321176,27.2412841852587,9.09991820853831));
#61797=CARTESIAN_POINT('Ctrl Pts',(57.3250753218085,29.3519760048347,9.22662103890378));
#61798=CARTESIAN_POINT('Ctrl Pts',(55.9705265275212,31.1419478563778,9.35332386926922));
#61799=CARTESIAN_POINT('Ctrl Pts',(53.7316355263593,30.9801802751439,9.48002669963468));
#61800=CARTESIAN_POINT('Ctrl Pts',(52.6484761883034,29.014075620299,9.60672953000012));
#61801=CARTESIAN_POINT('Ctrl Pts',(53.708021555563,27.0351452829349,9.73343236036558));
#61802=CARTESIAN_POINT('Ctrl Pts',(55.9448155980397,26.8465873953736,9.86013519073104));
#61803=CARTESIAN_POINT('Ctrl Pts',(57.3206951911261,28.6202156007059,9.98683802109648));
#61804=CARTESIAN_POINT('Ctrl Pts',(56.5819610682486,30.7399027382612,10.1135408514619));
#61805=CARTESIAN_POINT('Ctrl Pts',(54.4017465709424,31.2741933063581,10.2402436818274));
#61806=CARTESIAN_POINT('Ctrl Pts',(52.766659633492,29.7362426009061,10.3669465121928));
#61807=CARTESIAN_POINT('Ctrl Pts',(53.1665888366757,27.5274288247217,10.4936493425583));
#61808=CARTESIAN_POINT('Ctrl Pts',(55.2371193354502,26.6604195288858,10.6203521729237));
#61809=CARTESIAN_POINT('Ctrl Pts',(57.0915870781246,27.925232185686,10.7470550032892));
#61810=CARTESIAN_POINT('Ctrl Pts',(57.0402040479584,30.1693715417937,10.8737578336547));
#61811=CARTESIAN_POINT('Ctrl Pts',(55.1297903791825,31.3479814346657,11.0004606640201));
#61812=CARTESIAN_POINT('Ctrl Pts',(53.1011119261864,30.3871144304603,11.1271634943856));
#61813=CARTESIAN_POINT('Ctrl Pts',(52.8026972240355,28.162310993983,11.253866324751));
#61814=CARTESIAN_POINT('Ctrl Pts',(54.5064612681272,26.7008084289898,11.3805691551165));
#61815=CARTESIAN_POINT('Ctrl Pts',(56.6599370088555,27.3343255159861,11.5072719854819));
#61816=CARTESIAN_POINT('Ctrl Pts',(57.3008808238125,29.485602506866,11.6339748158474));
#61817=CARTESIAN_POINT('Ctrl Pts',(55.8452657423508,31.1943992765382,11.7606776462128));
#61818=CARTESIAN_POINT('Ctrl Pts',(53.6194458794751,30.9036629639631,11.8873804765783));
#61819=CARTESIAN_POINT('Ctrl Pts',(52.6515847050371,28.8783120283382,12.0140833069437));
#61820=CARTESIAN_POINT('Ctrl Pts',(53.8235957604794,26.9638429762661,12.1407861373092));
#61821=CARTESIAN_POINT('Ctrl Pts',(56.0675444619859,26.9047169208562,12.2674889676746));
#61822=CARTESIAN_POINT('Ctrl Pts',(57.3387483711783,28.7548094284558,12.3941917980401));
#61823=CARTESIAN_POINT('Ctrl Pts',(56.4788885358544,30.8283191894692,12.5208946284055));
#61824=CARTESIAN_POINT('Ctrl Pts',(54.2714678514121,31.2358674532577,12.647597458771));
#61825=CARTESIAN_POINT('Ctrl Pts',(52.7278844859831,29.6060968990407,12.7743002891364));
#61826=CARTESIAN_POINT('Ctrl Pts',(53.2546491130723,27.4240518277673,12.9010031195019));
#61827=CARTESIAN_POINT('Ctrl Pts',(55.3717746538996,26.6780081897687,13.0277059498673));
#61828=CARTESIAN_POINT('Ctrl Pts',(57.1501397295913,28.0477597449719,13.1544087802328));
#61829=CARTESIAN_POINT('Ctrl Pts',(56.9693009508439,30.2851910850408,13.2811116105982));
#61830=CARTESIAN_POINT('Ctrl Pts',(54.9940383212441,31.3515583808295,13.4078144409637));
#61831=CARTESIAN_POINT('Ctrl Pts',(53.0242079637134,30.2751894719645,13.5345172713291));
#61832=CARTESIAN_POINT('Ctrl Pts',(52.8547161236231,28.0368699725265,13.6612201016946));
#61833=CARTESIAN_POINT('Ctrl Pts',(54.6400034923536,26.6761530010465,13.7879229320601));
#61834=CARTESIAN_POINT('Ctrl Pts',(56.7533190983459,27.4329216677402,13.9146257624255));
#61835=CARTESIAN_POINT('Ctrl Pts',(57.2690131692052,29.6176095838284,14.041328592791));
#61836=CARTESIAN_POINT('Ctrl Pts',(55.7171860991359,31.2395326430462,14.1680314231564));
#61837=CARTESIAN_POINT('Ctrl Pts',(53.5118602120182,30.8207971692334,14.2947342535218));
#61838=CARTESIAN_POINT('Ctrl Pts',(52.6625249000395,28.742954250905,14.4214370838873));
#61839=CARTESIAN_POINT('Ctrl Pts',(53.9430931298965,26.899331004658,14.5481399142527));
#61840=CARTESIAN_POINT('Ctrl Pts',(56.186713195498,26.9698339595752,14.6748427446182));
#61841=CARTESIAN_POINT('Ctrl Pts',(57.349002110972,28.890220936824,14.8015455749836));
#61842=CARTESIAN_POINT('Ctrl Pts',(56.3708840907646,30.9106384194169,14.9282484053491));
#61843=CARTESIAN_POINT('Ctrl Pts',(54.1436186976438,31.1900852551985,15.0549512357145));
#61844=CARTESIAN_POINT('Ctrl Pts',(52.6966865662897,29.4739299380211,15.18165406608));
#61845=CARTESIAN_POINT('Ctrl Pts',(53.3485299215708,27.325930425545,15.3083568964455));
#61846=CARTESIAN_POINT('Ctrl Pts',(55.5051901492716,26.7033404098252,15.4350597268109));
#61847=CARTESIAN_POINT('Ctrl Pts',(57.2015219275906,28.1734629092404,15.5617625571764));
#61848=CARTESIAN_POINT('Ctrl Pts',(56.8918304755086,30.39672467294,15.6884653875418));
#61849=CARTESIAN_POINT('Ctrl Pts',(54.8583061447766,31.3472931669169,15.8151682179073));
#61850=CARTESIAN_POINT('Ctrl Pts',(52.9538930264383,30.1590119122794,15.9418710482727));
#61851=CARTESIAN_POINT('Ctrl Pts',(52.913889283001,27.9146408721142,16.0685738786382));
#61852=CARTESIAN_POINT('Ctrl Pts',(54.7747462609773,26.6592473191046,16.1952767090036));
#61853=CARTESIAN_POINT('Ctrl Pts',(56.8408540827227,27.5367438343933,16.3219795393691));
#61854=CARTESIAN_POINT('Ctrl Pts',(57.2295786327234,29.7475570082386,16.4486823697345));
#61855=CARTESIAN_POINT('Ctrl Pts',(55.5867147278486,31.2771974416349,16.5753852000999));
#61856=CARTESIAN_POINT('Ctrl Pts',(53.4092373090532,30.7318592382624,16.7020880304655));
#61857=CARTESIAN_POINT('Ctrl Pts',(52.6812602890962,28.6084536896598,16.8287908608308));
#61858=CARTESIAN_POINT('Ctrl Pts',(54.0661151546778,26.8418245076593,16.9554936911964));
#61859=CARTESIAN_POINT('Ctrl Pts',(56.3019243853996,27.041721354157,17.0821965215618));
#61860=CARTESIAN_POINT('Ctrl Pts',(57.3514222155374,29.0259985449642,17.2088993519273));
#61861=CARTESIAN_POINT('Ctrl Pts',(56.2583079146159,30.9865859035235,17.3356021822927));
#61862=CARTESIAN_POINT('Ctrl Pts',(54.0186254709554,31.1369993902211,17.4623050126582));
#61863=CARTESIAN_POINT('Ctrl Pts',(52.6731699156649,29.3401824785247,17.5890078430236));
#61864=CARTESIAN_POINT('Ctrl Pts',(53.4479181811372,27.2333918409509,17.715710673389));
#61865=CARTESIAN_POINT('Ctrl Pts',(55.6369208971794,26.7363317091943,17.8424135037545));
#61866=CARTESIAN_POINT('Ctrl Pts',(57.2455623187654,28.3019224737871,17.9691163341199));
#61867=CARTESIAN_POINT('Ctrl Pts',(56.8080509765289,30.5036003545943,18.0958191644854));
#61868=CARTESIAN_POINT('Ctrl Pts',(54.7230465000152,31.3352000168956,18.2225219948509));
#61869=CARTESIAN_POINT('Ctrl Pts',(52.890401606092,30.0389691893815,18.3492248252163));
#61870=CARTESIAN_POINT('Ctrl Pts',(52.9800193669072,27.7960313118718,18.4759276555818));
#61871=CARTESIAN_POINT('Ctrl Pts',(54.9102402233175,26.650147761549,18.6026304859472));
#61872=CARTESIAN_POINT('Ctrl Pts',(56.9222500435006,27.645445781696,18.7293333163127));
#61873=CARTESIAN_POINT('Ctrl Pts',(57.1827087237314,29.8750114213024,18.8560361466781));
#61874=CARTESIAN_POINT('Ctrl Pts',(55.4542867345813,31.3072680648001,18.9827389770436));
#61875=CARTESIAN_POINT('Ctrl Pts',(53.3119194054314,30.6371457681906,19.109441807409));
#61876=CARTESIAN_POINT('Ctrl Pts',(52.7077283919724,28.4752588875521,19.2361446377745));
#61877=CARTESIAN_POINT('Ctrl Pts',(54.1922515713913,26.7915152624158,19.3628474681399));
#61878=CARTESIAN_POINT('Ctrl Pts',(56.4127938164408,27.1201393689178,19.4895502985054));
#61879=CARTESIAN_POINT('Ctrl Pts',(57.3460006141201,29.1616894511321,19.6162531288708));
#61880=CARTESIAN_POINT('Ctrl Pts',(56.1415354352125,31.0559083662008,19.7429559592363));
#61881=CARTESIAN_POINT('Ctrl Pts',(53.8969050084927,31.0767868932071,19.8696587896017));
#61882=CARTESIAN_POINT('Ctrl Pts',(52.6574129592736,29.2053005519918,19.9963616199672));
#61883=CARTESIAN_POINT('Ctrl Pts',(53.5524824440479,27.1467446788788,20.1230644503326));
#61884=CARTESIAN_POINT('Ctrl Pts',(55.7665275916892,26.7768720658948,20.2497672806981));
#61885=CARTESIAN_POINT('Ctrl Pts',(57.2821140337366,28.4327100416997,20.3764701110635));
#61886=CARTESIAN_POINT('Ctrl Pts',(56.7182418484071,30.6054617125546,20.503172941429));
#61887=CARTESIAN_POINT('Ctrl Pts',(54.5887104611592,31.3153192601402,20.6298757717944));
#61888=CARTESIAN_POINT('Ctrl Pts',(52.8339454392039,29.9154616307104,20.7565786021598));
#61889=CARTESIAN_POINT('Ctrl Pts',(53.0528858388122,27.681436840953,20.8832814325254));
#61890=CARTESIAN_POINT('Ctrl Pts',(55.0460335250711,26.6488846728187,21.0099842628908));
#61891=CARTESIAN_POINT('Ctrl Pts',(56.9972355321144,27.7586650048169,21.1366870932563));
#61892=CARTESIAN_POINT('Ctrl Pts',(57.1285597534825,29.99954777245,21.2633899236217));
#61893=CARTESIAN_POINT('Ctrl Pts',(55.3203437390977,31.3296442417868,21.3900927539872));
#61894=CARTESIAN_POINT('Ctrl Pts',(53.2202310668697,30.5369725951186,21.5167955843526));
#61895=CARTESIAN_POINT('Ctrl Pts',(52.7418408968943,28.343814075626,21.643498414718));
#61896=CARTESIAN_POINT('Ctrl Pts',(54.3210818164914,26.7485709605453,21.7702012450835));
#61897=CARTESIAN_POINT('Ctrl Pts',(56.518951584052,27.2048266531433,21.8969040754489));
#61898=CARTESIAN_POINT('Ctrl Pts',(57.3327557174393,29.2968408217187,22.0236069058144));
#61899=CARTESIAN_POINT('Ctrl Pts',(56.0209554270959,31.1183752546229,22.1503097361798));
#61900=CARTESIAN_POINT('Ctrl Pts',(53.7788645019832,31.0096473324931,22.2770125665453));
#61901=CARTESIAN_POINT('Ctrl Pts',(52.6494657578868,29.0697363896565,22.4037153969107));
#61902=CARTESIAN_POINT('Ctrl Pts',(53.6618788749301,27.0662731610901,22.5304182272762));
#61903=CARTESIAN_POINT('Ctrl Pts',(55.8935684586045,26.8248355645479,22.6571210576416));
#61904=CARTESIAN_POINT('Ctrl Pts',(57.3110738969302,28.565371261504,22.7838238880071));
#61905=CARTESIAN_POINT('Ctrl Pts',(56.6226659052376,30.7020047032443,22.9105267183726));
#61906=CARTESIAN_POINT('Ctrl Pts',(54.4558179268847,31.2876473235127,23.037229548738));
#61907=CARTESIAN_POINT('Ctrl Pts',(52.7845718724283,29.7890380715951,23.1639323791035));
#61908=CARTESIAN_POINT('Ctrl Pts',(53.1325219577503,27.5709710820395,23.2906352094689));
#61909=CARTESIAN_POINT('Ctrl Pts',(55.1811312054231,26.6559899627326,23.4173380398344));
#61910=CARTESIAN_POINT('Ctrl Pts',(57.0666303447483,27.8749743362302,23.5440408701998));
#61911=CARTESIAN_POINT('Ctrl Pts',(57.065134231683,30.1232847911398,23.6707611309521));
#61912=CARTESIAN_POINT('Ctrl Pts',(55.8148535333292,30.9332788394173,23.7552471149158));
#61913=CARTESIAN_POINT('Ctrl Pts',(55.1561153962245,30.9850638875332,23.7974988220912));
#61914=CARTESIAN_POINT('Ctrl Pts',(54.0587888680759,30.9278577897226,4.75431987392162));
#61915=CARTESIAN_POINT('Ctrl Pts',(53.4193044926757,30.6156512483342,4.7965541507101));
#61916=CARTESIAN_POINT('Ctrl Pts',(52.4863630995982,29.3101644231945,4.88102270428707));
#61917=CARTESIAN_POINT('Ctrl Pts',(53.3726243051861,27.0561004487379,5.00772553465252));
#61918=CARTESIAN_POINT('Ctrl Pts',(55.7441036051655,26.5787535022794,5.13442836501797));
#61919=CARTESIAN_POINT('Ctrl Pts',(57.4363632704608,28.3049804919693,5.26113119538342));
#61920=CARTESIAN_POINT('Ctrl Pts',(56.909220925914,30.665856011611,5.38783402574887));
#61921=CARTESIAN_POINT('Ctrl Pts',(54.6420892557349,31.5081194254857,5.51453685611433));
#61922=CARTESIAN_POINT('Ctrl Pts',(52.7012435985727,30.0653388078979,5.64123968647978));
#61923=CARTESIAN_POINT('Ctrl Pts',(52.8549402866429,27.6516444337965,5.76794251684523));
#61924=CARTESIAN_POINT('Ctrl Pts',(54.9632531443315,26.4666606837572,5.89464534721069));
#61925=CARTESIAN_POINT('Ctrl Pts',(57.105028646608,27.5900050963139,6.02134817757613));
#61926=CARTESIAN_POINT('Ctrl Pts',(57.3287161714393,29.9981583367233,6.14805100794159));
#61927=CARTESIAN_POINT('Ctrl Pts',(55.4304758006111,31.4967791944333,6.27475383830703));
#61928=CARTESIAN_POINT('Ctrl Pts',(53.1399893681846,30.7203450583168,6.4014566686725));
#61929=CARTESIAN_POINT('Ctrl Pts',(52.54434019865,28.3763321248479,6.52815949903794));
#61930=CARTESIAN_POINT('Ctrl Pts',(54.1862850076286,26.6006059630024,6.65486232940339));
#61931=CARTESIAN_POINT('Ctrl Pts',(56.5696852343928,27.0112029573562,6.78156515976885));
#61932=CARTESIAN_POINT('Ctrl Pts',(57.5227909961055,29.2339890289928,6.90826799013429));
#61933=CARTESIAN_POINT('Ctrl Pts',(56.1771335736217,31.2435644609235,7.03497082049975));
#61934=CARTESIAN_POINT('Ctrl Pts',(53.7588739863169,31.2088076829662,7.16167365086519));
#61935=CARTESIAN_POINT('Ctrl Pts',(52.4715263961725,29.1613888503957,7.28837648123066));
#61936=CARTESIAN_POINT('Ctrl Pts',(53.4881198894316,26.9669127859905,7.4150793115961));
#61937=CARTESIAN_POINT('Ctrl Pts',(55.8823360949398,26.6249824980852,7.54178214196155));
#61938=CARTESIAN_POINT('Ctrl Pts',(57.4725690768737,28.4471643355324,7.66848497232701));
#61939=CARTESIAN_POINT('Ctrl Pts',(56.8098011013468,30.7730891352056,7.79518780269245));
#61940=CARTESIAN_POINT('Ctrl Pts',(54.4979452815009,31.4833779759637,7.92189063305792));
#61941=CARTESIAN_POINT('Ctrl Pts',(52.6435609111293,29.9308168085626,8.04859346342335));
#61942=CARTESIAN_POINT('Ctrl Pts',(52.9363600389347,27.5300968666704,8.17529629378881));
#61943=CARTESIAN_POINT('Ctrl Pts',(55.1095445714663,26.4687502893497,8.30199912415426));
#61944=CARTESIAN_POINT('Ctrl Pts',(57.1829122671806,27.7138743667884,8.42870195451973));
#61945=CARTESIAN_POINT('Ctrl Pts',(57.2672138250211,30.1309140472269,8.55540478488516));
#61946=CARTESIAN_POINT('Ctrl Pts',(55.2856338014677,31.5174666714988,8.68210761525061));
#61947=CARTESIAN_POINT('Ctrl Pts',(53.0437847186021,30.6101077241741,8.80881044561607));
#61948=CARTESIAN_POINT('Ctrl Pts',(52.5844358456948,28.2356212149373,8.93551327598151));
#61949=CARTESIAN_POINT('Ctrl Pts',(54.326145135019,26.5576354220616,9.06221610634698));
#61950=CARTESIAN_POINT('Ctrl Pts',(56.681869890704,27.1051282942199,9.18891893671242));
#61951=CARTESIAN_POINT('Ctrl Pts',(57.5050775140442,29.3792252091466,9.31562176707788));
#61952=CARTESIAN_POINT('Ctrl Pts',(56.0456625461001,31.3077727250115,9.44232459744333));
#61953=CARTESIAN_POINT('Ctrl Pts',(53.6334415523114,31.133481455198,9.56902742780878));
#61954=CARTESIAN_POINT('Ctrl Pts',(52.4664264124404,29.0151653237108,9.69573025817422));
#61955=CARTESIAN_POINT('Ctrl Pts',(53.6079994400906,26.8830305737127,9.82243308853968));
#61956=CARTESIAN_POINT('Ctrl Pts',(56.0179611332878,26.6798749512714,9.94913591890513));
#61957=CARTESIAN_POINT('Ctrl Pts',(57.5003582833259,28.5908135319605,10.0758387492706));
#61958=CARTESIAN_POINT('Ctrl Pts',(56.7044329974998,30.8746021625019,10.202541579636));
#61959=CARTESIAN_POINT('Ctrl Pts',(54.355431112801,31.4502563254235,10.3292444100015));
#61960=CARTESIAN_POINT('Ctrl Pts',(52.5937593587313,29.7932408757307,10.4559472403669));
#61961=CARTESIAN_POINT('Ctrl Pts',(53.0246501968509,27.4134256191966,10.5826500707324));
#61962=CARTESIAN_POINT('Ctrl Pts',(55.2554765902893,26.4792943800521,10.7093529010978));
#61963=CARTESIAN_POINT('Ctrl Pts',(57.2535131266198,27.842026037091,10.8360557314633));
#61964=CARTESIAN_POINT('Ctrl Pts',(57.1981521358314,30.2599017018651,10.9627585618287));
#61965=CARTESIAN_POINT('Ctrl Pts',(55.1398384634595,31.5297569675287,11.0894613921942));
#61966=CARTESIAN_POINT('Ctrl Pts',(52.9541042086769,30.494501763689,11.2161642225596));
#61967=CARTESIAN_POINT('Ctrl Pts',(52.6325868998799,28.0974589627044,11.3428670529251));
#61968=CARTESIAN_POINT('Ctrl Pts',(54.468252590388,26.5228100995293,11.4695698832905));
#61969=CARTESIAN_POINT('Ctrl Pts',(56.7884456630761,27.2053726791204,11.596272713656));
#61970=CARTESIAN_POINT('Ctrl Pts',(57.4790099314911,29.5231967796068,11.7229755440215));
#61971=CARTESIAN_POINT('Ctrl Pts',(55.9107043478092,31.3642848181859,11.8496783743869));
#61972=CARTESIAN_POINT('Ctrl Pts',(53.5125664309413,31.0510403429139,11.9763812047524));
#61973=CARTESIAN_POINT('Ctrl Pts',(52.4697755836688,28.8688912145425,12.1030840351178));
#61974=CARTESIAN_POINT('Ctrl Pts',(53.7325211444948,26.8062082000632,12.2297868654833));
#61975=CARTESIAN_POINT('Ctrl Pts',(56.1501913946096,26.7425047361315,12.3564896958487));
#61976=CARTESIAN_POINT('Ctrl Pts',(57.5198091006742,28.7358273163583,12.4831925262142));
#61977=CARTESIAN_POINT('Ctrl Pts',(56.5933808174717,30.9698636199331,12.6098953565796));
#61978=CARTESIAN_POINT('Ctrl Pts',(54.2150665027632,31.4089633694888,12.7365981869451));
#61979=CARTESIAN_POINT('Ctrl Pts',(52.5519823250081,29.6530195812916,12.8633010173105));
#61980=CARTESIAN_POINT('Ctrl Pts',(53.1195279052041,27.3020454036351,12.990003847676));
#61981=CARTESIAN_POINT('Ctrl Pts',(55.4005566258606,26.4982447161838,13.1167066780414));
#61982=CARTESIAN_POINT('Ctrl Pts',(57.3165987949426,27.9740394091908,13.2434095084069));
#61983=CARTESIAN_POINT('Ctrl Pts',(57.1217598776575,30.384687738151,13.3701123387723));
#61984=CARTESIAN_POINT('Ctrl Pts',(54.9935767812522,31.5336108329584,13.4968151691378));
#61985=CARTESIAN_POINT('Ctrl Pts',(52.8712465114121,30.3739118222972,13.6235179995032));
#61986=CARTESIAN_POINT('Ctrl Pts',(52.6886329876949,27.9623065746326,13.7502208298687));
#61987=CARTESIAN_POINT('Ctrl Pts',(54.6121333584417,26.4962459028513,13.8769236602341));
#61988=CARTESIAN_POINT('Ctrl Pts',(56.8890571875299,27.3116019270135,14.0036264905996));
#61989=CARTESIAN_POINT('Ctrl Pts',(57.444675153502,29.6654235526888,14.1303293209651));
#61990=CARTESIAN_POINT('Ctrl Pts',(55.7727090617147,31.4129123101694,14.2570321513305));
#61991=CARTESIAN_POINT('Ctrl Pts',(53.3966517189094,30.9617592615168,14.3837349816959));
#61992=CARTESIAN_POINT('Ctrl Pts',(52.4815627443869,28.7230543371655,14.5104378120614));
#61993=CARTESIAN_POINT('Ctrl Pts',(53.8612697361237,26.7367018542058,14.6371406424268));
#61994=CARTESIAN_POINT('Ctrl Pts',(56.2785859080682,26.8126629920581,14.7638434727923));
#61995=CARTESIAN_POINT('Ctrl Pts',(57.5308566623387,28.8817220844006,14.8905463031577));
#61996=CARTESIAN_POINT('Ctrl Pts',(56.4770149069683,31.0585558227109,15.0172491335232));
#61997=CARTESIAN_POINT('Ctrl Pts',(54.0773195500988,31.3596368148496,15.1439519638886));
#61998=CARTESIAN_POINT('Ctrl Pts',(52.5183691313298,29.5106205462822,15.2706547942541));
#61999=CARTESIAN_POINT('Ctrl Pts',(53.2206767583889,27.1963276593334,15.3973576246195));
#62000=CARTESIAN_POINT('Ctrl Pts',(55.5443008539925,26.5255381007245,15.524060454985));
#62001=CARTESIAN_POINT('Ctrl Pts',(57.3719588891393,28.1094742345918,15.6507632853505));
#62002=CARTESIAN_POINT('Ctrl Pts',(57.0382918093569,30.5048560098996,15.7774661157159));
#62003=CARTESIAN_POINT('Ctrl Pts',(54.8473365196951,31.5290154156122,15.9041689460814));
#62004=CARTESIAN_POINT('Ctrl Pts',(52.7954879471124,30.2487400527318,16.0308717764468));
#62005=CARTESIAN_POINT('Ctrl Pts',(52.7523872022796,27.8306147674328,16.1575746068123));
#62006=CARTESIAN_POINT('Ctrl Pts',(54.7573076143868,26.4780314203805,16.2842774371777));
#62007=CARTESIAN_POINT('Ctrl Pts',(56.9833689369161,27.4234617763278,16.4109802675432));
#62008=CARTESIAN_POINT('Ctrl Pts',(57.402187682369,29.8054312194704,16.5376830979086));
#62009=CARTESIAN_POINT('Ctrl Pts',(55.6321368852467,31.4534930342133,16.6643859282741));
#62010=CARTESIAN_POINT('Ctrl Pts',(53.2860839776272,30.865935952512,16.7910887586395));
#62011=CARTESIAN_POINT('Ctrl Pts',(52.501748585853,28.578141039759,16.917791589005));
#62012=CARTESIAN_POINT('Ctrl Pts',(53.9938158541446,26.6747433313176,17.0444944193704));
#62013=CARTESIAN_POINT('Ctrl Pts',(56.4027164936376,26.8901157498337,17.1711972497359));
#62014=CARTESIAN_POINT('Ctrl Pts',(57.5334641260503,29.0280112948501,17.2979000801013));
#62015=CARTESIAN_POINT('Ctrl Pts',(56.3557233320924,31.1403829931681,17.4246029104668));
#62016=CARTESIAN_POINT('Ctrl Pts',(53.9426496240763,31.3024411595428,17.5513057408322));
#62017=CARTESIAN_POINT('Ctrl Pts',(52.4930318735928,29.3665186540973,17.6780085711977));
#62018=CARTESIAN_POINT('Ctrl Pts',(53.3277594373305,27.0966249420605,17.8047114015631));
#62019=CARTESIAN_POINT('Ctrl Pts',(55.686229905235,26.5610835135692,17.9314142319286));
#62020=CARTESIAN_POINT('Ctrl Pts',(57.4194087900553,28.2478788546879,18.058117062294));
#62021=CARTESIAN_POINT('Ctrl Pts',(56.9480262867464,30.6200057705973,18.1848198926595));
#62022=CARTESIAN_POINT('Ctrl Pts',(54.7016053722045,31.5159860406461,18.3115227230249));
#62023=CARTESIAN_POINT('Ctrl Pts',(52.7270811613398,30.1194038875609,18.4382255533904));
#62024=CARTESIAN_POINT('Ctrl Pts',(52.8236369311127,27.7028227172024,18.5649283837558));
#62025=CARTESIAN_POINT('Ctrl Pts',(54.9032912198053,26.468227395192,18.6916312141213));
#62026=CARTESIAN_POINT('Ctrl Pts',(57.0710663930656,27.5405791881239,18.8183340444868));
#62027=CARTESIAN_POINT('Ctrl Pts',(57.3516892086208,29.9427528714775,18.9450368748522));
#62028=CARTESIAN_POINT('Ctrl Pts',(55.48945660945,31.4858916585581,19.0717397052177));
#62029=CARTESIAN_POINT('Ctrl Pts',(53.1812319370115,30.7638899749351,19.1984425355831));
#62030=CARTESIAN_POINT('Ctrl Pts',(52.5302657907506,28.4346345904763,19.3251453659486));
#62031=CARTESIAN_POINT('Ctrl Pts',(54.1297174734372,26.6205392555073,19.451848196314));
#62032=CARTESIAN_POINT('Ctrl Pts',(56.5221691909721,26.9746047139677,19.5785510266795));
#62033=CARTESIAN_POINT('Ctrl Pts',(57.5276227962348,29.1742070910521,19.7052538570449));
#62034=CARTESIAN_POINT('Ctrl Pts',(56.229910585439,31.2150722476805,19.8319566874103));
#62035=CARTESIAN_POINT('Ctrl Pts',(53.8115058324518,31.2375671440993,19.9586595177758));
#62036=CARTESIAN_POINT('Ctrl Pts',(52.4760550484659,29.2211944669454,20.0853623481413));
#62037=CARTESIAN_POINT('Ctrl Pts',(53.4404188343545,27.0032697482195,20.2120651785067));
#62038=CARTESIAN_POINT('Ctrl Pts',(55.8258704635605,26.6047624150779,20.3387680088722));
#62039=CARTESIAN_POINT('Ctrl Pts',(57.4587902580083,28.3887917070251,20.4654708392376));
#62040=CARTESIAN_POINT('Ctrl Pts',(56.8512643344329,30.7297530097437,20.5921736696031));
#62041=CARTESIAN_POINT('Ctrl Pts',(54.5568693341469,31.4945661596456,20.7188764999685));
#62042=CARTESIAN_POINT('Ctrl Pts',(52.6662542827978,29.9863346466896,20.845579330334));
#62043=CARTESIAN_POINT('Ctrl Pts',(52.9021445642136,27.5793565956363,20.9722821606994));
#62044=CARTESIAN_POINT('Ctrl Pts',(55.0495973388329,26.4668665209239,21.0989849910649));
#62045=CARTESIAN_POINT('Ctrl Pts',(57.1518570924653,27.6625635932472,21.2256878214303));
#62046=CARTESIAN_POINT('Ctrl Pts',(57.2933481447822,30.0769305516647,21.3523906517957));
#62047=CARTESIAN_POINT('Ctrl Pts',(55.3451440433139,31.5100001497084,21.4790934821613));
#62048=CARTESIAN_POINT('Ctrl Pts',(53.0824452899396,30.6559616162193,21.6057963125266));
#62049=CARTESIAN_POINT('Ctrl Pts',(52.5670192104037,28.293013611747,21.7324991428922));
#62050=CARTESIAN_POINT('Ctrl Pts',(54.268521471356,26.574270300707,21.8592019732576));
#62051=CARTESIAN_POINT('Ctrl Pts',(56.6365454583084,27.0658483005513,21.985904803623));
#62052=CARTESIAN_POINT('Ctrl Pts',(57.5133525089284,29.3198215820206,22.1126076339885));
#62053=CARTESIAN_POINT('Ctrl Pts',(56.0999955396154,31.282375184532,22.2393104643539));
#62054=CARTESIAN_POINT('Ctrl Pts',(53.6843268908365,31.1652297869952,22.3660132947194));
#62055=CARTESIAN_POINT('Ctrl Pts',(52.4674925923137,29.0751352268033,22.4927161250848));
#62056=CARTESIAN_POINT('Ctrl Pts',(53.5582844951136,26.916568303392,22.6194189554503));
#62057=CARTESIAN_POINT('Ctrl Pts',(55.9627465535904,26.6564391417817,22.7461217858157));
#62058=CARTESIAN_POINT('Ctrl Pts',(57.4899921297994,28.5317232652417,22.8728246161812));
#62059=CARTESIAN_POINT('Ctrl Pts',(56.7482891129976,30.8337701453811,22.9995274465467));
#62060=CARTESIAN_POINT('Ctrl Pts',(54.4136885536048,31.4647519228485,23.1262302769121));
#62061=CARTESIAN_POINT('Ctrl Pts',(52.6130583236143,29.8501236550651,23.2529331072776));
#62062=CARTESIAN_POINT('Ctrl Pts',(52.987945935458,27.4603388218333,23.379635937643));
#62063=CARTESIAN_POINT('Ctrl Pts',(55.1951539829876,26.4745218866781,23.5063387680084));
#62064=CARTESIAN_POINT('Ctrl Pts',(57.2266242981082,27.7878773360167,23.6330415983739));
#62065=CARTESIAN_POINT('Ctrl Pts',(57.2250123592762,30.2102470168422,23.7597618591261));
#62066=CARTESIAN_POINT('Ctrl Pts',(55.8779376927861,31.0829490139849,23.8442478430899));
#62067=CARTESIAN_POINT('Ctrl Pts',(55.1682015051339,31.138743146064,23.8864995502653));
#62068=CARTESIAN_POINT('Ctrl Pts',(53.9911581995026,31.0663838938146,4.84332060209571));
#62069=CARTESIAN_POINT('Ctrl Pts',(53.3057237132466,30.7317437704051,4.88555487888419));
#62070=CARTESIAN_POINT('Ctrl Pts',(52.3057458731769,29.332451268937,4.97002343246116));
#62071=CARTESIAN_POINT('Ctrl Pts',(53.2556893237274,26.9164216648475,5.09672626282661));
#62072=CARTESIAN_POINT('Ctrl Pts',(55.7975711244056,26.4047749826171,5.22342909319206));
#62073=CARTESIAN_POINT('Ctrl Pts',(57.6114280049078,28.2550399075399,5.35013192355752));
#62074=CARTESIAN_POINT('Ctrl Pts',(57.0464078792917,30.7855559938902,5.47683475392296));
#62075=CARTESIAN_POINT('Ctrl Pts',(54.6163716009993,31.6883401940828,5.60353758428842));
#62076=CARTESIAN_POINT('Ctrl Pts',(52.5360665973209,30.1418886630702,5.73024041465387));
#62077=CARTESIAN_POINT('Ctrl Pts',(52.700807151554,27.5547584266893,5.85694324501931));
#62078=CARTESIAN_POINT('Ctrl Pts',(54.9606127012548,26.2846277414455,5.98364607538478));
#62079=CARTESIAN_POINT('Ctrl Pts',(57.2562853518332,27.4886899983651,6.11034890575021));
#62080=CARTESIAN_POINT('Ctrl Pts',(57.4960459301408,30.0698809432301,6.23705173611568));
#62081=CARTESIAN_POINT('Ctrl Pts',(55.461407613052,31.6761851114186,6.36375456648113));
#62082=CARTESIAN_POINT('Ctrl Pts',(53.006338417493,30.8439603477291,6.49045739684658));
#62083=CARTESIAN_POINT('Ctrl Pts',(52.3678889131507,28.3315185076544,6.61716022721203));
#62084=CARTESIAN_POINT('Ctrl Pts',(54.1278155663995,26.4281976505747,6.74386305757748));
#62085=CARTESIAN_POINT('Ctrl Pts',(56.6824748713308,26.8682980669564,6.87056588794293));
#62086=CARTESIAN_POINT('Ctrl Pts',(57.7040659895162,29.2508022964232,6.99726871830839));
#62087=CARTESIAN_POINT('Ctrl Pts',(56.2617164348777,31.404775648651,7.12397154867383));
#62088=CARTESIAN_POINT('Ctrl Pts',(53.6696929521768,31.3675214245298,7.25067437903929));
#62089=CARTESIAN_POINT('Ctrl Pts',(52.2898430793299,29.1729854364138,7.37737720940473));
#62090=CARTESIAN_POINT('Ctrl Pts',(53.3794838361463,26.8208254280239,7.5040800397702));
#62091=CARTESIAN_POINT('Ctrl Pts',(55.9457363013156,26.4543257601017,7.63078287013563));
#62092=CARTESIAN_POINT('Ctrl Pts',(57.6502353773361,28.4074403625246,7.7574857005011));
#62093=CARTESIAN_POINT('Ctrl Pts',(56.9398442492839,30.900494347051,7.88418853086654));
#62094=CARTESIAN_POINT('Ctrl Pts',(54.4618701702737,31.6618209492118,8.01089136123201));
#62095=CARTESIAN_POINT('Ctrl Pts',(52.4742391238837,29.9977005936638,8.13759419159744));
#62096=CARTESIAN_POINT('Ctrl Pts',(52.7880773151889,27.4244770665284,8.2642970219629));
#62097=CARTESIAN_POINT('Ctrl Pts',(55.1174158899787,26.2868674955205,8.39099985232835));
#62098=CARTESIAN_POINT('Ctrl Pts',(57.3397652952198,27.621459887727,8.51770268269381));
#62099=CARTESIAN_POINT('Ctrl Pts',(57.4301243363657,30.2121758072282,8.64440551305926));
#62100=CARTESIAN_POINT('Ctrl Pts',(55.3061580008797,31.6983590858891,8.7711083434247));
#62101=CARTESIAN_POINT('Ctrl Pts',(52.9032209886726,30.7258019166539,8.89781117379017));
#62102=CARTESIAN_POINT('Ctrl Pts',(52.4108656304726,28.1806968238802,9.0245140041556));
#62103=CARTESIAN_POINT('Ctrl Pts',(54.2777253347274,26.3821394640313,9.15121683452108));
#62104=CARTESIAN_POINT('Ctrl Pts',(56.8027205492901,26.9689724031812,9.2779196648865));
#62105=CARTESIAN_POINT('Ctrl Pts',(57.68507970628,29.4064744134585,9.40462249525197));
#62106=CARTESIAN_POINT('Ctrl Pts',(56.1207985646789,31.4735975936453,9.53132532561742));
#62107=CARTESIAN_POINT('Ctrl Pts',(53.5352475782635,31.286782635252,9.65802815598287));
#62108=CARTESIAN_POINT('Ctrl Pts',(52.2843766365773,29.0162550271226,9.78473098634831));
#62109=CARTESIAN_POINT('Ctrl Pts',(53.5079773246182,26.7309158644907,9.91143381671377));
#62110=CARTESIAN_POINT('Ctrl Pts',(56.0911066685357,26.513162507169,10.0381366470792));
#62111=CARTESIAN_POINT('Ctrl Pts',(57.6800213755258,28.5614114632152,10.1648394774447));
#62112=CARTESIAN_POINT('Ctrl Pts',(56.8269049267509,31.0093015867427,10.2915423078101));
#62113=CARTESIAN_POINT('Ctrl Pts',(54.3091156546596,31.626319344489,10.4182451381756));
#62114=CARTESIAN_POINT('Ctrl Pts',(52.4208590839707,29.8502391505553,10.544947968541));
#62115=CARTESIAN_POINT('Ctrl Pts',(52.8827115570261,27.2994224136717,10.6716507989065));
#62116=CARTESIAN_POINT('Ctrl Pts',(55.2738338451284,26.2981692312182,10.7983536292719));
#62117=CARTESIAN_POINT('Ctrl Pts',(57.415439175115,27.758819888496,10.9250564596374));
#62118=CARTESIAN_POINT('Ctrl Pts',(57.3561002237046,30.3504318619362,11.0517592900028));
#62119=CARTESIAN_POINT('Ctrl Pts',(55.1498865477365,31.7115325003918,11.1784621203683));
#62120=CARTESIAN_POINT('Ctrl Pts',(52.8070964911674,30.6018890969175,11.3051649507338));
#62121=CARTESIAN_POINT('Ctrl Pts',(52.4624765757242,28.032606931426,11.4318677810992));
#62122=CARTESIAN_POINT('Ctrl Pts',(54.4300439126487,26.3448117700689,11.5585706114646));
#62123=CARTESIAN_POINT('Ctrl Pts',(56.9169543172966,27.0764198422547,11.6852734418301));
#62124=CARTESIAN_POINT('Ctrl Pts',(57.6571390391698,29.5607910523476,11.8119762721955));
#62125=CARTESIAN_POINT('Ctrl Pts',(55.9761429532675,31.5341703598337,11.938679102561));
#62126=CARTESIAN_POINT('Ctrl Pts',(53.4056869824076,31.1984177218646,12.0653819329264));
#62127=CARTESIAN_POINT('Ctrl Pts',(52.2879664623005,28.8594704007468,12.1920847632919));
#62128=CARTESIAN_POINT('Ctrl Pts',(53.6414465285101,26.6485734238602,12.3187875936574));
#62129=CARTESIAN_POINT('Ctrl Pts',(56.2328383272333,26.5802925514067,12.4454904240228));
#62130=CARTESIAN_POINT('Ctrl Pts',(57.7008698301702,28.7168452042609,12.5721932543883));
#62131=CARTESIAN_POINT('Ctrl Pts',(56.707873099089,31.111408050397,12.6988960847537));
#62132=CARTESIAN_POINT('Ctrl Pts',(54.1586651541145,31.5820592857199,12.8255989151192));
#62133=CARTESIAN_POINT('Ctrl Pts',(52.376080164033,29.6999422635425,12.9523017454846));
#62134=CARTESIAN_POINT('Ctrl Pts',(52.9844066973359,27.180038979503,13.0790045758501));
#62135=CARTESIAN_POINT('Ctrl Pts',(55.4293385978216,26.3184812425989,13.2057074062155));
#62136=CARTESIAN_POINT('Ctrl Pts',(57.4830578602938,27.9003190734096,13.332410236581));
#62137=CARTESIAN_POINT('Ctrl Pts',(57.2742188044711,30.4841843912612,13.4591130669464));
#62138=CARTESIAN_POINT('Ctrl Pts',(54.9931152412601,31.7156632850872,13.5858158973119));
#62139=CARTESIAN_POINT('Ctrl Pts',(52.718285059111,30.47263417263,13.7125187276773));
#62140=CARTESIAN_POINT('Ctrl Pts',(52.5225498517664,27.8877431767388,13.8392215580428));
#62141=CARTESIAN_POINT('Ctrl Pts',(54.5842632245302,26.316338804656,13.9659243884082));
#62142=CARTESIAN_POINT('Ctrl Pts',(57.0247952767137,27.1902821862869,14.0926272187737));
#62143=CARTESIAN_POINT('Ctrl Pts',(57.6203371377989,29.7132375215492,14.2193300491391));
#62144=CARTESIAN_POINT('Ctrl Pts',(55.8282320242933,31.5862919772926,14.3460328795046));
#62145=CARTESIAN_POINT('Ctrl Pts',(53.2814432258008,31.1027213538002,14.47273570987));
#62146=CARTESIAN_POINT('Ctrl Pts',(52.3006005887342,28.7031544234258,14.5994385402355));
#62147=CARTESIAN_POINT('Ctrl Pts',(53.7794463423511,26.5740727037537,14.7261413706009));
#62148=CARTESIAN_POINT('Ctrl Pts',(56.3704586206384,26.6554920245408,14.8528442009664));
#62149=CARTESIAN_POINT('Ctrl Pts',(57.7127112137053,28.8732232319774,14.9795470313318));
#62150=CARTESIAN_POINT('Ctrl Pts',(56.5831457231721,31.2064732260048,15.1062498616973));
#62151=CARTESIAN_POINT('Ctrl Pts',(54.0110204025537,31.5291883745005,15.2329526920627));
#62152=CARTESIAN_POINT('Ctrl Pts',(52.3400516963698,29.5473111545432,15.3596555224282));
#62153=CARTESIAN_POINT('Ctrl Pts',(53.0928235952072,27.0667248931217,15.4863583527936));
#62154=CARTESIAN_POINT('Ctrl Pts',(55.5834115587132,26.3477357916238,15.6130611831591));
#62155=CARTESIAN_POINT('Ctrl Pts',(57.5423958506882,28.0454855599432,15.7397640135245));
#62156=CARTESIAN_POINT('Ctrl Pts',(57.1847531432053,30.6129873468592,15.86646684389));
#62157=CARTESIAN_POINT('Ctrl Pts',(54.8363668946136,31.7107376643075,15.9931696742555));
#62158=CARTESIAN_POINT('Ctrl Pts',(52.6370828677864,30.3384681931841,16.1198725046209));
#62159=CARTESIAN_POINT('Ctrl Pts',(52.5908851215582,27.7465886627514,16.2465753349864));
#62160=CARTESIAN_POINT('Ctrl Pts',(54.7398689677963,26.2968155216564,16.3732781653518));
#62161=CARTESIAN_POINT('Ctrl Pts',(57.1258837911094,27.3101797182624,16.4999809957173));
#62162=CARTESIAN_POINT('Ctrl Pts',(57.5747967320147,29.8633054307021,16.6266838260827));
#62163=CARTESIAN_POINT('Ctrl Pts',(55.6775590426448,31.6297886267918,16.7533866564481));
#62164=CARTESIAN_POINT('Ctrl Pts',(53.1629306462013,31.0000126667616,16.8800894868136));
#62165=CARTESIAN_POINT('Ctrl Pts',(52.3222368826097,28.5478283898582,17.006792317179));
#62166=CARTESIAN_POINT('Ctrl Pts',(53.9215165536116,26.5076621549759,17.1334951475445));
#62167=CARTESIAN_POINT('Ctrl Pts',(56.5035086018754,26.7385101455104,17.2601979779099));
#62168=CARTESIAN_POINT('Ctrl Pts',(57.7155060365633,29.0300240447358,17.3869008082754));
#62169=CARTESIAN_POINT('Ctrl Pts',(56.4531387495689,31.2941800828128,17.5136036386409));
#62170=CARTESIAN_POINT('Ctrl Pts',(53.8666737771972,31.4678829288644,17.6403064690063));
#62171=CARTESIAN_POINT('Ctrl Pts',(52.3128938315209,29.39285482967,17.7670092993718));
#62172=CARTESIAN_POINT('Ctrl Pts',(53.2076006935238,26.9598580431702,17.8937121297372));
#62173=CARTESIAN_POINT('Ctrl Pts',(55.7355389132906,26.3858353179441,18.0204149601027));
#62174=CARTESIAN_POINT('Ctrl Pts',(57.5932552613452,28.1938352355886,18.1471177904681));
#62175=CARTESIAN_POINT('Ctrl Pts',(57.0880015969638,30.7364111866002,18.2738206208336));
#62176=CARTESIAN_POINT('Ctrl Pts',(54.6801642443937,31.6967720643965,18.400523451199));
#62177=CARTESIAN_POINT('Ctrl Pts',(52.5637607165875,30.1998385857402,18.5272262815645));
#62178=CARTESIAN_POINT('Ctrl Pts',(52.667254495318,27.609614122533,18.6539291119299));
#62179=CARTESIAN_POINT('Ctrl Pts',(54.8963422162931,26.2863070288349,18.7806319422954));
#62180=CARTESIAN_POINT('Ctrl Pts',(57.2198827426306,27.4357125945517,18.9073347726609));
#62181=CARTESIAN_POINT('Ctrl Pts',(57.5206696935102,30.0104943216526,19.0340376030263));
#62182=CARTESIAN_POINT('Ctrl Pts',(55.5246264843186,31.6645152523161,19.1607404333918));
#62183=CARTESIAN_POINT('Ctrl Pts',(53.0505444685914,30.8906341816795,19.2874432637572));
#62184=CARTESIAN_POINT('Ctrl Pts',(52.3528031895289,28.3940102934005,19.4141460941227));
#62185=CARTESIAN_POINT('Ctrl Pts',(54.0671833754831,26.4495632485988,19.5408489244881));
#62186=CARTESIAN_POINT('Ctrl Pts',(56.6315445655035,26.8290700590176,19.6675517548536));
#62187=CARTESIAN_POINT('Ctrl Pts',(57.7092449783493,29.1867247309721,19.794254585219));
#62188=CARTESIAN_POINT('Ctrl Pts',(56.3182857356656,31.3742361291603,19.9209574155844));
#62189=CARTESIAN_POINT('Ctrl Pts',(53.7261066564109,31.3983473949914,20.0476602459499));
#62190=CARTESIAN_POINT('Ctrl Pts',(52.2946971376583,29.2370883818991,20.1743630763153));
#62191=CARTESIAN_POINT('Ctrl Pts',(53.328355224661,26.8597948175601,20.3010659066808));
#62192=CARTESIAN_POINT('Ctrl Pts',(55.8852133354318,26.4326527642611,20.4277687370462));
#62193=CARTESIAN_POINT('Ctrl Pts',(57.6354664822799,28.3448733723503,20.5544715674117));
#62194=CARTESIAN_POINT('Ctrl Pts',(56.9842868204588,30.854044306933,20.6811743977772));
#62195=CARTESIAN_POINT('Ctrl Pts',(54.5250282071345,31.6738130591511,20.8078772281426));
#62196=CARTESIAN_POINT('Ctrl Pts',(52.4985631263916,30.0572076626689,20.9345800585081));
#62197=CARTESIAN_POINT('Ctrl Pts',(52.7514032896153,27.4772763503198,21.0612828888735));
#62198=CARTESIAN_POINT('Ctrl Pts',(55.0531611525946,26.2848483690293,21.1879857192389));
#62199=CARTESIAN_POINT('Ctrl Pts',(57.3064786528164,27.5664621816773,21.3146885496044));
#62200=CARTESIAN_POINT('Ctrl Pts',(57.4581365360819,30.1543133308796,21.4413913799699));
#62201=CARTESIAN_POINT('Ctrl Pts',(55.3699443475302,31.69035605763,21.5680942103353));
#62202=CARTESIAN_POINT('Ctrl Pts',(52.9446595130096,30.7749506373201,21.6947970407008));
#62203=CARTESIAN_POINT('Ctrl Pts',(52.3921975239131,28.242213147868,21.8214998710662));
#62204=CARTESIAN_POINT('Ctrl Pts',(54.2159611262207,26.3999696408687,21.9482027014317));
#62205=CARTESIAN_POINT('Ctrl Pts',(56.7541393325647,26.9268699479593,22.0749055317971));
#62206=CARTESIAN_POINT('Ctrl Pts',(57.6939493004178,29.3428023423225,22.2016083621626));
#62207=CARTESIAN_POINT('Ctrl Pts',(56.1790356521349,31.4463751144411,22.328311192528));
#62208=CARTESIAN_POINT('Ctrl Pts',(53.58978927969,31.3208122414973,22.4550140228935));
#62209=CARTESIAN_POINT('Ctrl Pts',(52.2855194267405,29.0805340639504,22.5817168532589));
#62210=CARTESIAN_POINT('Ctrl Pts',(53.4546901152972,26.7668634456938,22.7084196836244));
#62211=CARTESIAN_POINT('Ctrl Pts',(56.0319246485763,26.4880427190156,22.8351225139898));
#62212=CARTESIAN_POINT('Ctrl Pts',(57.6689103626689,28.4980752689794,22.9618253443553));
#62213=CARTESIAN_POINT('Ctrl Pts',(56.8739123207573,30.9655355875179,23.0885281747208));
#62214=CARTESIAN_POINT('Ctrl Pts',(54.371559180325,31.6418565221842,23.2152310050862));
#62215=CARTESIAN_POINT('Ctrl Pts',(52.4415447748001,29.9112092385352,23.3419338354517));
#62216=CARTESIAN_POINT('Ctrl Pts',(52.8433699131658,27.3497065616273,23.4686366658171));
#62217=CARTESIAN_POINT('Ctrl Pts',(55.209176760552,26.2930538106234,23.5953394961826));
#62218=CARTESIAN_POINT('Ctrl Pts',(57.386618251468,27.7007803358032,23.722042326548));
#62219=CARTESIAN_POINT('Ctrl Pts',(57.3848904868694,30.2972092425445,23.8487625873002));
#62220=CARTESIAN_POINT('Ctrl Pts',(55.9410218522429,31.2326191885525,23.933248571264));
#62221=CARTESIAN_POINT('Ctrl Pts',(55.1802876140434,31.2924224045949,23.9755002784394));
#62222=CARTESIAN_POINT('Ctrl Pts',(53.9235275309291,31.2049099979065,4.93232133026981));
#62223=CARTESIAN_POINT('Ctrl Pts',(53.1921429338175,30.847836292476,4.97455560705829));
#62224=CARTESIAN_POINT('Ctrl Pts',(52.1251286467557,29.3547381146796,5.05902416063525));
#62225=CARTESIAN_POINT('Ctrl Pts',(53.1387543422687,26.7767428809569,5.18572699100072));
#62226=CARTESIAN_POINT('Ctrl Pts',(55.8510386436457,26.2307964629548,5.31242982136615));
#62227=CARTESIAN_POINT('Ctrl Pts',(57.786492739355,28.2050993231106,5.43913265173162));
#62228=CARTESIAN_POINT('Ctrl Pts',(57.1835948326693,30.9052559761693,5.56583548209706));
#62229=CARTESIAN_POINT('Ctrl Pts',(54.5906539462635,31.8685609626798,5.69253831246252));
#62230=CARTESIAN_POINT('Ctrl Pts',(52.3708895960694,30.2184385182424,5.81924114282797));
#62231=CARTESIAN_POINT('Ctrl Pts',(52.5466740164649,27.4578724195821,5.94594397319342));
#62232=CARTESIAN_POINT('Ctrl Pts',(54.9579722581784,26.1025947991337,6.07264680355888));
#62233=CARTESIAN_POINT('Ctrl Pts',(57.4075420570585,27.3873749004164,6.19934963392432));
#62234=CARTESIAN_POINT('Ctrl Pts',(57.6633756888425,30.1416035497367,6.32605246428978));
#62235=CARTESIAN_POINT('Ctrl Pts',(55.4923394254929,31.855591028404,6.45275529465523));
#62236=CARTESIAN_POINT('Ctrl Pts',(52.8726874668012,30.9675756371415,6.57945812502068));
#62237=CARTESIAN_POINT('Ctrl Pts',(52.1914376276516,28.2867048904611,6.70616095538613));
#62238=CARTESIAN_POINT('Ctrl Pts',(54.0693461251703,26.2557893381471,6.83286378575158));
#62239=CARTESIAN_POINT('Ctrl Pts',(56.7952645082689,26.7253931765565,6.95956661611704));
#62240=CARTESIAN_POINT('Ctrl Pts',(57.8853409829267,29.2676155638537,7.08626944648249));
#62241=CARTESIAN_POINT('Ctrl Pts',(56.3462992961339,31.5659868363783,7.21297227684794));
#62242=CARTESIAN_POINT('Ctrl Pts',(53.5805119180366,31.5262351660934,7.33967510721339));
#62243=CARTESIAN_POINT('Ctrl Pts',(52.1081597624875,29.1845820224319,7.46637793757883));
#62244=CARTESIAN_POINT('Ctrl Pts',(53.2708477828606,26.6747380700575,7.5930807679443));
#62245=CARTESIAN_POINT('Ctrl Pts',(56.0091365076915,26.2836690221182,7.71978359830973));
#62246=CARTESIAN_POINT('Ctrl Pts',(57.8279016777983,28.3677163895168,7.84648642867521));
#62247=CARTESIAN_POINT('Ctrl Pts',(57.0698873972211,31.0278995588966,7.97318925904064));
#62248=CARTESIAN_POINT('Ctrl Pts',(54.4257950590463,31.84026392246,8.09989208940611));
#62249=CARTESIAN_POINT('Ctrl Pts',(52.3049173366382,30.0645843787649,8.22659491977155));
#62250=CARTESIAN_POINT('Ctrl Pts',(52.6397945914431,27.3188572663865,8.353297750137));
#62251=CARTESIAN_POINT('Ctrl Pts',(55.1252872084912,26.1049847016914,8.48000058050245));
#62252=CARTESIAN_POINT('Ctrl Pts',(57.496618323259,27.5290454086657,8.6067034108679));
#62253=CARTESIAN_POINT('Ctrl Pts',(57.5930348477102,30.2934375672296,8.73340624123336));
#62254=CARTESIAN_POINT('Ctrl Pts',(55.3266822002917,31.8792515002793,8.8601090715988));
#62255=CARTESIAN_POINT('Ctrl Pts',(52.7626572587432,30.8414961091338,8.98681190196427));
#62256=CARTESIAN_POINT('Ctrl Pts',(52.2372954152504,28.1257724328231,9.1135147323297));
#62257=CARTESIAN_POINT('Ctrl Pts',(54.2293055344357,26.2066435060008,9.24021756269518));
#62258=CARTESIAN_POINT('Ctrl Pts',(56.9235712078764,26.8328165121425,9.36692039306061));
#62259=CARTESIAN_POINT('Ctrl Pts',(57.8650818985156,29.4337236177705,9.49362322342607));
#62260=CARTESIAN_POINT('Ctrl Pts',(56.1959345832578,31.639422462279,9.6203260537915));
#62261=CARTESIAN_POINT('Ctrl Pts',(53.4370536042156,31.4400838153061,9.74702888415697));
#62262=CARTESIAN_POINT('Ctrl Pts',(52.1023268607143,29.0173447305344,9.87373171452243));
#62263=CARTESIAN_POINT('Ctrl Pts',(53.4079552091459,26.5788011552687,10.0004345448879));
#62264=CARTESIAN_POINT('Ctrl Pts',(56.1642522037837,26.3464500630666,10.1271373752533));
#62265=CARTESIAN_POINT('Ctrl Pts',(57.8596844677255,28.5320093944699,10.2538402056188));
#62266=CARTESIAN_POINT('Ctrl Pts',(56.9493768560022,31.1440010109833,10.3805430359842));
#62267=CARTESIAN_POINT('Ctrl Pts',(54.2628001965182,31.8023823635544,10.5072458663497));
#62268=CARTESIAN_POINT('Ctrl Pts',(52.24795880921,29.90723742538,10.6339486967151));
#62269=CARTESIAN_POINT('Ctrl Pts',(52.7407729172013,27.1854192081467,10.7606515270806));
#62270=CARTESIAN_POINT('Ctrl Pts',(55.2921910999675,26.1170440823845,10.887354357446));
#62271=CARTESIAN_POINT('Ctrl Pts',(57.5773652236103,27.675613739901,11.0140571878115));
#62272=CARTESIAN_POINT('Ctrl Pts',(57.5140483115778,30.4409620220074,11.1407600181769));
#62273=CARTESIAN_POINT('Ctrl Pts',(55.1599346320135,31.8933080332549,11.2674628485424));
#62274=CARTESIAN_POINT('Ctrl Pts',(52.660088773658,30.7092764301462,11.3941656789078));
#62275=CARTESIAN_POINT('Ctrl Pts',(52.2923662515686,27.9677549001475,11.5208685092733));
#62276=CARTESIAN_POINT('Ctrl Pts',(54.3918352349096,26.1668134406084,11.6475713396387));
#62277=CARTESIAN_POINT('Ctrl Pts',(57.0454629715172,26.9474670053891,11.7742741700042));
#62278=CARTESIAN_POINT('Ctrl Pts',(57.8352681468484,29.5983853250884,11.9009770003696));
#62279=CARTESIAN_POINT('Ctrl Pts',(56.0415815587258,31.7040559014815,12.0276798307351));
#62280=CARTESIAN_POINT('Ctrl Pts',(53.2988075338738,31.3457951008154,12.1543826611005));
#62281=CARTESIAN_POINT('Ctrl Pts',(52.1061573409321,28.8500495869511,12.281085491466));
#62282=CARTESIAN_POINT('Ctrl Pts',(53.5503719125255,26.4909386476573,12.4077883218315));
#62283=CARTESIAN_POINT('Ctrl Pts',(56.3154852598571,26.418080366682,12.5344911521969));
#62284=CARTESIAN_POINT('Ctrl Pts',(57.8819305596662,28.6978630921634,12.6611939825623));
#62285=CARTESIAN_POINT('Ctrl Pts',(56.8223653807064,31.2529524808608,12.7878968129278));
#62286=CARTESIAN_POINT('Ctrl Pts',(54.1022638054657,31.755155201951,12.9145996432933));
#62287=CARTESIAN_POINT('Ctrl Pts',(52.200178003058,29.7468649457934,13.0413024736587));
#62288=CARTESIAN_POINT('Ctrl Pts',(52.8492854894676,27.058032555371,13.1680053040242));
#62289=CARTESIAN_POINT('Ctrl Pts',(55.4581205697826,26.1387177690139,13.2947081343896));
#62290=CARTESIAN_POINT('Ctrl Pts',(57.6495169256451,27.8265987376286,13.4214109647551));
#62291=CARTESIAN_POINT('Ctrl Pts',(57.4266777312847,30.5836810443714,13.5481137951205));
#62292=CARTESIAN_POINT('Ctrl Pts',(54.9926537012681,31.8977157372161,13.674816625486));
#62293=CARTESIAN_POINT('Ctrl Pts',(52.5653236068099,30.5713565229626,13.8015194558514));
#62294=CARTESIAN_POINT('Ctrl Pts',(52.356466715838,27.8131797788449,13.9282222862168));
#62295=CARTESIAN_POINT('Ctrl Pts',(54.5563930906184,26.1364317064607,14.0549251165823));
#62296=CARTESIAN_POINT('Ctrl Pts',(57.1605333658978,27.0689624455601,14.1816279469477));
#62297=CARTESIAN_POINT('Ctrl Pts',(57.7959991220958,29.7610514904095,14.3083307773132));
#62298=CARTESIAN_POINT('Ctrl Pts',(55.8837549868721,31.7596716444159,14.4350336076787));
#62299=CARTESIAN_POINT('Ctrl Pts',(53.1662347326919,31.2436834460835,14.5617364380441));
#62300=CARTESIAN_POINT('Ctrl Pts',(52.1196384330817,28.6832545096864,14.6884392684096));
#62301=CARTESIAN_POINT('Ctrl Pts',(53.6976229485782,26.4114435533014,14.815142098775));
#62302=CARTESIAN_POINT('Ctrl Pts',(56.4623313332087,26.4983210570238,14.9418449291405));
#62303=CARTESIAN_POINT('Ctrl Pts',(57.894565765072,28.864724379554,15.0685477595059));
#62304=CARTESIAN_POINT('Ctrl Pts',(56.6892765393757,31.3543906292988,15.1952505898714));
#62305=CARTESIAN_POINT('Ctrl Pts',(53.9447212550088,31.6987399341516,15.3219534202368));
#62306=CARTESIAN_POINT('Ctrl Pts',(52.1617342614096,29.5840017628043,15.4486562506023));
#62307=CARTESIAN_POINT('Ctrl Pts',(52.9649704320257,26.9371221269099,15.5753590809677));
#62308=CARTESIAN_POINT('Ctrl Pts',(55.6225222634338,26.1699334825232,15.7020619113332));
#62309=CARTESIAN_POINT('Ctrl Pts',(57.712832812237,27.9814968852945,15.8287647416986));
#62310=CARTESIAN_POINT('Ctrl Pts',(57.3312144770535,30.7211186838188,15.9554675720641));
#62311=CARTESIAN_POINT('Ctrl Pts',(54.825397269532,31.8924599130027,16.0821704024296));
#62312=CARTESIAN_POINT('Ctrl Pts',(52.4786777884606,30.4281963336365,16.208873232795));
#62313=CARTESIAN_POINT('Ctrl Pts',(52.4293830408368,27.6625625580699,16.3355760631605));
#62314=CARTESIAN_POINT('Ctrl Pts',(54.7224303212057,26.1155996229323,16.4622788935259));
#62315=CARTESIAN_POINT('Ctrl Pts',(57.2683986453028,27.196897660197,16.5889817238913));
#62316=CARTESIAN_POINT('Ctrl Pts',(57.7474057816604,29.9211796419339,16.7156845542568));
#62317=CARTESIAN_POINT('Ctrl Pts',(55.7229812000429,31.8060842193703,16.8423873846222));
#62318=CARTESIAN_POINT('Ctrl Pts',(53.0397773147751,31.1340893810111,16.9690902149877));
#62319=CARTESIAN_POINT('Ctrl Pts',(52.1427251793666,28.5175157399575,17.0957930453531));
#62320=CARTESIAN_POINT('Ctrl Pts',(53.8492172530783,26.3405809786343,17.2224958757186));
#62321=CARTESIAN_POINT('Ctrl Pts',(56.6043007101135,26.586904541187,17.3491987060841));
#62322=CARTESIAN_POINT('Ctrl Pts',(57.8975479470761,29.0320367946217,17.4759015364495));
#62323=CARTESIAN_POINT('Ctrl Pts',(56.5505541670455,31.4479771724574,17.602604366815));
#62324=CARTESIAN_POINT('Ctrl Pts',(53.790697930318,31.6333246981861,17.7293071971804));
#62325=CARTESIAN_POINT('Ctrl Pts',(52.132755789449,29.4191910052424,17.8560100275459));
#62326=CARTESIAN_POINT('Ctrl Pts',(53.0874419497171,26.8230911442798,17.9827128579113));
#62327=CARTESIAN_POINT('Ctrl Pts',(55.7848479213462,26.2105871223189,18.1094156882768));
#62328=CARTESIAN_POINT('Ctrl Pts',(57.7671017326352,28.1397916164894,18.2361185186422));
#62329=CARTESIAN_POINT('Ctrl Pts',(57.2279769071813,30.8528166026031,18.3628213490077));
#62330=CARTESIAN_POINT('Ctrl Pts',(54.6587231165829,31.8775580881469,18.4895241793731));
#62331=CARTESIAN_POINT('Ctrl Pts',(52.4004402718352,30.2802732839195,18.6162270097386));
#62332=CARTESIAN_POINT('Ctrl Pts',(52.5108720595234,27.5164055278637,18.742929840104));
#62333=CARTESIAN_POINT('Ctrl Pts',(54.8893932127809,26.1043866624779,18.8696326704694));
#62334=CARTESIAN_POINT('Ctrl Pts',(57.3686990921956,27.3308460009795,18.996335500835));
#62335=CARTESIAN_POINT('Ctrl Pts',(57.6896501783996,30.0782357718278,19.1230383312003));
#62336=CARTESIAN_POINT('Ctrl Pts',(55.5597963591873,31.8431388460741,19.2497411615659));
#62337=CARTESIAN_POINT('Ctrl Pts',(52.9198570001715,31.0173783884239,19.3764439919313));
#62338=CARTESIAN_POINT('Ctrl Pts',(52.1753405883074,28.3533859963246,19.5031468222967));
#62339=CARTESIAN_POINT('Ctrl Pts',(54.004649277529,26.2785872416904,19.6298496526622));
#62340=CARTESIAN_POINT('Ctrl Pts',(56.7409199400349,26.6835354040676,19.7565524830276));
#62341=CARTESIAN_POINT('Ctrl Pts',(57.890867160464,29.199242370892,19.8832553133931));
#62342=CARTESIAN_POINT('Ctrl Pts',(56.4066608858923,31.53340001064,20.0099581437585));
#62343=CARTESIAN_POINT('Ctrl Pts',(53.6407074803699,31.5591276458837,20.136660974124));
#62344=CARTESIAN_POINT('Ctrl Pts',(52.1133392268507,29.2529822968528,20.2633638044895));
#62345=CARTESIAN_POINT('Ctrl Pts',(53.2162916149675,26.7163198869008,20.3900666348549));
#62346=CARTESIAN_POINT('Ctrl Pts',(55.944556207303,26.2605431134443,20.5167694652203));
#62347=CARTESIAN_POINT('Ctrl Pts',(57.8121427065516,28.3009550376753,20.6434722955858));
#62348=CARTESIAN_POINT('Ctrl Pts',(57.1173093064847,30.9783356041222,20.7701751259513));
#62349=CARTESIAN_POINT('Ctrl Pts',(54.4931870801222,31.8530599586564,20.8968779563167));
#62350=CARTESIAN_POINT('Ctrl Pts',(52.3308719699855,30.1280806786482,21.0235807866821));
#62351=CARTESIAN_POINT('Ctrl Pts',(52.6006620150167,27.3751961050032,21.1502836170476));
#62352=CARTESIAN_POINT('Ctrl Pts',(55.0567249663564,26.1028302171346,21.276986447413));
#62353=CARTESIAN_POINT('Ctrl Pts',(57.4611002131674,27.4703607701076,21.4036892777785));
#62354=CARTESIAN_POINT('Ctrl Pts',(57.6229249273816,30.2316961100944,21.5303921081439));
#62355=CARTESIAN_POINT('Ctrl Pts',(55.3947446517464,31.8707119655516,21.6570949385094));
#62356=CARTESIAN_POINT('Ctrl Pts',(52.8068737360795,30.8939396584208,21.7837977688749));
#62357=CARTESIAN_POINT('Ctrl Pts',(52.2173758374226,28.1914126839889,21.9105005992403));
#62358=CARTESIAN_POINT('Ctrl Pts',(54.1634007810851,26.2256689810304,22.0372034296058));
#62359=CARTESIAN_POINT('Ctrl Pts',(56.8717332068209,26.7878915953673,22.1639062599712));
#62360=CARTESIAN_POINT('Ctrl Pts',(57.874546091907,29.3657831026244,22.2906090903367));
#62361=CARTESIAN_POINT('Ctrl Pts',(56.2580757646544,31.6103750443502,22.4173119207021));
#62362=CARTESIAN_POINT('Ctrl Pts',(53.4952516685433,31.4763946959995,22.5440147510676));
#62363=CARTESIAN_POINT('Ctrl Pts',(52.1035462611674,29.0859329010972,22.6707175814331));
#62364=CARTESIAN_POINT('Ctrl Pts',(53.3510957354806,26.6171585879957,22.7974204117984));
#62365=CARTESIAN_POINT('Ctrl Pts',(56.1011027435622,26.3196462962494,22.924123242164));
#62366=CARTESIAN_POINT('Ctrl Pts',(57.847828595538,28.4644272727171,23.0508260725294));
#62367=CARTESIAN_POINT('Ctrl Pts',(56.9995355285173,31.0973010296546,23.1775289028948));
#62368=CARTESIAN_POINT('Ctrl Pts',(54.3294298070452,31.81896112152,23.3042317332603));
#62369=CARTESIAN_POINT('Ctrl Pts',(52.2700312259861,29.9722948220053,23.4309345636257));
#62370=CARTESIAN_POINT('Ctrl Pts',(52.6987938908735,27.2390743014212,23.5576373939912));
#62371=CARTESIAN_POINT('Ctrl Pts',(55.2231995381166,26.1115857345688,23.6843402243566));
#62372=CARTESIAN_POINT('Ctrl Pts',(57.5466122048277,27.6136833355897,23.8110430547221));
#62373=CARTESIAN_POINT('Ctrl Pts',(57.5447686144626,30.384171468247,23.9377633154743));
#62374=CARTESIAN_POINT('Ctrl Pts',(56.0041060116998,31.3822893631201,24.0222492994381));
#62375=CARTESIAN_POINT('Ctrl Pts',(55.192373722953,31.4461016631257,24.0645010066135));
#62376=CARTESIAN_POINT('Ctrl Pts',(57.0573849385052,27.6687909762881,23.7995));
#62377=CARTESIAN_POINT('Ctrl Pts',(57.065530420017,27.6816406375123,23.7995));
#62378=CARTESIAN_POINT('Ctrl Pts',(57.0736759015289,27.6944902987365,23.7995));
#62379=CARTESIAN_POINT('Ctrl Pts',(57.0818213830407,27.7073399599607,23.7995));
#62380=CARTESIAN_POINT('',(53.8384899895517,27.376374413452,4.92960110781498));
#62381=CARTESIAN_POINT('Ctrl Pts',(53.8371424194197,27.3753492875172,4.9305));
#62382=CARTESIAN_POINT('Ctrl Pts',(53.7923471686059,27.4001101047657,4.93049999999997));
#62383=CARTESIAN_POINT('Ctrl Pts',(53.7486565878578,27.4266536903292,4.9305));
#62384=CARTESIAN_POINT('Ctrl Pts',(53.7061911675431,27.4549560897793,4.9305));
#62385=CARTESIAN_POINT('Ctrl Pts',(53.6465096071238,27.4947327209836,4.9305));
#62386=CARTESIAN_POINT('Ctrl Pts',(53.5892465950656,27.5379810208987,4.9305));
#62387=CARTESIAN_POINT('Ctrl Pts',(53.5344833636967,27.5843580131219,4.9305));
#62388=CARTESIAN_POINT('Ctrl Pts',(53.5027210288969,27.6112563811908,4.93049999999999));
#62389=CARTESIAN_POINT('Ctrl Pts',(53.4717999231724,27.6392081762248,4.93049999999999));
#62390=CARTESIAN_POINT('Ctrl Pts',(53.441739198632,27.668153548885,4.93050000000001));
#62391=CARTESIAN_POINT('Ctrl Pts',(53.4320758759555,27.6774583304657,4.93050000000001));
#62392=CARTESIAN_POINT('Ctrl Pts',(53.422500525095,27.6868667842346,4.93049999999999));
#62393=CARTESIAN_POINT('Ctrl Pts',(53.4130168704631,27.6963739839462,4.9305));
#62394=CARTESIAN_POINT('Ctrl Pts',(53.3601668251658,27.7493552401086,4.93050000000002));
#62395=CARTESIAN_POINT('Ctrl Pts',(53.3102898631553,27.805270243235,4.93049999999999));
#62396=CARTESIAN_POINT('Ctrl Pts',(53.2634720446863,27.863741969491,4.93049999999999));
#62397=CARTESIAN_POINT('Ctrl Pts',(53.2239608869098,27.9130882585135,4.93049999999999));
#62398=CARTESIAN_POINT('Ctrl Pts',(53.1866286810685,27.9642566970573,4.93050000000001));
#62399=CARTESIAN_POINT('Ctrl Pts',(53.1515413985246,28.0170458610233,4.93049999999999));
#62400=CARTESIAN_POINT('Ctrl Pts',(53.1348137264051,28.042212809338,4.93049999999999));
#62401=CARTESIAN_POINT('Ctrl Pts',(53.1185965065014,28.0677484290916,4.93049999999998));
#62402=CARTESIAN_POINT('Ctrl Pts',(53.1028981687538,28.0936323966796,4.9305));
#62403=CARTESIAN_POINT('Ctrl Pts',(53.0952269344716,28.1062809957042,4.93050000000001));
#62404=CARTESIAN_POINT('Ctrl Pts',(53.0876783757228,28.1190149460074,4.93050000000001));
#62405=CARTESIAN_POINT('Ctrl Pts',(53.0802575695615,28.1318249982112,4.93050000000001));
#62406=CARTESIAN_POINT('Ctrl Pts',(53.0406280389758,28.20023486428,4.93050000000001));
#62407=CARTESIAN_POINT('Ctrl Pts',(53.0047367242393,28.2706403069767,4.93050000000001));
#62408=CARTESIAN_POINT('Ctrl Pts',(52.9726791564584,28.342639293023,4.9305));
#62409=CARTESIAN_POINT('Ctrl Pts',(52.9406215886776,28.4146382790693,4.93049999999999));
#62410=CARTESIAN_POINT('Ctrl Pts',(52.9123971908107,28.4882317069565,4.93049999999998));
#62411=CARTESIAN_POINT('Ctrl Pts',(52.8881358995463,28.5630593264738,4.93049999999998));
#62412=CARTESIAN_POINT('Ctrl Pts',(52.8639452198436,28.6376691630622,4.93049999999997));
#62413=CARTESIAN_POINT('Ctrl Pts',(52.8436940427735,28.7135069395457,4.9305));
#62414=CARTESIAN_POINT('Ctrl Pts',(52.8275539142239,28.7902434418759,4.93050000000001));
#62415=CARTESIAN_POINT('Ctrl Pts',(52.8220518507206,28.8164024100368,4.93050000000001));
#62416=CARTESIAN_POINT('Ctrl Pts',(52.8170279307067,28.842665994242,4.93050000000001));
#62417=CARTESIAN_POINT('Ctrl Pts',(52.8124902744209,28.8690215999907,4.93050000000001));
#62418=CARTESIAN_POINT('Ctrl Pts',(52.8102866450664,28.8818207153985,4.93050000000001));
#62419=CARTESIAN_POINT('Ctrl Pts',(52.8081977059568,28.8946415354413,4.9305));
#62420=CARTESIAN_POINT('Ctrl Pts',(52.8062244495756,28.9074826291637,4.93049999999999));
#62421=CARTESIAN_POINT('Ctrl Pts',(52.8041389781676,28.9210539694416,4.93049999999998));
#62422=CARTESIAN_POINT('Ctrl Pts',(52.8021840453567,28.9346396035822,4.93049999999998));
#62423=CARTESIAN_POINT('Ctrl Pts',(52.8003611168859,28.948231453112,4.93049999999998));
#62424=CARTESIAN_POINT('Ctrl Pts',(52.7895931013731,29.0285183370621,4.93049999999999));
#62425=CARTESIAN_POINT('Ctrl Pts',(52.7834170296039,29.1090878588739,4.9305));
#62426=CARTESIAN_POINT('Ctrl Pts',(52.7819626910031,29.1895648886972,4.9305));
#62427=CARTESIAN_POINT('Ctrl Pts',(52.7814701883797,29.2168179288706,4.9305));
#62428=CARTESIAN_POINT('Ctrl Pts',(52.7815195434031,29.2440606003883,4.93050000000001));
#62429=CARTESIAN_POINT('Ctrl Pts',(52.7821169991807,29.2712789634107,4.9305));
#62430=CARTESIAN_POINT('Ctrl Pts',(52.7838212494952,29.3489196951292,4.93049999999997));
#62431=CARTESIAN_POINT('Ctrl Pts',(52.7899813526817,29.4263621040423,4.93049999999998));
#62432=CARTESIAN_POINT('Ctrl Pts',(52.8003647568699,29.5033553971092,4.9305));
#62433=CARTESIAN_POINT('Ctrl Pts',(52.8109627235699,29.5819396784545,4.93050000000002));
#62434=CARTESIAN_POINT('Ctrl Pts',(52.8259604552607,29.6600568668912,4.93049999999998));
#62435=CARTESIAN_POINT('Ctrl Pts',(52.8451645866725,29.7374421551003,4.93049999999999));
#62436=CARTESIAN_POINT('Ctrl Pts',(52.8497696158219,29.7559986573601,4.93049999999999));
#62437=CARTESIAN_POINT('Ctrl Pts',(52.8546186499929,29.7745194397526,4.93049999999997));
#62438=CARTESIAN_POINT('Ctrl Pts',(52.8596995461917,29.792966320632,4.93049999999997));
#62439=CARTESIAN_POINT('Ctrl Pts',(52.8810906976902,29.8706297894632,4.93049999999997));
#62440=CARTESIAN_POINT('Ctrl Pts',(52.9066063850458,29.9470718181813,4.93050000000001));
#62441=CARTESIAN_POINT('Ctrl Pts',(52.9359741374881,30.0220262297436,4.93049999999999));
#62442=CARTESIAN_POINT('Ctrl Pts',(52.9662538136702,30.0993081162269,4.93049999999998));
#62443=CARTESIAN_POINT('Ctrl Pts',(53.0006285871345,30.1750093988147,4.93049999999999));
#62444=CARTESIAN_POINT('Ctrl Pts',(53.0388562578731,30.2488401603755,4.93049999999998));
#62445=CARTESIAN_POINT('Ctrl Pts',(53.0770839286116,30.3226709219363,4.93049999999997));
#62446=CARTESIAN_POINT('Ctrl Pts',(53.119164888844,30.3946320658828,4.93050000000001));
#62447=CARTESIAN_POINT('Ctrl Pts',(53.1649084323202,30.4644222759714,4.93050000000002));
#62448=CARTESIAN_POINT('Ctrl Pts',(53.1843231359478,30.4940429861746,4.93050000000002));
#62449=CARTESIAN_POINT('Ctrl Pts',(53.2043982041861,30.5232724122283,4.9305));
#62450=CARTESIAN_POINT('Ctrl Pts',(53.2251215945603,30.55208627748,4.9305));
#62451=CARTESIAN_POINT('Ctrl Pts',(53.2367479306124,30.5682515706257,4.93049999999999));
#62452=CARTESIAN_POINT('Ctrl Pts',(53.2485813425571,30.584289696419,4.93049999999999));
#62453=CARTESIAN_POINT('Ctrl Pts',(53.2605971587666,30.6001671053542,4.93049999999999));
#62454=CARTESIAN_POINT('Ctrl Pts',(53.3124157578432,30.6686389489339,4.9305));
#62455=CARTESIAN_POINT('Ctrl Pts',(53.3676995807456,30.734233482485,4.93049999999999));
#62456=CARTESIAN_POINT('Ctrl Pts',(53.4261926153321,30.796654168762,4.93049999999999));
#62457=CARTESIAN_POINT('Ctrl Pts',(53.4847629333864,30.8591573278859,4.93049999999999));
#62458=CARTESIAN_POINT('Ctrl Pts',(53.546551385425,30.9184791823246,4.93049999999999));
#62459=CARTESIAN_POINT('Ctrl Pts',(53.6113499889526,30.9743043144675,4.9305));
#62460=CARTESIAN_POINT('Ctrl Pts',(53.6747669431677,31.0289391315226,4.93050000000001));
#62461=CARTESIAN_POINT('Ctrl Pts',(53.7410676106959,31.080225534543,4.93049999999999));
#62462=CARTESIAN_POINT('Ctrl Pts',(53.8100963515205,31.1278383728564,4.93049999999999));
#62463=CARTESIAN_POINT('Ctrl Pts',(53.8475703604045,31.1536862139821,4.93049999999998));
#62464=CARTESIAN_POINT('Ctrl Pts',(53.8858490074175,31.1784508229889,4.93049999999998));
#62465=CARTESIAN_POINT('Ctrl Pts',(53.9249115396487,31.2020751695661,4.9305));
#62466=CARTESIAN_POINT('Ctrl Pts',(53.8393993796462,27.3776456112999,4.92960110781498));
#62467=CARTESIAN_POINT('Ctrl Pts',(53.8466111964845,27.3724864184906,4.92990073854331));
#62468=CARTESIAN_POINT('Ctrl Pts',(53.853857414901,27.3673753141965,4.93020036927164));
#62469=CARTESIAN_POINT('Ctrl Pts',(53.8611373905627,27.3623127528964,4.93049999999996));
#62470=CARTESIAN_POINT('Origin',(55.,29.,4.9305));
#62471=CARTESIAN_POINT('',(52.5495,29.,4.9305));
#62472=CARTESIAN_POINT('Origin',(55.,29.,4.9305));
#62473=CARTESIAN_POINT('',(56.1167974000718,31.181218424916,4.9305));
#62474=CARTESIAN_POINT('Origin',(55.,29.,4.9305));
#62475=CARTESIAN_POINT('Ctrl Pts',(56.1167974000718,31.181218424916,4.9305));
#62476=CARTESIAN_POINT('Ctrl Pts',(56.156542077517,31.1563402429025,4.93049999999999));
#62477=CARTESIAN_POINT('Ctrl Pts',(56.1954769538157,31.1302582487305,4.93049999999999));
#62478=CARTESIAN_POINT('Ctrl Pts',(56.2335395857427,31.1029688213438,4.93049999999999));
#62479=CARTESIAN_POINT('Ctrl Pts',(56.3028413187012,31.0532821729542,4.9305));
#62480=CARTESIAN_POINT('Ctrl Pts',(56.3692540097722,30.9995944471324,4.9305));
#62481=CARTESIAN_POINT('Ctrl Pts',(56.4326084716472,30.9422671449757,4.9305));
#62482=CARTESIAN_POINT('Ctrl Pts',(56.4644952752616,30.9134138586953,4.9305));
#62483=CARTESIAN_POINT('Ctrl Pts',(56.4956067164715,30.8836380847701,4.93049999999998));
#62484=CARTESIAN_POINT('Ctrl Pts',(56.5259169844523,30.8529834405448,4.93049999999998));
#62485=CARTESIAN_POINT('Ctrl Pts',(56.5406079272072,30.8381255836702,4.93049999999998));
#62486=CARTESIAN_POINT('Ctrl Pts',(56.5551106138877,30.8230612430467,4.9305));
#62487=CARTESIAN_POINT('Ctrl Pts',(56.569421847319,30.8077952915011,4.93050000000001));
#62488=CARTESIAN_POINT('Ctrl Pts',(56.5804379355535,30.7960443079108,4.93050000000001));
#62489=CARTESIAN_POINT('Ctrl Pts',(56.5913347634252,30.7841800385731,4.93050000000001));
#62490=CARTESIAN_POINT('Ctrl Pts',(56.6021089968716,30.7722075680246,4.9305));
#62491=CARTESIAN_POINT('Ctrl Pts',(56.6589136001418,30.7090855424019,4.93049999999999));
#62492=CARTESIAN_POINT('Ctrl Pts',(56.7123354273433,30.6429353418224,4.93049999999999));
#62493=CARTESIAN_POINT('Ctrl Pts',(56.7622061712803,30.5741150402067,4.9305));
#62494=CARTESIAN_POINT('Ctrl Pts',(56.8007927973022,30.5208665215059,4.9305));
#62495=CARTESIAN_POINT('Ctrl Pts',(56.8372527063867,30.4660187139076,4.93049999999998));
#62496=CARTESIAN_POINT('Ctrl Pts',(56.8714879584134,30.4097297951466,4.93049999999998));
#62497=CARTESIAN_POINT('Ctrl Pts',(56.88841288161,30.3819021738949,4.93049999999997));
#62498=CARTESIAN_POINT('Ctrl Pts',(56.9047938120668,30.3537222699618,4.9305));
#62499=CARTESIAN_POINT('Ctrl Pts',(56.9206172107038,30.3252089451577,4.9305));
#62500=CARTESIAN_POINT('Ctrl Pts',(56.9301861753971,30.3079659365857,4.9305));
#62501=CARTESIAN_POINT('Ctrl Pts',(56.9395535970338,30.2905961984367,4.93050000000001));
#62502=CARTESIAN_POINT('Ctrl Pts',(56.948701992001,30.2731319608337,4.93050000000001));
#62503=CARTESIAN_POINT('Ctrl Pts',(56.9872728773672,30.1995003446863,4.93050000000001));
#62504=CARTESIAN_POINT('Ctrl Pts',(57.0220010953548,30.1241106605415,4.93050000000001));
#62505=CARTESIAN_POINT('Ctrl Pts',(57.0527290708383,30.0472951628104,4.93050000000001));
#62506=CARTESIAN_POINT('Ctrl Pts',(57.0828377959204,29.9720277015854,4.9305));
#62507=CARTESIAN_POINT('Ctrl Pts',(57.1091060242923,29.8953903735951,4.93049999999997));
#62508=CARTESIAN_POINT('Ctrl Pts',(57.1313374504974,29.8176867055421,4.93049999999999));
#62509=CARTESIAN_POINT('Ctrl Pts',(57.1531068495254,29.7415979229254,4.9305));
#62510=CARTESIAN_POINT('Ctrl Pts',(57.1710055955889,29.6644858782793,4.93050000000001));
#62511=CARTESIAN_POINT('Ctrl Pts',(57.1848010612909,29.5866393720501,4.93050000000001));
#62512=CARTESIAN_POINT('Ctrl Pts',(57.1899692544381,29.5574757476596,4.93050000000001));
#62513=CARTESIAN_POINT('Ctrl Pts',(57.1945610611568,29.5282091413259,4.93050000000002));
#62514=CARTESIAN_POINT('Ctrl Pts',(57.1985624054365,29.4988552147064,4.9305));
#62515=CARTESIAN_POINT('Ctrl Pts',(57.2002889244207,29.4861894433988,4.93049999999999));
#62516=CARTESIAN_POINT('Ctrl Pts',(57.2019054985971,29.4735074191975,4.93049999999999));
#62517=CARTESIAN_POINT('Ctrl Pts',(57.2034109371338,29.4608104216605,4.93049999999999));
#62518=CARTESIAN_POINT('Ctrl Pts',(57.2050605906204,29.4468971028871,4.93049999999999));
#62519=CARTESIAN_POINT('Ctrl Pts',(57.206575805631,29.4329737711374,4.93050000000001));
#62520=CARTESIAN_POINT('Ctrl Pts',(57.2079548720302,29.4190491854131,4.93050000000001));
#62521=CARTESIAN_POINT('Ctrl Pts',(57.2156500436978,29.3413501873025,4.93050000000002));
#62522=CARTESIAN_POINT('Ctrl Pts',(57.2191185329822,29.2635419889306,4.93049999999998));
#62523=CARTESIAN_POINT('Ctrl Pts',(57.2181822895949,29.1859045445621,4.93049999999998));
#62524=CARTESIAN_POINT('Ctrl Pts',(57.2178350531444,29.1571101616343,4.93049999999998));
#62525=CARTESIAN_POINT('Ctrl Pts',(57.2168814224251,29.1283393057487,4.93050000000001));
#62526=CARTESIAN_POINT('Ctrl Pts',(57.2153104878672,29.0996065241017,4.9305));
#62527=CARTESIAN_POINT('Ctrl Pts',(57.2109695624812,29.0202099250287,4.93049999999998));
#62528=CARTESIAN_POINT('Ctrl Pts',(57.2019185379677,28.9411024317745,4.93050000000001));
#62529=CARTESIAN_POINT('Ctrl Pts',(57.1883457297054,28.8626076791341,4.93049999999999));
#62530=CARTESIAN_POINT('Ctrl Pts',(57.1752101981451,28.7866418008357,4.93049999999998));
#62531=CARTESIAN_POINT('Ctrl Pts',(57.15783874972,28.7112491714072,4.9305));
#62532=CARTESIAN_POINT('Ctrl Pts',(57.136363509946,28.6367490856546,4.93050000000001));
#62533=CARTESIAN_POINT('Ctrl Pts',(57.1318688602108,28.621156626887,4.93050000000001));
#62534=CARTESIAN_POINT('Ctrl Pts',(57.1271930748425,28.6055997454899,4.93049999999999));
#62535=CARTESIAN_POINT('Ctrl Pts',(57.122345532269,28.5901070630992,4.9305));
#62536=CARTESIAN_POINT('Ctrl Pts',(57.0991415837965,28.5159475485739,4.9305));
#62537=CARTESIAN_POINT('Ctrl Pts',(57.0719758581837,28.4431451575644,4.93050000000001));
#62538=CARTESIAN_POINT('Ctrl Pts',(57.0410525219349,28.3719899830229,4.93050000000001));
#62539=CARTESIAN_POINT('Ctrl Pts',(57.010229889292,28.3010665293603,4.93050000000002));
#62540=CARTESIAN_POINT('Ctrl Pts',(56.9756733982571,28.2317787781305,4.93050000000002));
#62541=CARTESIAN_POINT('Ctrl Pts',(56.9375430523185,28.1644427906323,4.9305));
#62542=CARTESIAN_POINT('Ctrl Pts',(56.8997300162386,28.0976671540083,4.93049999999999));
#62543=CARTESIAN_POINT('Ctrl Pts',(56.8584017016581,28.0328102169304,4.9305));
#62544=CARTESIAN_POINT('Ctrl Pts',(56.8136826037627,27.9702198192552,4.93050000000001));
#62545=CARTESIAN_POINT('Ctrl Pts',(56.7965878517277,27.9462934124539,4.93050000000001));
#62546=CARTESIAN_POINT('Ctrl Pts',(56.7789973254977,27.9226986854038,4.93050000000004));
#62547=CARTESIAN_POINT('Ctrl Pts',(56.7609170509524,27.8994569494047,4.93050000000003));
#62548=CARTESIAN_POINT('Ctrl Pts',(56.7532986544245,27.889663693202,4.93050000000002));
#62549=CARTESIAN_POINT('Ctrl Pts',(56.745593119741,27.8799330323037,4.93050000000001));
#62550=CARTESIAN_POINT('Ctrl Pts',(56.7378102773488,27.8702778958364,4.93050000000001));
#62551=CARTESIAN_POINT('Ctrl Pts',(56.6906550139252,27.8117786380373,4.93050000000002));
#62552=CARTESIAN_POINT('Ctrl Pts',(56.6405828747768,27.7559424449364,4.93050000000003));
#62553=CARTESIAN_POINT('Ctrl Pts',(56.5877479254413,27.703056258697,4.93050000000003));
#62554=CARTESIAN_POINT('Ctrl Pts',(56.5363848379517,27.6516433616474,4.93050000000003));
#62555=CARTESIAN_POINT('Ctrl Pts',(56.4824100357581,27.6030179442244,4.93050000000002));
#62556=CARTESIAN_POINT('Ctrl Pts',(56.4259391803423,27.5574841144824,4.93050000000001));
#62557=CARTESIAN_POINT('Ctrl Pts',(56.3702590108002,27.5125878340689,4.93050000000001));
#62558=CARTESIAN_POINT('Ctrl Pts',(56.3121516549929,27.4706967082956,4.93050000000002));
#62559=CARTESIAN_POINT('Ctrl Pts',(56.2517113699718,27.432149026189,4.93050000000001));
#62560=CARTESIAN_POINT('Ctrl Pts',(56.2218244016619,27.4130876774026,4.9305));
#62561=CARTESIAN_POINT('Ctrl Pts',(56.1913667829791,27.3948446290381,4.9305));
#62562=CARTESIAN_POINT('Ctrl Pts',(56.1603489846691,27.3774656255483,4.9305));
#62563=CARTESIAN_POINT('Ctrl Pts',(56.426474702112,27.0036056037862,4.66549903655386));
#62564=CARTESIAN_POINT('Ctrl Pts',(57.0889864356691,27.4769547815182,4.70775074246383));
#62565=CARTESIAN_POINT('Ctrl Pts',(57.8940851946881,29.1267095489036,4.79223672516228));
#62566=CARTESIAN_POINT('Ctrl Pts',(56.4666838667935,31.5011894340363,4.91895698464923));
#62567=CARTESIAN_POINT('Ctrl Pts',(53.7014160468368,31.5896772934095,5.04565981501467));
#62568=CARTESIAN_POINT('Ctrl Pts',(52.1202558948328,29.321686656546,5.17236264538012));
#62569=CARTESIAN_POINT('Ctrl Pts',(53.1626841165763,26.7589385357385,5.29906547574558));
#62570=CARTESIAN_POINT('Ctrl Pts',(55.8794910541278,26.2390763871994,5.42576830611103));
#62571=CARTESIAN_POINT('Ctrl Pts',(57.7947951629564,28.2345376750715,5.55247113647648));
#62572=CARTESIAN_POINT('Ctrl Pts',(57.1635435827332,30.9277042403169,5.67917396684193));
#62573=CARTESIAN_POINT('Ctrl Pts',(54.5608454099514,31.8642389468711,5.80587679720738));
#62574=CARTESIAN_POINT('Ctrl Pts',(52.3583190771025,30.1909403202993,5.93257962757283));
#62575=CARTESIAN_POINT('Ctrl Pts',(52.5628805448572,27.4324299216987,6.05928245793829));
#62576=CARTESIAN_POINT('Ctrl Pts',(54.9881452069412,26.1023015851809,6.18598528830373));
#62577=CARTESIAN_POINT('Ctrl Pts',(57.4242099589407,27.4125438522027,6.31268811866919));
#62578=CARTESIAN_POINT('Ctrl Pts',(57.6513395150985,30.1692774386449,6.43939094903464));
#62579=CARTESIAN_POINT('Ctrl Pts',(55.4625722652183,31.8605653501733,6.5660937794001));
#62580=CARTESIAN_POINT('Ctrl Pts',(52.8523101761262,30.9453117267534,6.69279660976554));
#62581=CARTESIAN_POINT('Ctrl Pts',(52.1990194571466,28.2574926847764,6.81949944013099));
#62582=CARTESIAN_POINT('Ctrl Pts',(54.0979777606297,26.2462453713895,6.94620227049645));
#62583=CARTESIAN_POINT('Ctrl Pts',(56.8188572391422,26.744214702256,7.0729051008619));
#62584=CARTESIAN_POINT('Ctrl Pts',(57.8823969521443,29.2976520266901,7.19960793122735));
#62585=CARTESIAN_POINT('Ctrl Pts',(56.3195012012023,31.5798692697846,7.3263107615928));
#62586=CARTESIAN_POINT('Ctrl Pts',(53.5542780881045,31.5113138120211,7.45301359195826));
#62587=CARTESIAN_POINT('Ctrl Pts',(52.1063944474859,29.1544532493034,7.57971642232369));
#62588=CARTESIAN_POINT('Ctrl Pts',(53.2951595215023,26.6568551394786,7.70641925268916));
#62589=CARTESIAN_POINT('Ctrl Pts',(56.0373724898025,26.2943268458236,7.8331220830546));
#62590=CARTESIAN_POINT('Ctrl Pts',(57.8343333185037,28.3972035684727,7.95982491342006));
#62591=CARTESIAN_POINT('Ctrl Pts',(57.0486541976706,31.0493474268912,8.0865277437855));
#62592=CARTESIAN_POINT('Ctrl Pts',(54.3962446755182,31.8341292148724,8.21323057415097));
#62593=CARTESIAN_POINT('Ctrl Pts',(52.2939760314182,30.0364570322204,8.33993340451641));
#62594=CARTESIAN_POINT('Ctrl Pts',(52.6574320639669,27.2943668732086,8.46663623488187));
#62595=CARTESIAN_POINT('Ctrl Pts',(55.1554322223572,26.1064468689031,8.59333906524731));
#62596=CARTESIAN_POINT('Ctrl Pts',(57.5118027903804,27.5551278117337,8.72004189561275));
#62597=CARTESIAN_POINT('Ctrl Pts',(57.5794227061629,30.320373962602,8.84674472597822));
#62598=CARTESIAN_POINT('Ctrl Pts',(55.2966768114875,31.8824974878954,8.97344755634366));
#62599=CARTESIAN_POINT('Ctrl Pts',(52.743599484584,30.818093950329,9.10015038670912));
#62600=CARTESIAN_POINT('Ctrl Pts',(52.2465506688147,28.0970461369549,9.22685321707458));
#62601=CARTESIAN_POINT('Ctrl Pts',(54.258440443602,26.1987684275468,9.35355604744002));
#62602=CARTESIAN_POINT('Ctrl Pts',(56.9460380903923,26.8529684098888,9.48025887780547));
#62603=CARTESIAN_POINT('Ctrl Pts',(57.8604089672616,29.4635401149875,9.60696170817093));
#62604=CARTESIAN_POINT('Ctrl Pts',(56.1683798056569,31.6517348147818,9.73366453853637));
#62605=CARTESIAN_POINT('Ctrl Pts',(53.411724849185,31.4236730273486,9.86036736890182));
#62606=CARTESIAN_POINT('Ctrl Pts',(52.1023036489946,28.9871642856403,9.9870701992673));
#62607=CARTESIAN_POINT('Ctrl Pts',(53.4332586912184,26.5623514261588,10.1137730296327));
#62608=CARTESIAN_POINT('Ctrl Pts',(56.1918258875868,26.3587200163801,10.2404758599982));
#62609=CARTESIAN_POINT('Ctrl Pts',(57.864403257041,28.5618186685331,10.3671786903636));
#62610=CARTESIAN_POINT('Ctrl Pts',(56.9269409976151,31.1641874433383,10.4938815207291));
#62611=CARTESIAN_POINT('Ctrl Pts',(54.2336532084122,31.7945521095904,10.6205843510945));
#62612=CARTESIAN_POINT('Ctrl Pts',(52.238659379947,29.8785253998825,10.74728718146));
#62613=CARTESIAN_POINT('Ctrl Pts',(52.7597946717299,27.16198776245,10.8739900118254));
#62614=CARTESIAN_POINT('Ctrl Pts',(55.3222014462345,26.1202439120236,11.0006928421909));
#62615=CARTESIAN_POINT('Ctrl Pts',(57.5910187824897,27.7025291652685,11.1273956725564));
#62616=CARTESIAN_POINT('Ctrl Pts',(57.4989039822355,30.4670677509103,11.2540985029218));
#62617=CARTESIAN_POINT('Ctrl Pts',(55.1297919029255,31.8948165676132,11.3808013332873));
#62618=CARTESIAN_POINT('Ctrl Pts',(52.6424136509631,30.6848131958851,11.5075041636527));
#62619=CARTESIAN_POINT('Ctrl Pts',(52.3032642785649,27.9396107568781,11.6342069940182));
#62620=CARTESIAN_POINT('Ctrl Pts',(54.4213761469714,26.1606332862943,11.7609098243836));
#62621=CARTESIAN_POINT('Ctrl Pts',(57.0667291372093,26.9688821866757,11.887612654749));
#62622=CARTESIAN_POINT('Ctrl Pts',(57.8288818702845,29.62788236332,12.0143154851145));
#62623=CARTESIAN_POINT('Ctrl Pts',(56.013362004813,31.7147571429862,12.14101831548));
#62624=CARTESIAN_POINT('Ctrl Pts',(53.2744683146323,31.3279495915903,12.2677211458454));
#62625=CARTESIAN_POINT('Ctrl Pts',(52.1078763136874,28.8199181262256,12.3944239762109));
#62626=CARTESIAN_POINT('Ctrl Pts',(53.5765827520745,26.4759769738567,12.5211268065763));
#62627=CARTESIAN_POINT('Ctrl Pts',(56.3423046914688,26.4319215328472,12.6478296369418));
#62628=CARTESIAN_POINT('Ctrl Pts',(57.8849207605029,28.7278950500041,12.7745324673072));
#62629=CARTESIAN_POINT('Ctrl Pts',(56.7988016845878,31.27181015882,12.9012352976727));
#62630=CARTESIAN_POINT('Ctrl Pts',(54.0736174142975,31.7456555142808,13.0279381280381));
#62631=CARTESIAN_POINT('Ctrl Pts',(52.19255146228,29.7176639925804,13.1546409584036));
#62632=CARTESIAN_POINT('Ctrl Pts',(52.8696280907382,27.0357381980954,13.281343788769));
#62633=CARTESIAN_POINT('Ctrl Pts',(55.4878961676276,26.1436445900751,13.4080466191345));
#62634=CARTESIAN_POINT('Ctrl Pts',(57.6615940433218,27.8542574256199,13.5347494494999));
#62635=CARTESIAN_POINT('Ctrl Pts',(57.410051718641,30.6088690473959,13.6614522798654));
#62636=CARTESIAN_POINT('Ctrl Pts',(54.9624741542151,31.897481787534,13.7881551102308));
#62637=CARTESIAN_POINT('Ctrl Pts',(52.5490900799565,30.5459137951471,13.9148579405963));
#62638=CARTESIAN_POINT('Ctrl Pts',(52.3689711726764,27.7857116454543,14.0415607709617));
#62639=CARTESIAN_POINT('Ctrl Pts',(54.586241490241,26.1319670863473,14.1682636013272));
#62640=CARTESIAN_POINT('Ctrl Pts',(57.1805278946999,27.0915694933719,14.2949664316926));
#62641=CARTESIAN_POINT('Ctrl Pts',(57.7879207976748,29.790130700635,14.4216692620581));
#62642=CARTESIAN_POINT('Ctrl Pts',(55.8549647654138,31.7687260875887,14.5483720924235));
#62643=CARTESIAN_POINT('Ctrl Pts',(53.1429662175641,31.2244627281851,14.675074922789));
#62644=CARTESIAN_POINT('Ctrl Pts',(52.1230938577475,28.6532725178718,14.8017777531545));
#62645=CARTESIAN_POINT('Ctrl Pts',(53.7246537356544,26.3980198301654,14.9284805835199));
#62646=CARTESIAN_POINT('Ctrl Pts',(56.488307073099,26.5136872774414,15.0551834138854));
#62647=CARTESIAN_POINT('Ctrl Pts',(57.8958174054756,28.8948788682595,15.1818862442508));
#62648=CARTESIAN_POINT('Ctrl Pts',(56.6646635875745,31.3718566648084,15.3085890746163));
#62649=CARTESIAN_POINT('Ctrl Pts',(53.9166709929956,31.6876024930737,15.4352919049817));
#62650=CARTESIAN_POINT('Ctrl Pts',(52.1558060426984,29.5544092634894,15.5619947353472));
#62651=CARTESIAN_POINT('Ctrl Pts',(52.986566039947,26.9160392070151,15.6886975657126));
#62652=CARTESIAN_POINT('Ctrl Pts',(55.6519638148733,26.1765708646597,15.8154003960781));
#62653=CARTESIAN_POINT('Ctrl Pts',(57.7232932129982,28.0098065975625,15.9421032264435));
#62654=CARTESIAN_POINT('Ctrl Pts',(57.3131622268308,30.7453049620501,16.068806056809));
#62655=CARTESIAN_POINT('Ctrl Pts',(54.7952815496182,31.8904842594738,16.1955088871744));
#62656=CARTESIAN_POINT('Ctrl Pts',(52.463939994279,30.4018589606574,16.3222117175399));
#62657=CARTESIAN_POINT('Ctrl Pts',(52.4434522266802,27.6358620374293,16.4489145479053));
#62658=CARTESIAN_POINT('Ctrl Pts',(54.7524866676209,26.1128654259824,16.5756173782708));
#62659=CARTESIAN_POINT('Ctrl Pts',(57.2870548579027,27.2206211827898,16.7023202086362));
#62660=CARTESIAN_POINT('Ctrl Pts',(57.7376623496078,29.9497440485375,16.8290230390017));
#62661=CARTESIAN_POINT('Ctrl Pts',(55.6937163229126,31.8134616687487,16.9557258693671));
#62662=CARTESIAN_POINT('Ctrl Pts',(53.0176571014176,31.1135575531868,17.0824286997326));
#62663=CARTESIAN_POINT('Ctrl Pts',(52.1479055325239,28.4877832033359,17.209131530098));
#62664=CARTESIAN_POINT('Ctrl Pts',(53.8769778433068,26.3287399726403,17.3358343604635));
#62665=CARTESIAN_POINT('Ctrl Pts',(56.6293461323619,26.6037445713885,17.4625371908289));
#62666=CARTESIAN_POINT('Ctrl Pts',(57.8970568529781,29.062213252654,17.5892400211944));
#62667=CARTESIAN_POINT('Ctrl Pts',(56.5249740407513,31.4639933184218,17.7159428515598));
#62668=CARTESIAN_POINT('Ctrl Pts',(53.7633373416581,31.6205866457067,17.8426456819253));
#62669=CARTESIAN_POINT('Ctrl Pts',(52.1285456626905,29.3893056471977,17.9693485122907));
#62670=CARTESIAN_POINT('Ctrl Pts',(53.1102185455736,26.8032899707292,18.0960513426562));
#62671=CARTESIAN_POINT('Ctrl Pts',(55.8138572424009,26.2189129306717,18.2227541730216));
#62672=CARTESIAN_POINT('Ctrl Pts',(57.7759105323216,28.1686579436003,18.3494570033871));
#62673=CARTESIAN_POINT('Ctrl Pts',(57.2085586214295,30.8759204977563,18.4761598337526));
#62674=CARTESIAN_POINT('Ctrl Pts',(54.6287716560576,31.8738473193346,18.602862664118));
#62675=CARTESIAN_POINT('Ctrl Pts',(52.3872473590691,30.2531290976998,18.7295654944835));
#62676=CARTESIAN_POINT('Ctrl Pts',(52.5264590553553,27.490561662949,18.8562683248489));
#62677=CARTESIAN_POINT('Ctrl Pts',(54.9195572717431,26.1033920069047,18.9829711552144));
#62678=CARTESIAN_POINT('Ctrl Pts',(57.3859547724023,27.3556068833019,19.1096739855798));
#62679=CARTESIAN_POINT('Ctrl Pts',(57.6782741318717,30.1061901160017,19.2363768159453));
#62680=CARTESIAN_POINT('Ctrl Pts',(55.530154421177,31.8488146987648,19.3630796463107));
#62681=CARTESIAN_POINT('Ctrl Pts',(52.8989588567946,30.9956039218132,19.4897824766762));
#62682=CARTESIAN_POINT('Ctrl Pts',(52.1822285941116,28.3240020692746,19.6164853070416));
#62683=CARTESIAN_POINT('Ctrl Pts',(54.033047092729,26.2683684411494,19.7431881374071));
#62684=CARTESIAN_POINT('Ctrl Pts',(56.7649515212204,26.7017930846051,19.8698909677725));
#62685=CARTESIAN_POINT('Ctrl Pts',(57.8886349695947,29.2293401634538,19.996593798138));
#62686=CARTESIAN_POINT('Ctrl Pts',(56.3801988917198,31.5479128551569,20.1232966285034));
#62687=CARTESIAN_POINT('Ctrl Pts',(53.6141278092525,31.5448314618743,20.2499994588689));
#62688=CARTESIAN_POINT('Ctrl Pts',(52.1108612323695,29.222903744055,20.3767022892343));
#62689=CARTESIAN_POINT('Ctrl Pts',(53.2401732414635,26.6978664942751,20.5034051195998));
#62690=CARTESIAN_POINT('Ctrl Pts',(55.9730365556825,26.2705295822934,20.6301079499652));
#62691=CARTESIAN_POINT('Ctrl Pts',(57.8192705283958,28.3302817142776,20.7568107803307));
#62692=CARTESIAN_POINT('Ctrl Pts',(57.096589743788,31.0002800668915,20.8835136106961));
#62693=CARTESIAN_POINT('Ctrl Pts',(54.4634997615441,31.847626450769,21.0102164410616));
#62694=CARTESIAN_POINT('Ctrl Pts',(52.3192679391206,30.1002201992904,21.136919271427));
#62695=CARTESIAN_POINT('Ctrl Pts',(52.6177148327956,27.3502950867379,21.2636221017925));
#62696=CARTESIAN_POINT('Ctrl Pts',(55.0868961587425,26.1035784106085,21.3903249321579));
#62697=CARTESIAN_POINT('Ctrl Pts',(57.4768977873141,27.4960764560288,21.5170277625234));
#62698=CARTESIAN_POINT('Ctrl Pts',(57.609954259127,30.2589471314825,21.6437305928888));
#62699=CARTESIAN_POINT('Ctrl Pts',(55.3648243972843,31.8746673638808,21.7704334232543));
#62700=CARTESIAN_POINT('Ctrl Pts',(52.7872675667032,30.8709950298697,21.8971362536197));
#62701=CARTESIAN_POINT('Ctrl Pts',(52.2259481112485,28.1624756293933,22.0238390839852));
#62702=CARTESIAN_POINT('Ctrl Pts',(54.1923419291723,26.2171059332353,22.1505419143506));
#62703=CARTESIAN_POINT('Ctrl Pts',(56.894669215097,26.8075070798911,22.2772447447161));
#62704=CARTESIAN_POINT('Ctrl Pts',(57.8705833628646,29.395699817874,22.4039475750815));
#62705=CARTESIAN_POINT('Ctrl Pts',(56.2308140472889,31.6233401849381,22.530650405447));
#62706=CARTESIAN_POINT('Ctrl Pts',(53.4695535133207,31.4605802263176,22.6573532358124));
#62707=CARTESIAN_POINT('Ctrl Pts',(52.1027852305065,29.0557768047726,22.7840560661779));
#62708=CARTESIAN_POINT('Ctrl Pts',(53.3760486654888,26.6000844521299,22.9107588965434));
#62709=CARTESIAN_POINT('Ctrl Pts',(56.1288691699566,26.3313190323434,23.0374617269088));
#62710=CARTESIAN_POINT('Ctrl Pts',(57.8534279746937,28.4940010520624,23.1641645572743));
#62711=CARTESIAN_POINT('Ctrl Pts',(56.9772382162707,31.1182392339781,23.2908673876397));
#62712=CARTESIAN_POINT('Ctrl Pts',(54.3007838883385,31.8113778822148,23.4175702180052));
#62713=CARTESIAN_POINT('Ctrl Pts',(52.2587135542228,29.9447003610909,23.5442730483706));
#62714=CARTESIAN_POINT('Ctrl Pts',(52.7200168224909,27.2132689961283,23.6709758787361));
#62715=CARTESIAN_POINT('Ctrl Pts',(54.4042650983531,26.4844591653022,23.755444432313));
#62716=CARTESIAN_POINT('Ctrl Pts',(55.215028655103,26.5557857257648,23.7976787091015));
#62717=CARTESIAN_POINT('Ctrl Pts',(56.336854785976,27.1290313811225,4.75449970191464));
#62718=CARTESIAN_POINT('Ctrl Pts',(56.9577434568089,27.5726418515725,4.79675140782461));
#62719=CARTESIAN_POINT('Ctrl Pts',(57.7122609590011,29.1187488755531,4.88123739052305));
#62720=CARTESIAN_POINT('Ctrl Pts',(56.3745377635746,31.3440493270392,5.00795765001001));
#62721=CARTESIAN_POINT('Ctrl Pts',(53.7830010793689,31.4269778347293,5.13466048037544));
#62722=CARTESIAN_POINT('Ctrl Pts',(52.3011791350529,29.3014763218384,5.26136331074091));
#62723=CARTESIAN_POINT('Ctrl Pts',(53.2781156031241,26.899735803426,5.38806614110635));
#62724=CARTESIAN_POINT('Ctrl Pts',(55.8242360156779,26.4125345931323,5.51476897147182));
#62725=CARTESIAN_POINT('Ctrl Pts',(57.6192089378726,28.2826287272744,5.64147180183725));
#62726=CARTESIAN_POINT('Ctrl Pts',(57.0276164652357,30.8065940011404,5.76817463220272));
#62727=CARTESIAN_POINT('Ctrl Pts',(54.5884358028779,31.6842898360794,5.89487746256816));
#62728=CARTESIAN_POINT('Ctrl Pts',(52.5242857237017,30.1161181229829,6.02158029293361));
#62729=CARTESIAN_POINT('Ctrl Pts',(52.7159953816362,27.5309143173537,6.14828312329906));
#62730=CARTESIAN_POINT('Ctrl Pts',(54.9888899979691,26.2843528255842,6.27498595366452));
#62731=CARTESIAN_POINT('Ctrl Pts',(57.2719061761293,27.5122776130781,6.40168878402996));
#62732=CARTESIAN_POINT('Ctrl Pts',(57.4847660563198,30.0958162368193,6.52839161439542));
#62733=CARTESIAN_POINT('Ctrl Pts',(55.4335106298776,31.6808470373252,6.65509444476087));
#62734=CARTESIAN_POINT('Ctrl Pts',(52.9872412629635,30.8230952769617,6.78179727512633));
#62735=CARTESIAN_POINT('Ctrl Pts',(52.3749942858467,28.3041415620556,6.90850010549177));
#62736=CARTESIAN_POINT('Ctrl Pts',(54.1546483467435,26.4192531776336,7.03520293585723));
#62737=CARTESIAN_POINT('Ctrl Pts',(56.7045854381815,26.8859370117407,7.16190576622267));
#62738=CARTESIAN_POINT('Ctrl Pts',(57.7013070437574,29.2789516952854,7.28860859658814));
#62739=CARTESIAN_POINT('Ctrl Pts',(56.2366020184702,31.4177860114852,7.41531142695358));
#62740=CARTESIAN_POINT('Ctrl Pts',(53.6451072323636,31.353537629316,7.54201425731903));
#62741=CARTESIAN_POINT('Ctrl Pts',(52.2881885491009,29.1447495460208,7.66871708768449));
#62742=CARTESIAN_POINT('Ctrl Pts',(53.4022680881541,26.8040659141131,7.79541991804993));
#62743=CARTESIAN_POINT('Ctrl Pts',(55.9721983683126,26.4643138780574,7.92212274841539));
#62744=CARTESIAN_POINT('Ctrl Pts',(57.6562630632586,28.4350749485684,8.04882557878084));
#62745=CARTESIAN_POINT('Ctrl Pts',(56.9199451381163,30.9205948144127,8.17552840914629));
#62746=CARTESIAN_POINT('Ctrl Pts',(54.4341762991682,31.656071782673,8.30223123951175));
#62747=CARTESIAN_POINT('Ctrl Pts',(52.4639851039711,29.9713404254074,8.42893406987719));
#62748=CARTESIAN_POINT('Ctrl Pts',(52.8046065926559,27.4015252389023,8.55563690024265));
#62749=CARTESIAN_POINT('Ctrl Pts',(55.1456670139649,26.2882376770822,8.6823397306081));
#62750=CARTESIAN_POINT('Ctrl Pts',(57.3539958870469,27.645903571127,8.80904256097356));
#62751=CARTESIAN_POINT('Ctrl Pts',(57.4173675037376,30.2374199476299,8.93574539133899));
#62752=CARTESIAN_POINT('Ctrl Pts',(55.2780377491013,31.7014012632341,9.06244822170446));
#62753=CARTESIAN_POINT('Ctrl Pts',(52.8853604458274,30.7038701038671,9.18915105206991));
#62754=CARTESIAN_POINT('Ctrl Pts',(52.4195392943965,28.1537752533991,9.31585388243536));
#62755=CARTESIAN_POINT('Ctrl Pts',(54.3050297768413,26.3747590274706,9.44255671280081));
#62756=CARTESIAN_POINT('Ctrl Pts',(56.8237760059684,26.9878581424317,9.56925954316626));
#62757=CARTESIAN_POINT('Ctrl Pts',(57.68070047935,29.4344176733702,9.69596237353171));
#62758=CARTESIAN_POINT('Ctrl Pts',(56.0949749986577,31.4851365208452,9.82266520389716));
#62759=CARTESIAN_POINT('Ctrl Pts',(53.5115100648683,31.2714029778829,9.94936803426261));
#62760=CARTESIAN_POINT('Ctrl Pts',(52.2843547597365,28.9879707041789,10.0760708646281));
#62761=CARTESIAN_POINT('Ctrl Pts',(53.5316910184738,26.7154995054294,10.2027736949935));
#62762=CARTESIAN_POINT('Ctrl Pts',(56.1169480534857,26.5246614735075,10.329476525359));
#62763=CARTESIAN_POINT('Ctrl Pts',(57.6844438232736,28.5893479153682,10.4561793557244));
#62764=CARTESIAN_POINT('Ctrl Pts',(56.8058787100404,31.0282198745568,10.5828821860899));
#62765=CARTESIAN_POINT('Ctrl Pts',(54.2817998282517,31.6189811546143,10.7095850164553));
#62766=CARTESIAN_POINT('Ctrl Pts',(52.4121437848409,29.8233310297726,10.8362878468208));
#62767=CARTESIAN_POINT('Ctrl Pts',(52.9005381516877,27.277462998248,10.9629906771862));
#62768=CARTESIAN_POINT('Ctrl Pts',(55.3019587692717,26.3011679050775,11.0896935075517));
#62769=CARTESIAN_POINT('Ctrl Pts',(57.428235043213,27.7840442648531,11.2163963379172));
#62770=CARTESIAN_POINT('Ctrl Pts',(57.34190746138,30.3748975297296,11.3430991682826));
#62771=CARTESIAN_POINT('Ctrl Pts',(55.1216375771333,31.7129463825798,11.469801998648));
#62772=CARTESIAN_POINT('Ctrl Pts',(52.7905317287469,30.5789628663303,11.5965048290135));
#62773=CARTESIAN_POINT('Ctrl Pts',(52.4726898062928,28.0062309324054,11.723207659379));
#62774=CARTESIAN_POINT('Ctrl Pts',(54.4577288569815,26.3390197703904,11.8499104897444));
#62775=CARTESIAN_POINT('Ctrl Pts',(56.9368844987602,27.0964895026856,11.9766133201099));
#62776=CARTESIAN_POINT('Ctrl Pts',(57.6511541085528,29.5884349306662,12.1033161504753));
#62777=CARTESIAN_POINT('Ctrl Pts',(55.9496963696971,31.5441993986927,12.2300189808408));
#62778=CARTESIAN_POINT('Ctrl Pts',(53.3828768301873,31.1816934772279,12.3567218112062));
#62779=CARTESIAN_POINT('Ctrl Pts',(52.2895773153514,28.831231977359,12.4834246415716));
#62780=CARTESIAN_POINT('Ctrl Pts',(53.6660105801299,26.634551627577,12.6101274719371));
#62781=CARTESIAN_POINT('Ctrl Pts',(56.2579728531963,26.5932640203909,12.7368303023026));
#62782=CARTESIAN_POINT('Ctrl Pts',(57.7036722909489,28.7449903568908,12.863533132668));
#62783=CARTESIAN_POINT('Ctrl Pts',(56.6857898969414,31.1290810689813,12.9902359630335));
#62784=CARTESIAN_POINT('Ctrl Pts',(54.1318184672272,31.5731565442227,13.1169387933989));
#62785=CARTESIAN_POINT('Ctrl Pts',(52.3689326502071,29.6725759256601,13.2436416237644));
#62786=CARTESIAN_POINT('Ctrl Pts',(53.0034711596436,27.1591452081848,13.3703444541298));
#62787=CARTESIAN_POINT('Ctrl Pts',(55.4572435289504,26.3230984085781,13.4970472844953));
#62788=CARTESIAN_POINT('Ctrl Pts',(57.4943763319966,27.9262400224913,13.6237501148607));
#62789=CARTESIAN_POINT('Ctrl Pts',(57.2586374435837,30.5077899964403,13.7504529452262));
#62790=CARTESIAN_POINT('Ctrl Pts',(54.9648317586977,31.7154441569895,13.8771557755916));
#62791=CARTESIAN_POINT('Ctrl Pts',(52.7030713185765,30.4487899804244,14.0038586059571));
#62792=CARTESIAN_POINT('Ctrl Pts',(52.5342685891023,27.8620007099138,14.1305614363225));
#62793=CARTESIAN_POINT('Ctrl Pts',(54.6122363451726,26.3121545574719,14.257264266688));
#62794=CARTESIAN_POINT('Ctrl Pts',(57.0435337182411,27.2114688380306,14.3839670970534));
#62795=CARTESIAN_POINT('Ctrl Pts',(57.6127664625076,29.7404898293159,14.5106699274189));
#62796=CARTESIAN_POINT('Ctrl Pts',(55.8012506193009,31.5947776821905,14.6373727577843));
#62797=CARTESIAN_POINT('Ctrl Pts',(53.2596365038281,31.0847082952096,14.7640755881498));
#62798=CARTESIAN_POINT('Ctrl Pts',(52.3038387996787,28.675056071288,14.8907784185152));
#62799=CARTESIAN_POINT('Ctrl Pts',(53.804778833622,26.5614922312271,15.0174812488807));
#62800=CARTESIAN_POINT('Ctrl Pts',(56.3948024670389,26.6698927379054,15.1441840792461));
#62801=CARTESIAN_POINT('Ctrl Pts',(57.7138843416507,28.9014832244368,15.2708869096116));
#62802=CARTESIAN_POINT('Ctrl Pts',(56.5600791803697,31.2228420380001,15.3975897399771));
#62803=CARTESIAN_POINT('Ctrl Pts',(53.9847323856103,31.518750770937,15.5242925703425));
#62804=CARTESIAN_POINT('Ctrl Pts',(52.3344958039333,29.5195778629568,15.6509954007079));
#62805=CARTESIAN_POINT('Ctrl Pts',(53.1130623475071,27.0469664440852,15.7776982310734));
#62806=CARTESIAN_POINT('Ctrl Pts',(55.6110034372893,26.3539560520383,15.9044010614389));
#62807=CARTESIAN_POINT('Ctrl Pts',(57.5521991802746,28.0720166385492,16.0311038918043));
#62808=CARTESIAN_POINT('Ctrl Pts',(57.1678351456911,30.6356541676133,16.1578067221698));
#62809=CARTESIAN_POINT('Ctrl Pts',(54.8081432220527,31.7088862566892,16.2845095525352));
#62810=CARTESIAN_POINT('Ctrl Pts',(52.6232708851051,30.3137855568301,16.4112123829007));
#62811=CARTESIAN_POINT('Ctrl Pts',(52.604070285103,27.7215655761057,16.5379152132661));
#62812=CARTESIAN_POINT('Ctrl Pts',(54.7680369778069,26.2942529809203,16.6646180436316));
#62813=CARTESIAN_POINT('Ctrl Pts',(57.1433680022858,27.3324127064224,16.791320873997));
#62814=CARTESIAN_POINT('Ctrl Pts',(57.5656655593267,29.8900752847982,16.9180237043625));
#62815=CARTESIAN_POINT('Ctrl Pts',(55.6501327959216,31.6367026989388,17.0447265347279));
#62816=CARTESIAN_POINT('Ctrl Pts',(53.142200077231,30.9807708655682,17.1714293650934));
#62817=CARTESIAN_POINT('Ctrl Pts',(52.32709165241,28.519963813544,17.2981321954588));
#62818=CARTESIAN_POINT('Ctrl Pts',(53.9475330037683,26.4965649605458,17.4248350258243));
#62819=CARTESIAN_POINT('Ctrl Pts',(56.5269805849585,26.7542920786345,17.5515378561897));
#62820=CARTESIAN_POINT('Ctrl Pts',(57.7150459194364,29.0583046334003,17.6782406865552));
#62821=CARTESIAN_POINT('Ctrl Pts',(56.4291657902164,31.3091901002298,17.8049435169206));
#62822=CARTESIAN_POINT('Ctrl Pts',(53.8410320975238,31.4559452713678,17.9316463472861));
#62823=CARTESIAN_POINT('Ctrl Pts',(52.3089480886971,29.3648470715205,18.0583491776515));
#62824=CARTESIAN_POINT('Ctrl Pts',(53.2289462420482,26.9413008084306,18.185052008017));
#62825=CARTESIAN_POINT('Ctrl Pts',(55.7627257237678,26.3936379289848,18.3117548383824));
#62826=CARTESIAN_POINT('Ctrl Pts',(57.6015107559083,28.2208879658114,18.4384576687479));
#62827=CARTESIAN_POINT('Ctrl Pts',(57.0698033822789,30.7580636318493,18.5651604991133));
#62828=CARTESIAN_POINT('Ctrl Pts',(54.6520945043367,31.6932945514762,18.6918633294788));
#62829=CARTESIAN_POINT('Ctrl Pts',(52.5513965530351,30.1743998188159,18.8185661598443));
#62830=CARTESIAN_POINT('Ctrl Pts',(52.6818621141615,27.5853938650053,18.9452689902097));
#62831=CARTESIAN_POINT('Ctrl Pts',(54.9246111787976,26.2853747403073,19.0719718205751));
#62832=CARTESIAN_POINT('Ctrl Pts',(57.2360544157466,27.4589177748269,19.1986746509406));
#62833=CARTESIAN_POINT('Ctrl Pts',(57.5100084747716,30.0366924478834,19.325377481306));
#62834=CARTESIAN_POINT('Ctrl Pts',(55.4968468590487,31.6698346341256,19.4520803116715));
#62835=CARTESIAN_POINT('Ctrl Pts',(53.0309591865401,30.8702278069414,19.578783142037));
#62836=CARTESIAN_POINT('Ctrl Pts',(52.3592583281211,28.3664724178689,19.7054859724024));
#62837=CARTESIAN_POINT('Ctrl Pts',(54.093797022839,26.4399863400551,19.8321888027679));
#62838=CARTESIAN_POINT('Ctrl Pts',(56.6540664090754,26.8461805810787,19.9588916331333));
#62839=CARTESIAN_POINT('Ctrl Pts',(57.7071531505767,29.2149316035369,20.0855944634988));
#62840=CARTESIAN_POINT('Ctrl Pts',(56.2934863066709,31.3878372954132,20.2122972938642));
#62841=CARTESIAN_POINT('Ctrl Pts',(53.7011968258471,31.3849494942125,20.3390001242296));
#62842=CARTESIAN_POINT('Ctrl Pts',(52.2923747030794,29.2088995596001,20.4657029545951));
#62843=CARTESIAN_POINT('Ctrl Pts',(53.3507363844905,26.8425006833086,20.5924057849606));
#62844=CARTESIAN_POINT('Ctrl Pts',(55.9119044133541,26.4420117050176,20.719108615326));
#62845=CARTESIAN_POINT('Ctrl Pts',(57.6421466102883,28.3723575369419,20.8458114456915));
#62846=CARTESIAN_POINT('Ctrl Pts',(56.9648690783381,30.8746101678194,20.9725142760569));
#62847=CARTESIAN_POINT('Ctrl Pts',(54.4972060069519,31.6687210391787,21.0992171064224));
#62848=CARTESIAN_POINT('Ctrl Pts',(52.4876880184416,30.0310975980655,21.2259199367878));
#62849=CARTESIAN_POINT('Ctrl Pts',(52.7673846422782,27.453939698,21.3526227671533));
#62850=CARTESIAN_POINT('Ctrl Pts',(55.0814368074849,26.2855494329837,21.4793255975187));
#62851=CARTESIAN_POINT('Ctrl Pts',(57.3212838310008,27.5905621848581,21.6060284278842));
#62852=CARTESIAN_POINT('Ctrl Pts',(57.4459808767212,30.1798523279252,21.7327312582496));
#62853=CARTESIAN_POINT('Ctrl Pts',(55.3419038843298,31.6940630757792,21.8594340886151));
#62854=CARTESIAN_POINT('Ctrl Pts',(52.9262850303917,30.7534476121557,21.9861369189805));
#62855=CARTESIAN_POINT('Ctrl Pts',(52.4002311162387,28.215094062615,22.112839749346));
#62856=CARTESIAN_POINT('Ctrl Pts',(54.2430839777112,26.3919444582436,22.2395425797114));
#62857=CARTESIAN_POINT('Ctrl Pts',(56.7756344394286,26.9452529728523,22.3662454100769));
#62858=CARTESIAN_POINT('Ctrl Pts',(57.6902356568308,29.3708395210595,22.4929482404423));
#62859=CARTESIAN_POINT('Ctrl Pts',(56.1534867371489,31.4585258163257,22.6196510708078));
#62860=CARTESIAN_POINT('Ctrl Pts',(53.5657055765741,31.3059914395681,22.7463539011732));
#62861=CARTESIAN_POINT('Ctrl Pts',(52.2848060853352,29.0522725627704,22.8730567315387));
#62862=CARTESIAN_POINT('Ctrl Pts',(53.4780752785037,26.750861910584,22.9997595619041));
#62863=CARTESIAN_POINT('Ctrl Pts',(56.0579466641524,26.4989819878525,23.1264623922696));
#62864=CARTESIAN_POINT('Ctrl Pts',(57.6741580756808,28.5257910187628,23.253165222635));
#62865=CARTESIAN_POINT('Ctrl Pts',(56.8530159480028,30.9851584143716,23.3798680530005));
#62866=CARTESIAN_POINT('Ctrl Pts',(54.3447129458923,31.634749828694,23.5065708833659));
#62867=CARTESIAN_POINT('Ctrl Pts',(52.4309380325199,29.8853484728245,23.6332737137315));
#62868=CARTESIAN_POINT('Ctrl Pts',(52.8632593916422,27.3255224293559,23.7599765440968));
#62869=CARTESIAN_POINT('Ctrl Pts',(54.4416928297007,26.6425009155755,23.8444450976738));
#62870=CARTESIAN_POINT('Ctrl Pts',(55.2015192321819,26.7093463027249,23.8866793744623));
#62871=CARTESIAN_POINT('Ctrl Pts',(56.24723486984,27.2544571584588,4.84350036727542));
#62872=CARTESIAN_POINT('Ctrl Pts',(56.8265004779488,27.6683289216268,4.88575207318538));
#62873=CARTESIAN_POINT('Ctrl Pts',(57.5304367233141,29.1107882022024,4.97023805588383));
#62874=CARTESIAN_POINT('Ctrl Pts',(56.2823916603557,31.1869092200421,5.09695831537079));
#62875=CARTESIAN_POINT('Ctrl Pts',(53.8645861119009,31.264278376049,5.22366114573623));
#62876=CARTESIAN_POINT('Ctrl Pts',(52.4821023752731,29.2812659871308,5.35036397610169));
#62877=CARTESIAN_POINT('Ctrl Pts',(53.393547089672,27.0405330711135,5.47706680646714));
#62878=CARTESIAN_POINT('Ctrl Pts',(55.7689809772278,26.5859927990651,5.60376963683258));
#62879=CARTESIAN_POINT('Ctrl Pts',(57.4436227127888,28.3307197794772,5.73047246719804));
#62880=CARTESIAN_POINT('Ctrl Pts',(56.8916893477383,30.6854837619637,5.85717529756349));
#62881=CARTESIAN_POINT('Ctrl Pts',(54.6160261958042,31.5043407252877,5.98387812792894));
#62882=CARTESIAN_POINT('Ctrl Pts',(52.6902523703009,30.0412959256666,6.1105809582944));
#62883=CARTESIAN_POINT('Ctrl Pts',(52.8691102184153,27.6293987130087,6.23728378865985));
#62884=CARTESIAN_POINT('Ctrl Pts',(54.989634788997,26.4664040659876,6.3639866190253));
#62885=CARTESIAN_POINT('Ctrl Pts',(57.1196023933181,27.6120113739534,6.49068944939075));
#62886=CARTESIAN_POINT('Ctrl Pts',(57.3181925975411,30.0223550349936,6.6173922797562));
#62887=CARTESIAN_POINT('Ctrl Pts',(55.4044489945367,31.5011287244771,6.74409511012166));
#62888=CARTESIAN_POINT('Ctrl Pts',(53.1221723498006,30.7008788271698,6.8707979404871));
#62889=CARTESIAN_POINT('Ctrl Pts',(52.5509691145466,28.3507904393347,6.99750077085256));
#62890=CARTESIAN_POINT('Ctrl Pts',(54.2113189328573,26.5922609838778,7.124203601218));
#62891=CARTESIAN_POINT('Ctrl Pts',(56.5903136372207,27.0276593212251,7.25090643158346));
#62892=CARTESIAN_POINT('Ctrl Pts',(57.5202171353705,29.2602513638809,7.37760926194891));
#62893=CARTESIAN_POINT('Ctrl Pts',(56.1537028357381,31.2557027531859,7.50431209231437));
#62894=CARTESIAN_POINT('Ctrl Pts',(53.7359363766226,31.1957614466111,7.63101492267981));
#62895=CARTESIAN_POINT('Ctrl Pts',(52.4699826507158,29.1350458427381,7.75771775304527));
#62896=CARTESIAN_POINT('Ctrl Pts',(53.5093766548059,26.9512766887474,7.88442058341071));
#62897=CARTESIAN_POINT('Ctrl Pts',(55.9070242468225,26.6343009102913,8.01112341377616));
#62898=CARTESIAN_POINT('Ctrl Pts',(57.4781928080136,28.472946328664,8.13782624414162));
#62899=CARTESIAN_POINT('Ctrl Pts',(56.7912360785621,30.7918422019342,8.26452907450708));
#62900=CARTESIAN_POINT('Ctrl Pts',(54.4721079228182,31.4780143504736,8.39123190487252));
#62901=CARTESIAN_POINT('Ctrl Pts',(52.633994176524,29.9062238185945,8.51793473523798));
#62902=CARTESIAN_POINT('Ctrl Pts',(52.9517811213449,27.508683604596,8.64463756560342));
#62903=CARTESIAN_POINT('Ctrl Pts',(55.1359018055727,26.4700284852613,8.77134039596887));
#62904=CARTESIAN_POINT('Ctrl Pts',(57.1961889837133,27.7366793305203,8.89804322633434));
#62905=CARTESIAN_POINT('Ctrl Pts',(57.2553123013122,30.1544659326576,9.02474605669978));
#62906=CARTESIAN_POINT('Ctrl Pts',(55.2593986867151,31.5203050385728,9.15144888706523));
#62907=CARTESIAN_POINT('Ctrl Pts',(53.0271214070709,30.5896462574052,9.27815171743069));
#62908=CARTESIAN_POINT('Ctrl Pts',(52.5925279199782,28.2105043698432,9.40485454779613));
#62909=CARTESIAN_POINT('Ctrl Pts',(54.3516191100807,26.5507496273943,9.53155737816158));
#62910=CARTESIAN_POINT('Ctrl Pts',(56.7015139215443,27.1227478749746,9.65826020852703));
#62911=CARTESIAN_POINT('Ctrl Pts',(57.5009919914385,29.4052952317528,9.7849630388925));
#62912=CARTESIAN_POINT('Ctrl Pts',(56.0215701916583,31.3185382269086,9.91166586925794));
#62913=CARTESIAN_POINT('Ctrl Pts',(53.6112952805514,31.1191329284173,10.0383686996234));
#62914=CARTESIAN_POINT('Ctrl Pts',(52.4664058704783,28.9887771227173,10.1650715299889));
#62915=CARTESIAN_POINT('Ctrl Pts',(53.6301233457291,26.8686475847,10.2917743603543));
#62916=CARTESIAN_POINT('Ctrl Pts',(56.0420702193846,26.6906029306347,10.4184771907198));
#62917=CARTESIAN_POINT('Ctrl Pts',(57.5044843895061,28.6168771622033,10.5451800210852));
#62918=CARTESIAN_POINT('Ctrl Pts',(56.6848164224656,30.8922523057753,10.6718828514507));
#62919=CARTESIAN_POINT('Ctrl Pts',(54.3299464480911,31.4434101996381,10.7985856818161));
#62920=CARTESIAN_POINT('Ctrl Pts',(52.5856281897347,29.7681366596626,10.9252885121816));
#62921=CARTESIAN_POINT('Ctrl Pts',(53.0412816316454,27.3929382340459,11.051991342547));
#62922=CARTESIAN_POINT('Ctrl Pts',(55.2817160923089,26.4820918981314,11.1786941729125));
#62923=CARTESIAN_POINT('Ctrl Pts',(57.2654513039361,27.8655593644377,11.3053970032779));
#62924=CARTESIAN_POINT('Ctrl Pts',(57.1849109405247,30.2827273085489,11.4320998336434));
#62925=CARTESIAN_POINT('Ctrl Pts',(55.1134832513411,31.5310761975464,11.5588026640088));
#62926=CARTESIAN_POINT('Ctrl Pts',(52.9386498065307,30.4731125367757,11.6855054943743));
#62927=CARTESIAN_POINT('Ctrl Pts',(52.6421153340208,28.0728511079328,11.8122083247397));
#62928=CARTESIAN_POINT('Ctrl Pts',(54.4940815669917,26.5174062544863,11.9389111551052));
#62929=CARTESIAN_POINT('Ctrl Pts',(56.8070398603111,27.2240968186954,12.0656139854706));
#62930=CARTESIAN_POINT('Ctrl Pts',(57.4734263468209,29.5489874980123,12.1923168158361));
#62931=CARTESIAN_POINT('Ctrl Pts',(55.8860307345812,31.3736416543992,12.3190196462015));
#62932=CARTESIAN_POINT('Ctrl Pts',(53.4912853457422,31.0354373628656,12.445722476567));
#62933=CARTESIAN_POINT('Ctrl Pts',(52.4712783170154,28.8425458284923,12.5724253069325));
#62934=CARTESIAN_POINT('Ctrl Pts',(53.755438408185,26.7931262812974,12.6991281372979));
#62935=CARTESIAN_POINT('Ctrl Pts',(56.1736410149237,26.7546065079344,12.8258309676634));
#62936=CARTESIAN_POINT('Ctrl Pts',(57.522423821395,28.7620856637776,12.9525337980288));
#62937=CARTESIAN_POINT('Ctrl Pts',(56.572778109295,30.9863519791427,13.0792366283943));
#62938=CARTESIAN_POINT('Ctrl Pts',(54.1900195201569,31.4006575741647,13.2059394587597));
#62939=CARTESIAN_POINT('Ctrl Pts',(52.5453138381343,29.62748785874,13.3326422891252));
#62940=CARTESIAN_POINT('Ctrl Pts',(53.1373142285489,27.2825522182742,13.4593451194906));
#62941=CARTESIAN_POINT('Ctrl Pts',(55.4265908902734,26.5025522270812,13.5860479498561));
#62942=CARTESIAN_POINT('Ctrl Pts',(57.3271586206714,27.9982226193627,13.7127507802215));
#62943=CARTESIAN_POINT('Ctrl Pts',(57.1072231685262,30.406710945485,13.839453610587));
#62944=CARTESIAN_POINT('Ctrl Pts',(54.9671893631805,31.5334065264448,13.9661564409524));
#62945=CARTESIAN_POINT('Ctrl Pts',(52.8570525571963,30.3516661657017,14.0928592713179));
#62946=CARTESIAN_POINT('Ctrl Pts',(52.6995660055283,27.9382897743733,14.2195621016833));
#62947=CARTESIAN_POINT('Ctrl Pts',(54.6382312001043,26.4923420285965,14.3462649320488));
#62948=CARTESIAN_POINT('Ctrl Pts',(56.9065395417823,27.3313681826892,14.4729677624142));
#62949=CARTESIAN_POINT('Ctrl Pts',(57.4376121273402,29.6908489579968,14.5996705927797));
#62950=CARTESIAN_POINT('Ctrl Pts',(55.747536473188,31.4208292767924,14.7263734231451));
#62951=CARTESIAN_POINT('Ctrl Pts',(53.3763067900918,30.9449538622341,14.8530762535106));
#62952=CARTESIAN_POINT('Ctrl Pts',(52.4845837416101,28.6968396247043,14.979779083876));
#62953=CARTESIAN_POINT('Ctrl Pts',(53.8849039315895,26.7249646322888,15.1064819142415));
#62954=CARTESIAN_POINT('Ctrl Pts',(56.3012978609789,26.8260981983693,15.2331847446069));
#62955=CARTESIAN_POINT('Ctrl Pts',(57.5319512778258,28.9080875806142,15.3598875749724));
#62956=CARTESIAN_POINT('Ctrl Pts',(56.4554947731649,31.0738274111919,15.4865904053378));
#62957=CARTESIAN_POINT('Ctrl Pts',(54.052793778225,31.3498990488002,15.6132932357033));
#62958=CARTESIAN_POINT('Ctrl Pts',(52.513185565168,29.4847464624241,15.7399960660687));
#62959=CARTESIAN_POINT('Ctrl Pts',(53.2395586550675,27.1778936811554,15.8666988964342));
#62960=CARTESIAN_POINT('Ctrl Pts',(55.5700430597053,26.531341239417,15.9934017267996));
#62961=CARTESIAN_POINT('Ctrl Pts',(57.3811051475509,28.1342266795359,16.1201045571651));
#62962=CARTESIAN_POINT('Ctrl Pts',(57.0225080645516,30.5260033731763,16.2468073875305));
#62963=CARTESIAN_POINT('Ctrl Pts',(54.8210048944872,31.5272882539046,16.373510217896));
#62964=CARTESIAN_POINT('Ctrl Pts',(52.7826017759313,30.2257121530027,16.5002130482614));
#62965=CARTESIAN_POINT('Ctrl Pts',(52.764688343526,27.8072691147822,16.6269158786269));
#62966=CARTESIAN_POINT('Ctrl Pts',(54.7835872879929,26.475640535858,16.7536187089924));
#62967=CARTESIAN_POINT('Ctrl Pts',(56.9996811466689,27.444204230055,16.8803215393578));
#62968=CARTESIAN_POINT('Ctrl Pts',(57.3936687690455,29.8304065210588,17.0070243697233));
#62969=CARTESIAN_POINT('Ctrl Pts',(55.6065492689305,31.4599437291291,17.1337272000887));
#62970=CARTESIAN_POINT('Ctrl Pts',(53.2667430530446,30.8479841779496,17.2604300304542));
#62971=CARTESIAN_POINT('Ctrl Pts',(52.506277772296,28.5521444237522,17.3871328608196));
#62972=CARTESIAN_POINT('Ctrl Pts',(54.0180881642297,26.6643899484512,17.5138356911851));
#62973=CARTESIAN_POINT('Ctrl Pts',(56.4246150375551,26.9048395858806,17.6405385215505));
#62974=CARTESIAN_POINT('Ctrl Pts',(57.5330349858947,29.0543960141468,17.767241351916));
#62975=CARTESIAN_POINT('Ctrl Pts',(56.3333575396814,31.1543868820377,17.8939441822814));
#62976=CARTESIAN_POINT('Ctrl Pts',(53.9187268533894,31.291303897029,18.0206470126469));
#62977=CARTESIAN_POINT('Ctrl Pts',(52.4893505147037,29.3403884958433,18.1473498430123));
#62978=CARTESIAN_POINT('Ctrl Pts',(53.3476739385227,27.079311646132,18.2740526733778));
#62979=CARTESIAN_POINT('Ctrl Pts',(55.7115942051347,26.5683629272977,18.4007555037432));
#62980=CARTESIAN_POINT('Ctrl Pts',(57.427110979495,28.2731179880225,18.5274583341087));
#62981=CARTESIAN_POINT('Ctrl Pts',(56.9310481431283,30.6402067659422,18.6541611644741));
#62982=CARTESIAN_POINT('Ctrl Pts',(54.6754173526158,31.5127417836177,18.7808639948396));
#62983=CARTESIAN_POINT('Ctrl Pts',(52.7155457470008,30.0956705399321,18.9075668252051));
#62984=CARTESIAN_POINT('Ctrl Pts',(52.8372651729678,27.6802260670616,19.0342696555705));
#62985=CARTESIAN_POINT('Ctrl Pts',(54.9296650858523,26.46735747371,19.160972485936));
#62986=CARTESIAN_POINT('Ctrl Pts',(57.0861540590909,27.5622286663519,19.2876753163014));
#62987=CARTESIAN_POINT('Ctrl Pts',(57.3417428176716,29.9671947797651,19.4143781466669));
#62988=CARTESIAN_POINT('Ctrl Pts',(55.4635392969205,31.4908545694863,19.5410809770323));
#62989=CARTESIAN_POINT('Ctrl Pts',(53.1629595162855,30.7448516920698,19.6677838073978));
#62990=CARTESIAN_POINT('Ctrl Pts',(52.5362880621304,28.4089427664633,19.7944866377632));
#62991=CARTESIAN_POINT('Ctrl Pts',(54.1545469529491,26.6116042389608,19.9211894681287));
#62992=CARTESIAN_POINT('Ctrl Pts',(56.5431812969302,26.9905680775522,20.0478922984941));
#62993=CARTESIAN_POINT('Ctrl Pts',(57.5256713315587,29.20052304362,20.1745951288596));
#62994=CARTESIAN_POINT('Ctrl Pts',(56.2067737216222,31.2277617356693,20.301297959225));
#62995=CARTESIAN_POINT('Ctrl Pts',(53.7882658424417,31.2250675265509,20.4280007895905));
#62996=CARTESIAN_POINT('Ctrl Pts',(52.4738881737893,29.1948953751452,20.5547036199559));
#62997=CARTESIAN_POINT('Ctrl Pts',(53.4612995275174,26.9871348723422,20.6814064503214));
#62998=CARTESIAN_POINT('Ctrl Pts',(55.8507722710256,26.6134938277417,20.8081092806868));
#62999=CARTESIAN_POINT('Ctrl Pts',(57.4650226921806,28.4144333596062,20.9348121110523));
#63000=CARTESIAN_POINT('Ctrl Pts',(56.8331484128879,30.7489402687474,21.0615149414177));
#63001=CARTESIAN_POINT('Ctrl Pts',(54.5309122523596,31.4898156275883,21.1882177717832));
#63002=CARTESIAN_POINT('Ctrl Pts',(52.6561080977626,29.9619749968406,21.3149206021486));
#63003=CARTESIAN_POINT('Ctrl Pts',(52.9170544517607,27.5575843092621,21.441623432514));
#63004=CARTESIAN_POINT('Ctrl Pts',(55.0759774562272,26.4675204553589,21.5683262628795));
#63005=CARTESIAN_POINT('Ctrl Pts',(57.1656698746875,27.6850479136874,21.695029093245));
#63006=CARTESIAN_POINT('Ctrl Pts',(57.2820074943153,30.1007575243678,21.8217319236104));
#63007=CARTESIAN_POINT('Ctrl Pts',(55.3189833713753,31.5134587876777,21.9484347539759));
#63008=CARTESIAN_POINT('Ctrl Pts',(53.0653024940802,30.6359001944415,22.0751375843413));
#63009=CARTESIAN_POINT('Ctrl Pts',(52.5745141212291,28.2677124958368,22.2018404147068));
#63010=CARTESIAN_POINT('Ctrl Pts',(54.2938260262502,26.5667829832518,22.3285432450722));
#63011=CARTESIAN_POINT('Ctrl Pts',(56.6565996637603,27.0829988658134,22.4552460754377));
#63012=CARTESIAN_POINT('Ctrl Pts',(57.5098879507969,29.345979224245,22.5819489058031));
#63013=CARTESIAN_POINT('Ctrl Pts',(56.076159427009,31.2937114477132,22.7086517361686));
#63014=CARTESIAN_POINT('Ctrl Pts',(53.6618576398276,31.1514026528185,22.835354566534));
#63015=CARTESIAN_POINT('Ctrl Pts',(52.4668269401638,29.0487683207684,22.9620573968995));
#63016=CARTESIAN_POINT('Ctrl Pts',(53.5801018915184,26.9016393690381,23.0887602272649));
#63017=CARTESIAN_POINT('Ctrl Pts',(55.9870241583484,26.6666449433616,23.2154630576304));
#63018=CARTESIAN_POINT('Ctrl Pts',(57.4948881766679,28.5575809854631,23.3421658879959));
#63019=CARTESIAN_POINT('Ctrl Pts',(56.728793679735,30.8520775947651,23.4688687183613));
#63020=CARTESIAN_POINT('Ctrl Pts',(54.388642003446,31.4581217751733,23.5955715487267));
#63021=CARTESIAN_POINT('Ctrl Pts',(52.6031625108171,29.8259965845581,23.7222743790922));
#63022=CARTESIAN_POINT('Ctrl Pts',(53.0065019607934,27.4377758625836,23.8489772094577));
#63023=CARTESIAN_POINT('Ctrl Pts',(54.4791205610484,26.8005426658487,23.9334457630346));
#63024=CARTESIAN_POINT('Ctrl Pts',(55.1880098092608,26.8629068796849,23.9756800398231));
#63025=CARTESIAN_POINT('Ctrl Pts',(56.1576149537041,27.3798829357952,4.9325010326362));
#63026=CARTESIAN_POINT('Ctrl Pts',(56.6952574990887,27.764015991681,4.97475273854616));
#63027=CARTESIAN_POINT('Ctrl Pts',(57.3486124876272,29.1028275288519,5.05923872124462));
#63028=CARTESIAN_POINT('Ctrl Pts',(56.1902455571367,31.029769113045,5.18595898073157));
#63029=CARTESIAN_POINT('Ctrl Pts',(53.9461711444331,31.1015789173689,5.312661811097));
#63030=CARTESIAN_POINT('Ctrl Pts',(52.6630256154931,29.261055652423,5.43936464146247));
#63031=CARTESIAN_POINT('Ctrl Pts',(53.5089785762199,27.181330338801,5.56606747182791));
#63032=CARTESIAN_POINT('Ctrl Pts',(55.7137259387776,26.7594510049981,5.69277030219337));
#63033=CARTESIAN_POINT('Ctrl Pts',(57.268036487705,28.3788108316801,5.81947313255882));
#63034=CARTESIAN_POINT('Ctrl Pts',(56.7557622302409,30.5643735227871,5.94617596292426));
#63035=CARTESIAN_POINT('Ctrl Pts',(54.6436165887307,31.3243916144959,6.07287879328973));
#63036=CARTESIAN_POINT('Ctrl Pts',(52.8562190169,29.9664737283503,6.19958162365515));
#63037=CARTESIAN_POINT('Ctrl Pts',(53.0222250551942,27.7278831086637,6.32628445402062));
#63038=CARTESIAN_POINT('Ctrl Pts',(54.9903795800251,26.6484553063909,6.45298728438607));
#63039=CARTESIAN_POINT('Ctrl Pts',(56.9672986105068,27.7117451348286,6.57969011475152));
#63040=CARTESIAN_POINT('Ctrl Pts',(57.1516191387623,29.948893833168,6.70639294511698));
#63041=CARTESIAN_POINT('Ctrl Pts',(55.3753873591959,31.3214104116291,6.83309577548243));
#63042=CARTESIAN_POINT('Ctrl Pts',(53.2571034366377,30.578662377378,6.95979860584789));
#63043=CARTESIAN_POINT('Ctrl Pts',(52.7269439432466,28.397439316614,7.08650143621333));
#63044=CARTESIAN_POINT('Ctrl Pts',(54.267989518971,26.7652687901219,7.21320426657878));
#63045=CARTESIAN_POINT('Ctrl Pts',(56.4760418362601,27.1693816307097,7.33990709694424));
#63046=CARTESIAN_POINT('Ctrl Pts',(57.3391272269835,29.2415510324764,7.46660992730969));
#63047=CARTESIAN_POINT('Ctrl Pts',(56.070803653006,31.0936194948866,7.59331275767514));
#63048=CARTESIAN_POINT('Ctrl Pts',(53.8267655208816,31.0379852639061,7.72001558804059));
#63049=CARTESIAN_POINT('Ctrl Pts',(52.6517767523307,29.1253421394554,7.84671841840603));
#63050=CARTESIAN_POINT('Ctrl Pts',(53.6164852214576,27.098487463382,7.9734212487715));
#63051=CARTESIAN_POINT('Ctrl Pts',(55.8418501253325,26.8042879425251,8.10012407913695));
#63052=CARTESIAN_POINT('Ctrl Pts',(57.3001225527685,28.5108177087598,8.2268269095024));
#63053=CARTESIAN_POINT('Ctrl Pts',(56.6625270190076,30.6630895894556,8.35352973986785));
#63054=CARTESIAN_POINT('Ctrl Pts',(54.5100395464682,31.2999569182742,8.4802325702333));
#63055=CARTESIAN_POINT('Ctrl Pts',(52.8040032490768,29.8411072117814,8.60693540059876));
#63056=CARTESIAN_POINT('Ctrl Pts',(53.0989556500339,27.6158419702898,8.7336382309642));
#63057=CARTESIAN_POINT('Ctrl Pts',(55.1261365971803,26.6518192934402,8.86034106132966));
#63058=CARTESIAN_POINT('Ctrl Pts',(57.0383820803796,27.8274550899138,8.98704389169509));
#63059=CARTESIAN_POINT('Ctrl Pts',(57.0932570988867,30.0715119176853,9.11374672206057));
#63060=CARTESIAN_POINT('Ctrl Pts',(55.2407596243288,31.3392088139115,9.24044955242599));
#63061=CARTESIAN_POINT('Ctrl Pts',(53.1688823683142,30.4754224109433,9.36715238279147));
#63062=CARTESIAN_POINT('Ctrl Pts',(52.76551654556,28.2672334862874,9.49385521315691));
#63063=CARTESIAN_POINT('Ctrl Pts',(54.3982084433201,26.726740227318,9.62055804352238));
#63064=CARTESIAN_POINT('Ctrl Pts',(56.5792518371202,27.2576376075175,9.74726087388781));
#63065=CARTESIAN_POINT('Ctrl Pts',(57.321283503527,29.3761727901356,9.87396370425327));
#63066=CARTESIAN_POINT('Ctrl Pts',(55.948165384659,31.151939932972,10.0006665346187));
#63067=CARTESIAN_POINT('Ctrl Pts',(53.7110804962346,30.9668628789518,10.1273693649842));
#63068=CARTESIAN_POINT('Ctrl Pts',(52.6484569812201,28.9895835412558,10.2540721953497));
#63069=CARTESIAN_POINT('Ctrl Pts',(53.7285556729845,27.0217956639708,10.3807750257151));
#63070=CARTESIAN_POINT('Ctrl Pts',(55.9671923852834,26.856544387762,10.5074778560806));
#63071=CARTESIAN_POINT('Ctrl Pts',(57.3245249557388,28.6444064090384,10.634180686446));
#63072=CARTESIAN_POINT('Ctrl Pts',(56.5637541348908,30.7562847369938,10.7608835168115));
#63073=CARTESIAN_POINT('Ctrl Pts',(54.3780930679306,31.267839244662,10.8875863471769));
#63074=CARTESIAN_POINT('Ctrl Pts',(52.7591125946285,29.7129422895528,11.0142891775424));
#63075=CARTESIAN_POINT('Ctrl Pts',(53.1820251116031,27.5084134698438,11.1409920079078));
#63076=CARTESIAN_POINT('Ctrl Pts',(55.2614734153462,26.6630158911854,11.2676948382733));
#63077=CARTESIAN_POINT('Ctrl Pts',(57.1026675646594,27.9470744640223,11.3943976686387));
#63078=CARTESIAN_POINT('Ctrl Pts',(57.0279144196693,30.1905570873682,11.5211004990042));
#63079=CARTESIAN_POINT('Ctrl Pts',(55.1053289255489,31.3492060125132,11.6478033293696));
#63080=CARTESIAN_POINT('Ctrl Pts',(53.0867678843146,30.367262207221,11.7745061597351));
#63081=CARTESIAN_POINT('Ctrl Pts',(52.8115408617487,28.1394712834602,11.9012089901005));
#63082=CARTESIAN_POINT('Ctrl Pts',(54.5304342770019,26.6957927385822,12.027911820466));
#63083=CARTESIAN_POINT('Ctrl Pts',(56.677195221862,27.3517041347052,12.1546146508314));
#63084=CARTESIAN_POINT('Ctrl Pts',(57.295698585089,29.5095400653584,12.2813174811969));
#63085=CARTESIAN_POINT('Ctrl Pts',(55.8223650994653,31.2030839101057,12.4080203115623));
#63086=CARTESIAN_POINT('Ctrl Pts',(53.5996938612971,30.8891812485032,12.5347231419278));
#63087=CARTESIAN_POINT('Ctrl Pts',(52.6529793186795,28.8538596796258,12.6614259722933));
#63088=CARTESIAN_POINT('Ctrl Pts',(53.8448662362403,26.9517009350177,12.7881288026587));
#63089=CARTESIAN_POINT('Ctrl Pts',(56.0893091766512,26.9159489954782,12.9148316330242));
#63090=CARTESIAN_POINT('Ctrl Pts',(57.341175351841,28.7791809706643,13.0415344633896));
#63091=CARTESIAN_POINT('Ctrl Pts',(56.4597663216486,30.843622889304,13.1682372937551));
#63092=CARTESIAN_POINT('Ctrl Pts',(54.2482205730866,31.2281586041067,13.2949401241205));
#63093=CARTESIAN_POINT('Ctrl Pts',(52.7216950260614,29.5823997918197,13.421642954486));
#63094=CARTESIAN_POINT('Ctrl Pts',(53.2711572974542,27.4059592283635,13.5483457848514));
#63095=CARTESIAN_POINT('Ctrl Pts',(55.3959382515963,26.6820060455842,13.6750486152169));
#63096=CARTESIAN_POINT('Ctrl Pts',(57.1599409093461,28.0702052162341,13.8017514455823));
#63097=CARTESIAN_POINT('Ctrl Pts',(56.9558088934689,30.3056318945295,13.9284542759478));
#63098=CARTESIAN_POINT('Ctrl Pts',(54.9695469676632,31.3513688959002,14.0551571063132));
#63099=CARTESIAN_POINT('Ctrl Pts',(53.0110337958162,30.254542350979,14.1818599366787));
#63100=CARTESIAN_POINT('Ctrl Pts',(52.8648634219542,28.0145788388328,14.3085627670441));
#63101=CARTESIAN_POINT('Ctrl Pts',(54.6642260550361,26.6725294997212,14.4352655974096));
#63102=CARTESIAN_POINT('Ctrl Pts',(56.7695453653235,27.4512675273478,14.561968427775));
#63103=CARTESIAN_POINT('Ctrl Pts',(57.262457792173,29.641208086678,14.6886712581405));
#63104=CARTESIAN_POINT('Ctrl Pts',(55.693822327075,31.2468808713942,14.8153740885059));
#63105=CARTESIAN_POINT('Ctrl Pts',(53.4929770763557,30.8051994292586,14.9420769188714));
#63106=CARTESIAN_POINT('Ctrl Pts',(52.6653286835415,28.7186231781205,15.0687797492368));
#63107=CARTESIAN_POINT('Ctrl Pts',(53.9650290295572,26.8884370333506,15.1954825796023));
#63108=CARTESIAN_POINT('Ctrl Pts',(56.2077932549187,26.9823036588331,15.3221854099677));
#63109=CARTESIAN_POINT('Ctrl Pts',(57.3500182140011,28.9146919367915,15.4488882403332));
#63110=CARTESIAN_POINT('Ctrl Pts',(56.3509103659602,30.9248127843835,15.5755910706986));
#63111=CARTESIAN_POINT('Ctrl Pts',(54.1208551708396,31.1810473266634,15.7022939010641));
#63112=CARTESIAN_POINT('Ctrl Pts',(52.6918753264028,29.4499150618915,15.8289967314296));
#63113=CARTESIAN_POINT('Ctrl Pts',(53.3660549626277,27.3088209182255,15.955699561795));
#63114=CARTESIAN_POINT('Ctrl Pts',(55.5290826821211,26.7087264267957,16.0824023921605));
#63115=CARTESIAN_POINT('Ctrl Pts',(57.2100111148274,28.1964367205226,16.2091052225259));
#63116=CARTESIAN_POINT('Ctrl Pts',(56.8771809834118,30.4163525787395,16.3358080528913));
#63117=CARTESIAN_POINT('Ctrl Pts',(54.8338665669218,31.3456902511198,16.4625108832568));
#63118=CARTESIAN_POINT('Ctrl Pts',(52.9419326667575,30.1376387491754,16.5892137136222));
#63119=CARTESIAN_POINT('Ctrl Pts',(52.9253064019489,27.8929726534587,16.7159165439877));
#63120=CARTESIAN_POINT('Ctrl Pts',(54.7991375981788,26.6570280907958,16.8426193743531));
#63121=CARTESIAN_POINT('Ctrl Pts',(56.855994291052,27.5559957536877,16.9693222047186));
#63122=CARTESIAN_POINT('Ctrl Pts',(57.2216719787645,29.7707377573194,17.096025035084));
#63123=CARTESIAN_POINT('Ctrl Pts',(55.5629657419395,31.2831847593193,17.2227278654495));
#63124=CARTESIAN_POINT('Ctrl Pts',(53.391286028858,30.7151974903311,17.3494306958149));
#63125=CARTESIAN_POINT('Ctrl Pts',(52.6854638921822,28.5843250339603,17.4761335261804));
#63126=CARTESIAN_POINT('Ctrl Pts',(54.088643324691,26.8322149363567,17.6028363565458));
#63127=CARTESIAN_POINT('Ctrl Pts',(56.3222494901519,27.0553870931267,17.7295391869113));
#63128=CARTESIAN_POINT('Ctrl Pts',(57.3510240523529,29.0504873948933,17.8562420172768));
#63129=CARTESIAN_POINT('Ctrl Pts',(56.2375492891465,30.9995836638454,17.9829448476422));
#63130=CARTESIAN_POINT('Ctrl Pts',(53.996421609255,31.1266625226902,18.1096476780077));
#63131=CARTESIAN_POINT('Ctrl Pts',(52.6697529407101,29.3159299201662,18.2363505083731));
#63132=CARTESIAN_POINT('Ctrl Pts',(53.4664016349973,27.2173224838335,18.3630533387386));
#63133=CARTESIAN_POINT('Ctrl Pts',(55.6604626865017,26.7430879256107,18.489756169104));
#63134=CARTESIAN_POINT('Ctrl Pts',(57.2527112030815,28.3253480102336,18.6164589994695));
#63135=CARTESIAN_POINT('Ctrl Pts',(56.7922929039775,30.522349900035,18.7431618298349));
#63136=CARTESIAN_POINT('Ctrl Pts',(54.698740200895,31.3321890157593,18.8698646602004));
#63137=CARTESIAN_POINT('Ctrl Pts',(52.8796949409666,30.0169412610481,18.9965674905659));
#63138=CARTESIAN_POINT('Ctrl Pts',(52.992668231774,27.7750582691179,19.1232703209312));
#63139=CARTESIAN_POINT('Ctrl Pts',(54.9347189929068,26.6493402071125,19.2499731512967));
#63140=CARTESIAN_POINT('Ctrl Pts',(56.9362537024352,27.6655395578769,19.3766759816622));
#63141=CARTESIAN_POINT('Ctrl Pts',(57.1734771605715,29.8976971116468,19.5033788120276));
#63142=CARTESIAN_POINT('Ctrl Pts',(55.4302317347922,31.3118745048471,19.6300816423931));
#63143=CARTESIAN_POINT('Ctrl Pts',(53.2949598460309,30.6194755771981,19.7567844727585));
#63144=CARTESIAN_POINT('Ctrl Pts',(52.71331779614,28.4514131150576,19.883487303124));
#63145=CARTESIAN_POINT('Ctrl Pts',(54.2152968830592,26.7832221378665,20.0101901334894));
#63146=CARTESIAN_POINT('Ctrl Pts',(56.4322961847852,27.1349555740258,20.1368929638549));
#63147=CARTESIAN_POINT('Ctrl Pts',(57.3441895125406,29.1861144837031,20.2635957942203));
#63148=CARTESIAN_POINT('Ctrl Pts',(56.1200611365734,31.0676861759256,20.3902986245858));
#63149=CARTESIAN_POINT('Ctrl Pts',(53.8753348590363,31.0651855588891,20.5170014549512));
#63150=CARTESIAN_POINT('Ctrl Pts',(52.6554016444992,29.1808911906904,20.6437042853167));
#63151=CARTESIAN_POINT('Ctrl Pts',(53.5718626705443,27.1317690613758,20.7704071156822));
#63152=CARTESIAN_POINT('Ctrl Pts',(55.7896401286971,26.7849759504659,20.8971099460476));
#63153=CARTESIAN_POINT('Ctrl Pts',(57.2878987740729,28.4565091822705,21.0238127764131));
#63154=CARTESIAN_POINT('Ctrl Pts',(56.7014277474381,30.6232703696753,21.1505156067785));
#63155=CARTESIAN_POINT('Ctrl Pts',(54.5646184977673,31.310910215998,21.277218437144));
#63156=CARTESIAN_POINT('Ctrl Pts',(52.8245281770835,29.8928523956156,21.4039212675094));
#63157=CARTESIAN_POINT('Ctrl Pts',(53.0667242612434,27.6612289205243,21.5306240978748));
#63158=CARTESIAN_POINT('Ctrl Pts',(55.0705181049695,26.6494914777341,21.6573269282403));
#63159=CARTESIAN_POINT('Ctrl Pts',(57.0100559183742,27.7795336425169,21.7840297586058));
#63160=CARTESIAN_POINT('Ctrl Pts',(57.1180341119095,30.0216627208105,21.9107325889712));
#63161=CARTESIAN_POINT('Ctrl Pts',(55.2960628584209,31.3328544995762,22.0374354193367));
#63162=CARTESIAN_POINT('Ctrl Pts',(53.2043199577687,30.5183527767275,22.1641382497021));
#63163=CARTESIAN_POINT('Ctrl Pts',(52.7487971262193,28.3203309290585,22.2908410800676));
#63164=CARTESIAN_POINT('Ctrl Pts',(54.3445680747892,26.7416215082599,22.417543910433));
#63165=CARTESIAN_POINT('Ctrl Pts',(56.5375648880919,27.2207447587746,22.5442467407985));
#63166=CARTESIAN_POINT('Ctrl Pts',(57.3295402447631,29.3211189274305,22.6709495711639));
#63167=CARTESIAN_POINT('Ctrl Pts',(55.998832116869,31.1288970791007,22.7976524015294));
#63168=CARTESIAN_POINT('Ctrl Pts',(53.7580097030809,30.996813866069,22.9243552318949));
#63169=CARTESIAN_POINT('Ctrl Pts',(52.6488477949925,29.0452640787664,23.0510580622602));
#63170=CARTESIAN_POINT('Ctrl Pts',(53.6821285045334,27.0524168274922,23.1777608926258));
#63171=CARTESIAN_POINT('Ctrl Pts',(55.9161016525442,26.8343078988708,23.3044637229911));
#63172=CARTESIAN_POINT('Ctrl Pts',(57.315618277655,28.5893709521635,23.4311665533567));
#63173=CARTESIAN_POINT('Ctrl Pts',(56.6045714114671,30.7189967751585,23.5578693837221));
#63174=CARTESIAN_POINT('Ctrl Pts',(54.4325710609997,31.2814937216525,23.6845722140876));
#63175=CARTESIAN_POINT('Ctrl Pts',(52.7753869891141,29.7666446962917,23.811275044453));
#63176=CARTESIAN_POINT('Ctrl Pts',(53.1497445299447,27.5500292958113,23.9379778748185));
#63177=CARTESIAN_POINT('Ctrl Pts',(54.516548292396,26.9585844161219,24.0224464283954));
#63178=CARTESIAN_POINT('Ctrl Pts',(55.1745003863396,27.016467456645,24.0646807051839));
#63179=CARTESIAN_POINT('Ctrl Pts',(56.1167974000718,31.181218424916,4.9305));
#63180=CARTESIAN_POINT('Ctrl Pts',(56.1036115526316,31.1892689822654,4.9305));
#63181=CARTESIAN_POINT('Ctrl Pts',(56.0904257051915,31.1973195396149,4.9305));
#63182=CARTESIAN_POINT('Ctrl Pts',(56.0772398577513,31.2053700969644,4.9305));
#63183=CARTESIAN_POINT('Origin',(55.,29.,4.6));
#63184=CARTESIAN_POINT('',(53.6096550852048,28.9081480324703,4.7));
#63185=CARTESIAN_POINT('',(53.5566243270259,29.,4.65));
#63186=CARTESIAN_POINT('Ctrl Pts',(53.6096550852048,28.9081480324703,4.7));
#63187=CARTESIAN_POINT('Ctrl Pts',(53.5836070607731,28.9532645342227,4.67698273374721));
#63188=CARTESIAN_POINT('Ctrl Pts',(53.5566243270259,29.,4.65));
#63189=CARTESIAN_POINT('',(54.2252814053341,27.8418519675297,4.7));
#63190=CARTESIAN_POINT('Origin',(55.,29.,4.7));
#63191=CARTESIAN_POINT('',(54.278312163513,27.75,4.64999999999999));
#63192=CARTESIAN_POINT('Ctrl Pts',(54.278312163513,27.75,4.64999999999999));
#63193=CARTESIAN_POINT('Ctrl Pts',(54.2513294297658,27.7967354657773,4.6769827337472));
#63194=CARTESIAN_POINT('Ctrl Pts',(54.2252814053341,27.8418519675297,4.7));
#63195=CARTESIAN_POINT('',(54.3843736798707,27.75,4.7));
#63196=CARTESIAN_POINT('Ctrl Pts',(54.3843736798707,27.75,4.7));
#63197=CARTESIAN_POINT('Ctrl Pts',(54.3322776310074,27.75,4.6769827337472));
#63198=CARTESIAN_POINT('Ctrl Pts',(54.278312163513,27.75,4.64999999999999));
#63199=CARTESIAN_POINT('',(55.6156263201293,27.75,4.7));
#63200=CARTESIAN_POINT('Origin',(55.,29.,4.7));
#63201=CARTESIAN_POINT('',(55.721687836487,27.75,4.64999999999999));
#63202=CARTESIAN_POINT('Ctrl Pts',(55.721687836487,27.75,4.64999999999999));
#63203=CARTESIAN_POINT('Ctrl Pts',(55.6677223689926,27.75,4.6769827337472));
#63204=CARTESIAN_POINT('Ctrl Pts',(55.6156263201293,27.75,4.7));
#63205=CARTESIAN_POINT('',(55.7747185946659,27.8418519675297,4.7));
#63206=CARTESIAN_POINT('Ctrl Pts',(55.7747185946659,27.8418519675297,4.7));
#63207=CARTESIAN_POINT('Ctrl Pts',(55.7486705702342,27.7967354657773,4.6769827337472));
#63208=CARTESIAN_POINT('Ctrl Pts',(55.721687836487,27.75,4.64999999999999));
#63209=CARTESIAN_POINT('',(56.3903449147952,28.9081480324703,4.7));
#63210=CARTESIAN_POINT('Origin',(55.,29.,4.7));
#63211=CARTESIAN_POINT('',(56.4433756729741,29.,4.65));
#63212=CARTESIAN_POINT('Ctrl Pts',(56.4433756729741,29.,4.65));
#63213=CARTESIAN_POINT('Ctrl Pts',(56.4163929392269,28.9532645342227,4.67698273374721));
#63214=CARTESIAN_POINT('Ctrl Pts',(56.3903449147952,28.9081480324703,4.7));
#63215=CARTESIAN_POINT('',(56.3903449147952,29.0918519675297,4.7));
#63216=CARTESIAN_POINT('Ctrl Pts',(56.3903449147952,29.0918519675297,4.7));
#63217=CARTESIAN_POINT('Ctrl Pts',(56.4163929392268,29.0467354657773,4.67698273374722));
#63218=CARTESIAN_POINT('Ctrl Pts',(56.4433756729741,29.,4.65));
#63219=CARTESIAN_POINT('',(55.7747185946659,30.1581480324703,4.7));
#63220=CARTESIAN_POINT('Origin',(55.,29.,4.7));
#63221=CARTESIAN_POINT('',(55.721687836487,30.25,4.65000000000001));
#63222=CARTESIAN_POINT('Ctrl Pts',(55.721687836487,30.25,4.65000000000001));
#63223=CARTESIAN_POINT('Ctrl Pts',(55.7486705702342,30.2032645342227,4.67698273374721));
#63224=CARTESIAN_POINT('Ctrl Pts',(55.7747185946659,30.1581480324703,4.7));
#63225=CARTESIAN_POINT('',(55.6156263201293,30.25,4.7));
#63226=CARTESIAN_POINT('Ctrl Pts',(55.6156263201293,30.25,4.7));
#63227=CARTESIAN_POINT('Ctrl Pts',(55.6677223689926,30.25,4.67698273374721));
#63228=CARTESIAN_POINT('Ctrl Pts',(55.721687836487,30.25,4.65000000000001));
#63229=CARTESIAN_POINT('',(54.3843736798707,30.25,4.7));
#63230=CARTESIAN_POINT('Origin',(55.,29.,4.7));
#63231=CARTESIAN_POINT('',(54.278312163513,30.25,4.65000000000001));
#63232=CARTESIAN_POINT('Ctrl Pts',(54.278312163513,30.25,4.65000000000001));
#63233=CARTESIAN_POINT('Ctrl Pts',(54.3322776310074,30.25,4.67698273374721));
#63234=CARTESIAN_POINT('Ctrl Pts',(54.3843736798707,30.25,4.7));
#63235=CARTESIAN_POINT('',(54.2252814053341,30.1581480324703,4.7));
#63236=CARTESIAN_POINT('Ctrl Pts',(54.2252814053341,30.1581480324703,4.7));
#63237=CARTESIAN_POINT('Ctrl Pts',(54.2513294297658,30.2032645342228,4.67698273374719));
#63238=CARTESIAN_POINT('Ctrl Pts',(54.278312163513,30.25,4.65000000000001));
#63239=CARTESIAN_POINT('',(53.6096550852048,29.0918519675297,4.7));
#63240=CARTESIAN_POINT('Origin',(55.,29.,4.7));
#63241=CARTESIAN_POINT('Ctrl Pts',(53.5566243270259,29.,4.65));
#63242=CARTESIAN_POINT('Ctrl Pts',(53.5836070607731,29.0467354657773,4.67698273374721));
#63243=CARTESIAN_POINT('Ctrl Pts',(53.6096550852048,29.0918519675297,4.7));
#63244=CARTESIAN_POINT('',(53.4066243270259,29.,4.5));
#63245=CARTESIAN_POINT('',(53.5066243270259,29.,4.6));
#63246=CARTESIAN_POINT('Origin',(55.,29.,4.5));
#63247=CARTESIAN_POINT('Origin',(55.,29.,4.6));
#63248=CARTESIAN_POINT('',(56.3903449147952,28.9081480324703,4.5));
#63249=CARTESIAN_POINT('',(56.3903449147952,28.9081480324703,4.6));
#63250=CARTESIAN_POINT('',(55.7747185946659,27.8418519675297,4.5));
#63251=CARTESIAN_POINT('',(55.7747185946659,27.8418519675297,4.6));
#63252=CARTESIAN_POINT('Origin',(55.,29.,4.5));
#63253=CARTESIAN_POINT('Origin',(55.,29.,4.6));
#63254=CARTESIAN_POINT('',(55.7747185946659,30.1581480324703,4.5));
#63255=CARTESIAN_POINT('',(55.7747185946659,30.1581480324703,4.6));
#63256=CARTESIAN_POINT('',(56.3903449147952,29.0918519675297,4.5));
#63257=CARTESIAN_POINT('',(56.3903449147952,29.0918519675297,4.6));
#63258=CARTESIAN_POINT('Origin',(55.,29.,4.5));
#63259=CARTESIAN_POINT('Origin',(55.,29.,4.6));
#63260=CARTESIAN_POINT('',(54.3843736798707,27.75,4.5));
#63261=CARTESIAN_POINT('',(54.3843736798707,27.75,4.6));
#63262=CARTESIAN_POINT('',(55.6156263201293,27.75,4.5));
#63263=CARTESIAN_POINT('Origin',(55.,29.,4.5));
#63264=CARTESIAN_POINT('',(55.6156263201293,27.75,4.6));
#63265=CARTESIAN_POINT('Origin',(55.,29.,4.6));
#63266=CARTESIAN_POINT('',(54.3843736798707,30.25,4.5));
#63267=CARTESIAN_POINT('',(54.3843736798707,30.25,4.6));
#63268=CARTESIAN_POINT('',(55.6156263201293,30.25,4.5));
#63269=CARTESIAN_POINT('',(55.6156263201293,30.25,4.6));
#63270=CARTESIAN_POINT('Origin',(55.,29.,4.5));
#63271=CARTESIAN_POINT('Origin',(55.,29.,4.6));
#63272=CARTESIAN_POINT('',(53.6096550852048,28.9081480324703,4.5));
#63273=CARTESIAN_POINT('',(53.6096550852048,28.9081480324703,4.6));
#63274=CARTESIAN_POINT('',(54.2252814053341,27.8418519675297,4.5));
#63275=CARTESIAN_POINT('Origin',(55.,29.,4.5));
#63276=CARTESIAN_POINT('',(54.2252814053341,27.8418519675297,4.6));
#63277=CARTESIAN_POINT('Origin',(55.,29.,4.6));
#63278=CARTESIAN_POINT('',(54.2252814053341,30.1581480324703,4.5));
#63279=CARTESIAN_POINT('',(54.2252814053341,30.1581480324703,4.6));
#63280=CARTESIAN_POINT('',(53.6096550852048,29.0918519675297,4.5));
#63281=CARTESIAN_POINT('Origin',(55.,29.,4.5));
#63282=CARTESIAN_POINT('',(53.6096550852048,29.0918519675297,4.6));
#63283=CARTESIAN_POINT('Origin',(55.721687836487,30.25,4.5));
#63284=CARTESIAN_POINT('',(56.3708439182435,30.25,4.5));
#63285=CARTESIAN_POINT('',(55.721687836487,30.25,7.));
#63286=CARTESIAN_POINT('',(55.721687836487,30.25,4.5));
#63287=CARTESIAN_POINT('',(54.278312163513,30.25,7.));
#63288=CARTESIAN_POINT('',(55.721687836487,30.25,7.));
#63289=CARTESIAN_POINT('',(54.278312163513,30.25,4.5));
#63290=CARTESIAN_POINT('Origin',(56.4433756729741,29.,4.5));
#63291=CARTESIAN_POINT('',(56.5154537138523,28.8751571710889,4.5));
#63292=CARTESIAN_POINT('',(56.4433756729741,29.,7.));
#63293=CARTESIAN_POINT('',(56.4433756729741,29.,4.5));
#63294=CARTESIAN_POINT('',(56.4433756729741,29.,7.));
#63295=CARTESIAN_POINT('Origin',(55.721687836487,27.75,4.5));
#63296=CARTESIAN_POINT('',(56.1546097956088,28.4998428289111,4.5));
#63297=CARTESIAN_POINT('',(55.721687836487,27.75,7.));
#63298=CARTESIAN_POINT('',(55.721687836487,27.75,4.5));
#63299=CARTESIAN_POINT('',(55.721687836487,27.75,7.));
#63300=CARTESIAN_POINT('Origin',(57.02,29.,4.5));
#63301=CARTESIAN_POINT('Origin',(57.02,29.,4.5));
#63302=CARTESIAN_POINT('Origin',(57.02,29.,4.5));
#63303=CARTESIAN_POINT('',(55.6491560817565,27.75,4.5));
#63304=CARTESIAN_POINT('Origin',(57.02,29.,4.5));
#63305=CARTESIAN_POINT('Origin',(57.02,29.,4.5));
#63306=CARTESIAN_POINT('',(53.9895462861477,28.2501571710889,4.5));
#63307=CARTESIAN_POINT('Origin',(57.02,29.,4.5));
#63308=CARTESIAN_POINT('',(54.3503902043912,30.3748428289111,4.5));
#63309=CARTESIAN_POINT('Origin',(56.4433756729741,29.,7.));
#63310=CARTESIAN_POINT('',(54.278312163513,27.75,7.));
#63311=CARTESIAN_POINT('',(54.278312163513,27.75,7.));
#63312=CARTESIAN_POINT('Origin',(55.,29.,7.));
#63313=CARTESIAN_POINT('Origin',(56.4433756729741,29.,7.));
#63314=CARTESIAN_POINT('Origin',(55.,29.,7.));
#63315=CARTESIAN_POINT('Origin',(56.4433756729741,29.,7.));
#63316=CARTESIAN_POINT('Origin',(55.,29.,7.));
#63317=CARTESIAN_POINT('Origin',(56.4433756729741,29.,7.));
#63318=CARTESIAN_POINT('Origin',(55.,29.,7.));
#63319=CARTESIAN_POINT('Origin',(56.4433756729741,29.,7.));
#63320=CARTESIAN_POINT('',(53.5566243270259,29.,7.));
#63321=CARTESIAN_POINT('',(54.278312163513,30.25,7.));
#63322=CARTESIAN_POINT('Origin',(55.,29.,7.));
#63323=CARTESIAN_POINT('Origin',(56.4433756729741,29.,7.));
#63324=CARTESIAN_POINT('',(53.5566243270259,29.,7.));
#63325=CARTESIAN_POINT('Origin',(55.,29.,7.));
#63326=CARTESIAN_POINT('Origin',(55.,29.,7.));
#63327=CARTESIAN_POINT('',(55.,29.,7.86726760035252));
#63328=CARTESIAN_POINT('',(53.5566243270259,29.,7.));
#63329=CARTESIAN_POINT('Origin',(54.278312163513,27.75,4.5));
#63330=CARTESIAN_POINT('',(54.278312163513,27.75,4.5));
#63331=CARTESIAN_POINT('Origin',(53.5566243270259,29.,4.5));
#63332=CARTESIAN_POINT('',(53.5566243270259,29.,4.5));
#63333=CARTESIAN_POINT('Origin',(54.278312163513,30.25,4.5));
#63334=CARTESIAN_POINT('Origin',(57.02,29.,4.5));
#63335=CARTESIAN_POINT('',(52.98,29.,4.5));
#63336=CARTESIAN_POINT('Origin',(55.,29.,4.5));
#63337=CARTESIAN_POINT('Origin',(55.,29.,4.74));
#63338=CARTESIAN_POINT('',(52.74,29.,4.74));
#63339=CARTESIAN_POINT('Origin',(55.,29.,24.125));
#63340=CARTESIAN_POINT('',(53.25,29.,24.5));
#63341=CARTESIAN_POINT('',(52.875,29.,24.125));
#63342=CARTESIAN_POINT('Origin',(55.,29.,24.5));
#63343=CARTESIAN_POINT('Origin',(55.,29.,24.5));
#81025=UNCERTAINTY_MEASURE_WITH_UNIT(LENGTH_MEASURE(0.01),#81041,
'DISTANCE_ACCURACY_VALUE',
'Maximum model space distance between geometric entities at asserted c
onnectivities');
#81028=UNCERTAINTY_MEASURE_WITH_UNIT(LENGTH_MEASURE(0.01),#81041,
'DISTANCE_ACCURACY_VALUE',
'Maximum model space distance between geometric entities at asserted c
onnectivities');
#81037=(
GEOMETRIC_REPRESENTATION_CONTEXT(3)
GLOBAL_UNCERTAINTY_ASSIGNED_CONTEXT((#81025))
GLOBAL_UNIT_ASSIGNED_CONTEXT((#81041,#81043,#81044))
REPRESENTATION_CONTEXT('','3D')
);
#81040=(
GEOMETRIC_REPRESENTATION_CONTEXT(3)
GLOBAL_UNCERTAINTY_ASSIGNED_CONTEXT((#81028))
GLOBAL_UNIT_ASSIGNED_CONTEXT((#81041,#81043,#81044))
REPRESENTATION_CONTEXT('','3D')
);
#81041=(
LENGTH_UNIT()
NAMED_UNIT(*)
SI_UNIT(.MILLI.,.METRE.)
);
#81043=(
NAMED_UNIT(*)
PLANE_ANGLE_UNIT()
SI_UNIT($,.RADIAN.)
);
#81044=(
NAMED_UNIT(*)
SI_UNIT($,.STERADIAN.)
SOLID_ANGLE_UNIT()
);
#81053=SHAPE_DEFINITION_REPRESENTATION(#81064,#81137);
#81064=PRODUCT_DEFINITION_SHAPE('',$,#81149);
#81137=SHAPE_REPRESENTATION('',(#16363),#81037);
#81140=PRODUCT_DEFINITION_CONTEXT('part definition',#81175,'design');
#81149=PRODUCT_DEFINITION('ISO 4026 - M5 x 20 - 45H',
'ISO 4026 - M5 x 20 - 45H',#81160,#81140);
#81160=PRODUCT_DEFINITION_FORMATION('',$,#81185);
#81175=APPLICATION_CONTEXT(
'Core Data for Automotive Mechanical Design Process');
#81176=PRODUCT_CONTEXT('part definition',#81175,'mechanical');
#81185=PRODUCT('ISO 4026 - M5 x 20 - 45H','ISO 4026 - M5 x 20 - 45H',$,
(#81176));
#81196=PRESENTATION_STYLE_ASSIGNMENT((#81207));
#81207=SURFACE_STYLE_USAGE(.BOTH.,#81218);
#81218=SURFACE_SIDE_STYLE('',(#81229));
#81229=SURFACE_STYLE_FILL_AREA(#81240);
#81240=FILL_AREA_STYLE('Opaque(196,201,207)',(#81251));
#81251=FILL_AREA_STYLE_COLOUR('Opaque(196,201,207)',#81262);
#81262=COLOUR_RGB('Opaque(196,201,207)', 0.66274510, 0.83137255, 0.94901961);
ENDSEC;
END-ISO-10303-21;
